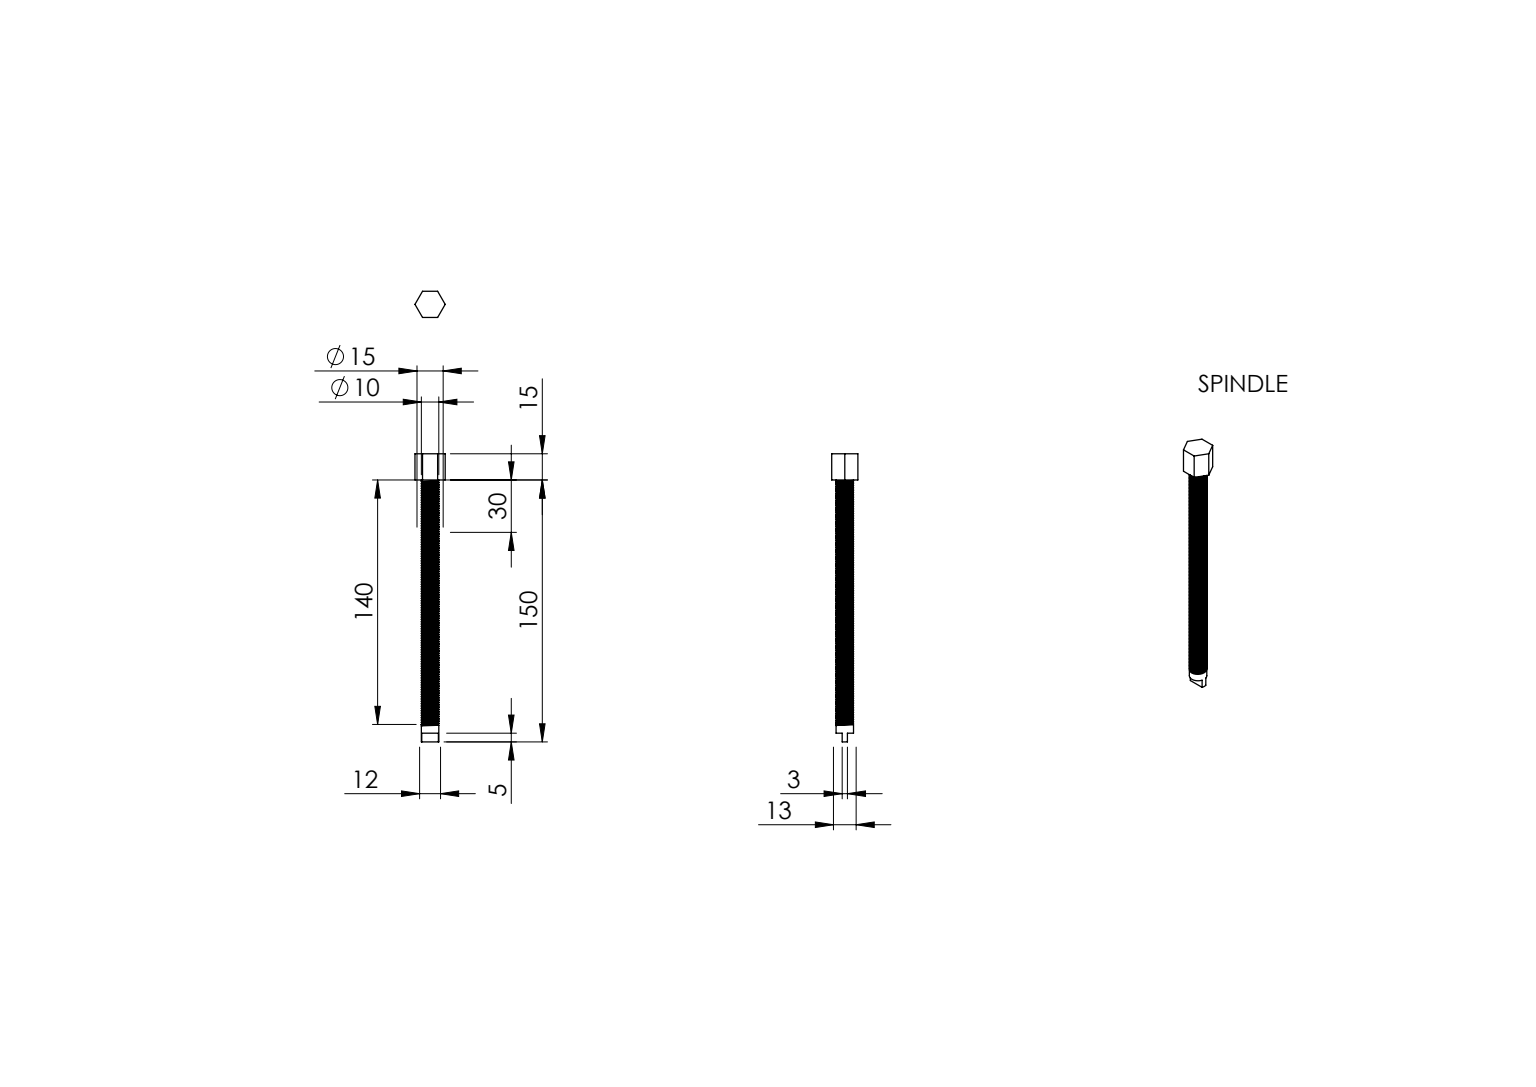
ISO-10303-21;
HEADER;
FILE_DESCRIPTION (('STEP AP214'),
    '1' );
FILE_NAME ('spindle.step',
    '2026-10-25T05:52:03',
    ( '' ),
    ( '' ),
    'SwSTEP 2.0',
    'SolidWorks 2026',
    '' );
FILE_SCHEMA (( 'AUTOMOTIVE_DESIGN' ));
ENDSEC;

DATA;
#2=AXIS2_PLACEMENT_3D ( 'NONE', #55045, #55372, #11606 ) ;
#7=ADVANCED_FACE ( 'NONE', ( #40534 ), #45685, .T. ) ;
#11=CARTESIAN_POINT ( 'NONE',  ( -4.458734124999999437, -91.56249999863440792, 0.000000000000000000 ) ) ;
#13=ORIENTED_EDGE ( 'NONE', *, *, #42928, .F. ) ;
#14=CARTESIAN_POINT ( 'NONE',  ( 4.330127018922154569, 30.00000000000000000, -7.499999999999971578 ) ) ;
#17=CARTESIAN_POINT ( 'NONE',  ( -6.972266317189433020E-16, -38.25000000000000000, -5.000000000000000000 ) ) ;
#19=CARTESIAN_POINT ( 'NONE',  ( -2.229367062499996610, 0.8541666680322613781, 3.861377020970582219 ) ) ;
#20=CARTESIAN_POINT ( 'NONE',  ( 0.000000000000000000, -120.0000000000000000, 0.000000000000000000 ) ) ;
#21=CARTESIAN_POINT ( 'NONE',  ( -3.152548672688508926E-16, -17.81249999863440792, -5.148502694627439702 ) ) ;
#22=EDGE_CURVE ( 'NONE', #55212, #17569, #39568, .T. ) ;
#25=LINE ( 'NONE', #58862, #59314 ) ;
#27=( BOUNDED_CURVE ( )  B_SPLINE_CURVE ( 2, ( #54507, #43875, #30044, #63521, #19445, #58375, #54824, #39058, #10756 ),
 .UNSPECIFIED., .F., .F. ) 
 B_SPLINE_CURVE_WITH_KNOTS ( ( 3, 2, 2, 2, 3 ),
 ( 0.2339285714285714302, 0.2345238095238095233, 0.2357142857142857095, 0.2369047619047618958, 0.2374999999999999889 ),
 .UNSPECIFIED. ) 
 CURVE ( )  GEOMETRIC_REPRESENTATION_ITEM ( )  RATIONAL_B_SPLINE_CURVE ( ( 0.9330127018922194093, 0.9330127018922194093, 1.000000000000000000, 0.8660254037844387076, 1.000000000000000000, 0.8660254037844387076, 1.000000000000000000, 0.9330127018922194093, 0.9330127018922194093 ) ) 
 REPRESENTATION_ITEM ( '' )  );
#28=CARTESIAN_POINT ( 'NONE',  ( 2.229367062500001939, 22.77083333469892423, 3.861377020970579999 ) ) ;
#29=ORIENTED_EDGE ( 'NONE', *, *, #3156, .T. ) ;
#30=CARTESIAN_POINT ( 'NONE',  ( -2.229367062499996610, -99.14583333196773651, 3.861377020970582219 ) ) ;
#32=CARTESIAN_POINT ( 'NONE',  ( -5.000000000000000000, -103.9583333306021444, -2.886751345948128211 ) ) ;
#33=CARTESIAN_POINT ( 'NONE',  ( -2.229367062499996610, -13.14583333196774007, 3.861377020970582219 ) ) ;
#36=CARTESIAN_POINT ( 'NONE',  ( 1.975475456537005874E-15, -87.75000000000001421, 5.000000000000000000 ) ) ;
#37=CARTESIAN_POINT ( 'NONE',  ( -3.535250795749689387E-16, -41.12499999726880162, -5.773502691896257311 ) ) ;
#39=CARTESIAN_POINT ( 'NONE',  ( -4.458734124999999437, 14.68750000136559386, 0.000000000000000000 ) ) ;
#41=VERTEX_POINT ( 'NONE', #30888 ) ;
#43=CARTESIAN_POINT ( 'NONE',  ( -4.458734124999999437, -60.31249999863440081, 0.000000000000000000 ) ) ;
#44=AXIS2_PLACEMENT_3D ( 'NONE', #51313, #36828, #41317 ) ;
#46=CARTESIAN_POINT ( 'NONE',  ( 5.000000000000000888, -109.4583333306021444, 2.886751345948126879 ) ) ;
#47=CARTESIAN_POINT ( 'NONE',  ( -5.000000000000000000, 6.999999999999999112, 0.000000000000000000 ) ) ;
#51=CARTESIAN_POINT ( 'NONE',  ( -4.458734124999998549, -53.22916666530107932, 2.574251347313722516 ) ) ;
#52=CARTESIAN_POINT ( 'NONE',  ( 5.000000000000000000, -87.29166666393548724, -2.886751345948129988 ) ) ;
#53=CARTESIAN_POINT ( 'NONE',  ( 4.458734124999999437, -32.81249999863440792, -5.460374474430324690E-16 ) ) ;
#56=CARTESIAN_POINT ( 'NONE',  ( -2.499999999999996447, -107.7083333306021444, 4.330127018922195425 ) ) ;
#58=CARTESIAN_POINT ( 'NONE',  ( -5.000000000000000000, -40.08333333333332860, -2.886751345948128211 ) ) ;
#61=ORIENTED_EDGE ( 'NONE', *, *, #4808, .T. ) ;
#62=CARTESIAN_POINT ( 'NONE',  ( -4.458734124999999437, -103.3958333319677365, -2.574251347313719407 ) ) ;
#63=CARTESIAN_POINT ( 'NONE',  ( -4.458734124999999437, 1.437500001365592972, 0.000000000000000000 ) ) ;
#70=ORIENTED_EDGE ( 'NONE', *, *, #62981, .F. ) ;
#71=CYLINDRICAL_SURFACE ( 'NONE', #27152, 5.000000000000000000 ) ;
#75=CARTESIAN_POINT ( 'NONE',  ( 2.229367062499998831, -23.89583333196773651, -3.861377020970580887 ) ) ;
#76=CARTESIAN_POINT ( 'NONE',  ( 1.464175926609780648E-14, 21.87500000273118062, -5.000000000000000000 ) ) ;
#84=ADVANCED_FACE ( 'NONE', ( #59208 ), #45044, .T. ) ;
#89=CARTESIAN_POINT ( 'NONE',  ( -2.229367062500000163, -75.72916666530106511, -3.861377020970580443 ) ) ;
#90=CARTESIAN_POINT ( 'NONE',  ( 0.000000000000000000, -120.0000000000000000, 5.000000000000000000 ) ) ;
#91=EDGE_CURVE ( 'NONE', #38750, #62586, #59395, .T. ) ;
#99=CARTESIAN_POINT ( 'NONE',  ( -2.229367062499996610, 2.604166668032259491, 3.861377020970582219 ) ) ;
#100=VERTEX_POINT ( 'NONE', #15137 ) ;
#102=CARTESIAN_POINT ( 'NONE',  ( -5.000000000000000000, -19.99999999999999645, 0.000000000000000000 ) ) ;
#103=CARTESIAN_POINT ( 'NONE',  ( -6.972266317189433020E-16, -41.12499999726880162, -5.000000000000000000 ) ) ;
#110=ADVANCED_FACE ( 'NONE', ( #11584 ), #11897, .T. ) ;
#111=CARTESIAN_POINT ( 'NONE',  ( 2.229367062500001939, -80.97916666530106511, 3.861377020970579999 ) ) ;
#113=CARTESIAN_POINT ( 'NONE',  ( 1.975475456537005874E-15, -0.6249999972688137229, 5.000000000000000000 ) ) ;
#114=CARTESIAN_POINT ( 'NONE',  ( -2.229367062499996610, 0.8541666680322613781, 3.861377020970582219 ) ) ;
#115=CARTESIAN_POINT ( 'NONE',  ( 5.000000000000000000, -83.41666666666667140, -2.886751345948129988 ) ) ;
#117=CARTESIAN_POINT ( 'NONE',  ( 4.458734125000001214, -63.14583333196774362, 2.574251347313718519 ) ) ;
#118=CARTESIAN_POINT ( 'NONE',  ( 5.000000000000000000, -24.37499999726881228, -6.123233995736766282E-16 ) ) ;
#120=CARTESIAN_POINT ( 'NONE',  ( 4.458734124999998549, 28.27083333469892779, -2.574251347313721627 ) ) ;
#121=CARTESIAN_POINT ( 'NONE',  ( -5.000000000000000000, -64.87499999726881583, 0.000000000000000000 ) ) ;
#123=CARTESIAN_POINT ( 'NONE',  ( -2.229367062499996610, -44.14583333196774362, 3.861377020970582219 ) ) ;
#124=CARTESIAN_POINT ( 'NONE',  ( 4.458734124999998549, -31.97916666530107577, -2.574251347313721627 ) ) ;
#127=CARTESIAN_POINT ( 'NONE',  ( -2.499999999999996447, 28.16666666666666785, 4.330127018922195425 ) ) ;
#129=CARTESIAN_POINT ( 'NONE',  ( -6.972266317189433020E-16, -50.24999999999999289, -5.000000000000000000 ) ) ;
#130=CARTESIAN_POINT ( 'NONE',  ( 4.458734124999998549, -37.72916666530107221, -2.574251347313721627 ) ) ;
#131=CARTESIAN_POINT ( 'NONE',  ( -2.500000000000000444, -73.04166666393548724, -4.330127018922193649 ) ) ;
#134=CARTESIAN_POINT ( 'NONE',  ( 9.457646018065525792E-16, -74.31249999863440792, 5.148502694627439702 ) ) ;
#139=CARTESIAN_POINT ( 'NONE',  ( -5.000000000000000000, -20.08333333333333215, -2.886751345948128211 ) ) ;
#143=VERTEX_POINT ( 'NONE', #12854 ) ;
#145=CARTESIAN_POINT ( 'NONE',  ( 5.000000000000000000, 22.70833333606451632, -2.886751345948129988 ) ) ;
#146=CARTESIAN_POINT ( 'NONE',  ( 1.975475456537005874E-15, 4.375000002731185056, 5.000000000000000000 ) ) ;
#151=CARTESIAN_POINT ( 'NONE',  ( -4.999999999999998224, -40.79166666393548724, 2.886751345948131764 ) ) ;
#152=CARTESIAN_POINT ( 'NONE',  ( -1.339745962155610925, 0.2053418012614791066, 5.000000000000000000 ) ) ;
#155=CARTESIAN_POINT ( 'NONE',  ( 4.458734124999999437, -23.81249999863440436, -5.460374474430324690E-16 ) ) ;
#156=CARTESIAN_POINT ( 'NONE',  ( -1.339745962155613812, -72.08034179853027013, -5.000000000000000000 ) ) ;
#159=( BOUNDED_CURVE ( )  B_SPLINE_CURVE ( 2, ( #57542, #18604, #23441, #33707, #13470, #33086, #62682, #47554, #43658 ),
 .UNSPECIFIED., .F., .F. ) 
 B_SPLINE_CURVE_WITH_KNOTS ( ( 3, 2, 2, 2, 3 ),
 ( 0.8089285714285714413, 0.8095238095238095344, 0.8107142857142857206, 0.8119047619047619069, 0.8125000000000000000 ),
 .UNSPECIFIED. ) 
 CURVE ( )  GEOMETRIC_REPRESENTATION_ITEM ( )  RATIONAL_B_SPLINE_CURVE ( ( 0.9330127018922194093, 0.9330127018922194093, 1.000000000000000000, 0.8660254037844387076, 1.000000000000000000, 0.8660254037844387076, 1.000000000000000000, 0.9330127018922194093, 0.9330127018922194093 ) ) 
 REPRESENTATION_ITEM ( '' )  );
#167=ORIENTED_EDGE ( 'NONE', *, *, #56942, .T. ) ;
#172=EDGE_LOOP ( 'NONE', ( #31219, #33556, #46683, #22321 ) ) ;
#174=CARTESIAN_POINT ( 'NONE',  ( -3.152548672688508926E-16, 18.43750000136559564, -5.148502694627439702 ) ) ;
#182=CARTESIAN_POINT ( 'NONE',  ( 9.457646018065525792E-16, -58.06249999863440081, 5.148502694627439702 ) ) ;
#183=DIRECTION ( 'NONE',  ( -0.000000000000000000, 1.000000000000000000, -0.000000000000000000 ) ) ;
#184=CARTESIAN_POINT ( 'NONE',  ( -2.229367062499996610, 16.85416666803225993, 3.861377020970582219 ) ) ;
#186=ADVANCED_FACE ( 'NONE', ( #26707 ), #62074, .T. ) ;
#187=CARTESIAN_POINT ( 'NONE',  ( 4.458734124999998549, -51.97916666530107221, -2.574251347313721627 ) ) ;
#188=CARTESIAN_POINT ( 'NONE',  ( 5.000000000000000000, -11.37499999726881583, -6.123233995736766282E-16 ) ) ;
#191=CARTESIAN_POINT ( 'NONE',  ( -2.500000000000000444, -74.16666666666665719, -4.330127018922193649 ) ) ;
#192=CARTESIAN_POINT ( 'NONE',  ( -4.458734124999997661, -109.2291666653010509, 2.574251347313722516 ) ) ;
#193=CARTESIAN_POINT ( 'NONE',  ( 4.458734124999998549, -12.97916666530107399, -2.574251347313721627 ) ) ;
#194=ORIENTED_EDGE ( 'NONE', *, *, #3576, .F. ) ;
#195=CARTESIAN_POINT ( 'NONE',  ( 1.339745962155608039, 23.29465819873852084, 5.000000000000003553 ) ) ;
#196=CARTESIAN_POINT ( 'NONE',  ( -2.229367062500000163, -96.47916666530105090, -3.861377020970580443 ) ) ;
#198=CARTESIAN_POINT ( 'NONE',  ( 9.457646018065525792E-16, -97.31249999863440792, 5.148502694627439702 ) ) ;
#199=FACE_OUTER_BOUND ( 'NONE', #51701, .T. ) ;
#200=CARTESIAN_POINT ( 'NONE',  ( -2.499999999999996447, -58.70833333060214443, 4.330127018922195425 ) ) ;
#204=CARTESIAN_POINT ( 'NONE',  ( -2.229367062500000163, -16.47916666530107577, -3.861377020970580443 ) ) ;
#205=CARTESIAN_POINT ( 'NONE',  ( -3.152548672688508926E-16, 4.187500001365595637, -5.148502694627439702 ) ) ;
#206=CARTESIAN_POINT ( 'NONE',  ( 9.457646018065525792E-16, -61.31249999863440792, 5.148502694627439702 ) ) ;
#211=CARTESIAN_POINT ( 'NONE',  ( -2.500000000000000444, -4.166666666666666075, -4.330127018922193649 ) ) ;
#212=ORIENTED_EDGE ( 'NONE', *, *, #23608, .F. ) ;
#216=DIRECTION ( 'NONE',  ( -0.000000000000000000, 1.000000000000000000, -0.000000000000000000 ) ) ;
#217=CARTESIAN_POINT ( 'NONE',  ( 2.229367062500001939, -84.97916666530107932, 3.861377020970579999 ) ) ;
#218=CARTESIAN_POINT ( 'NONE',  ( -2.229367062499996610, 19.60416666803225993, 3.861377020970582219 ) ) ;
#220=CARTESIAN_POINT ( 'NONE',  ( -4.999999999999998224, -88.79166666393548724, 2.886751345948131764 ) ) ;
#221=CYLINDRICAL_SURFACE ( 'NONE', #8092, 5.000000000000000000 ) ;
#224=CARTESIAN_POINT ( 'NONE',  ( -3.535250795749689387E-16, -77.25000000000000000, -5.773502691896257311 ) ) ;
#227=DIRECTION ( 'NONE',  ( 0.000000000000000000, 0.000000000000000000, 1.000000000000000000 ) ) ;
#228=ORIENTED_EDGE ( 'NONE', *, *, #38170, .T. ) ;
#241=CARTESIAN_POINT ( 'NONE',  ( 2.229367062499998831, -55.89583333196773651, -3.861377020970580887 ) ) ;
#245=ORIENTED_EDGE ( 'NONE', *, *, #34105, .T. ) ;
#248=VERTEX_POINT ( 'NONE', #17988 ) ;
#251=CARTESIAN_POINT ( 'NONE',  ( 2.229367062500001939, -104.2291666653010651, 3.861377020970579999 ) ) ;
#256=CARTESIAN_POINT ( 'NONE',  ( -4.458734124999997661, -41.22916666530107932, 2.574251347313722516 ) ) ;
#258=( BOUNDED_CURVE ( )  B_SPLINE_CURVE ( 2, ( #61184, #52477, #22580, #23193, #34020, #53641, #56988, #29181, #48808 ),
 .UNSPECIFIED., .F., .F. ) 
 B_SPLINE_CURVE_WITH_KNOTS ( ( 3, 2, 2, 2, 3 ),
 ( 0.2267857142857142849, 0.2273809523809523780, 0.2285714285714285643, 0.2297619047619047505, 0.2303571428571428714 ),
 .UNSPECIFIED. ) 
 CURVE ( )  GEOMETRIC_REPRESENTATION_ITEM ( )  RATIONAL_B_SPLINE_CURVE ( ( 0.9330127018922194093, 0.9330127018922194093, 1.000000000000000000, 0.8660254037844387076, 1.000000000000000000, 0.8660254037844387076, 1.000000000000000000, 0.9330127018922178550, 0.9330127018922194093 ) ) 
 REPRESENTATION_ITEM ( '' )  );
#260=CARTESIAN_POINT ( 'NONE',  ( 2.500000000000002220, 2.458333336064519870, 4.330127018922192761 ) ) ;
#261=CARTESIAN_POINT ( 'NONE',  ( -3.152548672688508926E-16, -11.56249999863440792, -5.148502694627439702 ) ) ;
#262=CARTESIAN_POINT ( 'NONE',  ( -4.458734124999999437, -101.5624999986344079, 0.000000000000000000 ) ) ;
#265=CARTESIAN_POINT ( 'NONE',  ( 4.458734125000001214, -33.14583333196774362, 2.574251347313718519 ) ) ;
#266=CARTESIAN_POINT ( 'NONE',  ( 1.060575238724906964E-15, 7.375000002731186832, 5.773502691896257311 ) ) ;
#270=DIRECTION ( 'NONE',  ( -0.000000000000000000, 1.000000000000000000, -0.000000000000000000 ) ) ;
#273=CARTESIAN_POINT ( 'NONE',  ( 4.458734124999998549, 6.020833334698928674, -2.574251347313721627 ) ) ;
#276=CARTESIAN_POINT ( 'NONE',  ( 1.339745962155615144, 9.294658198738520838, 4.999999999999999112 ) ) ;
#277=CARTESIAN_POINT ( 'NONE',  ( 5.000000000000000000, -96.41666666666664298, -2.886751345948129988 ) ) ;
#278=CARTESIAN_POINT ( 'NONE',  ( -2.229367062499996610, -29.14583333196774007, 3.861377020970582219 ) ) ;
#279=CARTESIAN_POINT ( 'NONE',  ( -4.999999999999998224, -35.91666666666666430, 2.886751345948131764 ) ) ;
#280=CARTESIAN_POINT ( 'NONE',  ( -3.152548672688508926E-16, -79.81249999863440792, -5.148502694627439702 ) ) ;
#282=CARTESIAN_POINT ( 'NONE',  ( 0.000000000000000000, -120.0000000000000000, 0.000000000000000000 ) ) ;
#284=CARTESIAN_POINT ( 'NONE',  ( -3.152548672688508926E-16, -3.562499998634408360, -5.148502694627439702 ) ) ;
#285=CARTESIAN_POINT ( 'NONE',  ( 9.457646018065525792E-16, 21.68750000136559208, 5.148502694627439702 ) ) ;
#286=CARTESIAN_POINT ( 'NONE',  ( 9.457646018065525792E-16, -42.31249999863440081, 5.148502694627439702 ) ) ;
#287=DIRECTION ( 'NONE',  ( 0.000000000000000000, 0.000000000000000000, 1.000000000000000000 ) ) ;
#291=CARTESIAN_POINT ( 'NONE',  ( 4.458734124999998549, -71.72916666530107932, -2.574251347313721627 ) ) ;
#292=CARTESIAN_POINT ( 'NONE',  ( 1.060575238724906964E-15, -104.6249999972688158, 5.773502691896257311 ) ) ;
#293=ADVANCED_FACE ( 'NONE', ( #61447 ), #37614, .T. ) ;
#295=CARTESIAN_POINT ( 'NONE',  ( -2.499999999999996447, 10.16666666666666785, 4.330127018922195425 ) ) ;
#296=CARTESIAN_POINT ( 'NONE',  ( -4.330127018922205195, 45.00000000000000000, -7.499999999999943157 ) ) ;
#298=CARTESIAN_POINT ( 'NONE',  ( 1.060575238724906964E-15, -58.75000000000000000, 5.773502691896257311 ) ) ;
#299=DIRECTION ( 'NONE',  ( -0.000000000000000000, 1.000000000000000000, -0.000000000000000000 ) ) ;
#302=CARTESIAN_POINT ( 'NONE',  ( 2.499999999999998668, -67.33333333333332860, -4.330127018922193649 ) ) ;
#309=ORIENTED_EDGE ( 'NONE', *, *, #57908, .T. ) ;
#310=CARTESIAN_POINT ( 'NONE',  ( -2.500000000000000444, -24.16666666666666430, -4.330127018922193649 ) ) ;
#311=CARTESIAN_POINT ( 'NONE',  ( 5.000000000000000000, -98.50000000000000000, -6.123233995736766282E-16 ) ) ;
#313=ORIENTED_EDGE ( 'NONE', *, *, #36524, .T. ) ;
#317=CARTESIAN_POINT ( 'NONE',  ( -3.152548672688508926E-16, -38.81249999863440081, -5.148502694627439702 ) ) ;
#318=CARTESIAN_POINT ( 'NONE',  ( -6.972266317189433020E-16, -68.12499999726881583, -5.000000000000000000 ) ) ;
#326=CARTESIAN_POINT ( 'NONE',  ( -4.458734124999999437, -88.64583333196773651, -2.574251347313719407 ) ) ;
#327=CARTESIAN_POINT ( 'NONE',  ( 6.123233995736766282E-16, -120.0000000000000000, -5.000000000000000000 ) ) ;
#329=CARTESIAN_POINT ( 'NONE',  ( -6.972266317189433020E-16, -19.12499999726880873, -5.000000000000000000 ) ) ;
#330=FACE_OUTER_BOUND ( 'NONE', #56792, .T. ) ;
#333=ORIENTED_EDGE ( 'NONE', *, *, #57023, .T. ) ;
#334=( BOUNDED_CURVE ( )  B_SPLINE_CURVE ( 2, ( #33009, #33633, #47175, #33318, #13071, #4059, #62915, #32690, #52322 ),
 .UNSPECIFIED., .F., .F. ) 
 B_SPLINE_CURVE_WITH_KNOTS ( ( 3, 2, 2, 2, 3 ),
 ( 0.05892857142857142738, 0.05952380952380952051, 0.06071428571428571369, 0.06190476190476190688, 0.06250000000000000000 ),
 .UNSPECIFIED. ) 
 CURVE ( )  GEOMETRIC_REPRESENTATION_ITEM ( )  RATIONAL_B_SPLINE_CURVE ( ( 0.9330127018922194093, 0.9330127018922194093, 1.000000000000000000, 0.8660254037844387076, 1.000000000000000000, 0.8660254037844387076, 1.000000000000000000, 0.9330127018922194093, 0.9330127018922194093 ) ) 
 REPRESENTATION_ITEM ( '' )  );
#335=CARTESIAN_POINT ( 'NONE',  ( -3.152548672688508926E-16, 5.437500001365592084, -5.148502694627439702 ) ) ;
#336=CARTESIAN_POINT ( 'NONE',  ( 2.500000000000002220, -1.541666663935480130, 4.330127018922192761 ) ) ;
#337=CARTESIAN_POINT ( 'NONE',  ( -4.458734124999998549, -17.47916666530106866, 2.574251347313722516 ) ) ;
#342=CARTESIAN_POINT ( 'NONE',  ( -4.458734124999999437, 21.35416666803225993, -2.574251347313719407 ) ) ;
#344=CARTESIAN_POINT ( 'NONE',  ( -4.458734124999999437, -97.31249999863440792, 0.000000000000000000 ) ) ;
#345=CARTESIAN_POINT ( 'NONE',  ( 1.339745962155612702, -47.29465819873852439, -5.000000000000000000 ) ) ;
#346=CARTESIAN_POINT ( 'NONE',  ( -2.499999999999996447, -103.7083333306021444, 4.330127018922195425 ) ) ;
#347=CARTESIAN_POINT ( 'NONE',  ( -3.152548672688508926E-16, -14.56249999863440436, -5.148502694627439702 ) ) ;
#350=CARTESIAN_POINT ( 'NONE',  ( -2.500000000000000444, -88.16666666666665719, -4.330127018922193649 ) ) ;
#351=CARTESIAN_POINT ( 'NONE',  ( 2.499999999999998668, -40.20833333060214443, -4.330127018922193649 ) ) ;
#353=CARTESIAN_POINT ( 'NONE',  ( -2.229367062500000163, 11.52083333469892601, -3.861377020970580443 ) ) ;
#354=CARTESIAN_POINT ( 'NONE',  ( 5.000000000000000888, -51.45833333060214443, 2.886751345948126879 ) ) ;
#357=CARTESIAN_POINT ( 'NONE',  ( -4.458734124999998549, -64.22916666530107932, 2.574251347313722516 ) ) ;
#358=ORIENTED_EDGE ( 'NONE', *, *, #35301, .F. ) ;
#361=CARTESIAN_POINT ( 'NONE',  ( -4.999999999999999112, 2.083333333333333037, 2.886751345948131764 ) ) ;
#363=CARTESIAN_POINT ( 'NONE',  ( -5.000000000000000000, -59.95833333060214443, -2.886751345948128211 ) ) ;
#364=CARTESIAN_POINT ( 'NONE',  ( -4.458734124999999437, -54.39583333196773651, -2.574251347313719407 ) ) ;
#365=CARTESIAN_POINT ( 'NONE',  ( 2.499999999999998668, -87.20833333060214443, -4.330127018922193649 ) ) ;
#367=CARTESIAN_POINT ( 'NONE',  ( 2.229367062500001939, -31.97916666530106866, 3.861377020970579999 ) ) ;
#368=CARTESIAN_POINT ( 'NONE',  ( -5.000000000000000000, 20.12500000273118772, 0.000000000000000000 ) ) ;
#370=CARTESIAN_POINT ( 'NONE',  ( -2.500000000000000444, -108.0416666639354730, -4.330127018922193649 ) ) ;
#372=CARTESIAN_POINT ( 'NONE',  ( -4.999999999999999112, -42.91666666666665719, 2.886751345948131764 ) ) ;
#375=EDGE_LOOP ( 'NONE', ( #48769, #4276, #28632, #46133 ) ) ;
#376=CARTESIAN_POINT ( 'NONE',  ( 4.458734124999999437, -100.8124999986344079, -5.460374474430324690E-16 ) ) ;
#377=CARTESIAN_POINT ( 'NONE',  ( -4.458734124999999437, 3.437500001365594748, 0.000000000000000000 ) ) ;
#378=CARTESIAN_POINT ( 'NONE',  ( 1.339745962155499015, -59.70534180126147561, 5.000000000000065725 ) ) ;
#382=AXIS2_PLACEMENT_3D ( 'NONE', #9332, #48570, #38915 ) ;
#383=FACE_BOUND ( 'NONE', #44585, .T. ) ;
#387=CARTESIAN_POINT ( 'NONE',  ( -4.999999999999998224, -10.91666666666666607, 2.886751345948131764 ) ) ;
#388=DIRECTION ( 'NONE',  ( -0.000000000000000000, 1.000000000000000000, -0.000000000000000000 ) ) ;
#393=CARTESIAN_POINT ( 'NONE',  ( 0.000000000000000000, -120.0000000000000000, 0.000000000000000000 ) ) ;
#394=CARTESIAN_POINT ( 'NONE',  ( -3.152548672688508926E-16, -22.81249999863440436, -5.148502694627439702 ) ) ;
#403=CARTESIAN_POINT ( 'NONE',  ( -5.000000000000000000, -82.87499999726881583, 0.000000000000000000 ) ) ;
#405=CARTESIAN_POINT ( 'NONE',  ( -2.229367062499996610, -71.39583333196773651, 3.861377020970582219 ) ) ;
#410=CARTESIAN_POINT ( 'NONE',  ( 5.000000000000000000, -31.37499999726880873, -6.123233995736766282E-16 ) ) ;
#413=CARTESIAN_POINT ( 'NONE',  ( -3.152548672688508926E-16, -4.812499998634402587, -5.148502694627439702 ) ) ;
#416=CARTESIAN_POINT ( 'NONE',  ( -1.339745962155613812, -45.20534180126146850, -5.000000000000000000 ) ) ;
#420=ORIENTED_EDGE ( 'NONE', *, *, #17481, .T. ) ;
#421=CARTESIAN_POINT ( 'NONE',  ( -4.458734124999997661, -81.22916666530106511, 2.574251347313722516 ) ) ;
#423=CARTESIAN_POINT ( 'NONE',  ( 2.229367062500001939, 1.020833334698927120, 3.861377020970579999 ) ) ;
#424=CARTESIAN_POINT ( 'NONE',  ( 5.000000000000000000, -86.50000000000000000, -6.123233995736766282E-16 ) ) ;
#426=CARTESIAN_POINT ( 'NONE',  ( 9.457646018065525792E-16, -63.31249999863440081, 5.148502694627439702 ) ) ;
#427=CARTESIAN_POINT ( 'NONE',  ( 5.000000000000000000, -27.37499999726880873, -6.123233995736766282E-16 ) ) ;
#430=CARTESIAN_POINT ( 'NONE',  ( 2.500000000000002220, -49.66666666666666430, 4.330127018922192761 ) ) ;
#431=( NAMED_UNIT ( * ) SI_UNIT ( $, .STERADIAN. ) SOLID_ANGLE_UNIT ( ) );
#432=CARTESIAN_POINT ( 'NONE',  ( -2.229367062500000163, -45.47916666530106511, -3.861377020970580443 ) ) ;
#433=CARTESIAN_POINT ( 'NONE',  ( 9.457646018065525792E-16, -30.31249999863440436, 5.148502694627439702 ) ) ;
#436=CARTESIAN_POINT ( 'NONE',  ( -4.999999999999999112, 19.08333333333333570, 2.886751345948131764 ) ) ;
#438=CARTESIAN_POINT ( 'NONE',  ( 0.000000000000000000, -120.0000000000000000, 5.000000000000000000 ) ) ;
#439=CARTESIAN_POINT ( 'NONE',  ( 2.229367062500001939, -35.97916666530107221, 3.861377020970579999 ) ) ;
#440=CARTESIAN_POINT ( 'NONE',  ( -3.535250795749689387E-16, -73.12499999726881583, -5.773502691896257311 ) ) ;
#444=CARTESIAN_POINT ( 'NONE',  ( 2.500000000000002220, -37.66666666666666430, 4.330127018922192761 ) ) ;
#446=CARTESIAN_POINT ( 'NONE',  ( -4.458734124999999437, -82.56249999863440792, 0.000000000000000000 ) ) ;
#450=DIRECTION ( 'NONE',  ( 0.000000000000000000, 0.000000000000000000, 1.000000000000000000 ) ) ;
#452=CARTESIAN_POINT ( 'NONE',  ( 2.500000000000002220, -26.66666666666666430, 4.330127018922192761 ) ) ;
#454=VERTEX_POINT ( 'NONE', #32796 ) ;
#456=VERTEX_POINT ( 'NONE', #52425 ) ;
#458=CARTESIAN_POINT ( 'NONE',  ( 5.000000000000000000, 19.62500000273118772, -6.123233995736766282E-16 ) ) ;
#459=( BOUNDED_CURVE ( )  B_SPLINE_CURVE ( 2, ( #55262, #6684, #6374, #54615, #16335, #1554, #60409, #25980, #45595 ),
 .UNSPECIFIED., .F., .F. ) 
 B_SPLINE_CURVE_WITH_KNOTS ( ( 3, 2, 2, 2, 3 ),
 ( 0.03035714285714285685, 0.03095238095238095344, 0.03214285714285713969, 0.03333333333333333287, 0.03392857142857143293 ),
 .UNSPECIFIED. ) 
 CURVE ( )  GEOMETRIC_REPRESENTATION_ITEM ( )  RATIONAL_B_SPLINE_CURVE ( ( 0.9330127018922194093, 0.9330127018922194093, 1.000000000000000000, 0.8660254037844387076, 1.000000000000000000, 0.8660254037844387076, 1.000000000000000000, 0.9330127018922189652, 0.9330127018922194093 ) ) 
 REPRESENTATION_ITEM ( '' )  );
#460=CARTESIAN_POINT ( 'NONE',  ( 5.000000000000000000, -48.37499999726880873, -6.123233995736766282E-16 ) ) ;
#462=ADVANCED_FACE ( 'NONE', ( #8357 ), #52728, .T. ) ;
#467=CARTESIAN_POINT ( 'NONE',  ( -2.500000000000000444, -0.1666666666666656582, -4.330127018922193649 ) ) ;
#468=EDGE_CURVE ( 'NONE', #15325, #14586, #24076, .T. ) ;
#469=DIRECTION ( 'NONE',  ( -0.000000000000000000, 1.000000000000000000, -0.000000000000000000 ) ) ;
#471=CARTESIAN_POINT ( 'NONE',  ( 4.458734124999999437, -19.81249999863440081, -5.460374474430324690E-16 ) ) ;
#479=ORIENTED_EDGE ( 'NONE', *, *, #43975, .F. ) ;
#480=CARTESIAN_POINT ( 'NONE',  ( -6.972266317189433020E-16, -87.25000000000001421, -5.000000000000000000 ) ) ;
#481=CARTESIAN_POINT ( 'NONE',  ( 5.000000000000000000, 11.70833333606451809, -2.886751345948130876 ) ) ;
#483=VERTEX_POINT ( 'NONE', #24090 ) ;
#486=CARTESIAN_POINT ( 'NONE',  ( 2.499999999999998668, -86.33333333333332860, -4.330127018922193649 ) ) ;
#488=ORIENTED_EDGE ( 'NONE', *, *, #59618, .T. ) ;
#489=CARTESIAN_POINT ( 'NONE',  ( -4.458734124999998549, 12.77083333469892601, 2.574251347313722516 ) ) ;
#494=CARTESIAN_POINT ( 'NONE',  ( 5.000000000000000000, -39.41666666666667851, -2.886751345948130876 ) ) ;
#496=CARTESIAN_POINT ( 'NONE',  ( 4.458734124999998549, -62.72916666530106511, -2.574251347313721627 ) ) ;
#498=CARTESIAN_POINT ( 'NONE',  ( 4.458734124999999437, 20.18750000136559208, -5.460374474430324690E-16 ) ) ;
#500=CARTESIAN_POINT ( 'NONE',  ( -4.458734124999999437, -50.56249999863440792, 0.000000000000000000 ) ) ;
#501=CARTESIAN_POINT ( 'NONE',  ( -2.500000000000000444, -12.04166666393547835, -4.330127018922193649 ) ) ;
#505=CARTESIAN_POINT ( 'NONE',  ( 1.975475456537005874E-15, -64.62499999726880162, 5.000000000000000000 ) ) ;
#506=CARTESIAN_POINT ( 'NONE',  ( -2.229367062499996610, -15.39583333196773651, 3.861377020970582219 ) ) ;
#508=CARTESIAN_POINT ( 'NONE',  ( -1.336351044127974539E-14, 23.24999999999999645, 5.000000000000000000 ) ) ;
#509=CARTESIAN_POINT ( 'NONE',  ( -2.229367062500000163, -103.4791666653010651, -3.861377020970580443 ) ) ;
#511=CARTESIAN_POINT ( 'NONE',  ( -2.229367062500000163, -98.72916666530105090, -3.861377020970580443 ) ) ;
#512=CARTESIAN_POINT ( 'NONE',  ( 6.123233995736766282E-16, -120.0000000000000000, -5.000000000000000000 ) ) ;
#513=CARTESIAN_POINT ( 'NONE',  ( -3.535250795749689387E-16, -58.12499999726880162, -5.773502691896257311 ) ) ;
#519=CARTESIAN_POINT ( 'NONE',  ( 2.229367062500001939, -15.97916666530107399, 3.861377020970579999 ) ) ;
#520=CARTESIAN_POINT ( 'NONE',  ( -4.458734124999999437, 5.437500001365592972, 0.000000000000000000 ) ) ;
#521=CARTESIAN_POINT ( 'NONE',  ( -4.458734124999997661, -62.47916666530106511, 2.574251347313722516 ) ) ;
#526=CARTESIAN_POINT ( 'NONE',  ( 1.060575238724906964E-15, -6.749999999999999112, 5.773502691896257311 ) ) ;
#527=EDGE_LOOP ( 'NONE', ( #5913, #22407, #27837, #31617 ) ) ;
#532=CARTESIAN_POINT ( 'NONE',  ( -4.458734124999998549, -93.22916666530107932, 2.574251347313722516 ) ) ;
#533=CARTESIAN_POINT ( 'NONE',  ( 9.457646018065525792E-16, 19.68750000136559208, 5.148502694627439702 ) ) ;
#534=( BOUNDED_CURVE ( )  B_SPLINE_CURVE ( 2, ( #52700, #32767, #28246, #52401, #4434, #8333, #37911, #43043, #33393 ),
 .UNSPECIFIED., .F., .F. ) 
 B_SPLINE_CURVE_WITH_KNOTS ( ( 3, 2, 2, 2, 3 ),
 ( 0.1982142857142857040, 0.1988095238095237971, 0.2000000000000000111, 0.2011904761904761973, 0.2017857142857142905 ),
 .UNSPECIFIED. ) 
 CURVE ( )  GEOMETRIC_REPRESENTATION_ITEM ( )  RATIONAL_B_SPLINE_CURVE ( ( 0.9330127018922194093, 0.9330127018922194093, 1.000000000000000000, 0.8660254037844387076, 1.000000000000000000, 0.8660254037844387076, 1.000000000000000000, 0.9330127018922194093, 0.9330127018922194093 ) ) 
 REPRESENTATION_ITEM ( '' )  );
#536=CARTESIAN_POINT ( 'NONE',  ( 1.975475456537005874E-15, -0.7499999999999996669, 5.000000000000000000 ) ) ;
#540=CARTESIAN_POINT ( 'NONE',  ( -2.499999999999996447, -74.83333333333332860, 4.330127018922195425 ) ) ;
#544=CARTESIAN_POINT ( 'NONE',  ( -4.999999999999998224, -97.91666666666667140, 2.886751345948131764 ) ) ;
#545=ORIENTED_EDGE ( 'NONE', *, *, #24179, .T. ) ;
#555=ORIENTED_EDGE ( 'NONE', *, *, #48721, .F. ) ;
#558=CARTESIAN_POINT ( 'NONE',  ( 4.458734125000001214, -60.14583333196774362, 2.574251347313718519 ) ) ;
#568=CARTESIAN_POINT ( 'NONE',  ( -4.458734124999998549, -105.4791666653010793, 2.574251347313722516 ) ) ;
#574=CARTESIAN_POINT ( 'NONE',  ( -4.458734124999999437, -44.31249999863440081, 0.000000000000000000 ) ) ;
#577=CARTESIAN_POINT ( 'NONE',  ( 2.229367062500001939, -46.97916666530106511, 3.861377020970579999 ) ) ;
#578=CARTESIAN_POINT ( 'NONE',  ( -2.499999999999996447, -70.83333333333332860, 4.330127018922195425 ) ) ;
#579=CARTESIAN_POINT ( 'NONE',  ( -4.458734124999999437, -10.39583333196773829, -2.574251347313719407 ) ) ;
#580=CARTESIAN_POINT ( 'NONE',  ( 2.499999999999998668, -100.3333333333333286, -4.330127018922193649 ) ) ;
#582=CARTESIAN_POINT ( 'NONE',  ( -2.229367062499996610, -33.39583333196772941, 3.861377020970582219 ) ) ;
#583=CARTESIAN_POINT ( 'NONE',  ( 1.060575238724906964E-15, 4.375000002731186832, 5.773502691896257311 ) ) ;
#586=( BOUNDED_CURVE ( )  B_SPLINE_CURVE ( 2, ( #13509, #41564, #52436, #23474, #18325, #8370, #57884, #43077, #62715 ),
 .UNSPECIFIED., .F., .F. ) 
 B_SPLINE_CURVE_WITH_KNOTS ( ( 3, 2, 2, 2, 3 ),
 ( 0.1375000000000000111, 0.1380952380952381042, 0.1392857142857142905, 0.1404761904761904767, 0.1410714285714285698 ),
 .UNSPECIFIED. ) 
 CURVE ( )  GEOMETRIC_REPRESENTATION_ITEM ( )  RATIONAL_B_SPLINE_CURVE ( ( 0.9330127018922194093, 0.9330127018922194093, 1.000000000000000000, 0.8660254037844387076, 1.000000000000000000, 0.8660254037844387076, 1.000000000000000000, 0.9330127018922194093, 0.9330127018922194093 ) ) 
 REPRESENTATION_ITEM ( '' )  );
#588=DIRECTION ( 'NONE',  ( 0.000000000000000000, 0.000000000000000000, 1.000000000000000000 ) ) ;
#591=CARTESIAN_POINT ( 'NONE',  ( -2.229367062500000163, -0.7291666653010709931, -3.861377020970580443 ) ) ;
#594=CARTESIAN_POINT ( 'NONE',  ( -6.972266317189433020E-16, -76.24999999999998579, -5.000000000000000000 ) ) ;
#595=CARTESIAN_POINT ( 'NONE',  ( -5.000000000000000000, -95.08333333333334281, -2.886751345948128211 ) ) ;
#596=CARTESIAN_POINT ( 'NONE',  ( 4.458734125000001214, -36.89583333196773651, 2.574251347313718519 ) ) ;
#597=CARTESIAN_POINT ( 'NONE',  ( -4.458734124999999437, -83.64583333196773651, -2.574251347313719407 ) ) ;
#601=EDGE_CURVE ( 'NONE', #58440, #60689, #40027, .T. ) ;
#602=CARTESIAN_POINT ( 'NONE',  ( -2.229367062499996610, -0.1458333319677394824, 3.861377020970582219 ) ) ;
#603=CARTESIAN_POINT ( 'NONE',  ( 9.457646018065525792E-16, 22.68750000136559564, 5.148502694627439702 ) ) ;
#604=CARTESIAN_POINT ( 'NONE',  ( -2.229367062500000163, -42.72916666530107932, -3.861377020970580443 ) ) ;
#607=AXIS2_PLACEMENT_3D ( 'NONE', #36007, #55638, #7380 ) ;
#611=CARTESIAN_POINT ( 'NONE',  ( -4.458734124999999437, -76.39583333196775072, -2.574251347313719407 ) ) ;
#612=CARTESIAN_POINT ( 'NONE',  ( -5.000000000000000000, -104.9583333306021444, -2.886751345948128211 ) ) ;
#615=CARTESIAN_POINT ( 'NONE',  ( -1.975475456537005874E-15, 28.25000000000000000, 5.000000000000000000 ) ) ;
#617=CARTESIAN_POINT ( 'NONE',  ( -5.000000000000000000, -61.08333333333333570, -2.886751345948128211 ) ) ;
#618=CARTESIAN_POINT ( 'NONE',  ( 1.975475456537005874E-15, -36.62499999726880873, 5.000000000000000000 ) ) ;
#621=CARTESIAN_POINT ( 'NONE',  ( 0.000000000000000000, -120.0000000000000000, 5.000000000000000000 ) ) ;
#622=CARTESIAN_POINT ( 'NONE',  ( -6.972266317189433020E-16, -71.12499999726878741, -5.000000000000000000 ) ) ;
#628=EDGE_LOOP ( 'NONE', ( #892, #35676, #47248, #5295 ) ) ;
#630=CARTESIAN_POINT ( 'NONE',  ( -5.000000000000000000, 11.12500000273118594, 0.000000000000000000 ) ) ;
#632=ORIENTED_EDGE ( 'NONE', *, *, #44976, .T. ) ;
#636=CARTESIAN_POINT ( 'NONE',  ( 9.457646018065525792E-16, -48.31249999863440081, 5.148502694627439702 ) ) ;
#637=CARTESIAN_POINT ( 'NONE',  ( 5.000000000000000000, -23.50000000000000000, -6.123233995736766282E-16 ) ) ;
#640=DIRECTION ( 'NONE',  ( -0.000000000000000000, 1.000000000000000000, -0.000000000000000000 ) ) ;
#646=CARTESIAN_POINT ( 'NONE',  ( -2.229367062500000163, -86.72916666530107932, -3.861377020970580443 ) ) ;
#648=ORIENTED_EDGE ( 'NONE', *, *, #24773, .F. ) ;
#649=CARTESIAN_POINT ( 'NONE',  ( 5.000000000000000000, -19.37499999726881583, -6.123233995736766282E-16 ) ) ;
#652=AXIS2_PLACEMENT_3D ( 'NONE', #63511, #37888, #42069 ) ;
#653=CARTESIAN_POINT ( 'NONE',  ( 1.339745962155612702, -38.29465819873851729, -5.000000000000000000 ) ) ;
#657=CARTESIAN_POINT ( 'NONE',  ( -3.152548672688508926E-16, 4.437500001365595637, -5.148502694627439702 ) ) ;
#659=CARTESIAN_POINT ( 'NONE',  ( -3.152548672688508926E-16, -15.81249999863440436, -5.148502694627439702 ) ) ;
#664=CARTESIAN_POINT ( 'NONE',  ( -4.458734124999999437, 19.35416666803225993, -2.574251347313719407 ) ) ;
#666=CARTESIAN_POINT ( 'NONE',  ( 4.458734124999999437, -96.81249999863440792, -5.460374474430324690E-16 ) ) ;
#669=CARTESIAN_POINT ( 'NONE',  ( 2.229367062499998831, -15.64583333196773651, -3.861377020970580887 ) ) ;
#670=CYLINDRICAL_SURFACE ( 'NONE', #55063, 5.000000000000000000 ) ;
#673=CARTESIAN_POINT ( 'NONE',  ( 5.000000000000000000, -42.29166666393548724, -2.886751345948129988 ) ) ;
#675=CARTESIAN_POINT ( 'NONE',  ( -2.229367062499996610, 12.85416666803226171, 3.861377020970582219 ) ) ;
#677=CARTESIAN_POINT ( 'NONE',  ( -5.000000000000000000, -47.87499999726880873, 0.000000000000000000 ) ) ;
#679=CARTESIAN_POINT ( 'NONE',  ( 2.229367062499998831, -60.64583333196774362, -3.861377020970580887 ) ) ;
#680=ORIENTED_EDGE ( 'NONE', *, *, #53512, .T. ) ;
#682=CARTESIAN_POINT ( 'NONE',  ( 5.000000000000000000, 4.583333333333331261, -2.886751345948129988 ) ) ;
#685=CARTESIAN_POINT ( 'NONE',  ( -4.458734124999999437, -54.31249999863440081, 0.000000000000000000 ) ) ;
#686=CARTESIAN_POINT ( 'NONE',  ( -2.500000000000000444, -88.04166666393548724, -4.330127018922193649 ) ) ;
#687=CARTESIAN_POINT ( 'NONE',  ( 4.458734124999999437, -35.81249999863440792, -5.460374474430324690E-16 ) ) ;
#691=CARTESIAN_POINT ( 'NONE',  ( 2.500000000000002220, -43.66666666666665719, 4.330127018922192761 ) ) ;
#692=CARTESIAN_POINT ( 'NONE',  ( -4.999999999999998224, -19.79166666393548013, 2.886751345948131764 ) ) ;
#693=CARTESIAN_POINT ( 'NONE',  ( 2.499999999999998668, -6.208333330602149758, -4.330127018922193649 ) ) ;
#694=ORIENTED_EDGE ( 'NONE', *, *, #17227, .T. ) ;
#695=CARTESIAN_POINT ( 'NONE',  ( -2.229367062500000163, -99.47916666530106511, -3.861377020970580443 ) ) ;
#696=CARTESIAN_POINT ( 'NONE',  ( 4.458734124999999437, 0.9375000013655959696, -5.460374474430324690E-16 ) ) ;
#698=DIRECTION ( 'NONE',  ( -0.000000000000000000, 1.000000000000000000, -0.000000000000000000 ) ) ;
#700=AXIS2_PLACEMENT_3D ( 'NONE', #30032, #21038, #15247 ) ;
#706=CARTESIAN_POINT ( 'NONE',  ( 5.000000000000000000, -33.41666666666666430, -2.886751345948130876 ) ) ;
#709=CARTESIAN_POINT ( 'NONE',  ( 1.975475456537005874E-15, -104.7500000000000000, 5.000000000000000000 ) ) ;
#712=CARTESIAN_POINT ( 'NONE',  ( -2.229367062500000163, -27.72916666530107221, -3.861377020970580443 ) ) ;
#718=( BOUNDED_CURVE ( )  B_SPLINE_CURVE ( 2, ( #63086, #49224, #9661, #38930, #18996, #18689, #48584, #44388, #39244 ),
 .UNSPECIFIED., .F., .F. ) 
 B_SPLINE_CURVE_WITH_KNOTS ( ( 3, 2, 2, 2, 3 ),
 ( 0.4874999999999999889, 0.4880952380952380820, 0.4892857142857142683, 0.4904761904761904545, 0.4910714285714285476 ),
 .UNSPECIFIED. ) 
 CURVE ( )  GEOMETRIC_REPRESENTATION_ITEM ( )  RATIONAL_B_SPLINE_CURVE ( ( 0.9330127018922194093, 0.9330127018922194093, 1.000000000000000000, 0.8660254037844387076, 1.000000000000000000, 0.8660254037844387076, 1.000000000000000000, 0.9330127018922194093, 0.9330127018922194093 ) ) 
 REPRESENTATION_ITEM ( '' )  );
#721=VERTEX_POINT ( 'NONE', #29522 ) ;
#724=CARTESIAN_POINT ( 'NONE',  ( 2.229367062500001939, -74.22916666530106511, 3.861377020970579999 ) ) ;
#729=CARTESIAN_POINT ( 'NONE',  ( 1.975475456537005874E-15, 8.249999999999998224, 5.000000000000000000 ) ) ;
#731=ADVANCED_FACE ( 'NONE', ( #5418 ), #49793, .T. ) ;
#732=CARTESIAN_POINT ( 'NONE',  ( 9.457646018065525792E-16, -6.312499998634404363, 5.148502694627439702 ) ) ;
#736=CARTESIAN_POINT ( 'NONE',  ( 1.339745962155615144, -91.70534180126148271, 4.999999999999999112 ) ) ;
#739=CARTESIAN_POINT ( 'NONE',  ( 1.339745962155612702, -47.16965819600733312, -5.000000000000000000 ) ) ;
#742=ORIENTED_EDGE ( 'NONE', *, *, #8306, .T. ) ;
#743=CARTESIAN_POINT ( 'NONE',  ( 4.458734125000000326, -83.89583333196773651, 2.574251347313718519 ) ) ;
#744=CARTESIAN_POINT ( 'NONE',  ( 2.229367062500001939, 2.020833334698927786, 3.861377020970579999 ) ) ;
#746=VECTOR ( 'NONE', #26616, 1000.000000000000000 ) ;
#747=CARTESIAN_POINT ( 'NONE',  ( 2.500000000000002220, -85.66666666666667140, 4.330127018922192761 ) ) ;
#750=CARTESIAN_POINT ( 'NONE',  ( -2.229367062499996610, -67.39583333196773651, 3.861377020970582219 ) ) ;
#752=CARTESIAN_POINT ( 'NONE',  ( 5.000000000000000000, -26.29166666393547658, -2.886751345948129988 ) ) ;
#753=EDGE_CURVE ( 'NONE', #43561, #42376, #30645, .T. ) ;
#756=CARTESIAN_POINT ( 'NONE',  ( -1.230605004983934782E-13, -37.62499999726881583, 5.000000000000000000 ) ) ;
#757=CARTESIAN_POINT ( 'NONE',  ( 0.000000000000000000, -120.0000000000000000, 0.000000000000000000 ) ) ;
#758=CARTESIAN_POINT ( 'NONE',  ( 4.458734125000001214, -44.89583333196774362, 2.574251347313718519 ) ) ;
#759=CARTESIAN_POINT ( 'NONE',  ( 4.458734125000000326, -32.14583333196773651, 2.574251347313718519 ) ) ;
#762=CARTESIAN_POINT ( 'NONE',  ( -4.999999999999999112, 18.08333333333333570, 2.886751345948131764 ) ) ;
#765=CARTESIAN_POINT ( 'NONE',  ( -3.152548672688508926E-16, -37.56249999863440792, -5.148502694627439702 ) ) ;
#766=CARTESIAN_POINT ( 'NONE',  ( 2.500000000000002220, -73.54166666393548724, 4.330127018922192761 ) ) ;
#767=EDGE_CURVE ( 'NONE', #37188, #62028, #48666, .T. ) ;
#771=CARTESIAN_POINT ( 'NONE',  ( 2.229367062500001939, -81.22916666530106511, 3.861377020970579999 ) ) ;
#775=CARTESIAN_POINT ( 'NONE',  ( 2.499999999999998668, -26.33333333333333215, -4.330127018922193649 ) ) ;
#781=CARTESIAN_POINT ( 'NONE',  ( 2.500000000000002220, 19.45833333606451632, 4.330127018922192761 ) ) ;
#787=EDGE_CURVE ( 'NONE', #24503, #3031, #46626, .T. ) ;
#788=CARTESIAN_POINT ( 'NONE',  ( 2.499999999999998668, 15.79166666939785202, -4.330127018922193649 ) ) ;
#792=CARTESIAN_POINT ( 'NONE',  ( 4.458734124999999437, -18.81249999863440792, -5.460374474430324690E-16 ) ) ;
#793=AXIS2_PLACEMENT_3D ( 'NONE', #44537, #6276, #15274 ) ;
#800=VERTEX_POINT ( 'NONE', #21492 ) ;
#801=CARTESIAN_POINT ( 'NONE',  ( 2.499999999999998668, 13.66666666666666785, -4.330127018922193649 ) ) ;
#803=ORIENTED_EDGE ( 'NONE', *, *, #57131, .F. ) ;
#805=CARTESIAN_POINT ( 'NONE',  ( -2.499999999999996447, -28.83333333333333570, 4.330127018922195425 ) ) ;
#810=CARTESIAN_POINT ( 'NONE',  ( 5.000000000000000888, 15.41666666666666607, 2.886751345948126879 ) ) ;
#813=ORIENTED_EDGE ( 'NONE', *, *, #11033, .F. ) ;
#815=EDGE_CURVE ( 'NONE', #26195, #10433, #15444, .T. ) ;
#817=CARTESIAN_POINT ( 'NONE',  ( 4.458734124999998549, 12.27083333469892423, -2.574251347313721627 ) ) ;
#823=CARTESIAN_POINT ( 'NONE',  ( 9.457646018065525792E-16, -66.06249999863440792, 5.148502694627439702 ) ) ;
#825=CARTESIAN_POINT ( 'NONE',  ( 9.457646018065525792E-16, 17.93750000136559208, 5.148502694627439702 ) ) ;
#829=CARTESIAN_POINT ( 'NONE',  ( -3.152548672688508926E-16, -47.81249999863440792, -5.148502694627439702 ) ) ;
#830=CARTESIAN_POINT ( 'NONE',  ( 2.499999999999998668, -9.208333330602146205, -4.330127018922193649 ) ) ;
#835=CARTESIAN_POINT ( 'NONE',  ( -6.972266317189433020E-16, -104.1249999972688016, -5.000000000000000000 ) ) ;
#836=CARTESIAN_POINT ( 'NONE',  ( -4.458734124999999437, -18.56249999863440792, 0.000000000000000000 ) ) ;
#839=( BOUNDED_CURVE ( )  B_SPLINE_CURVE ( 2, ( #2821, #22441, #42037, #31760, #12459, #52018, #26621, #2503, #46562 ),
 .UNSPECIFIED., .F., .F. ) 
 B_SPLINE_CURVE_WITH_KNOTS ( ( 3, 2, 2, 2, 3 ),
 ( 0.2232142857142857262, 0.2238095238095238193, 0.2250000000000000056, 0.2261904761904761918, 0.2267857142857142849 ),
 .UNSPECIFIED. ) 
 CURVE ( )  GEOMETRIC_REPRESENTATION_ITEM ( )  RATIONAL_B_SPLINE_CURVE ( ( 0.9330127018922194093, 0.9330127018922209636, 1.000000000000000000, 0.8660254037844387076, 1.000000000000000000, 0.8660254037844387076, 1.000000000000000000, 0.9330127018922194093, 0.9330127018922194093 ) ) 
 REPRESENTATION_ITEM ( '' )  );
#841=CARTESIAN_POINT ( 'NONE',  ( 9.457646018065525792E-16, -104.0624999986344221, 5.148502694627439702 ) ) ;
#844=CARTESIAN_POINT ( 'NONE',  ( 4.458734124999998549, -95.97916666530107932, -2.574251347313721627 ) ) ;
#846=CARTESIAN_POINT ( 'NONE',  ( 5.000000000000000000, -57.37499999726880162, -6.123233995736766282E-16 ) ) ;
#847=FACE_OUTER_BOUND ( 'NONE', #58279, .T. ) ;
#850=CARTESIAN_POINT ( 'NONE',  ( 2.229367062499998831, -19.64583333196774007, -3.861377020970580887 ) ) ;
#851=CARTESIAN_POINT ( 'NONE',  ( -2.229367062499996610, 6.604166668032259935, 3.861377020970582219 ) ) ;
#852=CARTESIAN_POINT ( 'NONE',  ( -3.152548672688508926E-16, -65.81249999863440792, -5.148502694627439702 ) ) ;
#853=CYLINDRICAL_SURFACE ( 'NONE', #14086, 5.000000000000000000 ) ;
#855=CYLINDRICAL_SURFACE ( 'NONE', #41979, 5.000000000000000000 ) ;
#857=CARTESIAN_POINT ( 'NONE',  ( -3.535250795749689387E-16, -11.25000000000000355, -5.773502691896257311 ) ) ;
#862=CARTESIAN_POINT ( 'NONE',  ( 2.499999999999998668, -38.20833333060213732, -4.330127018922193649 ) ) ;
#865=CARTESIAN_POINT ( 'NONE',  ( -6.972266317189433020E-16, -89.12499999726880162, -5.000000000000000000 ) ) ;
#866=CARTESIAN_POINT ( 'NONE',  ( -4.999999999999998224, -6.916666666666667851, 2.886751345948131764 ) ) ;
#867=CARTESIAN_POINT ( 'NONE',  ( -5.000000000000000000, 25.91666666666666430, -2.886751345948128211 ) ) ;
#869=CARTESIAN_POINT ( 'NONE',  ( 1.060575238724906964E-15, -76.74999999999998579, 5.773502691896257311 ) ) ;
#873=ORIENTED_EDGE ( 'NONE', *, *, #21285, .T. ) ;
#874=CARTESIAN_POINT ( 'NONE',  ( 5.000000000000000888, 26.41666666666666430, 2.886751345948126879 ) ) ;
#883=CARTESIAN_POINT ( 'NONE',  ( 2.229367062500001939, -60.22916666530106511, 3.861377020970579999 ) ) ;
#892=ORIENTED_EDGE ( 'NONE', *, *, #43199, .T. ) ;
#895=CARTESIAN_POINT ( 'NONE',  ( 4.458734124999999437, -108.0624999986343937, -5.460374474430324690E-16 ) ) ;
#901=CARTESIAN_POINT ( 'NONE',  ( 4.458734124999998549, -44.72916666530106511, -2.574251347313721627 ) ) ;
#903=ADVANCED_FACE ( 'NONE', ( #7018 ), #46246, .T. ) ;
#905=CARTESIAN_POINT ( 'NONE',  ( -4.458734124999999437, -49.39583333196772230, -2.574251347313719407 ) ) ;
#906=CARTESIAN_POINT ( 'NONE',  ( 4.648177544792955347E-16, 29.75000000000000355, -5.000000000000000000 ) ) ;
#908=CARTESIAN_POINT ( 'NONE',  ( 2.229367062499998831, -16.64583333196773651, -3.861377020970580887 ) ) ;
#909=EDGE_CURVE ( 'NONE', #38980, #44900, #59788, .T. ) ;
#910=AXIS2_PLACEMENT_3D ( 'NONE', #36745, #7477, #56375 ) ;
#911=CARTESIAN_POINT ( 'NONE',  ( -2.499999999999996447, -102.8333333333333286, 4.330127018922195425 ) ) ;
#913=CARTESIAN_POINT ( 'NONE',  ( -3.152548672688508926E-16, -32.81249999863440792, -5.148502694627439702 ) ) ;
#914=CARTESIAN_POINT ( 'NONE',  ( -2.500000000000000444, 5.958333336064519870, -4.330127018922193649 ) ) ;
#918=ADVANCED_FACE ( 'NONE', ( #38177 ), #14029, .T. ) ;
#921=DIRECTION ( 'NONE',  ( -0.000000000000000000, 1.000000000000000000, -0.000000000000000000 ) ) ;
#922=CARTESIAN_POINT ( 'NONE',  ( 4.458734124999998549, -2.979166665301069106, -2.574251347313721627 ) ) ;
#923=ORIENTED_EDGE ( 'NONE', *, *, #19611, .T. ) ;
#924=CARTESIAN_POINT ( 'NONE',  ( 1.975475456537005874E-15, 16.37500000273118417, 5.000000000000000000 ) ) ;
#925=ADVANCED_FACE ( 'NONE', ( #42359 ), #3454, .T. ) ;
#926=CARTESIAN_POINT ( 'NONE',  ( -6.972266317189433020E-16, 14.87500000273118594, -5.000000000000000000 ) ) ;
#927=CARTESIAN_POINT ( 'NONE',  ( -4.458734124999998549, -90.22916666530106511, 2.574251347313722516 ) ) ;
#928=CARTESIAN_POINT ( 'NONE',  ( 4.458734124999998549, -36.72916666530107221, -2.574251347313721627 ) ) ;
#930=CARTESIAN_POINT ( 'NONE',  ( -3.152548672688508926E-16, -82.81249999863442213, -5.148502694627439702 ) ) ;
#932=FACE_OUTER_BOUND ( 'NONE', #29020, .T. ) ;
#935=ADVANCED_FACE ( 'NONE', ( #47504 ), #8278, .T. ) ;
#936=CARTESIAN_POINT ( 'NONE',  ( 2.229367062499998831, -0.6458333319677399542, -3.861377020970580887 ) ) ;
#937=CARTESIAN_POINT ( 'NONE',  ( -4.458734124999999437, 19.35416666803225993, -2.574251347313719407 ) ) ;
#938=CARTESIAN_POINT ( 'NONE',  ( -2.229367062500000163, -49.72916666530107221, -3.861377020970580443 ) ) ;
#939=CARTESIAN_POINT ( 'NONE',  ( 1.339745962155612702, -11.29465819873852261, -5.000000000000000000 ) ) ;
#942=VERTEX_POINT ( 'NONE', #28513 ) ;
#944=AXIS2_PLACEMENT_3D ( 'NONE', #18569, #57192, #3782 ) ;
#946=CARTESIAN_POINT ( 'NONE',  ( -4.458734124999998549, -73.22916666530106511, 2.574251347313722516 ) ) ;
#947=CARTESIAN_POINT ( 'NONE',  ( -3.535250795749689387E-16, -109.1249999972687874, -5.773502691896257311 ) ) ;
#948=VECTOR ( 'NONE', #51988, 1000.000000000000000 ) ;
#950=CARTESIAN_POINT ( 'NONE',  ( 5.000000000000000888, -58.45833333060214443, 2.886751345948126879 ) ) ;
#951=DIRECTION ( 'NONE',  ( 0.000000000000000000, -1.000000000000000000, 0.000000000000000000 ) ) ;
#953=CARTESIAN_POINT ( 'NONE',  ( -4.999999999999999112, -58.91666666666665719, 2.886751345948131764 ) ) ;
#954=CARTESIAN_POINT ( 'NONE',  ( -5.000000000000000000, -75.08333333333332860, -2.886751345948128211 ) ) ;
#956=ORIENTED_EDGE ( 'NONE', *, *, #28390, .F. ) ;
#958=CARTESIAN_POINT ( 'NONE',  ( 1.975475456537005874E-15, -98.74999999999998579, 5.000000000000000000 ) ) ;
#969=VERTEX_POINT ( 'NONE', #23705 ) ;
#973=CARTESIAN_POINT ( 'NONE',  ( 2.229367062500001939, -48.22916666530106511, 3.861377020970579999 ) ) ;
#974=CARTESIAN_POINT ( 'NONE',  ( -4.999999999999998224, -15.79166666393548191, 2.886751345948131764 ) ) ;
#980=CARTESIAN_POINT ( 'NONE',  ( 0.000000000000000000, -120.0000000000000000, 0.000000000000000000 ) ) ;
#982=CARTESIAN_POINT ( 'NONE',  ( -4.458734124999998549, -94.47916666530106511, 2.574251347313722516 ) ) ;
#984=( BOUNDED_CURVE ( )  B_SPLINE_CURVE ( 2, ( #59068, #30097, #20468, #34605, #24972, #45223, #53603, #25608, #29453 ),
 .UNSPECIFIED., .F., .F. ) 
 B_SPLINE_CURVE_WITH_KNOTS ( ( 3, 2, 2, 2, 3 ),
 ( 0.8803571428571428381, 0.8809523809523809312, 0.8821428571428571175, 0.8833333333333333037, 0.8839285714285713969 ),
 .UNSPECIFIED. ) 
 CURVE ( )  GEOMETRIC_REPRESENTATION_ITEM ( )  RATIONAL_B_SPLINE_CURVE ( ( 0.9330127018922194093, 0.9330127018922194093, 1.000000000000000000, 0.8660254037844387076, 1.000000000000000000, 0.8660254037844387076, 1.000000000000000000, 0.9330127018922194093, 0.9330127018922194093 ) ) 
 REPRESENTATION_ITEM ( '' )  );
#986=CARTESIAN_POINT ( 'NONE',  ( 0.000000000000000000, -120.0000000000000000, 0.000000000000000000 ) ) ;
#991=EDGE_LOOP ( 'NONE', ( #39298, #2335, #23008, #40199 ) ) ;
#992=CARTESIAN_POINT ( 'NONE',  ( -2.229367062500000163, 4.520833334698926897, -3.861377020970580443 ) ) ;
#993=CARTESIAN_POINT ( 'NONE',  ( 2.500000000000002220, -50.54166666393547303, 4.330127018922192761 ) ) ;
#994=CARTESIAN_POINT ( 'NONE',  ( -2.229367062500000163, -19.72916666530107221, -3.861377020970580443 ) ) ;
#995=CARTESIAN_POINT ( 'NONE',  ( -2.500000000000000444, -101.1666666666666572, -4.330127018922193649 ) ) ;
#997=CARTESIAN_POINT ( 'NONE',  ( -5.000000000000000000, 4.041666669397852019, -2.886751345948128211 ) ) ;
#999=CARTESIAN_POINT ( 'NONE',  ( -2.229367062499996610, 16.60416666803225638, 3.861377020970582219 ) ) ;
#1000=ORIENTED_EDGE ( 'NONE', *, *, #7134, .T. ) ;
#1001=CARTESIAN_POINT ( 'NONE',  ( -1.339745962155613812, -19.08034179853029144, -5.000000000000000000 ) ) ;
#1002=LINE ( 'NONE', #6128, #35999 ) ;
#1003=CARTESIAN_POINT ( 'NONE',  ( -3.152548672688508926E-16, -21.56249999863440081, -5.148502694627439702 ) ) ;
#1007=CARTESIAN_POINT ( 'NONE',  ( -4.999999999999999112, -44.79166666393547303, 2.886751345948131764 ) ) ;
#1008=CARTESIAN_POINT ( 'NONE',  ( 2.500000000000002220, -67.54166666393547303, 4.330127018922192761 ) ) ;
#1009=CARTESIAN_POINT ( 'NONE',  ( 4.458734124999998549, 14.27083333469892601, -2.574251347313721627 ) ) ;
#1010=CARTESIAN_POINT ( 'NONE',  ( -1.339745962155610925, -8.669658196007331341, 5.000000000000000000 ) ) ;
#1011=CARTESIAN_POINT ( 'NONE',  ( -2.500000000000000444, -48.04166666393547303, -4.330127018922193649 ) ) ;
#1013=CARTESIAN_POINT ( 'NONE',  ( -4.458734124999998549, -69.22916666530107932, 2.574251347313722516 ) ) ;
#1014=EDGE_LOOP ( 'NONE', ( #25292, #37955, #18501, #1392 ) ) ;
#1016=CARTESIAN_POINT ( 'NONE',  ( -5.000000000000000000, 2.916666666666668739, -2.886751345948128211 ) ) ;
#1018=CARTESIAN_POINT ( 'NONE',  ( -6.972266317189433020E-16, -17.25000000000000000, -5.000000000000000000 ) ) ;
#1019=CARTESIAN_POINT ( 'NONE',  ( 4.458734125000001214, -59.89583333196774362, 2.574251347313718519 ) ) ;
#1020=CARTESIAN_POINT ( 'NONE',  ( 5.000000000000000888, -90.45833333060214443, 2.886751345948126879 ) ) ;
#1021=CARTESIAN_POINT ( 'NONE',  ( -4.458734124999997661, -33.22916666530106511, 2.574251347313722516 ) ) ;
#1022=CARTESIAN_POINT ( 'NONE',  ( -1.339745962155610925, -41.66965819600731891, 5.000000000000000000 ) ) ;
#1023=CARTESIAN_POINT ( 'NONE',  ( 1.975475456537005874E-15, -43.75000000000000000, 5.000000000000000000 ) ) ;
#1024=CARTESIAN_POINT ( 'NONE',  ( -5.000000000000000000, -107.9583333306021444, -2.886751345948128211 ) ) ;
#1027=CARTESIAN_POINT ( 'NONE',  ( -2.499999999999996447, -43.83333333333333570, 4.330127018922195425 ) ) ;
#1031=CARTESIAN_POINT ( 'NONE',  ( -2.229367062499996610, -106.1458333319677365, 3.861377020970582219 ) ) ;
#1032=CARTESIAN_POINT ( 'NONE',  ( 4.458734125000001214, 3.854166668032260823, 2.574251347313718519 ) ) ;
#1034=( BOUNDED_CURVE ( )  B_SPLINE_CURVE ( 2, ( #14476, #10930, #49533, #49847, #34097, #44379, #43745, #59193, #4835 ),
 .UNSPECIFIED., .F., .F. ) 
 B_SPLINE_CURVE_WITH_KNOTS ( ( 3, 2, 2, 2, 3 ),
 ( 0.6017857142857142572, 0.6023809523809523503, 0.6035714285714285365, 0.6047619047619047228, 0.6053571428571428159 ),
 .UNSPECIFIED. ) 
 CURVE ( )  GEOMETRIC_REPRESENTATION_ITEM ( )  RATIONAL_B_SPLINE_CURVE ( ( 0.9330127018922194093, 0.9330127018922194093, 1.000000000000000000, 0.8660254037844387076, 1.000000000000000000, 0.8660254037844387076, 1.000000000000000000, 0.9330127018922194093, 0.9330127018922194093 ) ) 
 REPRESENTATION_ITEM ( '' )  );
#1042=CARTESIAN_POINT ( 'NONE',  ( -6.972266317189433020E-16, -6.249999999999999112, -5.000000000000000000 ) ) ;
#1044=CARTESIAN_POINT ( 'NONE',  ( -5.000000000000000000, -55.95833333060214443, -2.886751345948128211 ) ) ;
#1047=CARTESIAN_POINT ( 'NONE',  ( -4.458734124999998549, -30.47916666530107221, 2.574251347313722516 ) ) ;
#1048=CARTESIAN_POINT ( 'NONE',  ( 0.000000000000000000, -120.0000000000000000, 0.000000000000000000 ) ) ;
#1055=CARTESIAN_POINT ( 'NONE',  ( 1.975475456537005874E-15, -20.62499999726881228, 5.000000000000000000 ) ) ;
#1057=CARTESIAN_POINT ( 'NONE',  ( -3.152548672688508926E-16, -78.81249999863440792, -5.148502694627439702 ) ) ;
#1060=FACE_OUTER_BOUND ( 'NONE', #7597, .T. ) ;
#1063=CARTESIAN_POINT ( 'NONE',  ( 2.229367062500001939, -3.229166665301069550, 3.861377020970579999 ) ) ;
#1064=ORIENTED_EDGE ( 'NONE', *, *, #24039, .F. ) ;
#1066=CARTESIAN_POINT ( 'NONE',  ( 5.000000000000000000, -91.41666666666665719, -2.886751345948130876 ) ) ;
#1074=CARTESIAN_POINT ( 'NONE',  ( -3.152548672688508926E-16, -80.56249999863440792, -5.148502694627439702 ) ) ;
#1075=CYLINDRICAL_SURFACE ( 'NONE', #55203, 5.000000000000000000 ) ;
#1076=CARTESIAN_POINT ( 'NONE',  ( -4.458734124999999437, -1.312499998634406140, 0.000000000000000000 ) ) ;
#1078=CARTESIAN_POINT ( 'NONE',  ( 0.000000000000000000, -120.0000000000000000, 0.000000000000000000 ) ) ;
#1079=CARTESIAN_POINT ( 'NONE',  ( 4.458734125000001214, -71.14583333196773651, 2.574251347313718519 ) ) ;
#1080=CARTESIAN_POINT ( 'NONE',  ( -5.000000000000000000, -27.95833333060214798, -2.886751345948128211 ) ) ;
#1082=CARTESIAN_POINT ( 'NONE',  ( -3.152548672688508926E-16, 29.43750000136559564, -5.148502694627439702 ) ) ;
#1084=CARTESIAN_POINT ( 'NONE',  ( -2.229367062499996610, -48.14583333196772941, 3.861377020970582219 ) ) ;
#1085=CARTESIAN_POINT ( 'NONE',  ( -2.229367062500000163, -33.72916666530107221, -3.861377020970580443 ) ) ;
#1087=CARTESIAN_POINT ( 'NONE',  ( -1.336351044127974539E-14, 22.37500000273118417, 5.000000000000000000 ) ) ;
#1088=CARTESIAN_POINT ( 'NONE',  ( -3.535250795749689387E-16, 18.75000000000000000, -5.773502691896257311 ) ) ;
#1091=CARTESIAN_POINT ( 'NONE',  ( -2.229367062499996610, -42.14583333196773651, 3.861377020970582219 ) ) ;
#1092=CARTESIAN_POINT ( 'NONE',  ( 2.499999999999998668, -73.20833333060214443, -4.330127018922193649 ) ) ;
#1096=CARTESIAN_POINT ( 'NONE',  ( 4.458734124999999437, -78.06249999863440792, -5.460374474430324690E-16 ) ) ;
#1100=CARTESIAN_POINT ( 'NONE',  ( -2.499999999999996447, -25.83333333333333215, 4.330127018922195425 ) ) ;
#1106=CARTESIAN_POINT ( 'NONE',  ( -4.999999999999999112, 24.20833333606451987, 2.886751345948131764 ) ) ;
#1110=( BOUNDED_CURVE ( )  B_SPLINE_CURVE ( 2, ( #33713, #52706, #63004, #19228, #38844, #58787, #33400, #14404, #9581 ),
 .UNSPECIFIED., .F., .F. ) 
 B_SPLINE_CURVE_WITH_KNOTS ( ( 3, 2, 2, 2, 3 ),
 ( 0.1267857142857142794, 0.1273809523809523725, 0.1285714285714285587, 0.1297619047619047727, 0.1303571428571428659 ),
 .UNSPECIFIED. ) 
 CURVE ( )  GEOMETRIC_REPRESENTATION_ITEM ( )  RATIONAL_B_SPLINE_CURVE ( ( 0.9330127018922194093, 0.9330127018922194093, 1.000000000000000000, 0.8660254037844387076, 1.000000000000000000, 0.8660254037844387076, 1.000000000000000000, 0.9330127018922194093, 0.9330127018922194093 ) ) 
 REPRESENTATION_ITEM ( '' )  );
#1113=CARTESIAN_POINT ( 'NONE',  ( 2.493747252781420335E-13, -91.12499999726880162, -5.000000000000000000 ) ) ;
#1114=CARTESIAN_POINT ( 'NONE',  ( 1.339745962155612702, 15.83034180399266511, -5.000000000000000000 ) ) ;
#1115=CARTESIAN_POINT ( 'NONE',  ( 5.000000000000000000, -33.37499999726880873, -6.123233995736766282E-16 ) ) ;
#1116=CARTESIAN_POINT ( 'NONE',  ( -4.999999999999998224, -61.91666666666666430, 2.886751345948131764 ) ) ;
#1117=CARTESIAN_POINT ( 'NONE',  ( 1.339745962155615144, -56.58034179853028434, 4.999999999999999112 ) ) ;
#1119=CARTESIAN_POINT ( 'NONE',  ( -2.500000000000000444, -79.16666666666665719, -4.330127018922193649 ) ) ;
#1120=CARTESIAN_POINT ( 'NONE',  ( -2.229367062499996610, -15.39583333196773651, 3.861377020970582219 ) ) ;
#1121=CARTESIAN_POINT ( 'NONE',  ( -1.339745962155497683, -78.08034179853028434, -5.000000000000066613 ) ) ;
#1124=AXIS2_PLACEMENT_3D ( 'NONE', #5510, #698, #6795 ) ;
#1134=CARTESIAN_POINT ( 'NONE',  ( -5.000000000000000000, -86.08333333333332860, -2.886751345948128211 ) ) ;
#1137=CARTESIAN_POINT ( 'NONE',  ( 5.000000000000000000, -99.50000000000000000, -6.123233995736766282E-16 ) ) ;
#1141=ORIENTED_EDGE ( 'NONE', *, *, #54678, .F. ) ;
#1143=CARTESIAN_POINT ( 'NONE',  ( -2.229367062500000163, 12.52083333469892601, -3.861377020970580443 ) ) ;
#1146=CARTESIAN_POINT ( 'NONE',  ( 5.000000000000000000, -44.41666666666665719, -2.886751345948130876 ) ) ;
#1148=CARTESIAN_POINT ( 'NONE',  ( 2.229367062499998831, -64.64583333196773651, -3.861377020970580887 ) ) ;
#1150=CARTESIAN_POINT ( 'NONE',  ( -4.458734124999998549, 17.77083333469892779, 2.574251347313722516 ) ) ;
#1151=CARTESIAN_POINT ( 'NONE',  ( -2.499999999999996447, 18.16666666666666430, 4.330127018922195425 ) ) ;
#1153=CARTESIAN_POINT ( 'NONE',  ( 2.229367062500001939, -52.22916666530107221, 3.861377020970579999 ) ) ;
#1154=ADVANCED_FACE ( 'NONE', ( #33345 ), #853, .T. ) ;
#1155=CARTESIAN_POINT ( 'NONE',  ( 5.000000000000000000, -7.374999997268813168, -6.123233995736766282E-16 ) ) ;
#1159=CARTESIAN_POINT ( 'NONE',  ( 0.000000000000000000, -120.0000000000000000, 5.000000000000000000 ) ) ;
#1160=CARTESIAN_POINT ( 'NONE',  ( 9.457646018065525792E-16, -17.31249999863440792, 5.148502694627439702 ) ) ;
#1161=ORIENTED_EDGE ( 'NONE', *, *, #40622, .F. ) ;
#1162=CARTESIAN_POINT ( 'NONE',  ( -6.972266317189433020E-16, -47.12499999726880873, -5.000000000000000000 ) ) ;
#1163=CARTESIAN_POINT ( 'NONE',  ( 2.229367062499998831, -105.6458333319677365, -3.861377020970580887 ) ) ;
#1165=ORIENTED_EDGE ( 'NONE', *, *, #33801, .T. ) ;
#1166=CARTESIAN_POINT ( 'NONE',  ( 9.457646018065525792E-16, -99.31249999863442213, 5.148502694627439702 ) ) ;
#1168=CARTESIAN_POINT ( 'NONE',  ( -3.535250795749689387E-16, -55.12499999726880162, -5.773502691896257311 ) ) ;
#1172=CARTESIAN_POINT ( 'NONE',  ( -2.229367062500000163, -25.47916666530106866, -3.861377020970580443 ) ) ;
#1173=CARTESIAN_POINT ( 'NONE',  ( 9.457646018065525792E-16, 7.687500001365596525, 5.148502694627439702 ) ) ;
#1174=CARTESIAN_POINT ( 'NONE',  ( 4.458734125000000326, -62.14583333196774362, 2.574251347313718519 ) ) ;
#1179=CARTESIAN_POINT ( 'NONE',  ( 5.000000000000000888, -11.58333333333333570, 2.886751345948126879 ) ) ;
#1181=EDGE_LOOP ( 'NONE', ( #9569, #56457, #6169, #33546 ) ) ;
#1183=( BOUNDED_CURVE ( )  B_SPLINE_CURVE ( 2, ( #28033, #13244, #17451, #56695, #22273, #7167, #56377, #26777, #61199 ),
 .UNSPECIFIED., .F., .F. ) 
 B_SPLINE_CURVE_WITH_KNOTS ( ( 3, 2, 2, 2, 3 ),
 ( 0.3553571428571428714, 0.3559523809523809645, 0.3571428571428571508, 0.3583333333333333370, 0.3589285714285714302 ),
 .UNSPECIFIED. ) 
 CURVE ( )  GEOMETRIC_REPRESENTATION_ITEM ( )  RATIONAL_B_SPLINE_CURVE ( ( 0.9330127018922194093, 0.9330127018922194093, 1.000000000000000000, 0.8660254037844387076, 1.000000000000000000, 0.8660254037844387076, 1.000000000000000000, 0.9330127018922194093, 0.9330127018922194093 ) ) 
 REPRESENTATION_ITEM ( '' )  );
#1184=CARTESIAN_POINT ( 'NONE',  ( 6.123233995736766282E-16, -120.0000000000000000, -5.000000000000000000 ) ) ;
#1185=CARTESIAN_POINT ( 'NONE',  ( 1.975475456537005874E-15, -92.74999999999998579, 5.000000000000000000 ) ) ;
#1190=CARTESIAN_POINT ( 'NONE',  ( 1.339745962155612702, -95.16965819600731891, -5.000000000000000000 ) ) ;
#1191=LINE ( 'NONE', #50372, #9804 ) ;
#1193=CARTESIAN_POINT ( 'NONE',  ( -2.499999999999996447, -72.83333333333332860, 4.330127018922195425 ) ) ;
#1195=ORIENTED_EDGE ( 'NONE', *, *, #5962, .T. ) ;
#1196=CARTESIAN_POINT ( 'NONE',  ( -1.230605004983934782E-13, -25.75000000000000355, 5.000000000000000000 ) ) ;
#1197=ORIENTED_EDGE ( 'NONE', *, *, #20141, .F. ) ;
#1202=VERTEX_POINT ( 'NONE', #39414 ) ;
#1204=EDGE_CURVE ( 'NONE', #32122, #25684, #59052, .T. ) ;
#1205=ORIENTED_EDGE ( 'NONE', *, *, #3063, .F. ) ;
#1208=EDGE_CURVE ( 'NONE', #47640, #6601, #61484, .T. ) ;
#1215=CARTESIAN_POINT ( 'NONE',  ( 0.000000000000000000, -120.0000000000000000, 0.000000000000000000 ) ) ;
#1217=PRODUCT_CONTEXT ( 'NONE', #16684, 'mechanical' ) ;
#1219=CARTESIAN_POINT ( 'NONE',  ( 4.458734124999999437, 29.18750000136559208, -5.460374474430324690E-16 ) ) ;
#1226=CARTESIAN_POINT ( 'NONE',  ( -2.229367062500000163, -43.47916666530106511, -3.861377020970580443 ) ) ;
#1229=CARTESIAN_POINT ( 'NONE',  ( -2.229367062500000163, -49.47916666530107221, -3.861377020970580443 ) ) ;
#1230=LINE ( 'NONE', #50088, #56356 ) ;
#1231=ADVANCED_FACE ( 'NONE', ( #34589 ), #45209, .T. ) ;
#1232=CARTESIAN_POINT ( 'NONE',  ( -4.458734124999999437, -17.31249999863440792, 0.000000000000000000 ) ) ;
#1233=CARTESIAN_POINT ( 'NONE',  ( 5.000000000000000000, -100.5000000000000000, -6.123233995736766282E-16 ) ) ;
#1234=CARTESIAN_POINT ( 'NONE',  ( -2.229367062500000163, -35.72916666530107221, -3.861377020970580443 ) ) ;
#1235=CARTESIAN_POINT ( 'NONE',  ( -4.999999999999999112, 4.208333336064518093, 2.886751345948131764 ) ) ;
#1236=CARTESIAN_POINT ( 'NONE',  ( 1.975475456537005874E-15, -50.75000000000000000, 5.000000000000000000 ) ) ;
#1240=CARTESIAN_POINT ( 'NONE',  ( -6.972266317189433020E-16, -30.12499999726880873, -5.000000000000000000 ) ) ;
#1241=CARTESIAN_POINT ( 'NONE',  ( 4.458734124999998549, -0.9791666653010712151, -2.574251347313721627 ) ) ;
#1242=ORIENTED_EDGE ( 'NONE', *, *, #53664, .F. ) ;
#1245=CARTESIAN_POINT ( 'NONE',  ( -2.229367062500000163, -87.47916666530107932, -3.861377020970580443 ) ) ;
#1246=CARTESIAN_POINT ( 'NONE',  ( -2.229367062500000163, -33.47916666530107221, -3.861377020970580443 ) ) ;
#1248=CARTESIAN_POINT ( 'NONE',  ( 2.229367062499998831, -83.89583333196773651, -3.861377020970580887 ) ) ;
#1252=CARTESIAN_POINT ( 'NONE',  ( 4.458734124999998549, -5.729166665301072214, -2.574251347313721627 ) ) ;
#1253=CARTESIAN_POINT ( 'NONE',  ( 4.458734125000001214, 21.85416666803225993, 2.574251347313718519 ) ) ;
#1254=CARTESIAN_POINT ( 'NONE',  ( 4.458734124999999437, -49.06249999863440792, -5.460374474430324690E-16 ) ) ;
#1261=CARTESIAN_POINT ( 'NONE',  ( 4.458734124999999437, -76.81249999863440792, -5.460374474430324690E-16 ) ) ;
#1262=CARTESIAN_POINT ( 'NONE',  ( 9.457646018065525792E-16, 28.68750000136559208, 5.148502694627439702 ) ) ;
#1266=CARTESIAN_POINT ( 'NONE',  ( -2.500000000000000444, 9.833333333333332149, -4.330127018922193649 ) ) ;
#1269=CARTESIAN_POINT ( 'NONE',  ( -2.500000000000000444, -58.16666666666665719, -4.330127018922193649 ) ) ;
#1271=DIRECTION ( 'NONE',  ( -0.000000000000000000, 1.000000000000000000, -0.000000000000000000 ) ) ;
#1274=CARTESIAN_POINT ( 'NONE',  ( -4.999999999999998224, -72.79166666393548724, 2.886751345948131764 ) ) ;
#1275=CARTESIAN_POINT ( 'NONE',  ( 5.000000000000000000, -52.29166666393547303, -2.886751345948130876 ) ) ;
#1286=EDGE_CURVE ( 'NONE', #12722, #37461, #37163, .T. ) ;
#1291=ADVANCED_FACE ( 'NONE', ( #21734 ), #1809, .T. ) ;
#1293=CARTESIAN_POINT ( 'NONE',  ( 4.458734124999999437, -48.06249999863440792, -5.460374474430324690E-16 ) ) ;
#1294=CARTESIAN_POINT ( 'NONE',  ( 5.000000000000000000, -23.41666666666667140, -2.886751345948130876 ) ) ;
#1297=ADVANCED_FACE ( 'NONE', ( #41638 ), #6305, .F. ) ;
#1304=CARTESIAN_POINT ( 'NONE',  ( 4.458734125000001214, -93.14583333196773651, 2.574251347313718519 ) ) ;
#1310=CARTESIAN_POINT ( 'NONE',  ( 1.339745962155615144, -82.58034179853028434, 4.999999999999999112 ) ) ;
#1311=ORIENTED_EDGE ( 'NONE', *, *, #48302, .T. ) ;
#1312=CARTESIAN_POINT ( 'NONE',  ( -4.458734124999999437, -4.395833331967740065, -2.574251347313719407 ) ) ;
#1314=CARTESIAN_POINT ( 'NONE',  ( 5.000000000000000000, -50.37499999726881583, -6.123233995736766282E-16 ) ) ;
#1315=CARTESIAN_POINT ( 'NONE',  ( 4.458734124999998549, -19.97916666530106866, -2.574251347313721627 ) ) ;
#1320=CARTESIAN_POINT ( 'NONE',  ( -2.229367062500000163, 15.27083333469892779, -3.861377020970580443 ) ) ;
#1321=ORIENTED_EDGE ( 'NONE', *, *, #37875, .F. ) ;
#1323=CARTESIAN_POINT ( 'NONE',  ( 4.458734124999998549, -21.72916666530107221, -2.574251347313721627 ) ) ;
#1324=DIRECTION ( 'NONE',  ( -0.000000000000000000, 1.000000000000000000, -0.000000000000000000 ) ) ;
#1326=CARTESIAN_POINT ( 'NONE',  ( 5.000000000000000000, -45.29166666393546592, -2.886751345948129988 ) ) ;
#1327=CARTESIAN_POINT ( 'NONE',  ( -5.000000000000000000, 21.12500000273118417, 0.000000000000000000 ) ) ;
#1328=CARTESIAN_POINT ( 'NONE',  ( -2.229367062500000163, 13.52083333469892779, -3.861377020970580443 ) ) ;
#1334=CARTESIAN_POINT ( 'NONE',  ( -4.458734124999999437, -69.39583333196773651, -2.574251347313719407 ) ) ;
#1336=CARTESIAN_POINT ( 'NONE',  ( -5.000000000000000000, 5.000000000000000888, 0.000000000000000000 ) ) ;
#1338=CARTESIAN_POINT ( 'NONE',  ( -4.458734124999999437, -60.39583333196773651, -2.574251347313719407 ) ) ;
#1339=CARTESIAN_POINT ( 'NONE',  ( -4.999999999999999112, -95.79166666393548724, 2.886751345948131764 ) ) ;
#1340=CARTESIAN_POINT ( 'NONE',  ( -4.458734124999999437, -34.31249999863440792, 0.000000000000000000 ) ) ;
#1341=LINE ( 'NONE', #40544, #38061 ) ;
#1346=CARTESIAN_POINT ( 'NONE',  ( -4.999999999999999112, -40.91666666666667140, 2.886751345948131764 ) ) ;
#1348=CARTESIAN_POINT ( 'NONE',  ( 1.339745962155612702, -17.16965819600733312, -5.000000000000000000 ) ) ;
#1349=ORIENTED_EDGE ( 'NONE', *, *, #54312, .T. ) ;
#1350=CARTESIAN_POINT ( 'NONE',  ( -4.458734124999999437, -108.3958333319677365, -2.574251347313719407 ) ) ;
#1351=CARTESIAN_POINT ( 'NONE',  ( 2.229367062500001939, -3.229166665301069550, 3.861377020970579999 ) ) ;
#1358=ORIENTED_EDGE ( 'NONE', *, *, #9494, .F. ) ;
#1359=CARTESIAN_POINT ( 'NONE',  ( 5.000000000000000000, -33.50000000000000000, -6.123233995736766282E-16 ) ) ;
#1360=CARTESIAN_POINT ( 'NONE',  ( -1.975475456537005874E-15, 28.37500000273118772, 5.000000000000000000 ) ) ;
#1363=( BOUNDED_CURVE ( )  B_SPLINE_CURVE ( 2, ( #26122, #14945, #56035, #36405, #34554, #39383, #16787, #16151, #11951 ),
 .UNSPECIFIED., .F., .F. ) 
 B_SPLINE_CURVE_WITH_KNOTS ( ( 3, 2, 2, 2, 3 ),
 ( 0.8196428571428571175, 0.8202380952380952106, 0.8214285714285713969, 0.8226190476190475831, 0.8232142857142856762 ),
 .UNSPECIFIED. ) 
 CURVE ( )  GEOMETRIC_REPRESENTATION_ITEM ( )  RATIONAL_B_SPLINE_CURVE ( ( 0.9330127018922194093, 0.9330127018922194093, 1.000000000000000000, 0.8660254037844387076, 1.000000000000000000, 0.8660254037844387076, 1.000000000000000000, 0.9330127018922194093, 0.9330127018922194093 ) ) 
 REPRESENTATION_ITEM ( '' )  );
#1367=CARTESIAN_POINT ( 'NONE',  ( 2.229367062499998831, -32.89583333196773651, -3.861377020970580887 ) ) ;
#1370=EDGE_CURVE ( 'NONE', #3563, #63012, #37238, .T. ) ;
#1374=EDGE_CURVE ( 'NONE', #51281, #47780, #57350, .T. ) ;
#1377=ORIENTED_EDGE ( 'NONE', *, *, #11489, .T. ) ;
#1378=CARTESIAN_POINT ( 'NONE',  ( -4.458734124999998549, -76.47916666530105090, 2.574251347313722516 ) ) ;
#1379=CARTESIAN_POINT ( 'NONE',  ( -6.972266317189433020E-16, 12.87500000273118417, -5.000000000000000000 ) ) ;
#1381=CARTESIAN_POINT ( 'NONE',  ( 5.000000000000000000, -16.50000000000000000, -6.123233995736766282E-16 ) ) ;
#1384=CARTESIAN_POINT ( 'NONE',  ( -4.458734124999998549, -4.479166665301070438, 2.574251347313722516 ) ) ;
#1385=EDGE_LOOP ( 'NONE', ( #55922, #57745, #15564, #16254 ) ) ;
#1386=CARTESIAN_POINT ( 'NONE',  ( 6.123233995736766282E-16, -120.0000000000000000, -5.000000000000000000 ) ) ;
#1391=FACE_OUTER_BOUND ( 'NONE', #60635, .T. ) ;
#1392=ORIENTED_EDGE ( 'NONE', *, *, #63423, .T. ) ;
#1393=CARTESIAN_POINT ( 'NONE',  ( 2.229367062499998831, -82.64583333196773651, -3.861377020970580887 ) ) ;
#1394=CARTESIAN_POINT ( 'NONE',  ( -5.000000000000000000, -97.00000000000000000, 0.000000000000000000 ) ) ;
#1395=CARTESIAN_POINT ( 'NONE',  ( 2.229367062500001939, -5.979166665301072214, 3.861377020970579999 ) ) ;
#1397=CARTESIAN_POINT ( 'NONE',  ( -4.458734124999999437, -72.64583333196773651, -2.574251347313719407 ) ) ;
#1398=CARTESIAN_POINT ( 'NONE',  ( -4.999999999999999112, -29.79166666393548368, 2.886751345948131764 ) ) ;
#1400=CARTESIAN_POINT ( 'NONE',  ( -2.500000000000000444, -41.16666666666667140, -4.330127018922193649 ) ) ;
#1403=CARTESIAN_POINT ( 'NONE',  ( -4.458734124999999437, -49.39583333196773651, -2.574251347313719407 ) ) ;
#1404=CARTESIAN_POINT ( 'NONE',  ( 4.458734124999999437, -32.06249999863440792, -5.460374474430324690E-16 ) ) ;
#1408=CARTESIAN_POINT ( 'NONE',  ( -4.999999999999999112, 20.08333333333333215, 2.886751345948131764 ) ) ;
#1410=CARTESIAN_POINT ( 'NONE',  ( 0.000000000000000000, -120.0000000000000000, 0.000000000000000000 ) ) ;
#1411=CARTESIAN_POINT ( 'NONE',  ( 2.229367062500001939, -42.97916666530107932, 3.861377020970579999 ) ) ;
#1412=CARTESIAN_POINT ( 'NONE',  ( 1.060575238724906964E-15, -77.62499999726881583, 5.773502691896257311 ) ) ;
#1416=EDGE_CURVE ( 'NONE', #60061, #26022, #22367, .T. ) ;
#1417=CARTESIAN_POINT ( 'NONE',  ( 1.339745962155615144, -37.70534180126148271, 4.999999999999999112 ) ) ;
#1418=CARTESIAN_POINT ( 'NONE',  ( 4.458734124999998549, -79.97916666530106511, -2.574251347313721627 ) ) ;
#1421=CARTESIAN_POINT ( 'NONE',  ( 2.499999999999998668, -29.33333333333332860, -4.330127018922193649 ) ) ;
#1425=VERTEX_POINT ( 'NONE', #55825 ) ;
#1427=CARTESIAN_POINT ( 'NONE',  ( -5.000000000000000000, 21.04166666939785202, -2.886751345948128211 ) ) ;
#1428=CARTESIAN_POINT ( 'NONE',  ( -2.499999999999996447, -60.70833333060214443, 4.330127018922195425 ) ) ;
#1438=CARTESIAN_POINT ( 'NONE',  ( 4.458734124999998549, -13.97916666530107221, -2.574251347313721627 ) ) ;
#1445=VERTEX_POINT ( 'NONE', #31049 ) ;
#1449=CARTESIAN_POINT ( 'NONE',  ( -6.972266317189433020E-16, -58.24999999999999289, -5.000000000000000000 ) ) ;
#1451=ORIENTED_EDGE ( 'NONE', *, *, #60890, .F. ) ;
#1452=CARTESIAN_POINT ( 'NONE',  ( -5.000000000000000000, -10.00000000000000178, 0.000000000000000000 ) ) ;
#1456=ORIENTED_EDGE ( 'NONE', *, *, #51051, .T. ) ;
#1458=CARTESIAN_POINT ( 'NONE',  ( 5.000000000000000000, 11.58333333333333393, -2.886751345948130876 ) ) ;
#1459=CARTESIAN_POINT ( 'NONE',  ( -4.458734124999998549, 14.77083333469892779, 2.574251347313722516 ) ) ;
#1462=CARTESIAN_POINT ( 'NONE',  ( -6.972266317189433020E-16, -73.12499999726878741, -5.000000000000000000 ) ) ;
#1464=CARTESIAN_POINT ( 'NONE',  ( -4.458734124999997661, -63.22916666530106511, 2.574251347313722516 ) ) ;
#1466=CARTESIAN_POINT ( 'NONE',  ( -2.229367062499996610, 12.85416666803226171, 3.861377020970582219 ) ) ;
#1468=CARTESIAN_POINT ( 'NONE',  ( 1.975475456537005874E-15, -80.62499999726881583, 5.000000000000000000 ) ) ;
#1469=CARTESIAN_POINT ( 'NONE',  ( -4.458734124999998549, -52.47916666530107221, 2.574251347313722516 ) ) ;
#1470=CARTESIAN_POINT ( 'NONE',  ( -2.500000000000000444, -15.04166666393548191, -4.330127018922193649 ) ) ;
#1475=CARTESIAN_POINT ( 'NONE',  ( 9.457646018065525792E-16, -18.31249999863440792, 5.148502694627439702 ) ) ;
#1476=ORIENTED_EDGE ( 'NONE', *, *, #16143, .T. ) ;
#1477=CARTESIAN_POINT ( 'NONE',  ( -3.152548672688508926E-16, -102.5624999986344079, -5.148502694627439702 ) ) ;
#1480=CARTESIAN_POINT ( 'NONE',  ( -4.458734124999999437, -100.6458333319677223, -2.574251347313719407 ) ) ;
#1481=CARTESIAN_POINT ( 'NONE',  ( 2.229367062499998831, -25.64583333196773651, -3.861377020970580887 ) ) ;
#1482=CARTESIAN_POINT ( 'NONE',  ( -5.000000000000000000, -58.95833333060213732, -2.886751345948128211 ) ) ;
#1486=CARTESIAN_POINT ( 'NONE',  ( 2.229367062500001939, -21.97916666530107221, 3.861377020970579999 ) ) ;
#1487=CARTESIAN_POINT ( 'NONE',  ( -4.458734124999997661, -65.47916666530106511, 2.574251347313722516 ) ) ;
#1492=CARTESIAN_POINT ( 'NONE',  ( 5.000000000000000000, -11.49999999999999645, -6.123233995736766282E-16 ) ) ;
#1494=VERTEX_POINT ( 'NONE', #33583 ) ;
#1496=DIRECTION ( 'NONE',  ( 0.000000000000000000, 0.000000000000000000, 1.000000000000000000 ) ) ;
#1497=CARTESIAN_POINT ( 'NONE',  ( -6.972266317189433020E-16, -92.24999999999998579, -5.000000000000000000 ) ) ;
#1499=AXIS2_PLACEMENT_3D ( 'NONE', #26170, #6879, #40327 ) ;
#1501=( BOUNDED_CURVE ( )  B_SPLINE_CURVE ( 2, ( #6880, #21036, #31302, #45470, #15576, #11369, #26811, #59967, #1751 ),
 .UNSPECIFIED., .F., .F. ) 
 B_SPLINE_CURVE_WITH_KNOTS ( ( 3, 2, 2, 2, 3 ),
 ( 0.2874999999999999778, 0.2880952380952380709, 0.2892857142857143127, 0.2904761904761904989, 0.2910714285714285920 ),
 .UNSPECIFIED. ) 
 CURVE ( )  GEOMETRIC_REPRESENTATION_ITEM ( )  RATIONAL_B_SPLINE_CURVE ( ( 0.9330127018922194093, 0.9330127018922194093, 1.000000000000000000, 0.8660254037844387076, 1.000000000000000000, 0.8660254037844387076, 1.000000000000000000, 0.9330127018922194093, 0.9330127018922194093 ) ) 
 REPRESENTATION_ITEM ( '' )  );
#1502=CYLINDRICAL_SURFACE ( 'NONE', #16298, 5.000000000000000000 ) ;
#1503=CARTESIAN_POINT ( 'NONE',  ( -1.339745962155613812, 25.79465819873851729, -5.000000000000000000 ) ) ;
#1505=CARTESIAN_POINT ( 'NONE',  ( 2.500000000000002220, -78.66666666666665719, 4.330127018922192761 ) ) ;
#1508=CARTESIAN_POINT ( 'NONE',  ( 5.000000000000000000, -80.29166666393547303, -2.886751345948130876 ) ) ;
#1523=CARTESIAN_POINT ( 'NONE',  ( -1.339745962155610925, -83.79465819873851729, 5.000000000000000000 ) ) ;
#1524=EDGE_LOOP ( 'NONE', ( #16159, #35442, #61894, #52375 ) ) ;
#1525=SHAPE_DEFINITION_REPRESENTATION ( #33781, #3639 ) ;
#1526=CARTESIAN_POINT ( 'NONE',  ( -2.229367062500000163, -75.47916666530106511, -3.861377020970580443 ) ) ;
#1527=CARTESIAN_POINT ( 'NONE',  ( 2.229367062500001939, -110.2291666653010651, 3.861377020970579999 ) ) ;
#1528=CARTESIAN_POINT ( 'NONE',  ( 1.339745962155615144, 20.29465819873851729, 4.999999999999999112 ) ) ;
#1533=CARTESIAN_POINT ( 'NONE',  ( 2.229367062500001939, -43.97916666530106511, 3.861377020970579999 ) ) ;
#1536=CARTESIAN_POINT ( 'NONE',  ( 2.229367062499998831, -51.64583333196773651, -3.861377020970580887 ) ) ;
#1540=CARTESIAN_POINT ( 'NONE',  ( 2.229367062499998831, -15.64583333196773651, -3.861377020970580887 ) ) ;
#1541=CARTESIAN_POINT ( 'NONE',  ( -5.000000000000000000, -102.0000000000000142, 0.000000000000000000 ) ) ;
#1542=AXIS2_PLACEMENT_3D ( 'NONE', #31166, #26034, #35687 ) ;
#1544=CARTESIAN_POINT ( 'NONE',  ( -4.458734124999999437, -37.64583333196773651, -2.574251347313719407 ) ) ;
#1545=CARTESIAN_POINT ( 'NONE',  ( 5.000000000000000000, 5.708333336064518981, -2.886751345948129988 ) ) ;
#1549=CARTESIAN_POINT ( 'NONE',  ( 5.000000000000000000, 24.58333333333333215, -2.886751345948130876 ) ) ;
#1550=CARTESIAN_POINT ( 'NONE',  ( -6.972266317189433020E-16, -81.12499999726881583, -5.000000000000000000 ) ) ;
#1551=CARTESIAN_POINT ( 'NONE',  ( -3.152548672688508926E-16, 1.187500001365596081, -5.148502694627439702 ) ) ;
#1553=VERTEX_POINT ( 'NONE', #23312 ) ;
#1554=CARTESIAN_POINT ( 'NONE',  ( 5.000000000000000888, 24.54166666939784847, 2.886751345948126879 ) ) ;
#1555=CARTESIAN_POINT ( 'NONE',  ( 2.499999999999998668, -57.33333333333333570, -4.330127018922193649 ) ) ;
#1556=CARTESIAN_POINT ( 'NONE',  ( -2.229367062499996610, -90.14583333196773651, 3.861377020970582219 ) ) ;
#1557=CARTESIAN_POINT ( 'NONE',  ( -3.152548672688508926E-16, -37.56249999863440792, -5.148502694627439702 ) ) ;
#1559=CARTESIAN_POINT ( 'NONE',  ( -2.229367062499996610, -81.39583333196773651, 3.861377020970582219 ) ) ;
#1561=CARTESIAN_POINT ( 'NONE',  ( -4.999999999999998224, -52.91666666666666430, 2.886751345948131764 ) ) ;
#1563=CARTESIAN_POINT ( 'NONE',  ( 9.457646018065525792E-16, -7.062499998634404363, 5.148502694627439702 ) ) ;
#1564=CARTESIAN_POINT ( 'NONE',  ( -4.458734124999998549, 24.52083333469892779, 2.574251347313722516 ) ) ;
#1566=CARTESIAN_POINT ( 'NONE',  ( 2.229367062499998831, -49.89583333196772941, -3.861377020970580887 ) ) ;
#1570=CARTESIAN_POINT ( 'NONE',  ( 1.339745962155612702, -109.1696581960073331, -5.000000000000000000 ) ) ;
#1574=CARTESIAN_POINT ( 'NONE',  ( -2.229367062500000163, -72.47916666530107932, -3.861377020970580443 ) ) ;
#1575=CARTESIAN_POINT ( 'NONE',  ( -4.458734124999999437, 27.43750000136559208, 0.000000000000000000 ) ) ;
#1581=CARTESIAN_POINT ( 'NONE',  ( 5.000000000000000888, -66.58333333333332860, 2.886751345948126879 ) ) ;
#1582=CARTESIAN_POINT ( 'NONE',  ( 1.975475456537005874E-15, -74.75000000000000000, 5.000000000000000000 ) ) ;
#1588=CARTESIAN_POINT ( 'NONE',  ( -6.972266317189433020E-16, -107.1249999972687874, -5.000000000000000000 ) ) ;
#1591=CARTESIAN_POINT ( 'NONE',  ( -6.972266317189433020E-16, -62.24999999999999289, -5.000000000000000000 ) ) ;
#1597=CARTESIAN_POINT ( 'NONE',  ( 0.000000000000000000, -120.0000000000000000, 5.000000000000000000 ) ) ;
#1598=CARTESIAN_POINT ( 'NONE',  ( 5.000000000000000000, 27.62500000273118417, -6.123233995736766282E-16 ) ) ;
#1603=CARTESIAN_POINT ( 'NONE',  ( 4.458734124999998549, -43.97916666530105800, -2.574251347313721627 ) ) ;
#1606=CARTESIAN_POINT ( 'NONE',  ( -6.972266317189433020E-16, -82.12499999726881583, -5.000000000000000000 ) ) ;
#1612=CARTESIAN_POINT ( 'NONE',  ( 2.229367062500001939, -95.22916666530106511, 3.861377020970579999 ) ) ;
#1613=DIRECTION ( 'NONE',  ( -0.000000000000000000, 1.000000000000000000, -0.000000000000000000 ) ) ;
#1619=VERTEX_POINT ( 'NONE', #52623 ) ;
#1620=CARTESIAN_POINT ( 'NONE',  ( -2.229367062500000163, -1.479166665301071770, -3.861377020970580443 ) ) ;
#1622=ADVANCED_FACE ( 'NONE', ( #51995 ), #17590, .T. ) ;
#1624=CARTESIAN_POINT ( 'NONE',  ( -2.229367062499996610, -20.39583333196774007, 3.861377020970582219 ) ) ;
#1629=CARTESIAN_POINT ( 'NONE',  ( 9.457646018065525792E-16, 17.68750000136559208, 5.148502694627439702 ) ) ;
#1632=DIRECTION ( 'NONE',  ( -0.000000000000000000, 1.000000000000000000, -0.000000000000000000 ) ) ;
#1633=CARTESIAN_POINT ( 'NONE',  ( 4.458734125000001214, -21.89583333196773296, 2.574251347313718519 ) ) ;
#1638=CARTESIAN_POINT ( 'NONE',  ( -4.999999999999999112, -48.79166666393547303, 2.886751345948131764 ) ) ;
#1639=CARTESIAN_POINT ( 'NONE',  ( -1.339745962155585168, -2.080341798530294550, -5.000000000000015987 ) ) ;
#1640=CARTESIAN_POINT ( 'NONE',  ( 2.229367062500001939, 9.020833334698927786, 3.861377020970579999 ) ) ;
#1641=CARTESIAN_POINT ( 'NONE',  ( 0.000000000000000000, -120.0000000000000000, 5.000000000000000000 ) ) ;
#1645=CARTESIAN_POINT ( 'NONE',  ( -2.229367062500000163, -69.47916666530107932, -3.861377020970580443 ) ) ;
#1647=CARTESIAN_POINT ( 'NONE',  ( 5.000000000000000000, 0.5000000000000004441, -6.123233995736766282E-16 ) ) ;
#1650=CARTESIAN_POINT ( 'NONE',  ( -4.458734124999999437, -58.39583333196774362, -2.574251347313719407 ) ) ;
#1651=CARTESIAN_POINT ( 'NONE',  ( 2.500000000000002220, -96.54166666393545881, 4.330127018922192761 ) ) ;
#1653=CARTESIAN_POINT ( 'NONE',  ( -4.999999999999998224, -79.91666666666667140, 2.886751345948131764 ) ) ;
#1654=CARTESIAN_POINT ( 'NONE',  ( 2.499999999999998668, -56.33333333333333570, -4.330127018922193649 ) ) ;
#1657=CARTESIAN_POINT ( 'NONE',  ( -5.000000000000000000, -41.08333333333333570, -2.886751345948128211 ) ) ;
#1659=DIRECTION ( 'NONE',  ( 0.000000000000000000, 0.000000000000000000, 1.000000000000000000 ) ) ;
#1660=VERTEX_POINT ( 'NONE', #26923 ) ;
#1661=CARTESIAN_POINT ( 'NONE',  ( 4.458734125000001214, -107.8958333319677365, 2.574251347313718519 ) ) ;
#1662=CARTESIAN_POINT ( 'NONE',  ( -2.229367062499996610, -1.395833331967737179, 3.861377020970582219 ) ) ;
#1663=CARTESIAN_POINT ( 'NONE',  ( 5.000000000000000000, -59.41666666666665719, -2.886751345948130876 ) ) ;
#1670=CARTESIAN_POINT ( 'NONE',  ( 3.253724281355068545E-15, 27.87500000273118772, -5.000000000000000000 ) ) ;
#1673=CARTESIAN_POINT ( 'NONE',  ( -2.500000000000000444, -56.04166666393548013, -4.330127018922193649 ) ) ;
#1675=CARTESIAN_POINT ( 'NONE',  ( -4.458734124999999437, -29.64583333196773651, -2.574251347313719407 ) ) ;
#1681=VECTOR ( 'NONE', #20231, 1000.000000000000000 ) ;
#1685=CARTESIAN_POINT ( 'NONE',  ( -4.999999999999998224, -93.79166666393547303, 2.886751345948131764 ) ) ;
#1686=ORIENTED_EDGE ( 'NONE', *, *, #60219, .F. ) ;
#1687=CARTESIAN_POINT ( 'NONE',  ( 2.229367062500001939, -76.22916666530106511, 3.861377020970579999 ) ) ;
#1690=CARTESIAN_POINT ( 'NONE',  ( 1.339745962155612702, -16.29465819873851729, -5.000000000000000000 ) ) ;
#1691=LINE ( 'NONE', #11628, #28101 ) ;
#1693=CARTESIAN_POINT ( 'NONE',  ( 4.458734124999999437, -3.062499998634407472, -5.460374474430324690E-16 ) ) ;
#1696=EDGE_CURVE ( 'NONE', #13658, #4410, #2677, .T. ) ;
#1698=VERTEX_POINT ( 'NONE', #56516 ) ;
#1705=CARTESIAN_POINT ( 'NONE',  ( -4.458734124999999437, -85.39583333196773651, -2.574251347313719407 ) ) ;
#1706=CYLINDRICAL_SURFACE ( 'NONE', #25393, 5.000000000000000000 ) ;
#1707=CARTESIAN_POINT ( 'NONE',  ( 2.229367062500001939, -2.979166665301069550, 3.861377020970579999 ) ) ;
#1709=CARTESIAN_POINT ( 'NONE',  ( -4.999999999999999112, -31.79166666393548724, 2.886751345948131764 ) ) ;
#1710=CARTESIAN_POINT ( 'NONE',  ( 4.458734124999999437, 22.18750000136559564, -5.460374474430324690E-16 ) ) ;
#1711=CARTESIAN_POINT ( 'NONE',  ( -1.339745962155613812, -38.08034179853029144, -5.000000000000000000 ) ) ;
#1714=CARTESIAN_POINT ( 'NONE',  ( 4.458734124999998549, -51.72916666530107221, -2.574251347313721627 ) ) ;
#1715=CARTESIAN_POINT ( 'NONE',  ( -4.458734124999997661, -37.47916666530107221, 2.574251347313722516 ) ) ;
#1718=CARTESIAN_POINT ( 'NONE',  ( 6.123233995736766282E-16, -120.0000000000000000, -5.000000000000000000 ) ) ;
#1719=CARTESIAN_POINT ( 'NONE',  ( 5.000000000000000000, 20.58333333333333570, -2.886751345948129988 ) ) ;
#1722=CARTESIAN_POINT ( 'NONE',  ( 2.500000000000002220, -26.54166666393547658, 4.330127018922192761 ) ) ;
#1723=CARTESIAN_POINT ( 'NONE',  ( -4.458734124999998549, -44.22916666530106511, 2.574251347313722516 ) ) ;
#1724=CARTESIAN_POINT ( 'NONE',  ( -5.000000000000000000, -76.95833333060214443, -2.886751345948128211 ) ) ;
#1725=VECTOR ( 'NONE', #54297, 1000.000000000000000 ) ;
#1730=CARTESIAN_POINT ( 'NONE',  ( 4.458734125000000326, -82.14583333196772230, 2.574251347313718519 ) ) ;
#1734=CARTESIAN_POINT ( 'NONE',  ( 1.060575238724906964E-15, -28.74999999999999645, 5.773502691896257311 ) ) ;
#1739=CARTESIAN_POINT ( 'NONE',  ( -2.229367062499996610, -90.14583333196773651, 3.861377020970582219 ) ) ;
#1740=CARTESIAN_POINT ( 'NONE',  ( 2.229367062500001939, 14.77083333469892779, 3.861377020970579999 ) ) ;
#1741=( BOUNDED_CURVE ( )  B_SPLINE_CURVE ( 2, ( #41175, #26079, #1654, #26718, #36681, #56315, #60187, #51171, #11275 ),
 .UNSPECIFIED., .F., .F. ) 
 B_SPLINE_CURVE_WITH_KNOTS ( ( 3, 2, 2, 2, 3 ),
 ( 0.6160714285714286031, 0.6166666666666666963, 0.6178571428571428825, 0.6190476190476190688, 0.6196428571428571619 ),
 .UNSPECIFIED. ) 
 CURVE ( )  GEOMETRIC_REPRESENTATION_ITEM ( )  RATIONAL_B_SPLINE_CURVE ( ( 0.9330127018922194093, 0.9330127018922194093, 1.000000000000000000, 0.8660254037844387076, 1.000000000000000000, 0.8660254037844387076, 1.000000000000000000, 0.9330127018922194093, 0.9330127018922194093 ) ) 
 REPRESENTATION_ITEM ( '' )  );
#1742=CARTESIAN_POINT ( 'NONE',  ( -4.999999999999999112, 16.20833333606451987, 2.886751345948131764 ) ) ;
#1749=CARTESIAN_POINT ( 'NONE',  ( -1.339745962155610925, -109.7946581987385315, 5.000000000000000000 ) ) ;
#1751=CARTESIAN_POINT ( 'NONE',  ( 1.975475456537005874E-15, -11.62499999726881406, 5.000000000000000000 ) ) ;
#1753=CARTESIAN_POINT ( 'NONE',  ( 1.975475456537005874E-15, -74.75000000000000000, 5.000000000000000000 ) ) ;
#1755=CARTESIAN_POINT ( 'NONE',  ( -2.229367062499996610, -16.39583333196773651, 3.861377020970582219 ) ) ;
#1763=FACE_OUTER_BOUND ( 'NONE', #1385, .T. ) ;
#1765=( BOUNDED_CURVE ( )  B_SPLINE_CURVE ( 2, ( #28669, #24484, #14503, #43771, #52507, #33197, #48286, #58889, #23856 ),
 .UNSPECIFIED., .F., .F. ) 
 B_SPLINE_CURVE_WITH_KNOTS ( ( 3, 2, 2, 2, 3 ),
 ( 0.3089285714285714413, 0.3095238095238095344, 0.3107142857142857206, 0.3119047619047619069, 0.3125000000000000000 ),
 .UNSPECIFIED. ) 
 CURVE ( )  GEOMETRIC_REPRESENTATION_ITEM ( )  RATIONAL_B_SPLINE_CURVE ( ( 0.9330127018922194093, 0.9330127018922194093, 1.000000000000000000, 0.8660254037844387076, 1.000000000000000000, 0.8660254037844387076, 1.000000000000000000, 0.9330127018922194093, 0.9330127018922194093 ) ) 
 REPRESENTATION_ITEM ( '' )  );
#1766=CARTESIAN_POINT ( 'NONE',  ( -1.339745962155610925, -27.79465819873851729, 5.000000000000000000 ) ) ;
#1767=CARTESIAN_POINT ( 'NONE',  ( 6.123233995736766282E-16, -120.0000000000000000, -5.000000000000000000 ) ) ;
#1771=CARTESIAN_POINT ( 'NONE',  ( -4.999999999999998224, -9.916666666666662522, 2.886751345948131764 ) ) ;
#1779=CARTESIAN_POINT ( 'NONE',  ( -4.458734124999998549, 13.77083333469892779, 2.574251347313722516 ) ) ;
#1783=CARTESIAN_POINT ( 'NONE',  ( -1.230605004983934782E-13, -25.75000000000000355, 5.000000000000000000 ) ) ;
#1786=CARTESIAN_POINT ( 'NONE',  ( -4.458734124999999437, -67.31249999863440792, 0.000000000000000000 ) ) ;
#1788=CARTESIAN_POINT ( 'NONE',  ( 4.458734125000001214, 15.10416666803225993, 2.574251347313718519 ) ) ;
#1791=CARTESIAN_POINT ( 'NONE',  ( 2.229367062499998831, -54.89583333196773651, -3.861377020970580887 ) ) ;
#1792=CARTESIAN_POINT ( 'NONE',  ( -4.999999999999999112, -13.79166666393548191, 2.886751345948131764 ) ) ;
#1796=CARTESIAN_POINT ( 'NONE',  ( -4.458734124999999437, -17.64583333196773651, -2.574251347313719407 ) ) ;
#1799=CARTESIAN_POINT ( 'NONE',  ( -4.458734124999999437, -101.3958333319677365, -2.574251347313719407 ) ) ;
#1801=ORIENTED_EDGE ( 'NONE', *, *, #51159, .T. ) ;
#1802=CARTESIAN_POINT ( 'NONE',  ( -4.458734124999999437, -104.6458333319677365, -2.574251347313719407 ) ) ;
#1803=CARTESIAN_POINT ( 'NONE',  ( -2.229367062499996610, -29.14583333196774007, 3.861377020970582219 ) ) ;
#1804=CARTESIAN_POINT ( 'NONE',  ( 5.000000000000000888, -61.45833333060214443, 2.886751345948126879 ) ) ;
#1807=CARTESIAN_POINT ( 'NONE',  ( 4.458734125000000326, -21.89583333196773296, 2.574251347313718519 ) ) ;
#1808=CARTESIAN_POINT ( 'NONE',  ( -4.458734124999999437, -65.64583333196773651, -2.574251347313719407 ) ) ;
#1809=CYLINDRICAL_SURFACE ( 'NONE', #53128, 5.000000000000000000 ) ;
#1813=CARTESIAN_POINT ( 'NONE',  ( -2.500000000000000444, -10.16666666666666430, -4.330127018922193649 ) ) ;
#1817=CARTESIAN_POINT ( 'NONE',  ( 1.975475456537005874E-15, -84.62499999726880162, 5.000000000000000000 ) ) ;
#1825=CARTESIAN_POINT ( 'NONE',  ( 5.000000000000000888, -95.45833333060213022, 2.886751345948126879 ) ) ;
#1826=FACE_OUTER_BOUND ( 'NONE', #36269, .T. ) ;
#1829=ORIENTED_EDGE ( 'NONE', *, *, #16228, .T. ) ;
#1830=DIRECTION ( 'NONE',  ( -0.000000000000000000, 1.000000000000000000, -0.000000000000000000 ) ) ;
#1832=CARTESIAN_POINT ( 'NONE',  ( 1.339745962155616255, 26.70534180126147561, -4.999999999999997335 ) ) ;
#1836=EDGE_LOOP ( 'NONE', ( #48086, #31159, #39054, #10785 ) ) ;
#1839=CARTESIAN_POINT ( 'NONE',  ( -6.972266317189433020E-16, -109.1249999972688016, -5.000000000000000000 ) ) ;
#1842=CARTESIAN_POINT ( 'NONE',  ( -6.972266317189433020E-16, -62.12499999726880162, -5.000000000000000000 ) ) ;
#1847=ORIENTED_EDGE ( 'NONE', *, *, #37550, .T. ) ;
#1848=CARTESIAN_POINT ( 'NONE',  ( -4.458734124999999437, -77.31249999863440792, 0.000000000000000000 ) ) ;
#1849=CARTESIAN_POINT ( 'NONE',  ( 2.229367062499998831, 29.35416666803225993, -3.861377020970580887 ) ) ;
#1850=CARTESIAN_POINT ( 'NONE',  ( -2.499999999999996447, -53.83333333333332860, 4.330127018922195425 ) ) ;
#1856=CARTESIAN_POINT ( 'NONE',  ( 2.229367062500001939, -44.97916666530106511, 3.861377020970579999 ) ) ;
#1858=DIRECTION ( 'NONE',  ( -0.000000000000000000, 1.000000000000000000, -0.000000000000000000 ) ) ;
#1859=CARTESIAN_POINT ( 'NONE',  ( 4.458734125000000326, -48.89583333196772941, 2.574251347313718519 ) ) ;
#1861=CARTESIAN_POINT ( 'NONE',  ( -4.458734124999999437, 26.60416666803225993, -2.574251347313719407 ) ) ;
#1862=AXIS2_PLACEMENT_3D ( 'NONE', #35867, #40358, #56122 ) ;
#1864=CARTESIAN_POINT ( 'NONE',  ( -5.000000000000000000, -107.9999999999999858, 0.000000000000000000 ) ) ;
#1866=CARTESIAN_POINT ( 'NONE',  ( -4.458734124999999437, -39.64583333196774362, -2.574251347313719407 ) ) ;
#1867=CARTESIAN_POINT ( 'NONE',  ( 2.500000000000002220, 2.458333336064519870, 4.330127018922192761 ) ) ;
#1872=CARTESIAN_POINT ( 'NONE',  ( -3.152548672688508926E-16, -96.56249999863440792, -5.148502694627439702 ) ) ;
#1873=CARTESIAN_POINT ( 'NONE',  ( 1.464175926609780648E-14, 24.74999999999999645, -5.000000000000000000 ) ) ;
#1874=CARTESIAN_POINT ( 'NONE',  ( -4.458734124999997661, -0.4791666653010707710, 2.574251347313722516 ) ) ;
#1875=ORIENTED_EDGE ( 'NONE', *, *, #27621, .F. ) ;
#1877=CARTESIAN_POINT ( 'NONE',  ( -5.000000000000000000, -76.00000000000000000, 0.000000000000000000 ) ) ;
#1878=CARTESIAN_POINT ( 'NONE',  ( -2.229367062500000163, -85.47916666530107932, -3.861377020970580443 ) ) ;
#1880=CARTESIAN_POINT ( 'NONE',  ( 9.457646018065525792E-16, -88.31249999863439371, 5.148502694627439702 ) ) ;
#1883=AXIS2_PLACEMENT_3D ( 'NONE', #26755, #6824, #31573 ) ;
#1886=CARTESIAN_POINT ( 'NONE',  ( 4.458734125000000326, -7.895833331967735624, 2.574251347313718519 ) ) ;
#1887=CARTESIAN_POINT ( 'NONE',  ( 4.458734124999998549, 19.02083333469892779, -2.574251347313721627 ) ) ;
#1888=CARTESIAN_POINT ( 'NONE',  ( -2.229367062499996610, -50.39583333196772941, 3.861377020970582219 ) ) ;
#1895=CARTESIAN_POINT ( 'NONE',  ( -4.458734124999998549, -74.22916666530106511, 2.574251347313722516 ) ) ;
#1896=CARTESIAN_POINT ( 'NONE',  ( 1.060575238724906964E-15, -109.6249999972688016, 5.773502691896257311 ) ) ;
#1901=CARTESIAN_POINT ( 'NONE',  ( 1.060575238724906964E-15, -62.75000000000000000, 5.773502691896257311 ) ) ;
#1902=CARTESIAN_POINT ( 'NONE',  ( 5.000000000000000888, -90.45833333060214443, 2.886751345948126879 ) ) ;
#1905=DIRECTION ( 'NONE',  ( -0.000000000000000000, 1.000000000000000000, -0.000000000000000000 ) ) ;
#1915=ORIENTED_EDGE ( 'NONE', *, *, #21762, .T. ) ;
#1917=CARTESIAN_POINT ( 'NONE',  ( 5.000000000000000888, -59.45833333060214443, 2.886751345948126879 ) ) ;
#1919=VERTEX_POINT ( 'NONE', #29736 ) ;
#1922=CARTESIAN_POINT ( 'NONE',  ( -3.152548672688508926E-16, -45.81249999863440081, -5.148502694627439702 ) ) ;
#1923=CARTESIAN_POINT ( 'NONE',  ( -5.000000000000000000, -96.00000000000000000, 0.000000000000000000 ) ) ;
#1926=CARTESIAN_POINT ( 'NONE',  ( -4.999999999999998224, -81.79166666393547303, 2.886751345948131764 ) ) ;
#1931=EDGE_CURVE ( 'NONE', #35992, #58774, #49368, .T. ) ;
#1932=CARTESIAN_POINT ( 'NONE',  ( -6.972266317189433020E-16, -59.12499999726880873, -5.000000000000000000 ) ) ;
#1936=CARTESIAN_POINT ( 'NONE',  ( -2.229367062500000163, -94.72916666530106511, -3.861377020970580443 ) ) ;
#1943=CARTESIAN_POINT ( 'NONE',  ( 5.000000000000000888, -60.58333333333332860, 2.886751345948126879 ) ) ;
#1944=EDGE_CURVE ( 'NONE', #5440, #14049, #63525, .T. ) ;
#1945=CARTESIAN_POINT ( 'NONE',  ( -4.458734124999999437, -2.395833331967737845, -2.574251347313719407 ) ) ;
#1947=CARTESIAN_POINT ( 'NONE',  ( -4.458734124999999437, -22.64583333196773296, -2.574251347313719407 ) ) ;
#1951=CARTESIAN_POINT ( 'NONE',  ( 1.975475456537005874E-15, 17.25000000000000000, 5.000000000000000000 ) ) ;
#1953=CARTESIAN_POINT ( 'NONE',  ( 2.229367062500001939, 14.77083333469892779, 3.861377020970579999 ) ) ;
#1955=DIRECTION ( 'NONE',  ( 0.000000000000000000, 0.000000000000000000, 1.000000000000000000 ) ) ;
#1956=CARTESIAN_POINT ( 'NONE',  ( 1.975475456537005874E-15, -57.62499999726880873, 5.000000000000000000 ) ) ;
#1957=CARTESIAN_POINT ( 'NONE',  ( 1.060575238724906964E-15, -83.75000000000000000, 5.773502691896257311 ) ) ;
#1958=CARTESIAN_POINT ( 'NONE',  ( 4.458734125000001214, -17.89583333196774007, 2.574251347313718519 ) ) ;
#1962=EDGE_CURVE ( 'NONE', #14760, #21496, #4343, .T. ) ;
#1963=CARTESIAN_POINT ( 'NONE',  ( 2.500000000000002220, -47.54166666393547303, 4.330127018922192761 ) ) ;
#1964=CARTESIAN_POINT ( 'NONE',  ( -4.458734124999999437, 9.604166668032259935, -2.574251347313719407 ) ) ;
#1965=DIRECTION ( 'NONE',  ( 0.000000000000000000, 0.000000000000000000, 1.000000000000000000 ) ) ;
#1968=CARTESIAN_POINT ( 'NONE',  ( 4.458734124999998549, -65.72916666530106511, -2.574251347313721627 ) ) ;
#1971=CARTESIAN_POINT ( 'NONE',  ( -2.500000000000000444, -2.166666666666663854, -4.330127018922193649 ) ) ;
#1974=CARTESIAN_POINT ( 'NONE',  ( -4.458734124999999437, -59.39583333196773651, -2.574251347313719407 ) ) ;
#1975=CARTESIAN_POINT ( 'NONE',  ( -3.535250795749689387E-16, -97.12499999726881583, -5.773502691896257311 ) ) ;
#1979=CARTESIAN_POINT ( 'NONE',  ( -2.500000000000000444, -49.16666666666666430, -4.330127018922193649 ) ) ;
#1981=CARTESIAN_POINT ( 'NONE',  ( -5.000000000000000000, -108.0833333333333712, -2.886751345948128211 ) ) ;
#1983=CARTESIAN_POINT ( 'NONE',  ( 4.458734124999999437, -106.8124999986343937, -5.460374474430324690E-16 ) ) ;
#1984=CARTESIAN_POINT ( 'NONE',  ( -2.229367062500000163, -0.7291666653010709931, -3.861377020970580443 ) ) ;
#1993=CARTESIAN_POINT ( 'NONE',  ( 0.000000000000000000, -120.0000000000000000, 0.000000000000000000 ) ) ;
#1996=CARTESIAN_POINT ( 'NONE',  ( -1.339745962155610925, -48.66965819600732601, 5.000000000000000000 ) ) ;
#1998=CARTESIAN_POINT ( 'NONE',  ( -2.229367062500000163, -30.72916666530107221, -3.861377020970580443 ) ) ;
#2007=DIRECTION ( 'NONE',  ( 0.000000000000000000, 0.000000000000000000, 1.000000000000000000 ) ) ;
#2010=CARTESIAN_POINT ( 'NONE',  ( 4.458734124999999437, -78.06249999863440792, -5.460374474430324690E-16 ) ) ;
#2011=CARTESIAN_POINT ( 'NONE',  ( -1.339745962155613812, 12.91965820146970678, -5.000000000000000000 ) ) ;
#2013=CARTESIAN_POINT ( 'NONE',  ( 1.339745962155615144, -16.70534180126147561, 4.999999999999999112 ) ) ;
#2016=CARTESIAN_POINT ( 'NONE',  ( 4.458734124999999437, -8.062499998634404363, -5.460374474430324690E-16 ) ) ;
#2021=CARTESIAN_POINT ( 'NONE',  ( -2.229367062499996610, -4.395833331967740065, 3.861377020970582219 ) ) ;
#2026=ORIENTED_EDGE ( 'NONE', *, *, #62327, .F. ) ;
#2027=CARTESIAN_POINT ( 'NONE',  ( -4.458734124999999437, -89.31249999863440792, 0.000000000000000000 ) ) ;
#2029=CARTESIAN_POINT ( 'NONE',  ( 4.458734124999998549, -0.7291666653010709931, -2.574251347313721627 ) ) ;
#2031=CARTESIAN_POINT ( 'NONE',  ( -2.499999999999996447, -31.70833333060214798, 4.330127018922195425 ) ) ;
#2033=CARTESIAN_POINT ( 'NONE',  ( 2.229367062500001939, 26.02083333469892779, 3.861377020970579999 ) ) ;
#2034=CARTESIAN_POINT ( 'NONE',  ( -1.339745962155613812, -56.20534180126148271, -5.000000000000000000 ) ) ;
#2036=CARTESIAN_POINT ( 'NONE',  ( 2.229367062500001939, -51.97916666530107221, 3.861377020970579999 ) ) ;
#2037=CARTESIAN_POINT ( 'NONE',  ( 4.458734124999998549, -37.97916666530107221, -2.574251347313721627 ) ) ;
#2039=CARTESIAN_POINT ( 'NONE',  ( -2.229367062499996610, -39.39583333196773651, 3.861377020970582219 ) ) ;
#2041=CARTESIAN_POINT ( 'NONE',  ( 5.000000000000000000, 13.58333333333333215, -2.886751345948129988 ) ) ;
#2043=CARTESIAN_POINT ( 'NONE',  ( -8.660254037844341113, 45.00000000000000000, 6.047423072554883697E-14 ) ) ;
#2044=CARTESIAN_POINT ( 'NONE',  ( -2.229367062499996610, -40.14583333196773651, 3.861377020970582219 ) ) ;
#2045=CARTESIAN_POINT ( 'NONE',  ( -4.999999999999999112, -76.79166666393547303, 2.886751345948131764 ) ) ;
#2048=CARTESIAN_POINT ( 'NONE',  ( -6.972266317189433020E-16, -59.25000000000000000, -5.000000000000000000 ) ) ;
#2049=CARTESIAN_POINT ( 'NONE',  ( 2.229367062499998831, -83.89583333196773651, -3.861377020970580887 ) ) ;
#2052=CARTESIAN_POINT ( 'NONE',  ( 2.499999999999998668, -30.33333333333332860, -4.330127018922193649 ) ) ;
#2054=ORIENTED_EDGE ( 'NONE', *, *, #50275, .T. ) ;
#2056=VERTEX_POINT ( 'NONE', #16554 ) ;
#2057=CARTESIAN_POINT ( 'NONE',  ( -4.458734124999999437, -90.39583333196773651, -2.574251347313719407 ) ) ;
#2058=CARTESIAN_POINT ( 'NONE',  ( 4.458734125000001214, 11.85416666803225993, 2.574251347313718519 ) ) ;
#2059=VECTOR ( 'NONE', #54352, 1000.000000000000000 ) ;
#2060=CARTESIAN_POINT ( 'NONE',  ( -5.000000000000000000, 18.04166666939785557, -2.886751345948128211 ) ) ;
#2064=( BOUNDED_CURVE ( )  B_SPLINE_CURVE ( 2, ( #15831, #36724, #60226, #50561, #56355, #55394, #50238, #25801, #36084 ),
 .UNSPECIFIED., .F., .F. ) 
 B_SPLINE_CURVE_WITH_KNOTS ( ( 3, 2, 2, 2, 3 ),
 ( 0.3125000000000000000, 0.3130952380952380931, 0.3142857142857142794, 0.3154761904761904656, 0.3160714285714285587 ),
 .UNSPECIFIED. ) 
 CURVE ( )  GEOMETRIC_REPRESENTATION_ITEM ( )  RATIONAL_B_SPLINE_CURVE ( ( 0.9330127018922194093, 0.9330127018922194093, 1.000000000000000000, 0.8660254037844387076, 1.000000000000000000, 0.8660254037844387076, 1.000000000000000000, 0.9330127018922194093, 0.9330127018922194093 ) ) 
 REPRESENTATION_ITEM ( '' )  );
#2068=CARTESIAN_POINT ( 'NONE',  ( -6.972266317189433020E-16, -52.12499999726880873, -5.000000000000000000 ) ) ;
#2070=EDGE_CURVE ( 'NONE', #4248, #1202, #45820, .T. ) ;
#2071=CARTESIAN_POINT ( 'NONE',  ( 5.000000000000000000, 28.70833333606451987, -2.886751345948130876 ) ) ;
#2073=CARTESIAN_POINT ( 'NONE',  ( -6.972266317189433020E-16, -96.25000000000000000, -5.000000000000000000 ) ) ;
#2074=CYLINDRICAL_SURFACE ( 'NONE', #5782, 5.000000000000000000 ) ;
#2075=CARTESIAN_POINT ( 'NONE',  ( 4.458734125000001214, -17.14583333196773651, 2.574251347313718519 ) ) ;
#2076=EDGE_CURVE ( 'NONE', #14691, #5147, #48299, .T. ) ;
#2082=EDGE_CURVE ( 'NONE', #53065, #23818, #20747, .T. ) ;
#2086=ORIENTED_EDGE ( 'NONE', *, *, #4425, .T. ) ;
#2089=CARTESIAN_POINT ( 'NONE',  ( -4.458734124999999437, -60.56249999863440081, 0.000000000000000000 ) ) ;
#2091=CARTESIAN_POINT ( 'NONE',  ( 1.975475456537005874E-15, -85.75000000000000000, 5.000000000000000000 ) ) ;
#2093=EDGE_CURVE ( 'NONE', #6014, #15910, #20426, .T. ) ;
#2096=ADVANCED_FACE ( 'NONE', ( #27466 ), #7234, .T. ) ;
#2103=CARTESIAN_POINT ( 'NONE',  ( -2.229367062500000163, 6.520833334698928674, -3.861377020970580443 ) ) ;
#2109=CARTESIAN_POINT ( 'NONE',  ( 2.229367062500001939, -72.97916666530107932, 3.861377020970579999 ) ) ;
#2110=CARTESIAN_POINT ( 'NONE',  ( 6.123233995736766282E-16, -120.0000000000000000, -5.000000000000000000 ) ) ;
#2111=CARTESIAN_POINT ( 'NONE',  ( 2.229367062500001939, 11.02083333469892956, 3.861377020970579999 ) ) ;
#2113=CARTESIAN_POINT ( 'NONE',  ( 4.458734125000001214, -57.14583333196773651, 2.574251347313718519 ) ) ;
#2114=CARTESIAN_POINT ( 'NONE',  ( -5.000000000000000000, -15.87499999726881406, 0.000000000000000000 ) ) ;
#2115=CARTESIAN_POINT ( 'NONE',  ( -2.499999999999996447, -32.70833333060215153, 4.330127018922195425 ) ) ;
#2119=CARTESIAN_POINT ( 'NONE',  ( -3.152548672688508926E-16, -20.81249999863440081, -5.148502694627439702 ) ) ;
#2120=( BOUNDED_CURVE ( )  B_SPLINE_CURVE ( 2, ( #43014, #52673, #32419, #36938, #12485, #62018, #61390, #32098, #52980 ),
 .UNSPECIFIED., .F., .F. ) 
 B_SPLINE_CURVE_WITH_KNOTS ( ( 3, 2, 2, 2, 3 ),
 ( 0.7267857142857142572, 0.7273809523809523503, 0.7285714285714285365, 0.7297619047619047228, 0.7303571428571428159 ),
 .UNSPECIFIED. ) 
 CURVE ( )  GEOMETRIC_REPRESENTATION_ITEM ( )  RATIONAL_B_SPLINE_CURVE ( ( 0.9330127018922194093, 0.9330127018922194093, 1.000000000000000000, 0.8660254037844387076, 1.000000000000000000, 0.8660254037844387076, 1.000000000000000000, 0.9330127018922194093, 0.9330127018922194093 ) ) 
 REPRESENTATION_ITEM ( '' )  );
#2122=CARTESIAN_POINT ( 'NONE',  ( 2.229367062499998831, -108.6458333319677365, -3.861377020970580887 ) ) ;
#2124=EDGE_LOOP ( 'NONE', ( #16966, #31387, #25754, #11709 ) ) ;
#2125=CARTESIAN_POINT ( 'NONE',  ( -4.458734124999999437, -102.5624999986344079, 0.000000000000000000 ) ) ;
#2126=CARTESIAN_POINT ( 'NONE',  ( -4.458734124999998549, -24.22916666530107577, 2.574251347313722516 ) ) ;
#2127=CARTESIAN_POINT ( 'NONE',  ( 2.500000000000002220, -60.54166666393547303, 4.330127018922192761 ) ) ;
#2130=CARTESIAN_POINT ( 'NONE',  ( 4.458734124999999437, -24.81249999863440436, -5.460374474430324690E-16 ) ) ;
#2131=CARTESIAN_POINT ( 'NONE',  ( -3.152548672688508926E-16, -67.81249999863440792, -5.148502694627439702 ) ) ;
#2135=CARTESIAN_POINT ( 'NONE',  ( 1.060575238724906964E-15, -12.74999999999999822, 5.773502691896257311 ) ) ;
#2139=CARTESIAN_POINT ( 'NONE',  ( 5.000000000000000888, -84.45833333060214443, 2.886751345948126879 ) ) ;
#2146=CARTESIAN_POINT ( 'NONE',  ( 0.000000000000000000, -120.0000000000000000, 0.000000000000000000 ) ) ;
#2149=ORIENTED_EDGE ( 'NONE', *, *, #40155, .F. ) ;
#2152=CARTESIAN_POINT ( 'NONE',  ( 1.975475456537005874E-15, -85.75000000000000000, 5.000000000000000000 ) ) ;
#2159=ORIENTED_EDGE ( 'NONE', *, *, #22101, .F. ) ;
#2162=( BOUNDED_CURVE ( )  B_SPLINE_CURVE ( 2, ( #4261, #52529, #43482, #28999, #4563, #18103, #63127, #34147, #32905 ),
 .UNSPECIFIED., .F., .F. ) 
 B_SPLINE_CURVE_WITH_KNOTS ( ( 3, 2, 2, 2, 3 ),
 ( 0.1589285714285714191, 0.1595238095238095122, 0.1607142857142857262, 0.1619047619047619124, 0.1625000000000000056 ),
 .UNSPECIFIED. ) 
 CURVE ( )  GEOMETRIC_REPRESENTATION_ITEM ( )  RATIONAL_B_SPLINE_CURVE ( ( 0.9330127018922194093, 0.9330127018922194093, 1.000000000000000000, 0.8660254037844387076, 1.000000000000000000, 0.8660254037844387076, 1.000000000000000000, 0.9330127018922194093, 0.9330127018922194093 ) ) 
 REPRESENTATION_ITEM ( '' )  );
#2164=ORIENTED_EDGE ( 'NONE', *, *, #52265, .F. ) ;
#2170=CARTESIAN_POINT ( 'NONE',  ( 4.458734124999999437, -77.81249999863440792, -5.460374474430324690E-16 ) ) ;
#2171=CARTESIAN_POINT ( 'NONE',  ( -4.458734124999998549, 23.77083333469892423, 2.574251347313722516 ) ) ;
#2172=CARTESIAN_POINT ( 'NONE',  ( 5.000000000000000888, -18.58333333333333215, 2.886751345948126879 ) ) ;
#2173=ORIENTED_EDGE ( 'NONE', *, *, #3151, .F. ) ;
#2174=CARTESIAN_POINT ( 'NONE',  ( -5.000000000000000000, 5.125000002731184168, 0.000000000000000000 ) ) ;
#2179=CARTESIAN_POINT ( 'NONE',  ( 0.000000000000000000, 45.00000000000000000, 0.000000000000000000 ) ) ;
#2182=CARTESIAN_POINT ( 'NONE',  ( 4.458734124999999437, -56.81249999863440081, -5.460374474430324690E-16 ) ) ;
#2184=CARTESIAN_POINT ( 'NONE',  ( -3.152548672688508926E-16, 27.43750000136559564, -5.148502694627439702 ) ) ;
#2185=CARTESIAN_POINT ( 'NONE',  ( 1.060575238724906964E-15, -105.7500000000000000, 5.773502691896257311 ) ) ;
#2187=CARTESIAN_POINT ( 'NONE',  ( 4.458734124999999437, -37.06249999863440792, -5.460374474430324690E-16 ) ) ;
#2188=CARTESIAN_POINT ( 'NONE',  ( -4.999999999999999112, 1.208333336064518759, 2.886751345948131764 ) ) ;
#2192=CARTESIAN_POINT ( 'NONE',  ( 5.000000000000000000, -71.50000000000000000, -6.123233995736766282E-16 ) ) ;
#2193=CARTESIAN_POINT ( 'NONE',  ( -2.229367062500000163, -98.47916666530105090, -3.861377020970580443 ) ) ;
#2194=CARTESIAN_POINT ( 'NONE',  ( -2.229367062500000163, -7.729166665301073991, -3.861377020970580443 ) ) ;
#2195=VERTEX_POINT ( 'NONE', #36812 ) ;
#2196=CYLINDRICAL_SURFACE ( 'NONE', #3727, 5.000000000000000000 ) ;
#2197=CARTESIAN_POINT ( 'NONE',  ( -4.999999999999998224, -85.79166666393547303, 2.886751345948131764 ) ) ;
#2198=CARTESIAN_POINT ( 'NONE',  ( 2.229367062499998831, -89.64583333196773651, -3.861377020970580887 ) ) ;
#2199=CARTESIAN_POINT ( 'NONE',  ( 5.000000000000000888, 27.41666666666666430, 2.886751345948126879 ) ) ;
#2200=CARTESIAN_POINT ( 'NONE',  ( -4.458734124999999437, -88.64583333196773651, -2.574251347313719407 ) ) ;
#2204=CARTESIAN_POINT ( 'NONE',  ( -4.458734124999997661, -7.229166665301073103, 2.574251347313722516 ) ) ;
#2205=CARTESIAN_POINT ( 'NONE',  ( 2.229367062499998831, 16.10416666803225993, -3.861377020970580887 ) ) ;
#2206=CARTESIAN_POINT ( 'NONE',  ( -3.152548672688508926E-16, -50.81249999863440792, -5.148502694627439702 ) ) ;
#2211=EDGE_LOOP ( 'NONE', ( #28542, #61628, #21308, #51062 ) ) ;
#2214=CARTESIAN_POINT ( 'NONE',  ( 4.458734124999999437, -78.81249999863440792, -5.460374474430324690E-16 ) ) ;
#2215=CARTESIAN_POINT ( 'NONE',  ( 5.000000000000000888, -108.4583333306021444, 2.886751345948126879 ) ) ;
#2220=CARTESIAN_POINT ( 'NONE',  ( -5.000000000000000000, -65.00000000000000000, 0.000000000000000000 ) ) ;
#2221=CARTESIAN_POINT ( 'NONE',  ( 1.339745962155615144, -63.58034179853028434, 4.999999999999999112 ) ) ;
#2223=ORIENTED_EDGE ( 'NONE', *, *, #18261, .T. ) ;
#2225=CARTESIAN_POINT ( 'NONE',  ( -6.972266317189433020E-16, 7.750000000000000000, -5.000000000000000000 ) ) ;
#2233=ORIENTED_EDGE ( 'NONE', *, *, #6777, .F. ) ;
#2235=CARTESIAN_POINT ( 'NONE',  ( 1.339745962155612702, -28.29465819873851729, -5.000000000000000000 ) ) ;
#2240=CARTESIAN_POINT ( 'NONE',  ( -4.458734124999998549, -50.47916666530107221, 2.574251347313722516 ) ) ;
#2247=( BOUNDED_CURVE ( )  B_SPLINE_CURVE ( 2, ( #54981, #10910, #2547, #1926, #41127, #11859, #41443, #31475, #1606 ),
 .UNSPECIFIED., .F., .F. ) 
 B_SPLINE_CURVE_WITH_KNOTS ( ( 3, 2, 2, 2, 3 ),
 ( 0.7910714285714285365, 0.7916666666666666297, 0.7928571428571428159, 0.7940476190476190022, 0.7946428571428570953 ),
 .UNSPECIFIED. ) 
 CURVE ( )  GEOMETRIC_REPRESENTATION_ITEM ( )  RATIONAL_B_SPLINE_CURVE ( ( 0.9330127018922194093, 0.9330127018922194093, 1.000000000000000000, 0.8660254037844387076, 1.000000000000000000, 0.8660254037844387076, 1.000000000000000000, 0.9330127018922194093, 0.9330127018922194093 ) ) 
 REPRESENTATION_ITEM ( '' )  );
#2250=CARTESIAN_POINT ( 'NONE',  ( 9.457646018065525792E-16, -92.31249999863439371, 5.148502694627439702 ) ) ;
#2252=VERTEX_POINT ( 'NONE', #27158 ) ;
#2253=LINE ( 'NONE', #6744, #62191 ) ;
#2256=DIRECTION ( 'NONE',  ( -0.000000000000000000, 1.000000000000000000, -0.000000000000000000 ) ) ;
#2257=CARTESIAN_POINT ( 'NONE',  ( 9.457646018065525792E-16, -1.062499998634405696, 5.148502694627439702 ) ) ;
#2258=CARTESIAN_POINT ( 'NONE',  ( 4.458734125000000326, -97.14583333196773651, 2.574251347313718519 ) ) ;
#2261=CARTESIAN_POINT ( 'NONE',  ( 4.458734124999998549, -22.97916666530107221, -2.574251347313721627 ) ) ;
#2264=CARTESIAN_POINT ( 'NONE',  ( -6.972266317189433020E-16, -72.25000000000000000, -5.000000000000000000 ) ) ;
#2265=CARTESIAN_POINT ( 'NONE',  ( 1.975475456537005874E-15, 23.37500000273118417, 5.000000000000000000 ) ) ;
#2267=CARTESIAN_POINT ( 'NONE',  ( -2.229367062499996610, 15.60416666803225993, 3.861377020970582219 ) ) ;
#2268=ORIENTED_EDGE ( 'NONE', *, *, #4808, .F. ) ;
#2269=CARTESIAN_POINT ( 'NONE',  ( -2.499999999999996447, -80.83333333333332860, 4.330127018922195425 ) ) ;
#2271=CARTESIAN_POINT ( 'NONE',  ( 2.499999999999998668, -85.33333333333332860, -4.330127018922193649 ) ) ;
#2272=CARTESIAN_POINT ( 'NONE',  ( -4.458734124999999437, -17.31249999863440792, 0.000000000000000000 ) ) ;
#2273=ADVANCED_FACE ( 'NONE', ( #17818 ), #37443, .T. ) ;
#2276=CARTESIAN_POINT ( 'NONE',  ( 5.000000000000000000, -48.37499999726880873, -6.123233995736766282E-16 ) ) ;
#2278=CARTESIAN_POINT ( 'NONE',  ( -2.229367062500000163, 9.520833334698927786, -3.861377020970580443 ) ) ;
#2279=CARTESIAN_POINT ( 'NONE',  ( -2.499999999999996447, -62.70833333060214443, 4.330127018922195425 ) ) ;
#2282=CARTESIAN_POINT ( 'NONE',  ( 4.458734124999999437, -65.81249999863440792, -5.460374474430324690E-16 ) ) ;
#2283=AXIS2_PLACEMENT_3D ( 'NONE', #9713, #54096, #35441 ) ;
#2285=CARTESIAN_POINT ( 'NONE',  ( 5.000000000000000000, 1.583333333333332593, -2.886751345948129988 ) ) ;
#2288=CARTESIAN_POINT ( 'NONE',  ( -4.458734124999998549, -58.22916666530105800, 2.574251347313722516 ) ) ;
#2289=CARTESIAN_POINT ( 'NONE',  ( -5.000000000000000000, -93.87499999726881583, 0.000000000000000000 ) ) ;
#2294=CARTESIAN_POINT ( 'NONE',  ( -5.000000000000000000, -49.00000000000000000, 0.000000000000000000 ) ) ;
#2295=CARTESIAN_POINT ( 'NONE',  ( -1.339745962155599601, 18.79465819873852084, -5.000000000000007994 ) ) ;
#2297=ORIENTED_EDGE ( 'NONE', *, *, #4813, .T. ) ;
#2298=CARTESIAN_POINT ( 'NONE',  ( -2.229367062500000163, -108.4791666653010651, -3.861377020970580443 ) ) ;
#2299=CARTESIAN_POINT ( 'NONE',  ( 2.229367062500001939, -0.2291666653010705768, 3.861377020970579999 ) ) ;
#2300=CARTESIAN_POINT ( 'NONE',  ( -2.499999999999996447, -99.70833333060214443, 4.330127018922195425 ) ) ;
#2306=ORIENTED_EDGE ( 'NONE', *, *, #44904, .F. ) ;
#2308=ORIENTED_EDGE ( 'NONE', *, *, #9368, .T. ) ;
#2312=CARTESIAN_POINT ( 'NONE',  ( 9.457646018065525792E-16, -31.31249999863440436, 5.148502694627439702 ) ) ;
#2319=CARTESIAN_POINT ( 'NONE',  ( -4.458734124999999437, -77.56249999863440792, 0.000000000000000000 ) ) ;
#2321=EDGE_LOOP ( 'NONE', ( #44063, #41136, #26482, #32285 ) ) ;
#2322=DIRECTION ( 'NONE',  ( -0.000000000000000000, 1.000000000000000000, -0.000000000000000000 ) ) ;
#2324=CARTESIAN_POINT ( 'NONE',  ( -3.152548672688508926E-16, -8.812499998634406140, -5.148502694627439702 ) ) ;
#2327=CARTESIAN_POINT ( 'NONE',  ( -2.499999999999996447, -92.70833333060214443, 4.330127018922195425 ) ) ;
#2328=CARTESIAN_POINT ( 'NONE',  ( -4.458734124999999437, -8.562499998634406140, 0.000000000000000000 ) ) ;
#2335=ORIENTED_EDGE ( 'NONE', *, *, #44341, .T. ) ;
#2336=CARTESIAN_POINT ( 'NONE',  ( 4.458734124999998549, -87.72916666530107932, -2.574251347313721627 ) ) ;
#2337=CARTESIAN_POINT ( 'NONE',  ( 0.000000000000000000, -120.0000000000000000, 0.000000000000000000 ) ) ;
#2338=CARTESIAN_POINT ( 'NONE',  ( -2.229367062499996610, -1.145833331967736957, 3.861377020970582219 ) ) ;
#2341=CARTESIAN_POINT ( 'NONE',  ( 5.000000000000000888, -29.45833333060214798, 2.886751345948126879 ) ) ;
#2343=CARTESIAN_POINT ( 'NONE',  ( 2.229367062500001939, 23.02083333469892423, 3.861377020970579999 ) ) ;
#2346=CARTESIAN_POINT ( 'NONE',  ( 4.458734125000001214, -49.89583333196772941, 2.574251347313718519 ) ) ;
#2347=CARTESIAN_POINT ( 'NONE',  ( -4.458734124999997661, -39.47916666530106511, 2.574251347313722516 ) ) ;
#2349=CARTESIAN_POINT ( 'NONE',  ( -5.000000000000000000, -18.00000000000000355, 0.000000000000000000 ) ) ;
#2350=CARTESIAN_POINT ( 'NONE',  ( 5.000000000000000888, 15.41666666666666607, 2.886751345948126879 ) ) ;
#2354=CARTESIAN_POINT ( 'NONE',  ( -3.152548672688508926E-16, -43.56249999863440081, -5.148502694627439702 ) ) ;
#2355=CARTESIAN_POINT ( 'NONE',  ( -5.000000000000000000, -77.95833333060214443, -2.886751345948128211 ) ) ;
#2357=CARTESIAN_POINT ( 'NONE',  ( 1.339745962155615144, -65.58034179853029855, 4.999999999999999112 ) ) ;
#2358=CARTESIAN_POINT ( 'NONE',  ( -1.339745962155610925, -63.66965819600734022, 5.000000000000000000 ) ) ;
#2359=ADVANCED_FACE ( 'NONE', ( #20525 ), #50429, .T. ) ;
#2360=CARTESIAN_POINT ( 'NONE',  ( 9.457646018065525792E-16, -84.31249999863440792, 5.148502694627439702 ) ) ;
#2362=CARTESIAN_POINT ( 'NONE',  ( -6.972266317189433020E-16, -64.24999999999998579, -5.000000000000000000 ) ) ;
#2363=CARTESIAN_POINT ( 'NONE',  ( 2.499999999999998668, -34.33333333333332860, -4.330127018922193649 ) ) ;
#2368=CARTESIAN_POINT ( 'NONE',  ( 4.458734125000001214, -90.89583333196772230, 2.574251347313718519 ) ) ;
#2369=CARTESIAN_POINT ( 'NONE',  ( -3.152548672688508926E-16, 12.18750000136559564, -5.148502694627439702 ) ) ;
#2370=CARTESIAN_POINT ( 'NONE',  ( -4.999999999999999112, 14.20833333606451809, 2.886751345948131764 ) ) ;
#2371=CARTESIAN_POINT ( 'NONE',  ( -2.500000000000000444, -44.04166666393546592, -4.330127018922193649 ) ) ;
#2375=CARTESIAN_POINT ( 'NONE',  ( -5.000000000000000000, -52.00000000000000711, 0.000000000000000000 ) ) ;
#2376=DIRECTION ( 'NONE',  ( 0.000000000000000000, 0.000000000000000000, 1.000000000000000000 ) ) ;
#2378=CARTESIAN_POINT ( 'NONE',  ( 2.499999999999998668, -109.3333333333333428, -4.330127018922193649 ) ) ;
#2381=CARTESIAN_POINT ( 'NONE',  ( -2.500000000000000444, -43.16666666666665719, -4.330127018922193649 ) ) ;
#2382=CARTESIAN_POINT ( 'NONE',  ( 9.457646018065525792E-16, -16.31249999863440436, 5.148502694627439702 ) ) ;
#2390=ORIENTED_EDGE ( 'NONE', *, *, #52798, .F. ) ;
#2392=VERTEX_POINT ( 'NONE', #53967 ) ;
#2393=CARTESIAN_POINT ( 'NONE',  ( 4.458734124999998549, -63.97916666530107221, -2.574251347313721627 ) ) ;
#2401=ORIENTED_EDGE ( 'NONE', *, *, #36542, .T. ) ;
#2402=CARTESIAN_POINT ( 'NONE',  ( 4.458734124999999437, 8.187500001365595637, -5.460374474430324690E-16 ) ) ;
#2407=CARTESIAN_POINT ( 'NONE',  ( 2.229367062499998831, -70.64583333196773651, -3.861377020970580887 ) ) ;
#2408=CARTESIAN_POINT ( 'NONE',  ( 2.229367062499998831, 12.35416666803226171, -3.861377020970580887 ) ) ;
#2409=( BOUNDED_CURVE ( )  B_SPLINE_CURVE ( 2, ( #60001, #11092, #55497, #10139, #59678, #19788, #50339, #25575, #24940 ),
 .UNSPECIFIED., .F., .F. ) 
 B_SPLINE_CURVE_WITH_KNOTS ( ( 3, 2, 2, 2, 3 ),
 ( 0.3875000000000000111, 0.3880952380952381042, 0.3892857142857142905, 0.3904761904761904767, 0.3910714285714285698 ),
 .UNSPECIFIED. ) 
 CURVE ( )  GEOMETRIC_REPRESENTATION_ITEM ( )  RATIONAL_B_SPLINE_CURVE ( ( 0.9330127018922194093, 0.9330127018922194093, 1.000000000000000000, 0.8660254037844387076, 1.000000000000000000, 0.8660254037844387076, 1.000000000000000000, 0.9330127018922194093, 0.9330127018922194093 ) ) 
 REPRESENTATION_ITEM ( '' )  );
#2410=CARTESIAN_POINT ( 'NONE',  ( 1.975475456537005874E-15, -69.62499999726880162, 5.000000000000000000 ) ) ;
#2411=ADVANCED_FACE ( 'NONE', ( #60084 ), #30472, .T. ) ;
#2412=CARTESIAN_POINT ( 'NONE',  ( -5.000000000000000000, -42.08333333333333570, -2.886751345948128211 ) ) ;
#2413=EDGE_CURVE ( 'NONE', #58748, #60011, #44630, .T. ) ;
#2414=CARTESIAN_POINT ( 'NONE',  ( -4.458734124999998549, -54.47916666530107932, 2.574251347313722516 ) ) ;
#2415=CARTESIAN_POINT ( 'NONE',  ( -2.499999999999996447, -14.70833333060214976, 4.330127018922195425 ) ) ;
#2416=CARTESIAN_POINT ( 'NONE',  ( -1.339745962155613812, -100.2053418012614685, -5.000000000000000000 ) ) ;
#2420=CARTESIAN_POINT ( 'NONE',  ( -4.458734124999999437, -19.64583333196774362, -2.574251347313719407 ) ) ;
#2422=CARTESIAN_POINT ( 'NONE',  ( -4.999999999999998224, -101.9166666666666572, 2.886751345948131764 ) ) ;
#2423=CARTESIAN_POINT ( 'NONE',  ( 4.458734125000001214, -106.8958333319677649, 2.574251347313718519 ) ) ;
#2426=CARTESIAN_POINT ( 'NONE',  ( 2.229367062500001939, -102.2291666653010651, 3.861377020970579999 ) ) ;
#2427=CARTESIAN_POINT ( 'NONE',  ( -2.229367062500000163, -26.47916666530106866, -3.861377020970580443 ) ) ;
#2428=CARTESIAN_POINT ( 'NONE',  ( 2.499999999999998668, -65.20833333060213022, -4.330127018922193649 ) ) ;
#2433=CARTESIAN_POINT ( 'NONE',  ( 4.458734124999998549, -25.72916666530107221, -2.574251347313721627 ) ) ;
#2435=CARTESIAN_POINT ( 'NONE',  ( 4.458734124999999437, -70.06249999863439371, -5.460374474430324690E-16 ) ) ;
#2438=CARTESIAN_POINT ( 'NONE',  ( -6.972266317189433020E-16, 6.750000000000000000, -5.000000000000000000 ) ) ;
#2440=CARTESIAN_POINT ( 'NONE',  ( 5.000000000000000000, -17.50000000000000000, -6.123233995736766282E-16 ) ) ;
#2445=LINE ( 'NONE', #36848, #63314 ) ;
#2446=CARTESIAN_POINT ( 'NONE',  ( 0.000000000000000000, -120.0000000000000000, 0.000000000000000000 ) ) ;
#2447=ADVANCED_FACE ( 'NONE', ( #11177 ), #20197, .T. ) ;
#2449=DIRECTION ( 'NONE',  ( -0.000000000000000000, 1.000000000000000000, -0.000000000000000000 ) ) ;
#2451=CARTESIAN_POINT ( 'NONE',  ( 1.975475456537005874E-15, -5.750000000000000000, 5.000000000000000000 ) ) ;
#2455=ORIENTED_EDGE ( 'NONE', *, *, #3063, .T. ) ;
#2462=ORIENTED_EDGE ( 'NONE', *, *, #3084, .T. ) ;
#2472=CARTESIAN_POINT ( 'NONE',  ( -2.229367062500000163, -78.47916666530106511, -3.861377020970580443 ) ) ;
#2473=CARTESIAN_POINT ( 'NONE',  ( -4.458734124999999437, 25.60416666803225993, -2.574251347313719407 ) ) ;
#2476=DIRECTION ( 'NONE',  ( -0.000000000000000000, 1.000000000000000000, -0.000000000000000000 ) ) ;
#2480=CARTESIAN_POINT ( 'NONE',  ( 2.500000000000002220, 0.4583333360645182042, 4.330127018922192761 ) ) ;
#2481=CARTESIAN_POINT ( 'NONE',  ( -1.339745962155610925, -82.79465819873851729, 5.000000000000000000 ) ) ;
#2482=( BOUNDED_CURVE ( )  B_SPLINE_CURVE ( 2, ( #63473, #34830, #58640, #14878, #24220, #10058, #34486, #54120, #53802 ),
 .UNSPECIFIED., .F., .F. ) 
 B_SPLINE_CURVE_WITH_KNOTS ( ( 3, 2, 2, 2, 3 ),
 ( 0.5124999999999999556, 0.5130952380952380487, 0.5142857142857142350, 0.5154761904761904212, 0.5160714285714286254 ),
 .UNSPECIFIED. ) 
 CURVE ( )  GEOMETRIC_REPRESENTATION_ITEM ( )  RATIONAL_B_SPLINE_CURVE ( ( 0.9330127018922194093, 0.9330127018922194093, 1.000000000000000000, 0.8660254037844387076, 1.000000000000000000, 0.8660254037844387076, 1.000000000000000000, 0.9330127018922130810, 0.9330127018922194093 ) ) 
 REPRESENTATION_ITEM ( '' )  );
#2484=CARTESIAN_POINT ( 'NONE',  ( 9.457646018065525792E-16, -54.06249999863440081, 5.148502694627439702 ) ) ;
#2486=CARTESIAN_POINT ( 'NONE',  ( -4.458734124999999437, 28.60416666803226349, -2.574251347313719407 ) ) ;
#2487=CARTESIAN_POINT ( 'NONE',  ( -2.499999999999996447, -106.8333333333333428, 4.330127018922195425 ) ) ;
#2490=CARTESIAN_POINT ( 'NONE',  ( 2.229367062500001939, -36.22916666530107221, 3.861377020970579999 ) ) ;
#2491=CARTESIAN_POINT ( 'NONE',  ( 2.500000000000002220, 3.458333336064517205, 4.330127018922192761 ) ) ;
#2496=CARTESIAN_POINT ( 'NONE',  ( 4.458734124999999437, -104.8124999986344079, -5.460374474430324690E-16 ) ) ;
#2497=CARTESIAN_POINT ( 'NONE',  ( 4.458734124999998549, -7.979166665301073991, -2.574251347313721627 ) ) ;
#2499=CARTESIAN_POINT ( 'NONE',  ( -2.229367062500000163, -95.47916666530107932, -3.861377020970580443 ) ) ;
#2501=CARTESIAN_POINT ( 'NONE',  ( -4.458734124999999437, -87.64583333196773651, -2.574251347313719407 ) ) ;
#2503=CARTESIAN_POINT ( 'NONE',  ( 1.339745962155615144, -2.580341798530292774, 4.999999999999999112 ) ) ;
#2505=CARTESIAN_POINT ( 'NONE',  ( 4.458734125000000326, -9.895833331967738289, 2.574251347313718519 ) ) ;
#2506=CARTESIAN_POINT ( 'NONE',  ( 9.457646018065525792E-16, 17.68750000136559564, 5.148502694627439702 ) ) ;
#2507=CARTESIAN_POINT ( 'NONE',  ( -2.229367062500000163, -51.72916666530107221, -3.861377020970580443 ) ) ;
#2508=CARTESIAN_POINT ( 'NONE',  ( -2.916731409357579869E-14, 17.37500000273118417, 5.000000000000000888 ) ) ;
#2511=CARTESIAN_POINT ( 'NONE',  ( 1.975475456537005874E-15, -38.75000000000000000, 5.000000000000000000 ) ) ;
#2513=ORIENTED_EDGE ( 'NONE', *, *, #57459, .T. ) ;
#2516=EDGE_CURVE ( 'NONE', #47219, #23230, #28945, .T. ) ;
#2517=CARTESIAN_POINT ( 'NONE',  ( -4.458734124999999437, -82.39583333196773651, -2.574251347313719407 ) ) ;
#2518=CARTESIAN_POINT ( 'NONE',  ( 4.458734124999999437, 22.93750000136559564, -5.460374474430324690E-16 ) ) ;
#2522=CARTESIAN_POINT ( 'NONE',  ( 1.975475456537005874E-15, -93.74999999999998579, 5.000000000000000000 ) ) ;
#2525=CARTESIAN_POINT ( 'NONE',  ( -5.000000000000000000, -64.00000000000000000, 0.000000000000000000 ) ) ;
#2526=FACE_OUTER_BOUND ( 'NONE', #42486, .T. ) ;
#2528=ORIENTED_EDGE ( 'NONE', *, *, #40622, .T. ) ;
#2530=CARTESIAN_POINT ( 'NONE',  ( -1.339745962155610259, 27.79465819873852084, -5.000000000000002665 ) ) ;
#2538=VERTEX_POINT ( 'NONE', #1873 ) ;
#2544=CARTESIAN_POINT ( 'NONE',  ( -2.229367062499996610, -51.39583333196773651, 3.861377020970582219 ) ) ;
#2547=CARTESIAN_POINT ( 'NONE',  ( -2.499999999999996447, -81.70833333060213022, 4.330127018922195425 ) ) ;
#2552=CARTESIAN_POINT ( 'NONE',  ( 1.975475456537005874E-15, 1.250000000000000000, 5.000000000000000000 ) ) ;
#2555=CARTESIAN_POINT ( 'NONE',  ( 2.229367062500001939, -99.22916666530105090, 3.861377020970579999 ) ) ;
#2556=CARTESIAN_POINT ( 'NONE',  ( 1.975475456537005874E-15, -35.62499999726880162, 5.000000000000000000 ) ) ;
#2560=CARTESIAN_POINT ( 'NONE',  ( 5.000000000000000000, -60.41666666666665719, -2.886751345948130876 ) ) ;
#2561=CARTESIAN_POINT ( 'NONE',  ( 2.229367062499998831, 0.3541666680322609340, -3.861377020970580887 ) ) ;
#2562=CARTESIAN_POINT ( 'NONE',  ( 9.457646018065525792E-16, -94.31249999863440792, 5.148502694627439702 ) ) ;
#2564=CARTESIAN_POINT ( 'NONE',  ( 9.457646018065525792E-16, -21.31249999863440081, 5.148502694627439702 ) ) ;
#2565=CARTESIAN_POINT ( 'NONE',  ( -5.000000000000000000, -67.08333333333332860, -2.886751345948128211 ) ) ;
#2569=CARTESIAN_POINT ( 'NONE',  ( 5.000000000000000000, 23.62500000273118417, -6.123233995736766282E-16 ) ) ;
#2571=CARTESIAN_POINT ( 'NONE',  ( 2.229367062500001939, 11.77083333469892601, 3.861377020970579999 ) ) ;
#2572=VERTEX_POINT ( 'NONE', #1550 ) ;
#2573=CARTESIAN_POINT ( 'NONE',  ( -1.339745962155610925, -4.794658198738520838, 5.000000000000000000 ) ) ;
#2574=CARTESIAN_POINT ( 'NONE',  ( 1.339745962155612702, -61.29465819873851729, -5.000000000000000000 ) ) ;
#2575=CARTESIAN_POINT ( 'NONE',  ( -2.500000000000000444, -92.16666666666665719, -4.330127018922193649 ) ) ;
#2576=CARTESIAN_POINT ( 'NONE',  ( -4.458734124999999437, -27.31249999863440081, 0.000000000000000000 ) ) ;
#2578=CARTESIAN_POINT ( 'NONE',  ( -4.458734124999999437, -70.64583333196773651, -2.574251347313719407 ) ) ;
#2582=CARTESIAN_POINT ( 'NONE',  ( -3.535250795749689387E-16, -52.12499999726881583, -5.773502691896257311 ) ) ;
#2583=CARTESIAN_POINT ( 'NONE',  ( 5.000000000000000000, -24.41666666666666430, -2.886751345948130876 ) ) ;
#2584=CARTESIAN_POINT ( 'NONE',  ( -2.229367062500000163, 10.52083333469892779, -3.861377020970580443 ) ) ;
#2585=CARTESIAN_POINT ( 'NONE',  ( 0.000000000000000000, -120.0000000000000000, 0.000000000000000000 ) ) ;
#2587=CARTESIAN_POINT ( 'NONE',  ( 4.458734124999999437, -73.81249999863440792, -5.460374474430324690E-16 ) ) ;
#2589=CARTESIAN_POINT ( 'NONE',  ( 5.000000000000000888, 1.416666666666666741, 2.886751345948126879 ) ) ;
#2592=CARTESIAN_POINT ( 'NONE',  ( -4.458734124999998549, -65.22916666530106511, 2.574251347313722516 ) ) ;
#2593=CARTESIAN_POINT ( 'NONE',  ( 5.000000000000000000, -94.29166666393547303, -2.886751345948129988 ) ) ;
#2594=AXIS2_PLACEMENT_3D ( 'NONE', #44281, #15661, #14382 ) ;
#2598=CARTESIAN_POINT ( 'NONE',  ( 5.000000000000000000, -49.41666666666667140, -2.886751345948129988 ) ) ;
#2599=CARTESIAN_POINT ( 'NONE',  ( 1.975475456537005874E-15, -22.74999999999999645, 5.000000000000000000 ) ) ;
#2600=CARTESIAN_POINT ( 'NONE',  ( -6.972266317189433020E-16, 15.75000000000000000, -5.000000000000000000 ) ) ;
#2601=ORIENTED_EDGE ( 'NONE', *, *, #27108, .F. ) ;
#2603=CARTESIAN_POINT ( 'NONE',  ( -3.152548672688508926E-16, 0.1875000013655953035, -5.148502694627439702 ) ) ;
#2607=( BOUNDED_CURVE ( )  B_SPLINE_CURVE ( 2, ( #61040, #21796, #55579, #1549, #16331, #26935, #56529, #55891, #51697 ),
 .UNSPECIFIED., .F., .F. ) 
 B_SPLINE_CURVE_WITH_KNOTS ( ( 3, 2, 2, 2, 3 ),
 ( 0.03750000000000000555, 0.03809523809523809867, 0.03928571428571428492, 0.04047619047619047811, 0.04107142857142857123 ),
 .UNSPECIFIED. ) 
 CURVE ( )  GEOMETRIC_REPRESENTATION_ITEM ( )  RATIONAL_B_SPLINE_CURVE ( ( 0.9330127018922194093, 0.9330127018922197424, 1.000000000000000000, 0.8660254037844387076, 1.000000000000000000, 0.8660254037844387076, 1.000000000000000000, 0.9330127018922194093, 0.9330127018922194093 ) ) 
 REPRESENTATION_ITEM ( '' )  );
#2608=CARTESIAN_POINT ( 'NONE',  ( -4.999999999999998224, -5.916666666666666963, 2.886751345948131764 ) ) ;
#2612=CARTESIAN_POINT ( 'NONE',  ( 2.500000000000002220, -100.5416666639354588, 4.330127018922192761 ) ) ;
#2618=CARTESIAN_POINT ( 'NONE',  ( -2.229367062499996610, -36.39583333196773651, 3.861377020970582219 ) ) ;
#2627=CARTESIAN_POINT ( 'NONE',  ( 5.000000000000000000, -70.29166666393547303, -2.886751345948130876 ) ) ;
#2628=CARTESIAN_POINT ( 'NONE',  ( 9.457646018065525792E-16, -83.31249999863440792, 5.148502694627439702 ) ) ;
#2632=DIRECTION ( 'NONE',  ( -0.000000000000000000, 1.000000000000000000, -0.000000000000000000 ) ) ;
#2634=CARTESIAN_POINT ( 'NONE',  ( -4.458734124999999437, -8.562499998634406140, 0.000000000000000000 ) ) ;
#2638=CARTESIAN_POINT ( 'NONE',  ( 2.499999999999998668, 2.791666669397851130, -4.330127018922193649 ) ) ;
#2639=CARTESIAN_POINT ( 'NONE',  ( 4.458734124999998549, -6.979166665301073103, -2.574251347313721627 ) ) ;
#2644=CARTESIAN_POINT ( 'NONE',  ( -2.229367062499996610, 26.60416666803225993, 3.861377020970582219 ) ) ;
#2646=CARTESIAN_POINT ( 'NONE',  ( -4.458734124999997661, -86.22916666530107932, 2.574251347313722516 ) ) ;
#2647=CARTESIAN_POINT ( 'NONE',  ( -6.972266317189433020E-16, -97.24999999999998579, -5.000000000000000000 ) ) ;
#2648=CARTESIAN_POINT ( 'NONE',  ( -4.458734124999999437, -10.31249999863440792, 0.000000000000000000 ) ) ;
#2649=DIRECTION ( 'NONE',  ( -0.000000000000000000, 1.000000000000000000, -0.000000000000000000 ) ) ;
#2650=FACE_OUTER_BOUND ( 'NONE', #1836, .T. ) ;
#2651=CARTESIAN_POINT ( 'NONE',  ( 2.500000000000002220, -31.54166666393548724, 4.330127018922192761 ) ) ;
#2652=CARTESIAN_POINT ( 'NONE',  ( -6.972266317189433020E-16, -23.24999999999999645, -5.000000000000000000 ) ) ;
#2653=CARTESIAN_POINT ( 'NONE',  ( 2.229367062499998831, 24.35416666803225993, -3.861377020970580887 ) ) ;
#2654=CARTESIAN_POINT ( 'NONE',  ( 5.000000000000000000, -7.500000000000000000, -6.123233995736766282E-16 ) ) ;
#2656=CARTESIAN_POINT ( 'NONE',  ( 4.458734125000001214, -51.89583333196773651, 2.574251347313718519 ) ) ;
#2659=CARTESIAN_POINT ( 'NONE',  ( -5.000000000000000000, 12.91666666666666785, -2.886751345948128211 ) ) ;
#2662=CARTESIAN_POINT ( 'NONE',  ( -2.229367062499996610, -49.14583333196772941, 3.861377020970582219 ) ) ;
#2663=CARTESIAN_POINT ( 'NONE',  ( -3.535250795749689387E-16, -81.12499999726881583, -5.773502691896257311 ) ) ;
#2667=CARTESIAN_POINT ( 'NONE',  ( -2.229367062499996610, -83.39583333196773651, 3.861377020970582219 ) ) ;
#2669=CARTESIAN_POINT ( 'NONE',  ( -2.499999999999996447, -30.83333333333333215, 4.330127018922195425 ) ) ;
#2670=CARTESIAN_POINT ( 'NONE',  ( 0.000000000000000000, -120.0000000000000000, 0.000000000000000000 ) ) ;
#2673=ORIENTED_EDGE ( 'NONE', *, *, #4895, .F. ) ;
#2674=CARTESIAN_POINT ( 'NONE',  ( 2.229367062499998831, -88.64583333196773651, -3.861377020970580887 ) ) ;
#2675=CARTESIAN_POINT ( 'NONE',  ( 2.229367062499998831, 15.10416666803225993, -3.861377020970580887 ) ) ;
#2676=CARTESIAN_POINT ( 'NONE',  ( -2.500000000000000444, 16.95833333606451987, -4.330127018922193649 ) ) ;
#2677=( BOUNDED_CURVE ( )  B_SPLINE_CURVE ( 2, ( #42016, #2481, #46540, #61656, #22094, #18211, #37832, #41693, #37207 ),
 .UNSPECIFIED., .F., .F. ) 
 B_SPLINE_CURVE_WITH_KNOTS ( ( 3, 2, 2, 2, 3 ),
 ( 0.8053571428571428825, 0.8059523809523809756, 0.8071428571428571619, 0.8083333333333333481, 0.8089285714285714413 ),
 .UNSPECIFIED. ) 
 CURVE ( )  GEOMETRIC_REPRESENTATION_ITEM ( )  RATIONAL_B_SPLINE_CURVE ( ( 0.9330127018922194093, 0.9330127018922194093, 1.000000000000000000, 0.8660254037844387076, 1.000000000000000000, 0.8660254037844387076, 1.000000000000000000, 0.9330127018922194093, 0.9330127018922194093 ) ) 
 REPRESENTATION_ITEM ( '' )  );
#2678=CARTESIAN_POINT ( 'NONE',  ( -2.499999999999996447, -34.70833333060213732, 4.330127018922195425 ) ) ;
#2681=AXIS2_PLACEMENT_3D ( 'NONE', #2146, #22705, #31706 ) ;
#2682=CARTESIAN_POINT ( 'NONE',  ( -1.339745962155613812, 14.91965820146970678, -5.000000000000000000 ) ) ;
#2683=CARTESIAN_POINT ( 'NONE',  ( 5.000000000000000000, -79.50000000000000000, -6.123233995736766282E-16 ) ) ;
#2684=CARTESIAN_POINT ( 'NONE',  ( -5.000000000000000000, 19.99999999999999645, 0.000000000000000000 ) ) ;
#2691=CARTESIAN_POINT ( 'NONE',  ( 4.458734124999999437, -19.06249999863440792, -5.460374474430324690E-16 ) ) ;
#2700=VERTEX_POINT ( 'NONE', #3054 ) ;
#2701=CARTESIAN_POINT ( 'NONE',  ( 6.123233995736766282E-16, -120.0000000000000000, -5.000000000000000000 ) ) ;
#2703=CARTESIAN_POINT ( 'NONE',  ( 2.229367062499998831, -60.89583333196774362, -3.861377020970580887 ) ) ;
#2704=CARTESIAN_POINT ( 'NONE',  ( 1.339745962155612702, -7.169658196007335782, -5.000000000000000000 ) ) ;
#2710=DIRECTION ( 'NONE',  ( 0.000000000000000000, 0.000000000000000000, 1.000000000000000000 ) ) ;
#2712=ORIENTED_EDGE ( 'NONE', *, *, #56737, .T. ) ;
#2714=CARTESIAN_POINT ( 'NONE',  ( 1.975475456537005874E-15, -45.74999999999999289, 5.000000000000000000 ) ) ;
#2716=CARTESIAN_POINT ( 'NONE',  ( 2.229367062499998831, 9.354166668032261711, -3.861377020970580887 ) ) ;
#2720=AXIS2_PLACEMENT_3D ( 'NONE', #6000, #60350, #59706 ) ;
#2721=VERTEX_POINT ( 'NONE', #47104 ) ;
#2722=CARTESIAN_POINT ( 'NONE',  ( 4.458734124999998549, -68.72916666530107932, -2.574251347313721627 ) ) ;
#2723=CARTESIAN_POINT ( 'NONE',  ( 5.000000000000000000, -10.29166666393547658, -2.886751345948130876 ) ) ;
#2724=CARTESIAN_POINT ( 'NONE',  ( 2.229367062499998831, 11.35416666803225993, -3.861377020970580887 ) ) ;
#2726=EDGE_CURVE ( 'NONE', #20337, #16995, #39645, .T. ) ;
#2727=VECTOR ( 'NONE', #57635, 1000.000000000000000 ) ;
#2729=CARTESIAN_POINT ( 'NONE',  ( -4.458734124999999437, -57.64583333196773651, -2.574251347313719407 ) ) ;
#2730=CARTESIAN_POINT ( 'NONE',  ( -3.535250795749689387E-16, -16.12499999726881228, -5.773502691896257311 ) ) ;
#2732=CARTESIAN_POINT ( 'NONE',  ( 1.975475456537005874E-15, -57.62499999726880873, 5.000000000000000000 ) ) ;
#2733=CARTESIAN_POINT ( 'NONE',  ( -4.458734124999999437, -34.39583333196772941, -2.574251347313719407 ) ) ;
#2734=CARTESIAN_POINT ( 'NONE',  ( 4.458734124999998549, -23.97916666530107577, -2.574251347313721627 ) ) ;
#2737=CARTESIAN_POINT ( 'NONE',  ( 2.229367062500001939, -107.9791666653010651, 3.861377020970579999 ) ) ;
#2740=CARTESIAN_POINT ( 'NONE',  ( -2.229367062500000163, -103.7291666653010651, -3.861377020970580443 ) ) ;
#2741=CARTESIAN_POINT ( 'NONE',  ( -4.458734124999999437, -25.31249999863440792, 0.000000000000000000 ) ) ;
#2742=CARTESIAN_POINT ( 'NONE',  ( 5.000000000000000000, -61.37499999726880873, -6.123233995736766282E-16 ) ) ;
#2746=CARTESIAN_POINT ( 'NONE',  ( -2.229367062499996610, -31.14583333196773651, 3.861377020970582219 ) ) ;
#2747=CARTESIAN_POINT ( 'NONE',  ( 9.457646018065525792E-16, -72.31249999863439371, 5.148502694627439702 ) ) ;
#2748=CARTESIAN_POINT ( 'NONE',  ( -1.339745962155613812, -40.08034179853028434, -5.000000000000000000 ) ) ;
#2750=CARTESIAN_POINT ( 'NONE',  ( 5.000000000000000000, -32.29166666393548724, -2.886751345948130876 ) ) ;
#2752=CARTESIAN_POINT ( 'NONE',  ( -4.999999999999999112, -16.91666666666666430, 2.886751345948131764 ) ) ;
#2754=VERTEX_POINT ( 'NONE', #18463 ) ;
#2757=CARTESIAN_POINT ( 'NONE',  ( -6.972266317189433020E-16, -8.124999997268814056, -5.000000000000000000 ) ) ;
#2761=CARTESIAN_POINT ( 'NONE',  ( 1.243387493232115550E-13, -20.12499999726881228, -5.000000000000000000 ) ) ;
#2762=CARTESIAN_POINT ( 'NONE',  ( -5.000000000000000000, -80.95833333060214443, -2.886751345948128211 ) ) ;
#2763=CARTESIAN_POINT ( 'NONE',  ( 0.000000000000000000, -120.0000000000000000, 5.000000000000000000 ) ) ;
#2766=ORIENTED_EDGE ( 'NONE', *, *, #63624, .T. ) ;
#2767=CARTESIAN_POINT ( 'NONE',  ( -2.500000000000000444, -30.04166666393548013, -4.330127018922193649 ) ) ;
#2769=VECTOR ( 'NONE', #9044, 1000.000000000000000 ) ;
#2774=EDGE_CURVE ( 'NONE', #57091, #47264, #46252, .T. ) ;
#2776=EDGE_CURVE ( 'NONE', #21697, #14134, #35538, .T. ) ;
#2782=CARTESIAN_POINT ( 'NONE',  ( -1.339745962155613812, -39.08034179853028434, -5.000000000000000000 ) ) ;
#2788=CARTESIAN_POINT ( 'NONE',  ( -2.229367062500000163, -81.47916666530106511, -3.861377020970580443 ) ) ;
#2790=CARTESIAN_POINT ( 'NONE',  ( 9.457646018065525792E-16, 21.93750000136559208, 5.148502694627439702 ) ) ;
#2791=CARTESIAN_POINT ( 'NONE',  ( 1.339745962155612702, -18.29465819873851729, -5.000000000000000000 ) ) ;
#2797=CARTESIAN_POINT ( 'NONE',  ( 5.000000000000000000, -74.37499999726880162, -6.123233995736766282E-16 ) ) ;
#2800=CARTESIAN_POINT ( 'NONE',  ( -2.229367062500000163, -53.47916666530107221, -3.861377020970580443 ) ) ;
#2802=CARTESIAN_POINT ( 'NONE',  ( -2.229367062499996610, 28.85416666803226349, 3.861377020970582219 ) ) ;
#2803=CARTESIAN_POINT ( 'NONE',  ( -3.535250795749689387E-16, -109.2499999999999858, -5.773502691896257311 ) ) ;
#2804=( BOUNDED_CURVE ( )  B_SPLINE_CURVE ( 2, ( #31119, #16336, #45915, #49468, #1877, #39488, #54616, #15057, #594 ),
 .UNSPECIFIED., .F., .F. ) 
 B_SPLINE_CURVE_WITH_KNOTS ( ( 3, 2, 2, 2, 3 ),
 ( 0.7553571428571428381, 0.7559523809523809312, 0.7571428571428571175, 0.7583333333333333037, 0.7589285714285713969 ),
 .UNSPECIFIED. ) 
 CURVE ( )  GEOMETRIC_REPRESENTATION_ITEM ( )  RATIONAL_B_SPLINE_CURVE ( ( 0.9330127018922194093, 0.9330127018922194093, 1.000000000000000000, 0.8660254037844387076, 1.000000000000000000, 0.8660254037844387076, 1.000000000000000000, 0.9330127018922194093, 0.9330127018922194093 ) ) 
 REPRESENTATION_ITEM ( '' )  );
#2805=CARTESIAN_POINT ( 'NONE',  ( 0.000000000000000000, -120.0000000000000000, 5.000000000000000000 ) ) ;
#2806=CARTESIAN_POINT ( 'NONE',  ( 4.458734124999999437, -38.06249999863440792, -5.460374474430324690E-16 ) ) ;
#2807=CARTESIAN_POINT ( 'NONE',  ( 1.060575238724906964E-15, 0.3750000027311871098, 5.773502691896257311 ) ) ;
#2811=CARTESIAN_POINT ( 'NONE',  ( 4.458734124999999437, -102.8124999986344079, -5.460374474430324690E-16 ) ) ;
#2812=CARTESIAN_POINT ( 'NONE',  ( -4.458734124999999437, -4.645833331967739177, -2.574251347313719407 ) ) ;
#2814=CIRCLE ( 'NONE', #11006, 5.000000000000000000 ) ;
#2816=CARTESIAN_POINT ( 'NONE',  ( 4.458734124999999437, -93.81249999863440792, -5.460374474430324690E-16 ) ) ;
#2818=CARTESIAN_POINT ( 'NONE',  ( -3.152548672688508926E-16, -88.81249999863439371, -5.148502694627439702 ) ) ;
#2821=CARTESIAN_POINT ( 'NONE',  ( 6.158835246850667461E-14, -2.124999997268816276, -4.999999999999999112 ) ) ;
#2824=CARTESIAN_POINT ( 'NONE',  ( 2.229367062500001939, -11.97916666530107044, 3.861377020970579999 ) ) ;
#2825=CARTESIAN_POINT ( 'NONE',  ( -4.458734124999999437, 18.35416666803225993, -2.574251347313719407 ) ) ;
#2826=CARTESIAN_POINT ( 'NONE',  ( 4.458734124999999437, -52.06249999863440792, -5.460374474430324690E-16 ) ) ;
#2828=CARTESIAN_POINT ( 'NONE',  ( -1.339745962155610925, -105.7946581987385315, 5.000000000000000000 ) ) ;
#2830=DIRECTION ( 'NONE',  ( -0.000000000000000000, 1.000000000000000000, -0.000000000000000000 ) ) ;
#2831=ORIENTED_EDGE ( 'NONE', *, *, #18533, .T. ) ;
#2834=CARTESIAN_POINT ( 'NONE',  ( 5.000000000000000000, 26.70833333606451632, -2.886751345948130876 ) ) ;
#2835=CARTESIAN_POINT ( 'NONE',  ( -3.152548672688508926E-16, -77.56249999863440792, -5.148502694627439702 ) ) ;
#2836=CARTESIAN_POINT ( 'NONE',  ( -3.152548672688508926E-16, 24.18750000136559564, -5.148502694627439702 ) ) ;
#2839=LINE ( 'NONE', #37245, #25673 ) ;
#2842=CARTESIAN_POINT ( 'NONE',  ( 5.000000000000000888, -62.58333333333333570, 2.886751345948126879 ) ) ;
#2843=CARTESIAN_POINT ( 'NONE',  ( 0.000000000000000000, -120.0000000000000000, 0.000000000000000000 ) ) ;
#2845=ORIENTED_EDGE ( 'NONE', *, *, #59869, .T. ) ;
#2846=CARTESIAN_POINT ( 'NONE',  ( 1.975475456537005874E-15, -18.62499999726881228, 5.000000000000000000 ) ) ;
#2847=CARTESIAN_POINT ( 'NONE',  ( 2.500000000000002220, 7.333333333333333925, 4.330127018922192761 ) ) ;
#2848=CARTESIAN_POINT ( 'NONE',  ( -5.000000000000000000, -108.9583333306021586, -2.886751345948128211 ) ) ;
#2851=CYLINDRICAL_SURFACE ( 'NONE', #652, 5.000000000000000000 ) ;
#2855=VERTEX_POINT ( 'NONE', #34186 ) ;
#2861=CARTESIAN_POINT ( 'NONE',  ( -4.458734124999998549, -53.47916666530106511, 2.574251347313722516 ) ) ;
#2863=EDGE_CURVE ( 'NONE', #20764, #3550, #59279, .T. ) ;
#2864=AXIS2_PLACEMENT_3D ( 'NONE', #6988, #26600, #46216 ) ;
#2877=CARTESIAN_POINT ( 'NONE',  ( 9.457646018065525792E-16, -99.31249999863442213, 5.148502694627439702 ) ) ;
#2880=EDGE_CURVE ( 'NONE', #63081, #9589, #45866, .T. ) ;
#2884=CARTESIAN_POINT ( 'NONE',  ( -6.972266317189433020E-16, -60.24999999999999289, -5.000000000000000000 ) ) ;
#2885=CARTESIAN_POINT ( 'NONE',  ( 2.229367062500001939, -6.979166665301073103, 3.861377020970579999 ) ) ;
#2886=CARTESIAN_POINT ( 'NONE',  ( -4.458734124999997661, -94.47916666530106511, 2.574251347313722516 ) ) ;
#2887=EDGE_CURVE ( 'NONE', #483, #4248, #10921, .T. ) ;
#2889=CARTESIAN_POINT ( 'NONE',  ( -4.458734124999999437, -20.64583333196774007, -2.574251347313719407 ) ) ;
#2896=CARTESIAN_POINT ( 'NONE',  ( 9.457646018065525792E-16, 9.687500001365593860, 5.148502694627439702 ) ) ;
#2897=VERTEX_POINT ( 'NONE', #40295 ) ;
#2898=DIRECTION ( 'NONE',  ( 0.000000000000000000, 0.000000000000000000, 1.000000000000000000 ) ) ;
#2899=CARTESIAN_POINT ( 'NONE',  ( 1.975475456537005874E-15, -61.74999999999999289, 5.000000000000000000 ) ) ;
#2900=CARTESIAN_POINT ( 'NONE',  ( 2.500000000000002220, -91.66666666666665719, 4.330127018922192761 ) ) ;
#2901=CARTESIAN_POINT ( 'NONE',  ( -2.229367062499996610, -23.14583333196773651, 3.861377020970582219 ) ) ;
#2903=CARTESIAN_POINT ( 'NONE',  ( 2.229367062500001939, -73.22916666530107932, 3.861377020970579999 ) ) ;
#2907=CARTESIAN_POINT ( 'NONE',  ( 4.458734125000000326, 6.104166668032262599, 2.574251347313718519 ) ) ;
#2908=DIRECTION ( 'NONE',  ( 0.000000000000000000, 0.000000000000000000, 1.000000000000000000 ) ) ;
#2911=CARTESIAN_POINT ( 'NONE',  ( -4.458734124999999437, -73.39583333196773651, -2.574251347313719407 ) ) ;
#2913=VECTOR ( 'NONE', #14624, 1000.000000000000000 ) ;
#2915=CARTESIAN_POINT ( 'NONE',  ( 2.499999999999998668, -1.333333333333332149, -4.330127018922193649 ) ) ;
#2918=CARTESIAN_POINT ( 'NONE',  ( 4.458734124999998549, -66.72916666530106511, -2.574251347313721627 ) ) ;
#2919=CARTESIAN_POINT ( 'NONE',  ( 5.000000000000000000, -100.3749999972688158, -6.123233995736766282E-16 ) ) ;
#2920=CARTESIAN_POINT ( 'NONE',  ( 1.975475456537005874E-15, -37.74999999999999289, 5.000000000000000000 ) ) ;
#2924=CARTESIAN_POINT ( 'NONE',  ( -3.535250795749689387E-16, -46.25000000000000000, -5.773502691896257311 ) ) ;
#2925=CARTESIAN_POINT ( 'NONE',  ( -1.339745962155610925, -22.79465819873851729, 5.000000000000000000 ) ) ;
#2926=CARTESIAN_POINT ( 'NONE',  ( -1.339745962155610925, 16.20534180126147916, 5.000000000000000000 ) ) ;
#2927=ORIENTED_EDGE ( 'NONE', *, *, #14223, .F. ) ;
#2928=CARTESIAN_POINT ( 'NONE',  ( -2.480964764533239819E-13, -94.75000000000000000, 5.000000000000000000 ) ) ;
#2932=AXIS2_PLACEMENT_3D ( 'NONE', #9738, #29342, #44147 ) ;
#2933=CARTESIAN_POINT ( 'NONE',  ( 1.975475456537005874E-15, -5.750000000000000000, 5.000000000000000000 ) ) ;
#2943=CARTESIAN_POINT ( 'NONE',  ( 2.229367062500001939, -36.22916666530107221, 3.861377020970579999 ) ) ;
#2944=LINE ( 'NONE', #61166, #46103 ) ;
#2952=CARTESIAN_POINT ( 'NONE',  ( 2.229367062500001939, -82.22916666530106511, 3.861377020970579999 ) ) ;
#2954=ORIENTED_EDGE ( 'NONE', *, *, #32208, .T. ) ;
#2957=DIRECTION ( 'NONE',  ( -0.000000000000000000, 1.000000000000000000, -0.000000000000000000 ) ) ;
#2959=CARTESIAN_POINT ( 'NONE',  ( 4.458734124999999437, -39.81249999863440081, -5.460374474430324690E-16 ) ) ;
#2960=CARTESIAN_POINT ( 'NONE',  ( 4.458734124999998549, -10.97916666530107044, -2.574251347313721627 ) ) ;
#2961=ORIENTED_EDGE ( 'NONE', *, *, #12199, .F. ) ;
#2962=DIRECTION ( 'NONE',  ( -0.000000000000000000, 1.000000000000000000, -0.000000000000000000 ) ) ;
#2963=EDGE_CURVE ( 'NONE', #7464, #1553, #17517, .T. ) ;
#2964=DIRECTION ( 'NONE',  ( -0.000000000000000000, 1.000000000000000000, -0.000000000000000000 ) ) ;
#2965=CARTESIAN_POINT ( 'NONE',  ( 2.229367062499998831, -4.895833331967740065, -3.861377020970580887 ) ) ;
#2970=CARTESIAN_POINT ( 'NONE',  ( 4.458734124999999437, 26.93750000136559564, -5.460374474430324690E-16 ) ) ;
#2972=CARTESIAN_POINT ( 'NONE',  ( 4.458734124999999437, -86.81249999863439371, -5.460374474430324690E-16 ) ) ;
#2974=CARTESIAN_POINT ( 'NONE',  ( 2.229367062500001939, -10.97916666530107044, 3.861377020970579999 ) ) ;
#2978=CARTESIAN_POINT ( 'NONE',  ( 2.500000000000002220, -35.54166666393547303, 4.330127018922192761 ) ) ;
#2980=CARTESIAN_POINT ( 'NONE',  ( -4.458734124999997661, 24.77083333469893134, 2.574251347313722516 ) ) ;
#2983=CARTESIAN_POINT ( 'NONE',  ( -2.229367062499996610, -59.14583333196773651, 3.861377020970582219 ) ) ;
#2986=CARTESIAN_POINT ( 'NONE',  ( 2.500000000000002220, 16.33333333333333215, 4.330127018922192761 ) ) ;
#2988=CARTESIAN_POINT ( 'NONE',  ( -5.000000000000000000, -46.08333333333333570, -2.886751345948128211 ) ) ;
#2989=CARTESIAN_POINT ( 'NONE',  ( -4.458734124999999437, -48.39583333196772941, -2.574251347313719407 ) ) ;
#2990=CARTESIAN_POINT ( 'NONE',  ( 5.000000000000000000, -84.37499999726880162, -6.123233995736766282E-16 ) ) ;
#2993=CARTESIAN_POINT ( 'NONE',  ( 5.000000000000000000, -37.37499999726881583, -6.123233995736766282E-16 ) ) ;
#2994=CARTESIAN_POINT ( 'NONE',  ( 1.975475456537005874E-15, -63.62499999726880873, 5.000000000000000000 ) ) ;
#2995=CARTESIAN_POINT ( 'NONE',  ( -4.458734124999997661, -84.47916666530107932, 2.574251347313722516 ) ) ;
#2997=CARTESIAN_POINT ( 'NONE',  ( -4.999999999999999112, -33.91666666666666430, 2.886751345948131764 ) ) ;
#2998=CARTESIAN_POINT ( 'NONE',  ( 5.000000000000000888, 8.541666669397853795, 2.886751345948126879 ) ) ;
#2999=EDGE_LOOP ( 'NONE', ( #61011, #60381, #46824, #52985 ) ) ;
#3002=CARTESIAN_POINT ( 'NONE',  ( -4.458734124999999437, -94.39583333196773651, -2.574251347313719407 ) ) ;
#3003=CARTESIAN_POINT ( 'NONE',  ( -4.458734124999999437, 13.43750000136559386, 0.000000000000000000 ) ) ;
#3004=CARTESIAN_POINT ( 'NONE',  ( -2.500000000000000444, 17.95833333606451632, -4.330127018922193649 ) ) ;
#3007=VECTOR ( 'NONE', #37825, 1000.000000000000000 ) ;
#3010=CARTESIAN_POINT ( 'NONE',  ( -5.000000000000000000, -82.08333333333332860, -2.886751345948128211 ) ) ;
#3012=CARTESIAN_POINT ( 'NONE',  ( 5.000000000000000888, -40.45833333060214443, 2.886751345948126879 ) ) ;
#3013=CARTESIAN_POINT ( 'NONE',  ( -1.339745962155610925, -25.66965819600733312, 5.000000000000000000 ) ) ;
#3014=CARTESIAN_POINT ( 'NONE',  ( 5.000000000000000000, -109.4166666666666572, -2.886751345948130876 ) ) ;
#3017=CARTESIAN_POINT ( 'NONE',  ( -5.000000000000000000, -43.00000000000000000, 0.000000000000000000 ) ) ;
#3018=CARTESIAN_POINT ( 'NONE',  ( -2.229367062499996610, -21.39583333196774007, 3.861377020970582219 ) ) ;
#3028=ORIENTED_EDGE ( 'NONE', *, *, #23709, .F. ) ;
#3029=CARTESIAN_POINT ( 'NONE',  ( 2.229367062500001939, -66.22916666530106511, 3.861377020970579999 ) ) ;
#3031=VERTEX_POINT ( 'NONE', #49628 ) ;
#3034=DIRECTION ( 'NONE',  ( -0.000000000000000000, 1.000000000000000000, -0.000000000000000000 ) ) ;
#3037=FACE_OUTER_BOUND ( 'NONE', #57444, .T. ) ;
#3038=CARTESIAN_POINT ( 'NONE',  ( -4.458734124999999437, 9.604166668032259935, -2.574251347313719407 ) ) ;
#3042=CARTESIAN_POINT ( 'NONE',  ( 1.975475456537005874E-15, -77.75000000000000000, 5.000000000000000000 ) ) ;
#3043=CARTESIAN_POINT ( 'NONE',  ( 0.000000000000000000, -120.0000000000000000, 0.000000000000000000 ) ) ;
#3045=CARTESIAN_POINT ( 'NONE',  ( -4.458734124999999437, -70.39583333196773651, -2.574251347313719407 ) ) ;
#3047=CARTESIAN_POINT ( 'NONE',  ( 9.457646018065525792E-16, 7.937500001365594748, 5.148502694627439702 ) ) ;
#3049=CARTESIAN_POINT ( 'NONE',  ( -6.972266317189433020E-16, -89.24999999999998579, -5.000000000000000000 ) ) ;
#3050=CARTESIAN_POINT ( 'NONE',  ( 2.229367062499998831, -59.89583333196774362, -3.861377020970580887 ) ) ;
#3051=CARTESIAN_POINT ( 'NONE',  ( -3.535250795749689387E-16, -20.12499999726881228, -5.773502691896257311 ) ) ;
#3054=CARTESIAN_POINT ( 'NONE',  ( -5.000000000000000000, 29.12500000273118417, 0.000000000000000000 ) ) ;
#3055=CARTESIAN_POINT ( 'NONE',  ( -4.458734124999999437, -38.39583333196773651, -2.574251347313719407 ) ) ;
#3056=CARTESIAN_POINT ( 'NONE',  ( 2.229367062499998831, -23.89583333196773651, -3.861377020970580887 ) ) ;
#3057=ORIENTED_EDGE ( 'NONE', *, *, #41664, .F. ) ;
#3059=CARTESIAN_POINT ( 'NONE',  ( 9.457646018065525792E-16, -108.0624999986343937, 5.148502694627439702 ) ) ;
#3062=CARTESIAN_POINT ( 'NONE',  ( 2.229367062499998831, -108.8958333319677365, -3.861377020970580887 ) ) ;
#3063=EDGE_CURVE ( 'NONE', #59413, #24823, #50379, .T. ) ;
#3064=CARTESIAN_POINT ( 'NONE',  ( 2.229367062499998831, -31.64583333196773651, -3.861377020970580887 ) ) ;
#3065=CARTESIAN_POINT ( 'NONE',  ( -2.499999999999996447, -61.70833333060214443, 4.330127018922195425 ) ) ;
#3068=CARTESIAN_POINT ( 'NONE',  ( -4.458734124999999437, -30.39583333196773651, -2.574251347313719407 ) ) ;
#3069=CARTESIAN_POINT ( 'NONE',  ( 2.229367062500001939, -67.22916666530106511, 3.861377020970579999 ) ) ;
#3072=CARTESIAN_POINT ( 'NONE',  ( 1.339745962155615144, -32.70534180126148271, 4.999999999999999112 ) ) ;
#3074=CARTESIAN_POINT ( 'NONE',  ( -2.499999999999996447, -16.83333333333333215, 4.330127018922195425 ) ) ;
#3077=CARTESIAN_POINT ( 'NONE',  ( -2.499999999999996447, -81.83333333333332860, 4.330127018922195425 ) ) ;
#3079=CARTESIAN_POINT ( 'NONE',  ( -4.999999999999998224, -86.79166666393547303, 2.886751345948131764 ) ) ;
#3082=CARTESIAN_POINT ( 'NONE',  ( 2.500000000000002220, 25.33333333333333215, 4.330127018922192761 ) ) ;
#3084=EDGE_CURVE ( 'NONE', #41255, #41671, #52460, .T. ) ;
#3086=CARTESIAN_POINT ( 'NONE',  ( 1.339745962155615144, -14.70534180126147916, 4.999999999999999112 ) ) ;
#3093=CYLINDRICAL_SURFACE ( 'NONE', #39880, 5.000000000000000000 ) ;
#3101=CARTESIAN_POINT ( 'NONE',  ( -5.000000000000000000, -12.08333333333333570, -2.886751345948128211 ) ) ;
#3106=CARTESIAN_POINT ( 'NONE',  ( -2.500000000000000444, 22.95833333606451632, -4.330127018922193649 ) ) ;
#3108=CARTESIAN_POINT ( 'NONE',  ( -2.229367062499996610, -81.14583333196773651, 3.861377020970582219 ) ) ;
#3109=CARTESIAN_POINT ( 'NONE',  ( 2.229367062499998831, 26.35416666803225993, -3.861377020970580887 ) ) ;
#3117=CARTESIAN_POINT ( 'NONE',  ( 9.457646018065525792E-16, -56.06249999863440792, 5.148502694627439702 ) ) ;
#3119=CARTESIAN_POINT ( 'NONE',  ( 2.229367062500001939, 22.02083333469892779, 3.861377020970579999 ) ) ;
#3120=CARTESIAN_POINT ( 'NONE',  ( -2.500000000000000444, -107.1666666666666572, -4.330127018922193649 ) ) ;
#3122=CARTESIAN_POINT ( 'NONE',  ( -3.152548672688508926E-16, -46.81249999863440081, -5.148502694627439702 ) ) ;
#3123=CARTESIAN_POINT ( 'NONE',  ( -2.499999999999996447, -3.708333330602147537, 4.330127018922195425 ) ) ;
#3127=CARTESIAN_POINT ( 'NONE',  ( 4.458734124999998549, -103.7291666653010651, -2.574251347313721627 ) ) ;
#3129=CARTESIAN_POINT ( 'NONE',  ( -4.458734124999999437, -6.645833331967741842, -2.574251347313719407 ) ) ;
#3131=CARTESIAN_POINT ( 'NONE',  ( -1.339745962155610925, -35.66965819600732601, 5.000000000000000000 ) ) ;
#3132=CARTESIAN_POINT ( 'NONE',  ( 4.458734124999998549, -95.72916666530109353, -2.574251347313721627 ) ) ;
#3134=CARTESIAN_POINT ( 'NONE',  ( -2.229367062500000163, -91.72916666530106511, -3.861377020970580443 ) ) ;
#3135=EDGE_CURVE ( 'NONE', #43948, #34069, #59007, .T. ) ;
#3137=DIRECTION ( 'NONE',  ( -0.000000000000000000, 1.000000000000000000, -0.000000000000000000 ) ) ;
#3139=AXIS2_PLACEMENT_3D ( 'NONE', #24468, #52495, #62143 ) ;
#3140=CARTESIAN_POINT ( 'NONE',  ( -2.229367062499996610, -14.14583333196774184, 3.861377020970582219 ) ) ;
#3141=CARTESIAN_POINT ( 'NONE',  ( -4.458734124999998549, 17.52083333469892779, 2.574251347313722516 ) ) ;
#3142=CARTESIAN_POINT ( 'NONE',  ( -4.458734124999999437, -55.64583333196773651, -2.574251347313719407 ) ) ;
#3143=CARTESIAN_POINT ( 'NONE',  ( 1.975475456537005874E-15, -68.74999999999998579, 5.000000000000000000 ) ) ;
#3150=CARTESIAN_POINT ( 'NONE',  ( 5.000000000000000888, -76.58333333333335702, 2.886751345948126879 ) ) ;
#3151=EDGE_CURVE ( 'NONE', #26615, #14537, #10538, .T. ) ;
#3152=CARTESIAN_POINT ( 'NONE',  ( -2.229367062499996610, -80.14583333196773651, 3.861377020970582219 ) ) ;
#3153=CARTESIAN_POINT ( 'NONE',  ( -2.229367062499996610, 23.60416666803225993, 3.861377020970582219 ) ) ;
#3155=LINE ( 'NONE', #28527, #6161 ) ;
#3156=EDGE_CURVE ( 'NONE', #49359, #15910, #1183, .T. ) ;
#3159=CARTESIAN_POINT ( 'NONE',  ( -5.000000000000000000, -68.99999999999998579, 0.000000000000000000 ) ) ;
#3164=CARTESIAN_POINT ( 'NONE',  ( -6.972266317189433020E-16, -34.25000000000000000, -5.000000000000000000 ) ) ;
#3165=CARTESIAN_POINT ( 'NONE',  ( 2.499999999999998668, -40.33333333333332860, -4.330127018922193649 ) ) ;
#3169=( BOUNDED_CURVE ( )  B_SPLINE_CURVE ( 2, ( #33180, #43129, #53730, #23839, #4843, #14172, #43442, #9981, #28961 ),
 .UNSPECIFIED., .F., .F. ) 
 B_SPLINE_CURVE_WITH_KNOTS ( ( 3, 2, 2, 2, 3 ),
 ( 0.8125000000000000000, 0.8130952380952380931, 0.8142857142857142794, 0.8154761904761904656, 0.8160714285714285587 ),
 .UNSPECIFIED. ) 
 CURVE ( )  GEOMETRIC_REPRESENTATION_ITEM ( )  RATIONAL_B_SPLINE_CURVE ( ( 0.9330127018922194093, 0.9330127018922194093, 1.000000000000000000, 0.8660254037844387076, 1.000000000000000000, 0.8660254037844387076, 1.000000000000000000, 0.9330127018922194093, 0.9330127018922194093 ) ) 
 REPRESENTATION_ITEM ( '' )  );
#3172=ORIENTED_EDGE ( 'NONE', *, *, #35301, .T. ) ;
#3175=ORIENTED_EDGE ( 'NONE', *, *, #41664, .T. ) ;
#3179=CARTESIAN_POINT ( 'NONE',  ( -3.152548672688508926E-16, -53.81249999863439371, -5.148502694627439702 ) ) ;
#3183=AXIS2_PLACEMENT_3D ( 'NONE', #41821, #17708, #61467 ) ;
#3185=ADVANCED_FACE ( 'NONE', ( #41874 ), #52171, .T. ) ;
#3190=FACE_OUTER_BOUND ( 'NONE', #21725, .T. ) ;
#3192=CARTESIAN_POINT ( 'NONE',  ( 4.458734124999999437, -98.06249999863440792, -5.460374474430324690E-16 ) ) ;
#3194=ORIENTED_EDGE ( 'NONE', *, *, #27163, .F. ) ;
#3198=CARTESIAN_POINT ( 'NONE',  ( 2.229367062499998831, -6.645833331967741842, -3.861377020970580887 ) ) ;
#3199=CARTESIAN_POINT ( 'NONE',  ( 2.229367062500001939, -93.22916666530106511, 3.861377020970579999 ) ) ;
#3201=CARTESIAN_POINT ( 'NONE',  ( 4.458734124999999437, -28.06249999863440081, -5.460374474430324690E-16 ) ) ;
#3202=CARTESIAN_POINT ( 'NONE',  ( -6.972266317189433020E-16, -69.24999999999998579, -5.000000000000000000 ) ) ;
#3208=CARTESIAN_POINT ( 'NONE',  ( -2.229367062499996610, 11.60416666803225993, 3.861377020970582219 ) ) ;
#3210=CARTESIAN_POINT ( 'NONE',  ( -1.339745962155610925, -52.66965819600733312, 5.000000000000000000 ) ) ;
#3211=CARTESIAN_POINT ( 'NONE',  ( 2.499999999999998668, -61.33333333333333570, -4.330127018922193649 ) ) ;
#3212=CARTESIAN_POINT ( 'NONE',  ( 5.000000000000000000, -92.50000000000000000, -6.123233995736766282E-16 ) ) ;
#3213=CARTESIAN_POINT ( 'NONE',  ( 9.457646018065525792E-16, -27.06249999863440081, 5.148502694627439702 ) ) ;
#3214=CARTESIAN_POINT ( 'NONE',  ( -1.339745962155613812, 6.919658201469707670, -5.000000000000000000 ) ) ;
#3215=CARTESIAN_POINT ( 'NONE',  ( 4.458734125000001214, -70.14583333196773651, 2.574251347313718519 ) ) ;
#3216=CYLINDRICAL_SURFACE ( 'NONE', #48840, 5.000000000000000000 ) ;
#3219=EDGE_CURVE ( 'NONE', #28403, #43327, #40978, .T. ) ;
#3221=CARTESIAN_POINT ( 'NONE',  ( -3.152548672688508926E-16, 4.437500001365595637, -5.148502694627439702 ) ) ;
#3224=EDGE_CURVE ( 'NONE', #42594, #4186, #20892, .T. ) ;
#3226=CARTESIAN_POINT ( 'NONE',  ( -4.458734124999998549, -72.22916666530107932, 2.574251347313722516 ) ) ;
#3228=CARTESIAN_POINT ( 'NONE',  ( 2.500000000000002220, -4.666666666666666075, 4.330127018922192761 ) ) ;
#3231=CARTESIAN_POINT ( 'NONE',  ( 2.229367062500001939, -61.97916666530106511, 3.861377020970579999 ) ) ;
#3232=CARTESIAN_POINT ( 'NONE',  ( 5.000000000000000000, -98.37499999726881583, -6.123233995736766282E-16 ) ) ;
#3233=EDGE_CURVE ( 'NONE', #4714, #42402, #36478, .T. ) ;
#3237=CARTESIAN_POINT ( 'NONE',  ( -2.229367062499996610, -106.3958333319677365, 3.861377020970582219 ) ) ;
#3239=CARTESIAN_POINT ( 'NONE',  ( 5.000000000000000000, -47.50000000000000000, -6.123233995736766282E-16 ) ) ;
#3243=ORIENTED_EDGE ( 'NONE', *, *, #3971, .F. ) ;
#3245=( BOUNDED_CURVE ( )  B_SPLINE_CURVE ( 2, ( #58511, #49491, #63036, #53680, #5112, #33433, #48536, #14120, #59148 ),
 .UNSPECIFIED., .F., .F. ) 
 B_SPLINE_CURVE_WITH_KNOTS ( ( 3, 2, 2, 2, 3 ),
 ( 0.6839285714285714413, 0.6845238095238095344, 0.6857142857142857206, 0.6869047619047619069, 0.6875000000000000000 ),
 .UNSPECIFIED. ) 
 CURVE ( )  GEOMETRIC_REPRESENTATION_ITEM ( )  RATIONAL_B_SPLINE_CURVE ( ( 0.9330127018922194093, 0.9330127018922194093, 1.000000000000000000, 0.8660254037844387076, 1.000000000000000000, 0.8660254037844387076, 1.000000000000000000, 0.9330127018922194093, 0.9330127018922194093 ) ) 
 REPRESENTATION_ITEM ( '' )  );
#3246=CARTESIAN_POINT ( 'NONE',  ( 0.000000000000000000, -120.0000000000000000, 0.000000000000000000 ) ) ;
#3249=EDGE_CURVE ( 'NONE', #40250, #22002, #18796, .T. ) ;
#3251=CARTESIAN_POINT ( 'NONE',  ( 6.123233995736766282E-16, -120.0000000000000000, -5.000000000000000000 ) ) ;
#3254=ORIENTED_EDGE ( 'NONE', *, *, #38398, .T. ) ;
#3261=CARTESIAN_POINT ( 'NONE',  ( 4.458734124999998549, -37.97916666530107932, -2.574251347313721627 ) ) ;
#3270=CARTESIAN_POINT ( 'NONE',  ( -3.152548672688508926E-16, -84.81249999863439371, -5.148502694627439702 ) ) ;
#3272=EDGE_LOOP ( 'NONE', ( #36500, #63136, #61501, #59483 ) ) ;
#3273=CARTESIAN_POINT ( 'NONE',  ( -1.339745962155613812, -95.08034179853028434, -5.000000000000000000 ) ) ;
#3274=( BOUNDED_CURVE ( )  B_SPLINE_CURVE ( 2, ( #8834, #9451, #48378, #50200, #20630, #53210, #55033, #5824, #28753 ),
 .UNSPECIFIED., .F., .F. ) 
 B_SPLINE_CURVE_WITH_KNOTS ( ( 3, 2, 2, 2, 3 ),
 ( 0.2017857142857142905, 0.2023809523809523836, 0.2035714285714285698, 0.2047619047619047561, 0.2053571428571428492 ),
 .UNSPECIFIED. ) 
 CURVE ( )  GEOMETRIC_REPRESENTATION_ITEM ( )  RATIONAL_B_SPLINE_CURVE ( ( 0.9330127018922194093, 0.9330127018922194093, 1.000000000000000000, 0.8660254037844387076, 1.000000000000000000, 0.8660254037844387076, 1.000000000000000000, 0.9330127018922194093, 0.9330127018922194093 ) ) 
 REPRESENTATION_ITEM ( '' )  );
#3277=CARTESIAN_POINT ( 'NONE',  ( 4.458734124999998549, -8.979166665301073991, -2.574251347313721627 ) ) ;
#3280=CARTESIAN_POINT ( 'NONE',  ( 2.229367062499998831, -6.895833331967741842, -3.861377020970580887 ) ) ;
#3285=CARTESIAN_POINT ( 'NONE',  ( 4.458734124999999437, 27.93750000136559208, -5.460374474430324690E-16 ) ) ;
#3287=CARTESIAN_POINT ( 'NONE',  ( 9.457646018065525792E-16, -92.06249999863439371, 5.148502694627439702 ) ) ;
#3289=CARTESIAN_POINT ( 'NONE',  ( 4.458734125000001214, -9.895833331967736513, 2.574251347313718519 ) ) ;
#3292=CARTESIAN_POINT ( 'NONE',  ( -2.500000000000000444, 14.83333333333333215, -4.330127018922193649 ) ) ;
#3293=CARTESIAN_POINT ( 'NONE',  ( 5.000000000000000888, -33.45833333060215153, 2.886751345948126879 ) ) ;
#3295=CARTESIAN_POINT ( 'NONE',  ( -4.458734124999997661, 18.77083333469892779, 2.574251347313722516 ) ) ;
#3297=CARTESIAN_POINT ( 'NONE',  ( 4.458734125000001214, -55.89583333196773651, 2.574251347313718519 ) ) ;
#3300=CARTESIAN_POINT ( 'NONE',  ( 5.000000000000000000, 12.58333333333333215, -2.886751345948129988 ) ) ;
#3302=CARTESIAN_POINT ( 'NONE',  ( -5.000000000000000000, -46.00000000000000000, 0.000000000000000000 ) ) ;
#3303=CARTESIAN_POINT ( 'NONE',  ( 4.458734124999998549, -50.72916666530107932, -2.574251347313721627 ) ) ;
#3304=CARTESIAN_POINT ( 'NONE',  ( 2.500000000000002220, -85.54166666393547303, 4.330127018922192761 ) ) ;
#3308=CARTESIAN_POINT ( 'NONE',  ( -3.152548672688508926E-16, -86.81249999863439371, -5.148502694627439702 ) ) ;
#3310=CARTESIAN_POINT ( 'NONE',  ( 5.000000000000000888, -33.58333333333332860, 2.886751345948126879 ) ) ;
#3315=ORIENTED_EDGE ( 'NONE', *, *, #51602, .T. ) ;
#3316=CARTESIAN_POINT ( 'NONE',  ( -2.229367062499996610, -98.14583333196773651, 3.861377020970582219 ) ) ;
#3317=CARTESIAN_POINT ( 'NONE',  ( 2.229367062499998831, 7.104166668032259935, -3.861377020970580887 ) ) ;
#3318=CARTESIAN_POINT ( 'NONE',  ( -2.499999999999996447, 10.29166666939785024, 4.330127018922195425 ) ) ;
#3319=CARTESIAN_POINT ( 'NONE',  ( -4.999999999999998224, -43.79166666393546592, 2.886751345948131764 ) ) ;
#3323=CARTESIAN_POINT ( 'NONE',  ( -4.999999999999998224, -39.91666666666667140, 2.886751345948131764 ) ) ;
#3324=CARTESIAN_POINT ( 'NONE',  ( -2.499999999999996447, -80.83333333333332860, 4.330127018922195425 ) ) ;
#3325=EDGE_CURVE ( 'NONE', #42376, #58224, #10165, .T. ) ;
#3328=CARTESIAN_POINT ( 'NONE',  ( 1.339745962155612702, -63.29465819873851729, -5.000000000000000000 ) ) ;
#3333=CARTESIAN_POINT ( 'NONE',  ( 2.229367062500001939, -19.22916666530106866, 3.861377020970579999 ) ) ;
#3341=ORIENTED_EDGE ( 'NONE', *, *, #11857, .F. ) ;
#3343=ORIENTED_EDGE ( 'NONE', *, *, #42928, .T. ) ;
#3344=CARTESIAN_POINT ( 'NONE',  ( -4.458734124999999437, -67.56249999863440792, 0.000000000000000000 ) ) ;
#3345=CARTESIAN_POINT ( 'NONE',  ( -6.972266317189433020E-16, -16.25000000000000000, -5.000000000000000000 ) ) ;
#3351=CARTESIAN_POINT ( 'NONE',  ( 0.000000000000000000, -120.0000000000000000, 0.000000000000000000 ) ) ;
#3352=CARTESIAN_POINT ( 'NONE',  ( -4.458734124999999437, 10.60416666803225993, -2.574251347313719407 ) ) ;
#3355=CARTESIAN_POINT ( 'NONE',  ( -5.000000000000000000, 6.125000002731185056, 0.000000000000000000 ) ) ;
#3357=ORIENTED_EDGE ( 'NONE', *, *, #61839, .F. ) ;
#3358=CARTESIAN_POINT ( 'NONE',  ( -4.458734124999999437, -72.39583333196773651, -2.574251347313719407 ) ) ;
#3359=CARTESIAN_POINT ( 'NONE',  ( -1.336351044127974539E-14, 22.24999999999999645, 5.000000000000000000 ) ) ;
#3360=CARTESIAN_POINT ( 'NONE',  ( -2.229367062500000163, 8.520833334698926009, -3.861377020970580443 ) ) ;
#3362=CARTESIAN_POINT ( 'NONE',  ( 1.975475456537005874E-15, -88.74999999999998579, 5.000000000000000000 ) ) ;
#3363=CARTESIAN_POINT ( 'NONE',  ( 2.229367062500001939, -60.22916666530106511, 3.861377020970579999 ) ) ;
#3364=CARTESIAN_POINT ( 'NONE',  ( 2.499999999999998668, -19.20833333060214798, -4.330127018922193649 ) ) ;
#3366=LINE ( 'NONE', #35310, #56306 ) ;
#3367=CARTESIAN_POINT ( 'NONE',  ( 5.000000000000000000, -30.37499999726881228, -6.123233995736766282E-16 ) ) ;
#3370=CARTESIAN_POINT ( 'NONE',  ( -4.458734124999998549, -43.22916666530105800, 2.574251347313722516 ) ) ;
#3371=CARTESIAN_POINT ( 'NONE',  ( 4.458734125000000326, -23.14583333196772941, 2.574251347313718519 ) ) ;
#3373=DIRECTION ( 'NONE',  ( -0.000000000000000000, 1.000000000000000000, -0.000000000000000000 ) ) ;
#3374=CARTESIAN_POINT ( 'NONE',  ( -2.229367062500000163, -108.4791666653010651, -3.861377020970580443 ) ) ;
#3377=CARTESIAN_POINT ( 'NONE',  ( -2.229367062499996610, -108.3958333319677365, 3.861377020970582219 ) ) ;
#3378=CARTESIAN_POINT ( 'NONE',  ( 2.229367062500001939, -30.97916666530107221, 3.861377020970579999 ) ) ;
#3379=CARTESIAN_POINT ( 'NONE',  ( -5.000000000000000000, -66.95833333060214443, -2.886751345948128211 ) ) ;
#3383=CARTESIAN_POINT ( 'NONE',  ( 4.458734124999998549, -29.72916666530107221, -2.574251347313721627 ) ) ;
#3384=CARTESIAN_POINT ( 'NONE',  ( 2.229367062499998831, -69.89583333196773651, -3.861377020970580887 ) ) ;
#3387=CARTESIAN_POINT ( 'NONE',  ( 5.000000000000000000, -32.37499999726880873, -6.123233995736766282E-16 ) ) ;
#3388=CARTESIAN_POINT ( 'NONE',  ( 0.000000000000000000, -120.0000000000000000, 0.000000000000000000 ) ) ;
#3389=CARTESIAN_POINT ( 'NONE',  ( 1.060575238724906964E-15, -14.75000000000000000, 5.773502691896257311 ) ) ;
#3391=ORIENTED_EDGE ( 'NONE', *, *, #468, .F. ) ;
#3392=CARTESIAN_POINT ( 'NONE',  ( -4.999999999999998224, -81.91666666666667140, 2.886751345948131764 ) ) ;
#3394=CARTESIAN_POINT ( 'NONE',  ( -3.535250795749689387E-16, 25.87500000273118772, -5.773502691896257311 ) ) ;
#3395=CARTESIAN_POINT ( 'NONE',  ( 1.339745962155612702, -81.16965819600734733, -5.000000000000000000 ) ) ;
#3404=ORIENTED_EDGE ( 'NONE', *, *, #38840, .T. ) ;
#3411=ORIENTED_EDGE ( 'NONE', *, *, #17799, .F. ) ;
#3412=( BOUNDED_CURVE ( )  B_SPLINE_CURVE ( 2, ( #11523, #60747, #55607, #7351, #45622, #16672, #21820, #27272, #36293 ),
 .UNSPECIFIED., .F., .F. ) 
 B_SPLINE_CURVE_WITH_KNOTS ( ( 3, 2, 2, 2, 3 ),
 ( 0.6196428571428571619, 0.6202380952380952550, 0.6214285714285714413, 0.6226190476190476275, 0.6232142857142857206 ),
 .UNSPECIFIED. ) 
 CURVE ( )  GEOMETRIC_REPRESENTATION_ITEM ( )  RATIONAL_B_SPLINE_CURVE ( ( 0.9330127018922194093, 0.9330127018922194093, 1.000000000000000000, 0.8660254037844387076, 1.000000000000000000, 0.8660254037844387076, 1.000000000000000000, 0.9330127018922194093, 0.9330127018922194093 ) ) 
 REPRESENTATION_ITEM ( '' )  );
#3413=CARTESIAN_POINT ( 'NONE',  ( 1.975475456537005874E-15, -11.74999999999999645, 5.000000000000000000 ) ) ;
#3416=EDGE_CURVE ( 'NONE', #54097, #21555, #54510, .T. ) ;
#3419=ORIENTED_EDGE ( 'NONE', *, *, #28398, .T. ) ;
#3420=CARTESIAN_POINT ( 'NONE',  ( 2.229367062499998831, -80.64583333196773651, -3.861377020970580887 ) ) ;
#3421=CARTESIAN_POINT ( 'NONE',  ( 4.458734124999999437, 23.18750000136559564, -5.460374474430324690E-16 ) ) ;
#3422=DIRECTION ( 'NONE',  ( 0.000000000000000000, 0.000000000000000000, 1.000000000000000000 ) ) ;
#3424=CARTESIAN_POINT ( 'NONE',  ( 2.499999999999998668, -69.20833333060214443, -4.330127018922193649 ) ) ;
#3430=CARTESIAN_POINT ( 'NONE',  ( 2.500000000000002220, 4.333333333333331261, 4.330127018922192761 ) ) ;
#3431=CARTESIAN_POINT ( 'NONE',  ( 4.458734124999998549, -53.72916666530107932, -2.574251347313721627 ) ) ;
#3433=CARTESIAN_POINT ( 'NONE',  ( -4.458734124999999437, 22.68750000136559564, 0.000000000000000000 ) ) ;
#3434=CARTESIAN_POINT ( 'NONE',  ( 5.000000000000000888, -97.58333333333332860, 2.886751345948126879 ) ) ;
#3436=CARTESIAN_POINT ( 'NONE',  ( 2.229367062499998831, -42.89583333196773651, -3.861377020970580887 ) ) ;
#3437=CARTESIAN_POINT ( 'NONE',  ( -2.499999999999996447, -2.708333330602146649, 4.330127018922195425 ) ) ;
#3441=CARTESIAN_POINT ( 'NONE',  ( -4.458734124999999437, -100.3958333319677365, -2.574251347313719407 ) ) ;
#3442=CARTESIAN_POINT ( 'NONE',  ( 4.458734124999998549, -6.979166665301073103, -2.574251347313721627 ) ) ;
#3445=CARTESIAN_POINT ( 'NONE',  ( 9.457646018065525792E-16, -91.06249999863439371, 5.148502694627439702 ) ) ;
#3447=CARTESIAN_POINT ( 'NONE',  ( -3.152548672688508926E-16, -93.81249999863440792, -5.148502694627439702 ) ) ;
#3451=CARTESIAN_POINT ( 'NONE',  ( -4.458734124999999437, -12.31249999863440259, 0.000000000000000000 ) ) ;
#3452=CARTESIAN_POINT ( 'NONE',  ( -3.152548672688508926E-16, 11.18750000136559564, -5.148502694627439702 ) ) ;
#3453=CARTESIAN_POINT ( 'NONE',  ( -4.458734124999999437, -53.56249999863439371, 0.000000000000000000 ) ) ;
#3454=CYLINDRICAL_SURFACE ( 'NONE', #36649, 5.000000000000000000 ) ;
#3457=LINE ( 'NONE', #27885, #15470 ) ;
#3458=ORIENTED_EDGE ( 'NONE', *, *, #37048, .T. ) ;
#3462=CYLINDRICAL_SURFACE ( 'NONE', #45221, 5.000000000000000000 ) ;
#3464=CARTESIAN_POINT ( 'NONE',  ( -4.458734124999999437, -81.39583333196773651, -2.574251347313719407 ) ) ;
#3465=CARTESIAN_POINT ( 'NONE',  ( -4.458734124999998549, 24.52083333469892779, 2.574251347313722516 ) ) ;
#3471=CARTESIAN_POINT ( 'NONE',  ( -5.000000000000000000, -72.08333333333332860, -2.886751345948128211 ) ) ;
#3475=CARTESIAN_POINT ( 'NONE',  ( 0.000000000000000000, -120.0000000000000000, 0.000000000000000000 ) ) ;
#3476=CARTESIAN_POINT ( 'NONE',  ( -4.999999999999998224, -108.7916666639354730, 2.886751345948131764 ) ) ;
#3482=VERTEX_POINT ( 'NONE', #15779 ) ;
#3485=ORIENTED_EDGE ( 'NONE', *, *, #31168, .F. ) ;
#3488=CARTESIAN_POINT ( 'NONE',  ( 2.229367062500001939, -51.22916666530107221, 3.861377020970579999 ) ) ;
#3496=ORIENTED_EDGE ( 'NONE', *, *, #18968, .T. ) ;
#3498=CARTESIAN_POINT ( 'NONE',  ( -2.229367062499996610, -99.39583333196773651, 3.861377020970582219 ) ) ;
#3503=CARTESIAN_POINT ( 'NONE',  ( 6.123233995736766282E-16, -120.0000000000000000, -5.000000000000000000 ) ) ;
#3504=CARTESIAN_POINT ( 'NONE',  ( 2.229367062499998831, -7.645833331967735624, -3.861377020970580887 ) ) ;
#3505=CARTESIAN_POINT ( 'NONE',  ( 2.229367062499998831, -92.89583333196773651, -3.861377020970580887 ) ) ;
#3506=AXIS2_PLACEMENT_3D ( 'NONE', #21936, #46383, #51216 ) ;
#3507=EDGE_CURVE ( 'NONE', #8539, #41687, #56207, .T. ) ;
#3509=CARTESIAN_POINT ( 'NONE',  ( 9.457646018065525792E-16, -30.31249999863440436, 5.148502694627439702 ) ) ;
#3511=CARTESIAN_POINT ( 'NONE',  ( -2.499999999999996447, -66.83333333333332860, 4.330127018922195425 ) ) ;
#3515=CARTESIAN_POINT ( 'NONE',  ( -5.000000000000000000, -34.00000000000000000, 0.000000000000000000 ) ) ;
#3517=CARTESIAN_POINT ( 'NONE',  ( 4.458734125000000326, 10.85416666803225993, 2.574251347313718519 ) ) ;
#3521=CARTESIAN_POINT ( 'NONE',  ( 1.060575238724906964E-15, -88.74999999999998579, 5.773502691896257311 ) ) ;
#3522=CARTESIAN_POINT ( 'NONE',  ( -3.152548672688508926E-16, -24.56249999863440792, -5.148502694627439702 ) ) ;
#3524=CARTESIAN_POINT ( 'NONE',  ( 2.229367062499998831, -73.89583333196773651, -3.861377020970580887 ) ) ;
#3527=EDGE_CURVE ( 'NONE', #39251, #38768, #46894, .T. ) ;
#3529=CARTESIAN_POINT ( 'NONE',  ( -4.458734124999999437, 0.6875000013655957476, 0.000000000000000000 ) ) ;
#3530=CARTESIAN_POINT ( 'NONE',  ( 4.458734124999998549, 28.02083333469892779, -2.574251347313721627 ) ) ;
#3531=CARTESIAN_POINT ( 'NONE',  ( -4.458734124999999437, -36.56249999863440792, 0.000000000000000000 ) ) ;
#3532=CARTESIAN_POINT ( 'NONE',  ( -1.339745962155610925, -3.669658196007335338, 5.000000000000000000 ) ) ;
#3534=CARTESIAN_POINT ( 'NONE',  ( -2.229367062500000163, -70.47916666530107932, -3.861377020970580443 ) ) ;
#3536=CARTESIAN_POINT ( 'NONE',  ( -5.000000000000000000, -8.000000000000000000, 0.000000000000000000 ) ) ;
#3539=CARTESIAN_POINT ( 'NONE',  ( -2.229367062499996610, -65.14583333196773651, 3.861377020970582219 ) ) ;
#3540=CARTESIAN_POINT ( 'NONE',  ( -5.000000000000000000, -100.8749999972688158, 0.000000000000000000 ) ) ;
#3544=EDGE_CURVE ( 'NONE', #28828, #31465, #43411, .T. ) ;
#3545=CARTESIAN_POINT ( 'NONE',  ( -4.458734124999999437, -106.5624999986343937, 0.000000000000000000 ) ) ;
#3547=CARTESIAN_POINT ( 'NONE',  ( -2.500000000000000444, -56.16666666666667140, -4.330127018922193649 ) ) ;
#3548=CARTESIAN_POINT ( 'NONE',  ( -5.000000000000000000, -23.00000000000000000, 0.000000000000000000 ) ) ;
#3550=VERTEX_POINT ( 'NONE', #54702 ) ;
#3551=DIRECTION ( 'NONE',  ( -0.000000000000000000, 1.000000000000000000, -0.000000000000000000 ) ) ;
#3557=( BOUNDED_CURVE ( )  B_SPLINE_CURVE ( 2, ( #44109, #54085, #44430, #14210, #58912, #49269, #53145, #34453, #53456 ),
 .UNSPECIFIED., .F., .F. ) 
 B_SPLINE_CURVE_WITH_KNOTS ( ( 3, 2, 2, 2, 3 ),
 ( 0.3589285714285714302, 0.3595238095238095233, 0.3607142857142857095, 0.3619047619047618958, 0.3624999999999999889 ),
 .UNSPECIFIED. ) 
 CURVE ( )  GEOMETRIC_REPRESENTATION_ITEM ( )  RATIONAL_B_SPLINE_CURVE ( ( 0.9330127018922194093, 0.9330127018922194093, 1.000000000000000000, 0.8660254037844387076, 1.000000000000000000, 0.8660254037844387076, 1.000000000000000000, 0.9330127018922194093, 0.9330127018922194093 ) ) 
 REPRESENTATION_ITEM ( '' )  );
#3563=VERTEX_POINT ( 'NONE', #50518 ) ;
#3567=CARTESIAN_POINT ( 'NONE',  ( -4.458734124999999437, -36.64583333196773651, -2.574251347313719407 ) ) ;
#3576=EDGE_CURVE ( 'NONE', #36690, #31117, #59855, .T. ) ;
#3578=CARTESIAN_POINT ( 'NONE',  ( 4.458734125000001214, -84.14583333196772230, 2.574251347313718519 ) ) ;
#3580=EDGE_LOOP ( 'NONE', ( #14311, #22974, #57435, #14940 ) ) ;
#3585=VERTEX_POINT ( 'NONE', #15136 ) ;
#3588=CARTESIAN_POINT ( 'NONE',  ( -3.152548672688508926E-16, -14.81249999863440436, -5.148502694627439702 ) ) ;
#3589=ADVANCED_FACE ( 'NONE', ( #5807 ), #25424, .T. ) ;
#3590=CARTESIAN_POINT ( 'NONE',  ( 0.000000000000000000, -120.0000000000000000, 0.000000000000000000 ) ) ;
#3594=CARTESIAN_POINT ( 'NONE',  ( 9.457646018065525792E-16, 24.68750000136559208, 5.148502694627439702 ) ) ;
#3596=CARTESIAN_POINT ( 'NONE',  ( -3.152548672688508926E-16, -91.56249999863440792, -5.148502694627439702 ) ) ;
#3598=DIRECTION ( 'NONE',  ( 0.000000000000000000, 0.000000000000000000, 1.000000000000000000 ) ) ;
#3599=CARTESIAN_POINT ( 'NONE',  ( -4.458734124999998549, -6.229166665301072214, 2.574251347313722516 ) ) ;
#3600=CARTESIAN_POINT ( 'NONE',  ( 1.975475456537005874E-15, -51.75000000000000000, 5.000000000000000000 ) ) ;
#3602=CARTESIAN_POINT ( 'NONE',  ( 5.000000000000000888, -36.45833333060214443, 2.886751345948126879 ) ) ;
#3604=CARTESIAN_POINT ( 'NONE',  ( -4.458734124999997661, 19.77083333469893134, 2.574251347313722516 ) ) ;
#3605=CARTESIAN_POINT ( 'NONE',  ( -2.500000000000000444, -4.166666666666666075, -4.330127018922193649 ) ) ;
#3607=CARTESIAN_POINT ( 'NONE',  ( 2.229367062499998831, -58.64583333196773651, -3.861377020970580887 ) ) ;
#3611=CARTESIAN_POINT ( 'NONE',  ( 2.500000000000002220, 9.333333333333332149, 4.330127018922192761 ) ) ;
#3614=CARTESIAN_POINT ( 'NONE',  ( 2.229367062500001939, -45.97916666530106511, 3.861377020970579999 ) ) ;
#3615=CARTESIAN_POINT ( 'NONE',  ( -3.535250795749689387E-16, -86.12499999726880162, -5.773502691896257311 ) ) ;
#3618=CARTESIAN_POINT ( 'NONE',  ( -5.000000000000000000, -104.9583333306021444, -2.886751345948128211 ) ) ;
#3619=CARTESIAN_POINT ( 'NONE',  ( -4.458734124999997661, -88.47916666530107932, 2.574251347313722516 ) ) ;
#3621=CARTESIAN_POINT ( 'NONE',  ( 5.000000000000000000, -37.50000000000000711, -6.123233995736766282E-16 ) ) ;
#3622=CARTESIAN_POINT ( 'NONE',  ( 1.339745962155615144, 8.419658201469706782, 4.999999999999999112 ) ) ;
#3623=VERTEX_POINT ( 'NONE', #56622 ) ;
#3626=CARTESIAN_POINT ( 'NONE',  ( -4.458734124999998549, -97.22916666530105090, 2.574251347313722516 ) ) ;
#3627=CARTESIAN_POINT ( 'NONE',  ( -4.458734124999999437, 6.437500001365593860, 0.000000000000000000 ) ) ;
#3628=CARTESIAN_POINT ( 'NONE',  ( 5.000000000000000000, 10.70833333606452165, -2.886751345948129988 ) ) ;
#3636=CARTESIAN_POINT ( 'NONE',  ( -6.972266317189433020E-16, -109.2499999999999716, -5.000000000000000000 ) ) ;
#3638=CARTESIAN_POINT ( 'NONE',  ( -6.972266317189433020E-16, -101.1249999972688158, -5.000000000000000000 ) ) ;
#3639=SHAPE_REPRESENTATION ( 'spindle', ( #43054 ), #29681 ) ;
#3640=CARTESIAN_POINT ( 'NONE',  ( -5.000000000000000000, 24.04166666939785202, -2.886751345948128211 ) ) ;
#3641=CARTESIAN_POINT ( 'NONE',  ( 9.457646018065525792E-16, -17.31249999863440436, 5.148502694627439702 ) ) ;
#3642=DIRECTION ( 'NONE',  ( -0.000000000000000000, 1.000000000000000000, -0.000000000000000000 ) ) ;
#3650=ADVANCED_FACE ( 'NONE', ( #11895 ), #17987, .T. ) ;
#3653=ORIENTED_EDGE ( 'NONE', *, *, #12294, .F. ) ;
#3654=CARTESIAN_POINT ( 'NONE',  ( -4.458734124999998549, -70.47916666530107932, 2.574251347313722516 ) ) ;
#3657=EDGE_CURVE ( 'NONE', #44744, #47006, #61104, .T. ) ;
#3661=CARTESIAN_POINT ( 'NONE',  ( -3.152548672688508926E-16, 3.187500001365594748, -5.148502694627439702 ) ) ;
#3662=ORIENTED_EDGE ( 'NONE', *, *, #24049, .T. ) ;
#3663=CARTESIAN_POINT ( 'NONE',  ( -5.000000000000000000, -54.99999999999999289, 0.000000000000000000 ) ) ;
#3664=CARTESIAN_POINT ( 'NONE',  ( -4.458734124999999437, 1.687500001365593194, 0.000000000000000000 ) ) ;
#3668=CARTESIAN_POINT ( 'NONE',  ( -6.972266317189433020E-16, 5.875000002731184168, -5.000000000000000000 ) ) ;
#3671=EDGE_CURVE ( 'NONE', #62900, #4805, #57254, .T. ) ;
#3672=CARTESIAN_POINT ( 'NONE',  ( 4.458734125000000326, -73.89583333196773651, 2.574251347313718519 ) ) ;
#3673=CYLINDRICAL_SURFACE ( 'NONE', #48970, 5.000000000000000000 ) ;
#3674=CARTESIAN_POINT ( 'NONE',  ( -2.229367062499996610, 4.854166668032261711, 3.861377020970582219 ) ) ;
#3677=CARTESIAN_POINT ( 'NONE',  ( -4.458734124999999437, -58.56249999863440081, 0.000000000000000000 ) ) ;
#3678=CARTESIAN_POINT ( 'NONE',  ( -5.000000000000000000, -18.87499999726881583, 0.000000000000000000 ) ) ;
#3680=CARTESIAN_POINT ( 'NONE',  ( 5.000000000000000000, -42.29166666393548724, -2.886751345948130876 ) ) ;
#3682=CARTESIAN_POINT ( 'NONE',  ( -6.972266317189433020E-16, -106.1249999972688016, -5.000000000000000000 ) ) ;
#3684=CARTESIAN_POINT ( 'NONE',  ( 4.458734125000001214, -41.89583333196773651, 2.574251347313718519 ) ) ;
#3685=CARTESIAN_POINT ( 'NONE',  ( -3.152548672688508926E-16, -28.81249999863440792, -5.148502694627439702 ) ) ;
#3687=CARTESIAN_POINT ( 'NONE',  ( -5.000000000000000000, 25.91666666666666430, -2.886751345948128211 ) ) ;
#3690=CARTESIAN_POINT ( 'NONE',  ( 4.458734125000001214, -110.1458333319677507, 2.574251347313718519 ) ) ;
#3691=CARTESIAN_POINT ( 'NONE',  ( 2.229367062499998831, -34.64583333196772941, -3.861377020970580887 ) ) ;
#3692=CARTESIAN_POINT ( 'NONE',  ( -2.499999999999996447, -68.70833333060214443, 4.330127018922195425 ) ) ;
#3693=VECTOR ( 'NONE', #27014, 1000.000000000000000 ) ;
#3696=CARTESIAN_POINT ( 'NONE',  ( -3.152548672688508926E-16, -27.56249999863440081, -5.148502694627439702 ) ) ;
#3697=CARTESIAN_POINT ( 'NONE',  ( -2.229367062500000163, -72.72916666530107932, -3.861377020970580443 ) ) ;
#3702=CARTESIAN_POINT ( 'NONE',  ( -5.000000000000000000, -18.99999999999999645, 0.000000000000000000 ) ) ;
#3707=CARTESIAN_POINT ( 'NONE',  ( -2.499999999999996447, 26.29166666939785202, 4.330127018922195425 ) ) ;
#3713=CARTESIAN_POINT ( 'NONE',  ( 1.975475456537005874E-15, -80.62499999726881583, 5.000000000000000000 ) ) ;
#3715=CARTESIAN_POINT ( 'NONE',  ( -6.972266317189433020E-16, -12.24999999999999645, -5.000000000000000000 ) ) ;
#3721=EDGE_LOOP ( 'NONE', ( #43039, #8029, #29160, #50605 ) ) ;
#3725=CARTESIAN_POINT ( 'NONE',  ( -1.339745962155610925, -102.6696581960073331, 5.000000000000000000 ) ) ;
#3727=AXIS2_PLACEMENT_3D ( 'NONE', #32943, #41395, #36578 ) ;
#3728=CARTESIAN_POINT ( 'NONE',  ( -6.972266317189433020E-16, -46.12499999726880873, -5.000000000000000000 ) ) ;
#3734=CARTESIAN_POINT ( 'NONE',  ( -2.229367062499996610, -84.14583333196773651, 3.861377020970582219 ) ) ;
#3735=CARTESIAN_POINT ( 'NONE',  ( 2.229367062499998831, 20.35416666803225993, -3.861377020970580887 ) ) ;
#3736=CARTESIAN_POINT ( 'NONE',  ( 5.000000000000000000, -12.37499999726881050, -6.123233995736766282E-16 ) ) ;
#3737=ORIENTED_EDGE ( 'NONE', *, *, #54173, .F. ) ;
#3744=CARTESIAN_POINT ( 'NONE',  ( 9.457646018065525792E-16, -61.06249999863440081, 5.148502694627439702 ) ) ;
#3746=CARTESIAN_POINT ( 'NONE',  ( 4.458734125000001214, 24.10416666803226349, 2.574251347313718519 ) ) ;
#3747=CARTESIAN_POINT ( 'NONE',  ( 2.493747252781420335E-13, -42.25000000000000711, -5.000000000000000000 ) ) ;
#3749=CARTESIAN_POINT ( 'NONE',  ( -2.229367062500000163, -44.72916666530106511, -3.861377020970580443 ) ) ;
#3750=CARTESIAN_POINT ( 'NONE',  ( 5.000000000000000000, -3.291666663935477910, -2.886751345948129988 ) ) ;
#3754=CARTESIAN_POINT ( 'NONE',  ( 4.458734125000000326, -104.8958333319677365, 2.574251347313718519 ) ) ;
#3755=CARTESIAN_POINT ( 'NONE',  ( -2.229367062499996610, -12.39583333196774007, 3.861377020970582219 ) ) ;
#3757=LINE ( 'NONE', #9200, #47426 ) ;
#3758=CARTESIAN_POINT ( 'NONE',  ( 4.458734124999999437, -90.81249999863440792, -5.460374474430324690E-16 ) ) ;
#3760=CARTESIAN_POINT ( 'NONE',  ( -2.229367062500000163, -89.72916666530106511, -3.861377020970580443 ) ) ;
#3761=CARTESIAN_POINT ( 'NONE',  ( 2.499999999999998668, -53.20833333060213732, -4.330127018922193649 ) ) ;
#3764=CARTESIAN_POINT ( 'NONE',  ( -2.229367062500000163, -11.47916666530107044, -3.861377020970580443 ) ) ;
#3765=CARTESIAN_POINT ( 'NONE',  ( 4.458734124999999437, 10.93750000136559386, -5.460374474430324690E-16 ) ) ;
#3766=CARTESIAN_POINT ( 'NONE',  ( 9.457646018065525792E-16, -56.31249999863440081, 5.148502694627439702 ) ) ;
#3770=CARTESIAN_POINT ( 'NONE',  ( 1.975475456537005874E-15, -63.74999999999998579, 5.000000000000000000 ) ) ;
#3771=EDGE_LOOP ( 'NONE', ( #48876, #9479, #16547, #41357 ) ) ;
#3776=CARTESIAN_POINT ( 'NONE',  ( -4.458734124999999437, -84.39583333196773651, -2.574251347313719407 ) ) ;
#3777=CARTESIAN_POINT ( 'NONE',  ( -3.152548672688508926E-16, 23.18750000136559208, -5.148502694627439702 ) ) ;
#3778=AXIS2_PLACEMENT_3D ( 'NONE', #53921, #5360, #48770 ) ;
#3781=CARTESIAN_POINT ( 'NONE',  ( 6.123233995736766282E-16, -120.0000000000000000, -5.000000000000000000 ) ) ;
#3782=DIRECTION ( 'NONE',  ( 0.000000000000000000, 0.000000000000000000, 1.000000000000000000 ) ) ;
#3784=CARTESIAN_POINT ( 'NONE',  ( 5.000000000000000888, -70.58333333333332860, 2.886751345948126879 ) ) ;
#3787=ORIENTED_EDGE ( 'NONE', *, *, #58331, .F. ) ;
#3788=CARTESIAN_POINT ( 'NONE',  ( 5.000000000000000000, -18.37499999726881583, -6.123233995736766282E-16 ) ) ;
#3789=( BOUNDED_CURVE ( )  B_SPLINE_CURVE ( 2, ( #49664, #35512, #6562, #55133, #25220, #50944, #34876, #26499, #46114 ),
 .UNSPECIFIED., .F., .F. ) 
 B_SPLINE_CURVE_WITH_KNOTS ( ( 3, 2, 2, 2, 3 ),
 ( 0.08035714285714286309, 0.08095238095238095621, 0.08214285714285714246, 0.08333333333333332871, 0.08392857142857143571 ),
 .UNSPECIFIED. ) 
 CURVE ( )  GEOMETRIC_REPRESENTATION_ITEM ( )  RATIONAL_B_SPLINE_CURVE ( ( 0.9330127018922192983, 0.9330127018922200755, 1.000000000000000000, 0.8660254037844387076, 1.000000000000000000, 0.8660254037844387076, 1.000000000000000000, 0.9330127018922185211, 0.9330127018922192983 ) ) 
 REPRESENTATION_ITEM ( '' )  );
#3791=CARTESIAN_POINT ( 'NONE',  ( 1.975475456537005874E-15, 16.24999999999999645, 5.000000000000000000 ) ) ;
#3794=FACE_OUTER_BOUND ( 'NONE', #3890, .T. ) ;
#3800=VERTEX_POINT ( 'NONE', #61130 ) ;
#3802=CARTESIAN_POINT ( 'NONE',  ( 9.457646018065525792E-16, -57.31249999863440081, 5.148502694627439702 ) ) ;
#3809=VERTEX_POINT ( 'NONE', #46639 ) ;
#3812=CARTESIAN_POINT ( 'NONE',  ( 2.229367062500001939, -102.2291666653010651, 3.861377020970579999 ) ) ;
#3814=( BOUNDED_CURVE ( )  B_SPLINE_CURVE ( 2, ( #34936, #29771, #43310, #63576, #15314, #5349, #54228, #62945, #24011 ),
 .UNSPECIFIED., .F., .F. ) 
 B_SPLINE_CURVE_WITH_KNOTS ( ( 3, 2, 2, 2, 3 ),
 ( 0.6875000000000000000, 0.6880952380952380931, 0.6892857142857142794, 0.6904761904761904656, 0.6910714285714285587 ),
 .UNSPECIFIED. ) 
 CURVE ( )  GEOMETRIC_REPRESENTATION_ITEM ( )  RATIONAL_B_SPLINE_CURVE ( ( 0.9330127018922194093, 0.9330127018922194093, 1.000000000000000000, 0.8660254037844387076, 1.000000000000000000, 0.8660254037844387076, 1.000000000000000000, 0.9330127018922194093, 0.9330127018922194093 ) ) 
 REPRESENTATION_ITEM ( '' )  );
#3818=VECTOR ( 'NONE', #8253, 1000.000000000000000 ) ;
#3820=VECTOR ( 'NONE', #27949, 1000.000000000000000 ) ;
#3821=CARTESIAN_POINT ( 'NONE',  ( -4.458734124999999437, -6.395833331967740953, -2.574251347313719407 ) ) ;
#3822=CARTESIAN_POINT ( 'NONE',  ( -3.152548672688508926E-16, -102.8124999986344079, -5.148502694627439702 ) ) ;
#3824=CARTESIAN_POINT ( 'NONE',  ( 4.458734125000001214, -29.14583333196774362, 2.574251347313718519 ) ) ;
#3828=CARTESIAN_POINT ( 'NONE',  ( -2.499999999999996447, -90.83333333333332860, 4.330127018922195425 ) ) ;
#3831=( BOUNDED_CURVE ( )  B_SPLINE_CURVE ( 2, ( #6948, #60984, #12074, #46811, #26559, #52277, #8214, #27817, #46178 ),
 .UNSPECIFIED., .F., .F. ) 
 B_SPLINE_CURVE_WITH_KNOTS ( ( 3, 2, 2, 2, 3 ),
 ( 0.2267857142857142849, 0.2273809523809523780, 0.2285714285714285643, 0.2297619047619047505, 0.2303571428571428714 ),
 .UNSPECIFIED. ) 
 CURVE ( )  GEOMETRIC_REPRESENTATION_ITEM ( )  RATIONAL_B_SPLINE_CURVE ( ( 0.9330127018922194093, 0.9330127018922194093, 1.000000000000000000, 0.8660254037844387076, 1.000000000000000000, 0.8660254037844387076, 1.000000000000000000, 0.9330127018922178550, 0.9330127018922194093 ) ) 
 REPRESENTATION_ITEM ( '' )  );
#3832=CARTESIAN_POINT ( 'NONE',  ( 4.458734125000000326, 5.854166668032262599, 2.574251347313718519 ) ) ;
#3836=CARTESIAN_POINT ( 'NONE',  ( -5.000000000000000000, -91.00000000000000000, 0.000000000000000000 ) ) ;
#3837=CARTESIAN_POINT ( 'NONE',  ( 9.457646018065525792E-16, -26.06249999863440792, 5.148502694627439702 ) ) ;
#3838=CARTESIAN_POINT ( 'NONE',  ( -5.000000000000000000, -76.95833333060214443, -2.886751345948128211 ) ) ;
#3839=CARTESIAN_POINT ( 'NONE',  ( -4.458734124999999437, -75.64583333196775072, -2.574251347313719407 ) ) ;
#3841=CARTESIAN_POINT ( 'NONE',  ( 1.975475456537005874E-15, -79.62499999726881583, 5.000000000000000000 ) ) ;
#3843=CARTESIAN_POINT ( 'NONE',  ( -2.229367062500000163, 5.520833334698927786, -3.861377020970580443 ) ) ;
#3844=CARTESIAN_POINT ( 'NONE',  ( 9.457646018065525792E-16, 27.68750000136559208, 5.148502694627439702 ) ) ;
#3845=CARTESIAN_POINT ( 'NONE',  ( 2.229367062499998831, -39.89583333196773651, -3.861377020970580887 ) ) ;
#3849=CARTESIAN_POINT ( 'NONE',  ( 9.457646018065525792E-16, -63.06249999863440081, 5.148502694627439702 ) ) ;
#3850=CARTESIAN_POINT ( 'NONE',  ( 1.060575238724906964E-15, -99.62499999726880162, 5.773502691896257311 ) ) ;
#3852=CARTESIAN_POINT ( 'NONE',  ( 1.339745962155615144, -41.70534180126147561, 4.999999999999999112 ) ) ;
#3853=CARTESIAN_POINT ( 'NONE',  ( -1.339745962155613812, -64.20534180126146850, -5.000000000000000000 ) ) ;
#3854=CARTESIAN_POINT ( 'NONE',  ( 4.458734124999999437, -105.0624999986344079, -5.460374474430324690E-16 ) ) ;
#3856=CARTESIAN_POINT ( 'NONE',  ( 5.000000000000000000, -52.41666666666666430, -2.886751345948129988 ) ) ;
#3857=CARTESIAN_POINT ( 'NONE',  ( -6.972266317189433020E-16, -75.25000000000000000, -5.000000000000000000 ) ) ;
#3860=LINE ( 'NONE', #27040, #55105 ) ;
#3865=VECTOR ( 'NONE', #61236, 1000.000000000000000 ) ;
#3866=CARTESIAN_POINT ( 'NONE',  ( -5.000000000000000000, -30.87499999726881228, 0.000000000000000000 ) ) ;
#3870=ORIENTED_EDGE ( 'NONE', *, *, #62642, .T. ) ;
#3871=DIRECTION ( 'NONE',  ( 0.000000000000000000, 0.000000000000000000, 1.000000000000000000 ) ) ;
#3878=CARTESIAN_POINT ( 'NONE',  ( -4.458734124999998549, -33.47916666530107221, 2.574251347313722516 ) ) ;
#3879=FACE_OUTER_BOUND ( 'NONE', #42621, .T. ) ;
#3884=EDGE_CURVE ( 'NONE', #23270, #21555, #26706, .T. ) ;
#3886=CARTESIAN_POINT ( 'NONE',  ( -1.339745962155610925, -24.66965819600733667, 5.000000000000000000 ) ) ;
#3888=CARTESIAN_POINT ( 'NONE',  ( -4.458734124999999437, -84.56249999863439371, 0.000000000000000000 ) ) ;
#3890=EDGE_LOOP ( 'NONE', ( #53784, #7300, #13847, #48952 ) ) ;
#3897=ADVANCED_FACE ( 'NONE', ( #56299 ), #22203, .T. ) ;
#3898=CARTESIAN_POINT ( 'NONE',  ( 4.458734125000001214, -12.14583333196774007, 2.574251347313718519 ) ) ;
#3901=CARTESIAN_POINT ( 'NONE',  ( -6.972266317189433020E-16, -77.12499999726881583, -5.000000000000000000 ) ) ;
#3903=CARTESIAN_POINT ( 'NONE',  ( 4.458734124999998549, 24.02083333469892423, -2.574251347313721627 ) ) ;
#3904=EDGE_LOOP ( 'NONE', ( #33694, #33349, #12495, #21799 ) ) ;
#3905=CARTESIAN_POINT ( 'NONE',  ( 2.229367062499998831, -92.64583333196773651, -3.861377020970580887 ) ) ;
#3908=CARTESIAN_POINT ( 'NONE',  ( -4.458734124999998549, -7.229166665301073103, 2.574251347313722516 ) ) ;
#3911=DIRECTION ( 'NONE',  ( 0.000000000000000000, 0.000000000000000000, 1.000000000000000000 ) ) ;
#3914=CARTESIAN_POINT ( 'NONE',  ( 1.060575238724906964E-15, -35.62499999726881583, 5.773502691896257311 ) ) ;
#3915=CARTESIAN_POINT ( 'NONE',  ( 1.339745962155612702, -29.29465819873852084, -5.000000000000000000 ) ) ;
#3916=CARTESIAN_POINT ( 'NONE',  ( -3.152548672688508926E-16, 17.43750000136559564, -5.148502694627439702 ) ) ;
#3919=CARTESIAN_POINT ( 'NONE',  ( 4.458734124999999437, -55.81249999863440081, -5.460374474430324690E-16 ) ) ;
#3922=CARTESIAN_POINT ( 'NONE',  ( 2.499999999999998668, 8.666666666666666075, -4.330127018922193649 ) ) ;
#3924=CARTESIAN_POINT ( 'NONE',  ( -1.339745962155613812, -46.20534180126146850, -5.000000000000000000 ) ) ;
#3925=CARTESIAN_POINT ( 'NONE',  ( -3.152548672688508926E-16, -46.56249999863440792, -5.148502694627439702 ) ) ;
#3926=CARTESIAN_POINT ( 'NONE',  ( -5.000000000000000000, -81.95833333060213022, -2.886751345948128211 ) ) ;
#3927=EDGE_CURVE ( 'NONE', #5440, #34951, #42747, .T. ) ;
#3929=FACE_OUTER_BOUND ( 'NONE', #47982, .T. ) ;
#3930=( BOUNDED_CURVE ( )  B_SPLINE_CURVE ( 2, ( #62335, #13119, #63270, #38196, #4404, #18256, #62960, #37559, #52671 ),
 .UNSPECIFIED., .F., .F. ) 
 B_SPLINE_CURVE_WITH_KNOTS ( ( 3, 2, 2, 2, 3 ),
 ( 0.8553571428571428159, 0.8559523809523809090, 0.8571428571428570953, 0.8583333333333332815, 0.8589285714285714857 ),
 .UNSPECIFIED. ) 
 CURVE ( )  GEOMETRIC_REPRESENTATION_ITEM ( )  RATIONAL_B_SPLINE_CURVE ( ( 0.9330127018922194093, 0.9330127018922194093, 1.000000000000000000, 0.8660254037844387076, 1.000000000000000000, 0.8660254037844387076, 1.000000000000000000, 0.9330127018922130810, 0.9330127018922194093 ) ) 
 REPRESENTATION_ITEM ( '' )  );
#3931=CARTESIAN_POINT ( 'NONE',  ( -1.339745962155613812, -105.0803417985302843, -5.000000000000000000 ) ) ;
#3932=CARTESIAN_POINT ( 'NONE',  ( -4.458734124999999437, -88.56249999863439371, 0.000000000000000000 ) ) ;
#3934=CARTESIAN_POINT ( 'NONE',  ( 1.060575238724906964E-15, -36.75000000000000711, 5.773502691896257311 ) ) ;
#3935=FACE_OUTER_BOUND ( 'NONE', #43740, .T. ) ;
#3937=CARTESIAN_POINT ( 'NONE',  ( 2.500000000000002220, -22.66666666666666785, 4.330127018922192761 ) ) ;
#3938=VERTEX_POINT ( 'NONE', #53983 ) ;
#3939=CARTESIAN_POINT ( 'NONE',  ( 4.458734124999998549, -93.72916666530105090, -2.574251347313721627 ) ) ;
#3940=CARTESIAN_POINT ( 'NONE',  ( 4.458734125000001214, 5.854166668032262599, 2.574251347313718519 ) ) ;
#3941=CARTESIAN_POINT ( 'NONE',  ( 5.000000000000000000, 13.70833333606451987, -2.886751345948129988 ) ) ;
#3945=DIRECTION ( 'NONE',  ( 0.000000000000000000, -1.000000000000000000, 0.000000000000000000 ) ) ;
#3948=DIRECTION ( 'NONE',  ( -0.000000000000000000, 1.000000000000000000, -0.000000000000000000 ) ) ;
#3950=ADVANCED_FACE ( 'NONE', ( #14736 ), #30260, .T. ) ;
#3951=CARTESIAN_POINT ( 'NONE',  ( 2.499999999999998668, -19.33333333333333570, -4.330127018922193649 ) ) ;
#3954=CARTESIAN_POINT ( 'NONE',  ( -4.458734124999998549, -17.47916666530106866, 2.574251347313722516 ) ) ;
#3966=CARTESIAN_POINT ( 'NONE',  ( 9.457646018065525792E-16, -65.31249999863440792, 5.148502694627439702 ) ) ;
#3969=ORIENTED_EDGE ( 'NONE', *, *, #18886, .T. ) ;
#3971=EDGE_CURVE ( 'NONE', #35606, #62202, #62722, .T. ) ;
#3973=CARTESIAN_POINT ( 'NONE',  ( 4.458734125000001214, -0.1458333319677394824, 2.574251347313718519 ) ) ;
#3975=CARTESIAN_POINT ( 'NONE',  ( -1.339745962155610925, -54.79465819873851018, 5.000000000000000000 ) ) ;
#3978=CARTESIAN_POINT ( 'NONE',  ( -6.972266317189433020E-16, 16.74999999999999645, -5.000000000000000000 ) ) ;
#3980=( BOUNDED_CURVE ( )  B_SPLINE_CURVE ( 2, ( #21109, #20796, #40399, #544, #6324, #16287, #49735, #50056, #25615 ),
 .UNSPECIFIED., .F., .F. ) 
 B_SPLINE_CURVE_WITH_KNOTS ( ( 3, 2, 2, 2, 3 ),
 ( 0.9124999999999999778, 0.9130952380952380709, 0.9142857142857142572, 0.9154761904761904434, 0.9160714285714285365 ),
 .UNSPECIFIED. ) 
 CURVE ( )  GEOMETRIC_REPRESENTATION_ITEM ( )  RATIONAL_B_SPLINE_CURVE ( ( 0.9330127018922194093, 0.9330127018922194093, 1.000000000000000000, 0.8660254037844387076, 1.000000000000000000, 0.8660254037844387076, 1.000000000000000000, 0.9330127018922194093, 0.9330127018922194093 ) ) 
 REPRESENTATION_ITEM ( '' )  );
#3982=CARTESIAN_POINT ( 'NONE',  ( -2.229367062500000163, -78.47916666530106511, -3.861377020970580443 ) ) ;
#3984=CARTESIAN_POINT ( 'NONE',  ( 9.457646018065525792E-16, 9.937500001365592084, 5.148502694627439702 ) ) ;
#3986=CARTESIAN_POINT ( 'NONE',  ( 2.229367062499998831, -57.89583333196773651, -3.861377020970580887 ) ) ;
#3987=CARTESIAN_POINT ( 'NONE',  ( -2.499999999999996447, -21.70833333060214798, 4.330127018922195425 ) ) ;
#3988=CYLINDRICAL_SURFACE ( 'NONE', #2932, 5.000000000000000000 ) ;
#3989=CARTESIAN_POINT ( 'NONE',  ( 5.000000000000000000, -42.37499999726880873, -6.123233995736766282E-16 ) ) ;
#3991=CARTESIAN_POINT ( 'NONE',  ( 4.458734124999998549, -38.72916666530106511, -2.574251347313721627 ) ) ;
#3993=CARTESIAN_POINT ( 'NONE',  ( 4.458734124999998549, -28.97916666530108287, -2.574251347313721627 ) ) ;
#3996=CARTESIAN_POINT ( 'NONE',  ( -2.499999999999996447, 24.16666666666666785, 4.330127018922195425 ) ) ;
#3999=CARTESIAN_POINT ( 'NONE',  ( -2.229367062499996610, -109.3958333319677365, 3.861377020970582219 ) ) ;
#4001=CARTESIAN_POINT ( 'NONE',  ( 2.229367062499998831, -32.64583333196773651, -3.861377020970580887 ) ) ;
#4002=CARTESIAN_POINT ( 'NONE',  ( 1.060575238724906964E-15, -68.62499999726881583, 5.773502691896257311 ) ) ;
#4007=CARTESIAN_POINT ( 'NONE',  ( 9.457646018065525792E-16, -77.31249999863440792, 5.148502694627439702 ) ) ;
#4010=EDGE_CURVE ( 'NONE', #37866, #62194, #3860, .T. ) ;
#4011=CARTESIAN_POINT ( 'NONE',  ( -5.000000000000000000, -27.87499999726880873, 0.000000000000000000 ) ) ;
#4012=CARTESIAN_POINT ( 'NONE',  ( 5.000000000000000888, -21.58333333333332860, 2.886751345948126879 ) ) ;
#4018=CARTESIAN_POINT ( 'NONE',  ( 2.499999999999998668, 24.79166666939785202, -4.330127018922193649 ) ) ;
#4019=CARTESIAN_POINT ( 'NONE',  ( -6.972266317189433020E-16, 0.8750000027311866102, -5.000000000000000000 ) ) ;
#4022=EDGE_CURVE ( 'NONE', #24536, #2392, #18332, .T. ) ;
#4024=CARTESIAN_POINT ( 'NONE',  ( -4.999999999999998224, -51.79166666393547303, 2.886751345948131764 ) ) ;
#4025=CARTESIAN_POINT ( 'NONE',  ( 5.000000000000000888, -14.58333333333333215, 2.886751345948126879 ) ) ;
#4028=ORIENTED_EDGE ( 'NONE', *, *, #7875, .T. ) ;
#4031=EDGE_CURVE ( 'NONE', #49961, #4714, #8119, .T. ) ;
#4035=ORIENTED_EDGE ( 'NONE', *, *, #40149, .T. ) ;
#4037=ORIENTED_EDGE ( 'NONE', *, *, #26102, .F. ) ;
#4038=DIRECTION ( 'NONE',  ( -0.000000000000000000, 1.000000000000000000, -0.000000000000000000 ) ) ;
#4039=CARTESIAN_POINT ( 'NONE',  ( -1.339745962155613812, -12.20534180126147739, -5.000000000000000000 ) ) ;
#4047=EDGE_LOOP ( 'NONE', ( #37236, #3028, #58834, #32365 ) ) ;
#4048=CARTESIAN_POINT ( 'NONE',  ( -4.458734124999998549, -84.22916666530107932, 2.574251347313722516 ) ) ;
#4049=CARTESIAN_POINT ( 'NONE',  ( 2.229367062499998831, 19.35416666803225993, -3.861377020970580887 ) ) ;
#4050=CARTESIAN_POINT ( 'NONE',  ( -6.972266317189433020E-16, -18.12499999726881228, -5.000000000000000000 ) ) ;
#4055=CARTESIAN_POINT ( 'NONE',  ( 1.339745962155615144, -4.580341798530294994, 4.999999999999999112 ) ) ;
#4058=CARTESIAN_POINT ( 'NONE',  ( -4.458734124999997661, -61.22916666530106511, 2.574251347313722516 ) ) ;
#4059=CARTESIAN_POINT ( 'NONE',  ( 5.000000000000000888, 21.41666666666666430, 2.886751345948126879 ) ) ;
#4060=CARTESIAN_POINT ( 'NONE',  ( 4.458734124999999437, 23.18750000136559564, -5.460374474430324690E-16 ) ) ;
#4061=CARTESIAN_POINT ( 'NONE',  ( 5.000000000000000000, -42.41666666666667140, -2.886751345948130876 ) ) ;
#4063=CARTESIAN_POINT ( 'NONE',  ( -4.458734124999999437, -44.56249999863440081, 0.000000000000000000 ) ) ;
#4064=CARTESIAN_POINT ( 'NONE',  ( 5.000000000000000000, -2.291666663935477466, -2.886751345948129988 ) ) ;
#4068=CARTESIAN_POINT ( 'NONE',  ( -4.458734124999999437, -106.3958333319677365, -2.574251347313719407 ) ) ;
#4069=CARTESIAN_POINT ( 'NONE',  ( -2.229367062500000163, -9.729166665301068662, -3.861377020970580443 ) ) ;
#4071=CARTESIAN_POINT ( 'NONE',  ( -6.972266317189433020E-16, -46.24999999999999289, -5.000000000000000000 ) ) ;
#4072=CARTESIAN_POINT ( 'NONE',  ( 9.457646018065525792E-16, -98.06249999863440792, 5.148502694627439702 ) ) ;
#4074=CARTESIAN_POINT ( 'NONE',  ( 4.458734124999998549, -91.97916666530107932, -2.574251347313721627 ) ) ;
#4075=CARTESIAN_POINT ( 'NONE',  ( 2.499999999999998668, -54.20833333060213732, -4.330127018922193649 ) ) ;
#4079=CARTESIAN_POINT ( 'NONE',  ( -4.458734124999999437, -13.39583333196774007, -2.574251347313719407 ) ) ;
#4080=CARTESIAN_POINT ( 'NONE',  ( 2.229367062499998831, 10.10416666803225993, -3.861377020970580887 ) ) ;
#4081=CARTESIAN_POINT ( 'NONE',  ( -2.229367062499996610, -59.39583333196773651, 3.861377020970582219 ) ) ;
#4082=CARTESIAN_POINT ( 'NONE',  ( -1.339745962155610925, -68.79465819873850307, 5.000000000000000000 ) ) ;
#4083=CARTESIAN_POINT ( 'NONE',  ( 2.499999999999998668, -15.20833333060214443, -4.330127018922193649 ) ) ;
#4092=CARTESIAN_POINT ( 'NONE',  ( 4.458734124999998549, -84.72916666530106511, -2.574251347313721627 ) ) ;
#4093=CARTESIAN_POINT ( 'NONE',  ( -2.229367062499996610, 18.60416666803225993, 3.861377020970582219 ) ) ;
#4099=CARTESIAN_POINT ( 'NONE',  ( 2.499999999999998668, -70.33333333333332860, -4.330127018922193649 ) ) ;
#4102=VERTEX_POINT ( 'NONE', #44018 ) ;
#4103=CARTESIAN_POINT ( 'NONE',  ( 2.500000000000002220, -79.66666666666665719, 4.330127018922192761 ) ) ;
#4104=CARTESIAN_POINT ( 'NONE',  ( -4.999999999999998224, -79.79166666393545881, 2.886751345948131764 ) ) ;
#4108=( BOUNDED_CURVE ( )  B_SPLINE_CURVE ( 2, ( #46172, #57105, #55827, #11742, #32007, #13022, #23004, #3072, #17545 ),
 .UNSPECIFIED., .F., .F. ) 
 B_SPLINE_CURVE_WITH_KNOTS ( ( 3, 2, 2, 2, 3 ),
 ( 0.4446428571428571175, 0.4452380952380952106, 0.4464285714285714524, 0.4476190476190476386, 0.4482142857142857317 ),
 .UNSPECIFIED. ) 
 CURVE ( )  GEOMETRIC_REPRESENTATION_ITEM ( )  RATIONAL_B_SPLINE_CURVE ( ( 0.9330127018922194093, 0.9330127018922194093, 1.000000000000000000, 0.8660254037844387076, 1.000000000000000000, 0.8660254037844387076, 1.000000000000000000, 0.9330127018922194093, 0.9330127018922194093 ) ) 
 REPRESENTATION_ITEM ( '' )  );
#4109=EDGE_CURVE ( 'NONE', #44442, #20861, #49990, .T. ) ;
#4115=VERTEX_POINT ( 'NONE', #5115 ) ;
#4118=CARTESIAN_POINT ( 'NONE',  ( 2.229367062500001939, -57.22916666530107932, 3.861377020970579999 ) ) ;
#4121=ORIENTED_EDGE ( 'NONE', *, *, #11770, .F. ) ;
#4128=CARTESIAN_POINT ( 'NONE',  ( 2.229367062499998831, -104.8958333319677365, -3.861377020970580887 ) ) ;
#4133=CARTESIAN_POINT ( 'NONE',  ( -2.229367062499996610, -39.14583333196773651, 3.861377020970582219 ) ) ;
#4136=CARTESIAN_POINT ( 'NONE',  ( 2.229367062499998831, -12.64583333196774007, -3.861377020970580887 ) ) ;
#4137=CARTESIAN_POINT ( 'NONE',  ( 4.458734124999999437, -99.06249999863440792, -5.460374474430324690E-16 ) ) ;
#4139=CARTESIAN_POINT ( 'NONE',  ( 4.458734125000001214, -28.14583333196774007, 2.574251347313718519 ) ) ;
#4143=CARTESIAN_POINT ( 'NONE',  ( 1.339745962155615144, -21.58034179853029855, 4.999999999999999112 ) ) ;
#4146=CARTESIAN_POINT ( 'NONE',  ( 9.457646018065525792E-16, 3.687500001365594748, 5.148502694627439702 ) ) ;
#4147=ORIENTED_EDGE ( 'NONE', *, *, #28311, .F. ) ;
#4149=AXIS2_PLACEMENT_3D ( 'NONE', #6578, #3034, #22009 ) ;
#4150=CARTESIAN_POINT ( 'NONE',  ( -5.000000000000000000, 16.12500000273118417, 0.000000000000000000 ) ) ;
#4151=CARTESIAN_POINT ( 'NONE',  ( 5.000000000000000000, -95.41666666666667140, -2.886751345948129988 ) ) ;
#4152=CARTESIAN_POINT ( 'NONE',  ( 4.458734124999998549, -30.72916666530107221, -2.574251347313721627 ) ) ;
#4154=CARTESIAN_POINT ( 'NONE',  ( 9.457646018065525792E-16, -76.31249999863439371, 5.148502694627439702 ) ) ;
#4158=CARTESIAN_POINT ( 'NONE',  ( -2.229367062500000163, 4.520833334698926897, -3.861377020970580443 ) ) ;
#4159=CARTESIAN_POINT ( 'NONE',  ( -2.229367062500000163, 29.27083333469892779, -3.861377020970580443 ) ) ;
#4160=CARTESIAN_POINT ( 'NONE',  ( 4.458734124999999437, -44.06249999863440081, -5.460374474430324690E-16 ) ) ;
#4167=CARTESIAN_POINT ( 'NONE',  ( 4.458734124999999437, -66.81249999863440792, -5.460374474430324690E-16 ) ) ;
#4168=CARTESIAN_POINT ( 'NONE',  ( 5.000000000000000888, -102.4583333306021444, 2.886751345948126879 ) ) ;
#4170=CARTESIAN_POINT ( 'NONE',  ( 0.000000000000000000, -120.0000000000000000, 0.000000000000000000 ) ) ;
#4171=CARTESIAN_POINT ( 'NONE',  ( -4.458734124999997661, -107.4791666653010651, 2.574251347313722516 ) ) ;
#4173=CARTESIAN_POINT ( 'NONE',  ( -2.499999999999996447, -55.83333333333332860, 4.330127018922195425 ) ) ;
#4178=CARTESIAN_POINT ( 'NONE',  ( -6.972266317189433020E-16, 20.74999999999999645, -5.000000000000000000 ) ) ;
#4186=VERTEX_POINT ( 'NONE', #38565 ) ;
#4187=LINE ( 'NONE', #19596, #44621 ) ;
#4194=CARTESIAN_POINT ( 'NONE',  ( -2.229367062499996610, -40.39583333196773651, 3.861377020970582219 ) ) ;
#4201=CARTESIAN_POINT ( 'NONE',  ( 1.975475456537005874E-15, -26.74999999999999645, 5.000000000000000000 ) ) ;
#4203=CARTESIAN_POINT ( 'NONE',  ( -3.152548672688508926E-16, -89.81249999863439371, -5.148502694627439702 ) ) ;
#4206=LINE ( 'NONE', #29253, #60123 ) ;
#4209=CARTESIAN_POINT ( 'NONE',  ( 1.975475456537005874E-15, -104.7500000000000000, 5.000000000000000000 ) ) ;
#4212=ORIENTED_EDGE ( 'NONE', *, *, #58230, .T. ) ;
#4213=CARTESIAN_POINT ( 'NONE',  ( -5.000000000000000000, -14.08333333333333037, -2.886751345948128211 ) ) ;
#4214=CARTESIAN_POINT ( 'NONE',  ( -3.152548672688508926E-16, -9.812499998634406140, -5.148502694627439702 ) ) ;
#4219=CARTESIAN_POINT ( 'NONE',  ( 2.229367062500001939, 18.77083333469892779, 3.861377020970579999 ) ) ;
#4221=CARTESIAN_POINT ( 'NONE',  ( -2.229367062499996610, -93.14583333196773651, 3.861377020970582219 ) ) ;
#4223=LINE ( 'NONE', #9039, #45216 ) ;
#4224=CARTESIAN_POINT ( 'NONE',  ( 4.458734124999998549, -11.72916666530107044, -2.574251347313721627 ) ) ;
#4228=CARTESIAN_POINT ( 'NONE',  ( -3.535250795749689387E-16, -43.12499999726880162, -5.773502691896257311 ) ) ;
#4229=CARTESIAN_POINT ( 'NONE',  ( 2.229367062499998831, 17.35416666803225993, -3.861377020970580887 ) ) ;
#4230=CARTESIAN_POINT ( 'NONE',  ( 5.000000000000000888, -46.45833333060214443, 2.886751345948126879 ) ) ;
#4232=CARTESIAN_POINT ( 'NONE',  ( 2.229367062499998831, -57.64583333196773651, -3.861377020970580887 ) ) ;
#4235=CARTESIAN_POINT ( 'NONE',  ( -5.000000000000000000, 8.000000000000000000, 0.000000000000000000 ) ) ;
#4238=CARTESIAN_POINT ( 'NONE',  ( -2.229367062500000163, -51.47916666530107221, -3.861377020970580443 ) ) ;
#4239=CARTESIAN_POINT ( 'NONE',  ( -4.999999999999999112, -82.79166666393547303, 2.886751345948131764 ) ) ;
#4243=CARTESIAN_POINT ( 'NONE',  ( -3.152548672688508926E-16, -90.81249999863440792, -5.148502694627439702 ) ) ;
#4245=CARTESIAN_POINT ( 'NONE',  ( 5.000000000000000888, -36.58333333333332149, 2.886751345948126879 ) ) ;
#4246=CARTESIAN_POINT ( 'NONE',  ( -2.499999999999996447, -19.70833333060214798, 4.330127018922195425 ) ) ;
#4248=VERTEX_POINT ( 'NONE', #38880 ) ;
#4249=CARTESIAN_POINT ( 'NONE',  ( 2.229367062499998831, -93.64583333196772230, -3.861377020970580887 ) ) ;
#4250=CARTESIAN_POINT ( 'NONE',  ( 2.229367062500001939, 9.770833334698927786, 3.861377020970579999 ) ) ;
#4251=CARTESIAN_POINT ( 'NONE',  ( 2.500000000000002220, 13.45833333606451987, 4.330127018922192761 ) ) ;
#4255=CARTESIAN_POINT ( 'NONE',  ( -1.339745962155640457, 3.205341801261477830, 4.999999999999984901 ) ) ;
#4261=CARTESIAN_POINT ( 'NONE',  ( -6.972266317189433020E-16, 6.875000002731185944, -5.000000000000000000 ) ) ;
#4262=CARTESIAN_POINT ( 'NONE',  ( 9.457646018065525792E-16, -23.31249999863440436, 5.148502694627439702 ) ) ;
#4263=CARTESIAN_POINT ( 'NONE',  ( -2.499999999999996447, 22.29166666939785202, 4.330127018922195425 ) ) ;
#4271=VERTEX_POINT ( 'NONE', #14437 ) ;
#4274=CARTESIAN_POINT ( 'NONE',  ( -4.458734124999999437, -69.56249999863439371, 0.000000000000000000 ) ) ;
#4275=SURFACE_SIDE_STYLE ('',( #38986 ) ) ;
#4276=ORIENTED_EDGE ( 'NONE', *, *, #50870, .F. ) ;
#4279=EDGE_CURVE ( 'NONE', #42594, #6575, #53054, .T. ) ;
#4280=CARTESIAN_POINT ( 'NONE',  ( -4.458734124999999437, -0.6458333319677399542, -2.574251347313719407 ) ) ;
#4281=ORIENTED_EDGE ( 'NONE', *, *, #45553, .F. ) ;
#4282=( BOUNDED_CURVE ( )  B_SPLINE_CURVE ( 2, ( #21909, #41506, #35428, #23169, #42152, #27674, #27049, #32823, #13201 ),
 .UNSPECIFIED., .F., .F. ) 
 B_SPLINE_CURVE_WITH_KNOTS ( ( 3, 2, 2, 2, 3 ),
 ( 0.7946428571428570953, 0.7952380952380951884, 0.7964285714285713746, 0.7976190476190476719, 0.7982142857142857650 ),
 .UNSPECIFIED. ) 
 CURVE ( )  GEOMETRIC_REPRESENTATION_ITEM ( )  RATIONAL_B_SPLINE_CURVE ( ( 0.9330127018922194093, 0.9330127018922194093, 1.000000000000000000, 0.8660254037844387076, 1.000000000000000000, 0.8660254037844387076, 1.000000000000000000, 0.9330127018922194093, 0.9330127018922194093 ) ) 
 REPRESENTATION_ITEM ( '' )  );
#4286=CARTESIAN_POINT ( 'NONE',  ( 1.339745962155615144, 16.29465819873851729, 4.999999999999999112 ) ) ;
#4289=CARTESIAN_POINT ( 'NONE',  ( -2.229367062499996610, -75.14583333196773651, 3.861377020970582219 ) ) ;
#4291=CARTESIAN_POINT ( 'NONE',  ( -4.458734124999999437, 6.687500001365593860, 0.000000000000000000 ) ) ;
#4292=( BOUNDED_CURVE ( )  B_SPLINE_CURVE ( 2, ( #59380, #14035, #53282, #53908, #54557, #19174, #10480, #48758, #10167 ),
 .UNSPECIFIED., .F., .F. ) 
 B_SPLINE_CURVE_WITH_KNOTS ( ( 3, 2, 2, 2, 3 ),
 ( 0.8625000000000000444, 0.8630952380952381375, 0.8642857142857143238, 0.8654761904761905100, 0.8660714285714286031 ),
 .UNSPECIFIED. ) 
 CURVE ( )  GEOMETRIC_REPRESENTATION_ITEM ( )  RATIONAL_B_SPLINE_CURVE ( ( 0.9330127018922194093, 0.9330127018922194093, 1.000000000000000000, 0.8660254037844387076, 1.000000000000000000, 0.8660254037844387076, 1.000000000000000000, 0.9330127018922194093, 0.9330127018922194093 ) ) 
 REPRESENTATION_ITEM ( '' )  );
#4294=CARTESIAN_POINT ( 'NONE',  ( 4.458734125000001214, -66.14583333196772230, 2.574251347313718519 ) ) ;
#4295=CARTESIAN_POINT ( 'NONE',  ( 5.000000000000000000, -18.37499999726881583, -6.123233995736766282E-16 ) ) ;
#4298=FACE_OUTER_BOUND ( 'NONE', #20781, .T. ) ;
#4301=CARTESIAN_POINT ( 'NONE',  ( -2.229367062500000163, -42.47916666530107932, -3.861377020970580443 ) ) ;
#4302=CARTESIAN_POINT ( 'NONE',  ( -4.458734124999999437, -29.56249999863440436, 0.000000000000000000 ) ) ;
#4304=CARTESIAN_POINT ( 'NONE',  ( 5.000000000000000000, 23.50000000000000000, -6.123233995736766282E-16 ) ) ;
#4306=CARTESIAN_POINT ( 'NONE',  ( -2.229367062500000163, -107.7291666653010651, -3.861377020970580443 ) ) ;
#4307=CARTESIAN_POINT ( 'NONE',  ( -4.458734124999999437, -37.39583333196773651, -2.574251347313719407 ) ) ;
#4308=CARTESIAN_POINT ( 'NONE',  ( 2.499999999999998668, -68.20833333060214443, -4.330127018922193649 ) ) ;
#4311=CARTESIAN_POINT ( 'NONE',  ( -3.152548672688508926E-16, -72.81249999863439371, -5.148502694627439702 ) ) ;
#4316=CARTESIAN_POINT ( 'NONE',  ( -5.000000000000000000, -20.99999999999999645, 0.000000000000000000 ) ) ;
#4320=CARTESIAN_POINT ( 'NONE',  ( -6.972266317189433020E-16, -16.12499999726881228, -5.000000000000000000 ) ) ;
#4322=FACE_OUTER_BOUND ( 'NONE', #21709, .T. ) ;
#4323=CARTESIAN_POINT ( 'NONE',  ( -5.000000000000000000, -110.8749999972688016, 0.000000000000000000 ) ) ;
#4328=ADVANCED_FACE ( 'NONE', ( #29223 ), #33749, .T. ) ;
#4331=CARTESIAN_POINT ( 'NONE',  ( -2.499999999999996447, -87.70833333060214443, 4.330127018922195425 ) ) ;
#4332=CARTESIAN_POINT ( 'NONE',  ( 1.975475456537005874E-15, 0.2500000000000001665, 5.000000000000000000 ) ) ;
#4336=ORIENTED_EDGE ( 'NONE', *, *, #30666, .F. ) ;
#4338=ORIENTED_EDGE ( 'NONE', *, *, #22028, .T. ) ;
#4339=CYLINDRICAL_SURFACE ( 'NONE', #40947, 5.000000000000000000 ) ;
#4340=DIRECTION ( 'NONE',  ( -0.000000000000000000, 1.000000000000000000, -0.000000000000000000 ) ) ;
#4343=( BOUNDED_CURVE ( )  B_SPLINE_CURVE ( 2, ( #33941, #24287, #39075, #58703, #29408, #49041, #4986, #24609, #35860 ),
 .UNSPECIFIED., .F., .F. ) 
 B_SPLINE_CURVE_WITH_KNOTS ( ( 3, 2, 2, 2, 3 ),
 ( 0.9303571428571428825, 0.9309523809523809756, 0.9321428571428571619, 0.9333333333333333481, 0.9339285714285714413 ),
 .UNSPECIFIED. ) 
 CURVE ( )  GEOMETRIC_REPRESENTATION_ITEM ( )  RATIONAL_B_SPLINE_CURVE ( ( 0.9330127018922194093, 0.9330127018922194093, 1.000000000000000000, 0.8660254037844387076, 1.000000000000000000, 0.8660254037844387076, 1.000000000000000000, 0.9330127018922194093, 0.9330127018922194093 ) ) 
 REPRESENTATION_ITEM ( '' )  );
#4348=EDGE_CURVE ( 'NONE', #55556, #52254, #44659, .T. ) ;
#4351=CARTESIAN_POINT ( 'NONE',  ( -3.152548672688508926E-16, 21.43750000136559564, -5.148502694627439702 ) ) ;
#4356=CARTESIAN_POINT ( 'NONE',  ( 5.000000000000000000, -4.374999997268816720, -6.123233995736766282E-16 ) ) ;
#4359=CARTESIAN_POINT ( 'NONE',  ( 4.458734125000000326, -61.89583333196774362, 2.574251347313718519 ) ) ;
#4361=CARTESIAN_POINT ( 'NONE',  ( 2.229367062499998831, 22.35416666803225993, -3.861377020970580887 ) ) ;
#4363=CARTESIAN_POINT ( 'NONE',  ( 2.499999999999998668, -102.2083333306021444, -4.330127018922193649 ) ) ;
#4365=CARTESIAN_POINT ( 'NONE',  ( -4.458734124999999437, -46.56249999863440792, 0.000000000000000000 ) ) ;
#4366=CARTESIAN_POINT ( 'NONE',  ( -4.999999999999999112, -1.791666663935480353, 2.886751345948131764 ) ) ;
#4371=CARTESIAN_POINT ( 'NONE',  ( 6.123233995736766282E-16, -120.0000000000000000, -5.000000000000000000 ) ) ;
#4372=( BOUNDED_CURVE ( )  B_SPLINE_CURVE ( 2, ( #32527, #42177, #2638, #37359, #60071, #30461, #260, #9886, #20830 ),
 .UNSPECIFIED., .F., .F. ) 
 B_SPLINE_CURVE_WITH_KNOTS ( ( 3, 2, 2, 2, 3 ),
 ( 0.1875000000000000000, 0.1880952380952380931, 0.1892857142857142794, 0.1904761904761904656, 0.1910714285714285865 ),
 .UNSPECIFIED. ) 
 CURVE ( )  GEOMETRIC_REPRESENTATION_ITEM ( )  RATIONAL_B_SPLINE_CURVE ( ( 0.9330127018922194093, 0.9330127018922194093, 1.000000000000000000, 0.8660254037844387076, 1.000000000000000000, 0.8660254037844387076, 1.000000000000000000, 0.9330127018922178550, 0.9330127018922194093 ) ) 
 REPRESENTATION_ITEM ( '' )  );
#4373=CARTESIAN_POINT ( 'NONE',  ( -3.152548672688508926E-16, -12.81249999863440259, -5.148502694627439702 ) ) ;
#4374=ORIENTED_EDGE ( 'NONE', *, *, #21746, .T. ) ;
#4375=CARTESIAN_POINT ( 'NONE',  ( -4.458734124999998549, -98.22916666530105090, 2.574251347313722516 ) ) ;
#4377=CARTESIAN_POINT ( 'NONE',  ( 4.458734124999998549, -89.97916666530105090, -2.574251347313721627 ) ) ;
#4378=CARTESIAN_POINT ( 'NONE',  ( -5.000000000000000000, -52.95833333060214443, -2.886751345948128211 ) ) ;
#4379=CARTESIAN_POINT ( 'NONE',  ( -4.999999999999998224, -36.79166666393548013, 2.886751345948131764 ) ) ;
#4382=CARTESIAN_POINT ( 'NONE',  ( -4.458734124999999437, -19.39583333196774007, -2.574251347313719407 ) ) ;
#4383=CARTESIAN_POINT ( 'NONE',  ( 4.458734125000001214, 8.854166668032261711, 2.574251347313718519 ) ) ;
#4384=CARTESIAN_POINT ( 'NONE',  ( 2.229367062499998831, -58.89583333196773651, -3.861377020970580887 ) ) ;
#4389=ORIENTED_EDGE ( 'NONE', *, *, #22773, .T. ) ;
#4392=CARTESIAN_POINT ( 'NONE',  ( -1.339745962155610925, -8.794658198738519062, 5.000000000000000000 ) ) ;
#4394=CARTESIAN_POINT ( 'NONE',  ( 4.458734124999999437, -86.81249999863439371, -5.460374474430324690E-16 ) ) ;
#4395=CARTESIAN_POINT ( 'NONE',  ( -4.458734124999998549, 17.52083333469892779, 2.574251347313722516 ) ) ;
#4400=CARTESIAN_POINT ( 'NONE',  ( 5.000000000000000000, -70.50000000000000000, -6.123233995736766282E-16 ) ) ;
#4404=CARTESIAN_POINT ( 'NONE',  ( -5.000000000000000000, -90.00000000000000000, 0.000000000000000000 ) ) ;
#4410=VERTEX_POINT ( 'NONE', #35985 ) ;
#4414=ORIENTED_EDGE ( 'NONE', *, *, #12655, .F. ) ;
#4416=DIRECTION ( 'NONE',  ( -0.000000000000000000, 1.000000000000000000, -0.000000000000000000 ) ) ;
#4417=CARTESIAN_POINT ( 'NONE',  ( -2.229367062499996610, -59.39583333196773651, 3.861377020970582219 ) ) ;
#4425=EDGE_CURVE ( 'NONE', #2855, #56096, #38521, .T. ) ;
#4428=CARTESIAN_POINT ( 'NONE',  ( -4.458734124999998549, -104.4791666653010651, 2.574251347313722516 ) ) ;
#4429=CARTESIAN_POINT ( 'NONE',  ( -2.500000000000000444, -27.04166666393548013, -4.330127018922193649 ) ) ;
#4430=ORIENTED_EDGE ( 'NONE', *, *, #31510, .F. ) ;
#4433=CARTESIAN_POINT ( 'NONE',  ( -2.229367062499996610, -38.14583333196773651, 3.861377020970582219 ) ) ;
#4434=CARTESIAN_POINT ( 'NONE',  ( -5.000000000000000000, 1.125000002731184390, 0.000000000000000000 ) ) ;
#4435=CARTESIAN_POINT ( 'NONE',  ( 4.458734124999998549, -12.72916666530107044, -2.574251347313721627 ) ) ;
#4436=CARTESIAN_POINT ( 'NONE',  ( 4.458734124999999437, -103.0624999986344079, -5.460374474430324690E-16 ) ) ;
#4438=CARTESIAN_POINT ( 'NONE',  ( 4.458734125000001214, -27.14583333196774717, 2.574251347313718519 ) ) ;
#4443=CARTESIAN_POINT ( 'NONE',  ( 2.499999999999998668, -17.33333333333333215, -4.330127018922193649 ) ) ;
#4446=CARTESIAN_POINT ( 'NONE',  ( 4.458734124999999437, 2.937500001365594304, -5.460374474430324690E-16 ) ) ;
#4449=ADVANCED_FACE ( 'NONE', ( #41426 ), #20557, .T. ) ;
#4450=CARTESIAN_POINT ( 'NONE',  ( 6.123233995736766282E-16, -120.0000000000000000, -5.000000000000000000 ) ) ;
#4451=CARTESIAN_POINT ( 'NONE',  ( 2.499999999999998668, -96.33333333333332860, -4.330127018922193649 ) ) ;
#4452=CARTESIAN_POINT ( 'NONE',  ( 4.458734125000001214, -27.89583333196774007, 2.574251347313718519 ) ) ;
#4453=CARTESIAN_POINT ( 'NONE',  ( 5.000000000000000000, -73.50000000000000000, -6.123233995736766282E-16 ) ) ;
#4454=CARTESIAN_POINT ( 'NONE',  ( -2.229367062500000163, -74.72916666530106511, -3.861377020970580443 ) ) ;
#4456=DIRECTION ( 'NONE',  ( 0.000000000000000000, 0.000000000000000000, 1.000000000000000000 ) ) ;
#4457=AXIS2_PLACEMENT_3D ( 'NONE', #16713, #2256, #46299 ) ;
#4459=ADVANCED_FACE ( 'NONE', ( #60754 ), #40792, .T. ) ;
#4460=CARTESIAN_POINT ( 'NONE',  ( 2.229367062499998831, 2.354166668032262599, -3.861377020970580887 ) ) ;
#4461=CARTESIAN_POINT ( 'NONE',  ( -2.229367062500000163, 25.27083333469892779, -3.861377020970580443 ) ) ;
#4462=CARTESIAN_POINT ( 'NONE',  ( 4.458734125000000326, -45.14583333196774362, 2.574251347313718519 ) ) ;
#4468=CARTESIAN_POINT ( 'NONE',  ( 4.458734125000001214, -70.89583333196773651, 2.574251347313718519 ) ) ;
#4469=CARTESIAN_POINT ( 'NONE',  ( 5.000000000000000000, -104.3749999972688158, -6.123233995736766282E-16 ) ) ;
#4470=( BOUNDED_CURVE ( )  B_SPLINE_CURVE ( 2, ( #42801, #56981, #17427, #42482, #62121, #37042, #62753, #3273, #37351 ),
 .UNSPECIFIED., .F., .F. ) 
 B_SPLINE_CURVE_WITH_KNOTS ( ( 3, 2, 2, 2, 3 ),
 ( 0.8839285714285713969, 0.8845238095238094900, 0.8857142857142856762, 0.8869047619047618625, 0.8874999999999999556 ),
 .UNSPECIFIED. ) 
 CURVE ( )  GEOMETRIC_REPRESENTATION_ITEM ( )  RATIONAL_B_SPLINE_CURVE ( ( 0.9330127018922194093, 0.9330127018922194093, 1.000000000000000000, 0.8660254037844387076, 1.000000000000000000, 0.8660254037844387076, 1.000000000000000000, 0.9330127018922194093, 0.9330127018922194093 ) ) 
 REPRESENTATION_ITEM ( '' )  );
#4474=CARTESIAN_POINT ( 'NONE',  ( -4.999999999999999112, -51.91666666666667140, 2.886751345948131764 ) ) ;
#4487=DIRECTION ( 'NONE',  ( -0.000000000000000000, 1.000000000000000000, -0.000000000000000000 ) ) ;
#4493=CARTESIAN_POINT ( 'NONE',  ( -4.458734124999999437, -42.64583333196773651, -2.574251347313719407 ) ) ;
#4496=CARTESIAN_POINT ( 'NONE',  ( 1.975475456537005874E-15, -29.74999999999999645, 5.000000000000000000 ) ) ;
#4500=AXIS2_PLACEMENT_3D ( 'NONE', #34995, #35309, #54285 ) ;
#4501=EDGE_CURVE ( 'NONE', #36690, #26096, #27451, .T. ) ;
#4504=CARTESIAN_POINT ( 'NONE',  ( 4.458734125000001214, -88.14583333196773651, 2.574251347313718519 ) ) ;
#4511=ORIENTED_EDGE ( 'NONE', *, *, #52265, .T. ) ;
#4512=CARTESIAN_POINT ( 'NONE',  ( -6.972266317189433020E-16, -71.12499999726878741, -5.000000000000000000 ) ) ;
#4513=CARTESIAN_POINT ( 'NONE',  ( -2.229367062500000163, -12.72916666530107044, -3.861377020970580443 ) ) ;
#4516=CARTESIAN_POINT ( 'NONE',  ( -1.339745962155613812, 3.919658201469705894, -5.000000000000000000 ) ) ;
#4518=( BOUNDED_CURVE ( )  B_SPLINE_CURVE ( 2, ( #45378, #35100, #56, #10638, #10956, #1024, #370, #39583, #10326 ),
 .UNSPECIFIED., .F., .F. ) 
 B_SPLINE_CURVE_WITH_KNOTS ( ( 3, 2, 2, 2, 3 ),
 ( 0.9767857142857142572, 0.9773809523809523503, 0.9785714285714285365, 0.9797619047619047228, 0.9803571428571428159 ),
 .UNSPECIFIED. ) 
 CURVE ( )  GEOMETRIC_REPRESENTATION_ITEM ( )  RATIONAL_B_SPLINE_CURVE ( ( 0.9330127018922194093, 0.9330127018922194093, 1.000000000000000000, 0.8660254037844387076, 1.000000000000000000, 0.8660254037844387076, 1.000000000000000000, 0.9330127018922194093, 0.9330127018922194093 ) ) 
 REPRESENTATION_ITEM ( '' )  );
#4519=CARTESIAN_POINT ( 'NONE',  ( 4.458734125000000326, 21.85416666803225993, 2.574251347313718519 ) ) ;
#4520=ORIENTED_EDGE ( 'NONE', *, *, #47358, .F. ) ;
#4521=CARTESIAN_POINT ( 'NONE',  ( 4.458734125000000326, -90.89583333196773651, 2.574251347313718519 ) ) ;
#4524=CARTESIAN_POINT ( 'NONE',  ( 9.457646018065525792E-16, -15.06249999863440259, 5.148502694627439702 ) ) ;
#4525=CARTESIAN_POINT ( 'NONE',  ( 3.253724281355068545E-15, 28.75000000000000000, -5.000000000000000000 ) ) ;
#4526=DIRECTION ( 'NONE',  ( -0.000000000000000000, 1.000000000000000000, -0.000000000000000000 ) ) ;
#4528=CARTESIAN_POINT ( 'NONE',  ( 1.060575238724906964E-15, -40.62499999726880162, 5.773502691896257311 ) ) ;
#4529=CARTESIAN_POINT ( 'NONE',  ( 2.500000000000002220, -49.54166666393547303, 4.330127018922192761 ) ) ;
#4530=CARTESIAN_POINT ( 'NONE',  ( -2.229367062499996610, 16.85416666803225993, 3.861377020970582219 ) ) ;
#4531=CARTESIAN_POINT ( 'NONE',  ( -5.000000000000000000, 12.04166666939785202, -2.886751345948128211 ) ) ;
#4534=CARTESIAN_POINT ( 'NONE',  ( 2.229367062499998831, -64.64583333196773651, -3.861377020970580887 ) ) ;
#4536=CARTESIAN_POINT ( 'NONE',  ( -2.500000000000000444, 8.833333333333332149, -4.330127018922193649 ) ) ;
#4539=CARTESIAN_POINT ( 'NONE',  ( 2.229367062499998831, -53.64583333196773651, -3.861377020970580887 ) ) ;
#4540=CARTESIAN_POINT ( 'NONE',  ( 1.060575238724906964E-15, -89.62499999726881583, 5.773502691896257311 ) ) ;
#4544=CARTESIAN_POINT ( 'NONE',  ( 9.457646018065525792E-16, -90.31249999863439371, 5.148502694627439702 ) ) ;
#4546=CARTESIAN_POINT ( 'NONE',  ( 5.000000000000000888, -35.58333333333332860, 2.886751345948126879 ) ) ;
#4547=CARTESIAN_POINT ( 'NONE',  ( -1.339745962155610925, 19.20534180126147916, 5.000000000000000000 ) ) ;
#4550=CARTESIAN_POINT ( 'NONE',  ( -4.458734124999998549, -103.2291666653010509, 2.574251347313722516 ) ) ;
#4551=CARTESIAN_POINT ( 'NONE',  ( 9.457646018065525792E-16, 10.68750000136559386, 5.148502694627439702 ) ) ;
#4552=CARTESIAN_POINT ( 'NONE',  ( -1.339745962155613812, -44.08034179853027723, -5.000000000000000000 ) ) ;
#4558=ORIENTED_EDGE ( 'NONE', *, *, #49892, .T. ) ;
#4559=CARTESIAN_POINT ( 'NONE',  ( -1.339745962155610925, -10.79465819873852261, 5.000000000000000000 ) ) ;
#4563=CARTESIAN_POINT ( 'NONE',  ( 5.000000000000000000, 6.625000002731185944, -6.123233995736766282E-16 ) ) ;
#4564=CARTESIAN_POINT ( 'NONE',  ( -2.229367062500000163, -26.72916666530106866, -3.861377020970580443 ) ) ;
#4567=( BOUNDED_CURVE ( )  B_SPLINE_CURVE ( 2, ( #7718, #31832, #2269, #22511, #32460, #42106, #12215, #7401, #37601 ),
 .UNSPECIFIED., .F., .F. ) 
 B_SPLINE_CURVE_WITH_KNOTS ( ( 3, 2, 2, 2, 3 ),
 ( 0.7910714285714285365, 0.7916666666666666297, 0.7928571428571428159, 0.7940476190476190022, 0.7946428571428570953 ),
 .UNSPECIFIED. ) 
 CURVE ( )  GEOMETRIC_REPRESENTATION_ITEM ( )  RATIONAL_B_SPLINE_CURVE ( ( 0.9330127018922194093, 0.9330127018922194093, 1.000000000000000000, 0.8660254037844387076, 1.000000000000000000, 0.8660254037844387076, 1.000000000000000000, 0.9330127018922194093, 0.9330127018922194093 ) ) 
 REPRESENTATION_ITEM ( '' )  );
#4573=VERTEX_POINT ( 'NONE', #11211 ) ;
#4576=CARTESIAN_POINT ( 'NONE',  ( 2.229367062499998831, -73.89583333196773651, -3.861377020970580887 ) ) ;
#4578=PRESENTATION_STYLE_ASSIGNMENT (( #54434 ) ) ;
#4584=CARTESIAN_POINT ( 'NONE',  ( -2.229367062499996610, -0.3958333319677397322, 3.861377020970582219 ) ) ;
#4586=VECTOR ( 'NONE', #28624, 1000.000000000000000 ) ;
#4588=CARTESIAN_POINT ( 'NONE',  ( 5.000000000000000000, -69.37499999726880162, -6.123233995736766282E-16 ) ) ;
#4591=CARTESIAN_POINT ( 'NONE',  ( 1.975475456537005874E-15, 6.375000002731185944, 5.000000000000000000 ) ) ;
#4593=VERTEX_POINT ( 'NONE', #54961 ) ;
#4594=CARTESIAN_POINT ( 'NONE',  ( 4.458734124999999437, -73.81249999863440792, -5.460374474430324690E-16 ) ) ;
#4596=CARTESIAN_POINT ( 'NONE',  ( 9.457646018065525792E-16, 1.937500001365593416, 5.148502694627439702 ) ) ;
#4598=CARTESIAN_POINT ( 'NONE',  ( 9.457646018065525792E-16, -67.31249999863440792, 5.148502694627439702 ) ) ;
#4599=CARTESIAN_POINT ( 'NONE',  ( -3.535250795749689387E-16, -27.12499999726881583, -5.773502691896257311 ) ) ;
#4601=FACE_OUTER_BOUND ( 'NONE', #46987, .T. ) ;
#4604=CARTESIAN_POINT ( 'NONE',  ( 4.458734124999998549, -45.72916666530106511, -2.574251347313721627 ) ) ;
#4605=CARTESIAN_POINT ( 'NONE',  ( 4.458734124999999437, -28.06249999863440081, -5.460374474430324690E-16 ) ) ;
#4608=CARTESIAN_POINT ( 'NONE',  ( 1.060575238724906964E-15, 28.24999999999999645, 5.773502691896257311 ) ) ;
#4610=CARTESIAN_POINT ( 'NONE',  ( -6.972266317189433020E-16, -54.12499999726880162, -5.000000000000000000 ) ) ;
#4611=CARTESIAN_POINT ( 'NONE',  ( -3.152548672688508926E-16, -35.56249999863440792, -5.148502694627439702 ) ) ;
#4612=CARTESIAN_POINT ( 'NONE',  ( -2.500000000000000444, -67.04166666393547303, -4.330127018922193649 ) ) ;
#4615=CARTESIAN_POINT ( 'NONE',  ( -3.152548672688508926E-16, -76.81249999863440792, -5.148502694627439702 ) ) ;
#4618=CARTESIAN_POINT ( 'NONE',  ( -4.999999999999998224, -27.79166666393548013, 2.886751345948131764 ) ) ;
#4619=CARTESIAN_POINT ( 'NONE',  ( 0.000000000000000000, -120.0000000000000000, 0.000000000000000000 ) ) ;
#4620=CARTESIAN_POINT ( 'NONE',  ( -5.000000000000000000, -21.08333333333333570, -2.886751345948128211 ) ) ;
#4624=CARTESIAN_POINT ( 'NONE',  ( 1.975475456537005874E-15, -58.75000000000000000, 5.000000000000000000 ) ) ;
#4626=CARTESIAN_POINT ( 'NONE',  ( 1.060575238724906964E-15, 26.37500000273118417, 5.773502691896257311 ) ) ;
#4634=LINE ( 'NONE', #24258, #26583 ) ;
#4635=CARTESIAN_POINT ( 'NONE',  ( 5.000000000000000000, -89.29166666393547303, -2.886751345948130876 ) ) ;
#4637=CARTESIAN_POINT ( 'NONE',  ( 9.457646018065525792E-16, -23.06249999863440792, 5.148502694627439702 ) ) ;
#4638=CARTESIAN_POINT ( 'NONE',  ( 1.339745962155615144, -97.58034179853028434, 4.999999999999999112 ) ) ;
#4644=ORIENTED_EDGE ( 'NONE', *, *, #1370, .F. ) ;
#4647=EDGE_LOOP ( 'NONE', ( #40631, #25304, #24848, #59086 ) ) ;
#4649=CARTESIAN_POINT ( 'NONE',  ( -5.000000000000000000, -28.99999999999999645, 0.000000000000000000 ) ) ;
#4651=ORIENTED_EDGE ( 'NONE', *, *, #26359, .F. ) ;
#4654=CARTESIAN_POINT ( 'NONE',  ( 1.975475456537005874E-15, -86.62499999726880162, 5.000000000000000000 ) ) ;
#4657=ADVANCED_FACE ( 'NONE', ( #61388 ), #27902, .T. ) ;
#4659=CARTESIAN_POINT ( 'NONE',  ( -4.458734124999998549, 19.77083333469892779, 2.574251347313722516 ) ) ;
#4661=ORIENTED_EDGE ( 'NONE', *, *, #53617, .T. ) ;
#4664=CARTESIAN_POINT ( 'NONE',  ( -6.972266317189433020E-16, -79.12499999726881583, -5.000000000000000000 ) ) ;
#4666=CARTESIAN_POINT ( 'NONE',  ( 2.229367062500001939, -57.97916666530107932, 3.861377020970579999 ) ) ;
#4668=CARTESIAN_POINT ( 'NONE',  ( -4.458734124999999437, 16.68750000136559564, 0.000000000000000000 ) ) ;
#4671=CARTESIAN_POINT ( 'NONE',  ( -3.152548672688508926E-16, -49.81249999863440081, -5.148502694627439702 ) ) ;
#4673=CARTESIAN_POINT ( 'NONE',  ( -5.000000000000000000, -9.958333330602144429, -2.886751345948128211 ) ) ;
#4677=CARTESIAN_POINT ( 'NONE',  ( -4.458734124999997661, -108.2291666653010651, 2.574251347313722516 ) ) ;
#4678=CARTESIAN_POINT ( 'NONE',  ( 4.458734124999998549, -9.979166665301068662, -2.574251347313721627 ) ) ;
#4681=CARTESIAN_POINT ( 'NONE',  ( 4.458734125000001214, -100.8958333319677365, 2.574251347313718519 ) ) ;
#4683=CARTESIAN_POINT ( 'NONE',  ( -4.458734124999999437, -95.56249999863440792, 0.000000000000000000 ) ) ;
#4685=CARTESIAN_POINT ( 'NONE',  ( -3.535250795749689387E-16, -50.12499999726881583, -5.773502691896257311 ) ) ;
#4686=CARTESIAN_POINT ( 'NONE',  ( -1.339745962155610925, -36.66965819600732601, 5.000000000000000000 ) ) ;
#4689=CARTESIAN_POINT ( 'NONE',  ( -2.229367062500000163, -20.47916666530107221, -3.861377020970580443 ) ) ;
#4690=CARTESIAN_POINT ( 'NONE',  ( -2.229367062500000163, 11.27083333469892601, -3.861377020970580443 ) ) ;
#4691=CARTESIAN_POINT ( 'NONE',  ( 2.229367062500001939, -61.22916666530106511, 3.861377020970579999 ) ) ;
#4696=CARTESIAN_POINT ( 'NONE',  ( -5.000000000000000000, -3.999999999999996447, 0.000000000000000000 ) ) ;
#4697=EDGE_LOOP ( 'NONE', ( #61118, #37356, #57344, #313 ) ) ;
#4700=CARTESIAN_POINT ( 'NONE',  ( -4.999999999999998224, -8.916666666666662522, 2.886751345948131764 ) ) ;
#4701=CARTESIAN_POINT ( 'NONE',  ( -6.972266317189433020E-16, -67.12499999726881583, -5.000000000000000000 ) ) ;
#4702=CARTESIAN_POINT ( 'NONE',  ( 4.458734124999999437, -82.81249999863440792, -5.460374474430324690E-16 ) ) ;
#4703=CARTESIAN_POINT ( 'NONE',  ( 4.458734125000001214, 20.85416666803226349, 2.574251347313718519 ) ) ;
#4706=EDGE_CURVE ( 'NONE', #54885, #42214, #34018, .T. ) ;
#4707=EDGE_CURVE ( 'NONE', #63145, #49750, #17126, .T. ) ;
#4712=CARTESIAN_POINT ( 'NONE',  ( 2.500000000000002220, -73.66666666666665719, 4.330127018922192761 ) ) ;
#4714=VERTEX_POINT ( 'NONE', #22466 ) ;
#4727=EDGE_LOOP ( 'NONE', ( #46555, #26307, #57460, #4558 ) ) ;
#4729=DIRECTION ( 'NONE',  ( -0.000000000000000000, 1.000000000000000000, -0.000000000000000000 ) ) ;
#4730=CARTESIAN_POINT ( 'NONE',  ( -4.458734124999998549, -57.47916666530108643, 2.574251347313722516 ) ) ;
#4733=ORIENTED_EDGE ( 'NONE', *, *, #14068, .T. ) ;
#4739=CARTESIAN_POINT ( 'NONE',  ( 9.457646018065525792E-16, -103.3124999986344079, 5.148502694627439702 ) ) ;
#4744=CARTESIAN_POINT ( 'NONE',  ( 4.458734124999999437, -38.81249999863440081, -5.460374474430324690E-16 ) ) ;
#4747=CARTESIAN_POINT ( 'NONE',  ( -4.458734124999998549, -13.22916666530107221, 2.574251347313722516 ) ) ;
#4748=CARTESIAN_POINT ( 'NONE',  ( -3.152548672688508926E-16, -100.8124999986343937, -5.148502694627439702 ) ) ;
#4749=ORIENTED_EDGE ( 'NONE', *, *, #23243, .F. ) ;
#4751=CARTESIAN_POINT ( 'NONE',  ( 2.229367062499998831, -33.89583333196772941, -3.861377020970580887 ) ) ;
#4752=DIRECTION ( 'NONE',  ( 1.000000000000000000, 0.000000000000000000, -3.614007241618347908E-17 ) ) ;
#4757=CARTESIAN_POINT ( 'NONE',  ( -4.458734124999999437, 2.354166668032262599, -2.574251347313719407 ) ) ;
#4760=CARTESIAN_POINT ( 'NONE',  ( -2.499999999999996447, 2.166666666666667407, 4.330127018922195425 ) ) ;
#4761=CARTESIAN_POINT ( 'NONE',  ( -1.339745962155610925, 16.33034180399266333, 5.000000000000000000 ) ) ;
#4762=CARTESIAN_POINT ( 'NONE',  ( -3.535250795749689387E-16, -94.25000000000000000, -5.773502691896257311 ) ) ;
#4763=CARTESIAN_POINT ( 'NONE',  ( -3.152548672688508926E-16, -32.56249999863440792, -5.148502694627439702 ) ) ;
#4765=CARTESIAN_POINT ( 'NONE',  ( 4.458734125000001214, -78.14583333196775072, 2.574251347313718519 ) ) ;
#4766=VECTOR ( 'NONE', #3551, 1000.000000000000000 ) ;
#4769=VECTOR ( 'NONE', #10133, 1000.000000000000000 ) ;
#4771=CARTESIAN_POINT ( 'NONE',  ( 4.458734124999999437, 0.1875000013655953035, -5.460374474430324690E-16 ) ) ;
#4772=CARTESIAN_POINT ( 'NONE',  ( 4.458734125000001214, 24.85416666803225993, 2.574251347313718519 ) ) ;
#4773=CARTESIAN_POINT ( 'NONE',  ( 2.229367062500001939, -42.22916666530107932, 3.861377020970579999 ) ) ;
#4778=CARTESIAN_POINT ( 'NONE',  ( 4.458734124999998549, -69.72916666530107932, -2.574251347313721627 ) ) ;
#4779=CARTESIAN_POINT ( 'NONE',  ( -2.500000000000000444, -108.0416666639354730, -4.330127018922193649 ) ) ;
#4782=ADVANCED_FACE ( 'NONE', ( #9229 ), #29148, .T. ) ;
#4783=CARTESIAN_POINT ( 'NONE',  ( -6.972266317189433020E-16, -58.12499999726880162, -5.000000000000000000 ) ) ;
#4784=CARTESIAN_POINT ( 'NONE',  ( 2.229367062500001939, -109.2291666653010651, 3.861377020970579999 ) ) ;
#4786=CARTESIAN_POINT ( 'NONE',  ( -5.000000000000000000, -55.08333333333332860, -2.886751345948128211 ) ) ;
#4787=ADVANCED_FACE ( 'NONE', ( #49417 ), #53293, .T. ) ;
#4788=CARTESIAN_POINT ( 'NONE',  ( 6.123233995736766282E-16, -120.0000000000000000, -5.000000000000000000 ) ) ;
#4790=ORIENTED_EDGE ( 'NONE', *, *, #47134, .T. ) ;
#4791=DIRECTION ( 'NONE',  ( 0.000000000000000000, 0.000000000000000000, 1.000000000000000000 ) ) ;
#4792=CARTESIAN_POINT ( 'NONE',  ( -2.499999999999996447, 13.16666666666666607, 4.330127018922195425 ) ) ;
#4795=EDGE_CURVE ( 'NONE', #456, #10433, #18874, .T. ) ;
#4802=CARTESIAN_POINT ( 'NONE',  ( 1.339745962155615144, 5.294658198738519950, 4.999999999999999112 ) ) ;
#4805=VERTEX_POINT ( 'NONE', #8919 ) ;
#4808=EDGE_CURVE ( 'NONE', #33230, #23099, #14292, .T. ) ;
#4810=CARTESIAN_POINT ( 'NONE',  ( -4.458734124999999437, -40.56249999863440081, 0.000000000000000000 ) ) ;
#4813=EDGE_CURVE ( 'NONE', #27768, #11599, #43042, .T. ) ;
#4814=CARTESIAN_POINT ( 'NONE',  ( -5.000000000000000000, -56.95833333060214443, -2.886751345948128211 ) ) ;
#4819=ADVANCED_FACE ( 'NONE', ( #49092 ), #5038, .T. ) ;
#4822=CARTESIAN_POINT ( 'NONE',  ( 4.458734125000001214, -91.14583333196773651, 2.574251347313718519 ) ) ;
#4823=CARTESIAN_POINT ( 'NONE',  ( 1.339745962155612702, -108.2946581987385315, -5.000000000000000000 ) ) ;
#4830=CARTESIAN_POINT ( 'NONE',  ( 4.458734124999999437, 4.187500001365595637, -5.460374474430324690E-16 ) ) ;
#4831=CARTESIAN_POINT ( 'NONE',  ( -1.339745962155610925, -70.66965819600731891, 5.000000000000000000 ) ) ;
#4832=CARTESIAN_POINT ( 'NONE',  ( -2.229367062499996610, -14.39583333196774184, 3.861377020970582219 ) ) ;
#4833=CARTESIAN_POINT ( 'NONE',  ( 1.975475456537005874E-15, -105.6249999972688016, 5.000000000000000000 ) ) ;
#4835=CARTESIAN_POINT ( 'NONE',  ( 1.975475456537005874E-15, -55.62499999726880873, 5.000000000000000000 ) ) ;
#4837=CARTESIAN_POINT ( 'NONE',  ( 4.458734124999999437, 20.93750000136559208, -5.460374474430324690E-16 ) ) ;
#4839=CARTESIAN_POINT ( 'NONE',  ( 4.458734125000000326, -98.89583333196773651, 2.574251347313718519 ) ) ;
#4842=CARTESIAN_POINT ( 'NONE',  ( 2.229367062499998831, -13.64583333196774184, -3.861377020970580887 ) ) ;
#4843=CARTESIAN_POINT ( 'NONE',  ( -5.000000000000000000, -84.87499999726880162, 0.000000000000000000 ) ) ;
#4846=CARTESIAN_POINT ( 'NONE',  ( -5.000000000000000000, -88.08333333333332860, -2.886751345948128211 ) ) ;
#4847=CARTESIAN_POINT ( 'NONE',  ( -3.535250795749689387E-16, -42.12499999726880873, -5.773502691896257311 ) ) ;
#4849=CARTESIAN_POINT ( 'NONE',  ( 2.229367062500001939, 13.02083333469892779, 3.861377020970579999 ) ) ;
#4853=CARTESIAN_POINT ( 'NONE',  ( 4.458734125000001214, -63.89583333196772941, 2.574251347313718519 ) ) ;
#4856=CARTESIAN_POINT ( 'NONE',  ( 1.975475456537005874E-15, -45.74999999999999289, 5.000000000000000000 ) ) ;
#4857=CARTESIAN_POINT ( 'NONE',  ( -5.000000000000000000, 12.00000000000000000, 0.000000000000000000 ) ) ;
#4859=CARTESIAN_POINT ( 'NONE',  ( 2.229367062500001939, -50.97916666530107221, 3.861377020970579999 ) ) ;
#4860=CARTESIAN_POINT ( 'NONE',  ( -5.000000000000000000, -91.87499999726880162, 0.000000000000000000 ) ) ;
#4861=AXIS2_PLACEMENT_3D ( 'NONE', #9735, #23910, #29031 ) ;
#4862=CARTESIAN_POINT ( 'NONE',  ( -3.152548672688508926E-16, -26.56249999863440436, -5.148502694627439702 ) ) ;
#4864=CARTESIAN_POINT ( 'NONE',  ( -1.339745962155610925, -16.79465819873852084, 5.000000000000000000 ) ) ;
#4869=CARTESIAN_POINT ( 'NONE',  ( -2.500000000000000444, -36.16666666666666430, -4.330127018922193649 ) ) ;
#4872=ORIENTED_EDGE ( 'NONE', *, *, #43262, .T. ) ;
#4873=CARTESIAN_POINT ( 'NONE',  ( -4.458734124999999437, -99.31249999863440792, 0.000000000000000000 ) ) ;
#4874=CARTESIAN_POINT ( 'NONE',  ( -4.458734124999999437, 2.354166668032262599, -2.574251347313719407 ) ) ;
#4881=VERTEX_POINT ( 'NONE', #39435 ) ;
#4883=FACE_OUTER_BOUND ( 'NONE', #375, .T. ) ;
#4886=CARTESIAN_POINT ( 'NONE',  ( -1.339745962155610925, -89.66965819600733312, 5.000000000000000000 ) ) ;
#4887=CARTESIAN_POINT ( 'NONE',  ( -4.458734124999999437, -22.64583333196773296, -2.574251347313719407 ) ) ;
#4888=CARTESIAN_POINT ( 'NONE',  ( -1.339745962155618253, 22.33034180399266333, 4.999999999999996447 ) ) ;
#4895=EDGE_CURVE ( 'NONE', #11599, #62971, #59075, .T. ) ;
#4896=ORIENTED_EDGE ( 'NONE', *, *, #62203, .T. ) ;
#4898=EDGE_LOOP ( 'NONE', ( #55155, #25428, #63452, #40701 ) ) ;
#4899=CARTESIAN_POINT ( 'NONE',  ( -4.458734124999999437, -75.64583333196775072, -2.574251347313719407 ) ) ;
#4903=CARTESIAN_POINT ( 'NONE',  ( 5.000000000000000888, 12.41666666666666607, 2.886751345948126879 ) ) ;
#4904=( BOUNDED_CURVE ( )  B_SPLINE_CURVE ( 2, ( #9818, #29428, #20122, #5979, #34919, #39405, #48741, #39724, #25587 ),
 .UNSPECIFIED., .F., .F. ) 
 B_SPLINE_CURVE_WITH_KNOTS ( ( 3, 2, 2, 2, 3 ),
 ( 0.2696428571428571286, 0.2702380952380952217, 0.2714285714285714080, 0.2726190476190475942, 0.2732142857142857428 ),
 .UNSPECIFIED. ) 
 CURVE ( )  GEOMETRIC_REPRESENTATION_ITEM ( )  RATIONAL_B_SPLINE_CURVE ( ( 0.9330127018922194093, 0.9330127018922194093, 1.000000000000000000, 0.8660254037844387076, 1.000000000000000000, 0.8660254037844387076, 1.000000000000000000, 0.9330127018922163007, 0.9330127018922194093 ) ) 
 REPRESENTATION_ITEM ( '' )  );
#4905=VECTOR ( 'NONE', #10783, 1000.000000000000000 ) ;
#4908=CARTESIAN_POINT ( 'NONE',  ( 2.229367062500001939, 3.770833334698926009, 3.861377020970579999 ) ) ;
#4909=ORIENTED_EDGE ( 'NONE', *, *, #60890, .T. ) ;
#4910=FACE_OUTER_BOUND ( 'NONE', #50234, .T. ) ;
#4911=DIRECTION ( 'NONE',  ( 0.000000000000000000, -1.000000000000000000, 0.000000000000000000 ) ) ;
#4917=EDGE_LOOP ( 'NONE', ( #4281, #56889, #33435, #10917 ) ) ;
#4918=CARTESIAN_POINT ( 'NONE',  ( 9.457646018065525792E-16, -77.06249999863440792, 5.148502694627439702 ) ) ;
#4920=CARTESIAN_POINT ( 'NONE',  ( -2.229367062500000163, 1.520833334698927564, -3.861377020970580443 ) ) ;
#4921=CARTESIAN_POINT ( 'NONE',  ( 2.500000000000002220, -87.66666666666667140, 4.330127018922192761 ) ) ;
#4922=DIRECTION ( 'NONE',  ( -0.000000000000000000, 1.000000000000000000, -0.000000000000000000 ) ) ;
#4923=CARTESIAN_POINT ( 'NONE',  ( -3.152548672688508926E-16, -63.81249999863440792, -5.148502694627439702 ) ) ;
#4924=CARTESIAN_POINT ( 'NONE',  ( -2.500000000000000444, -24.04166666393548368, -4.330127018922193649 ) ) ;
#4925=DIRECTION ( 'NONE',  ( 0.000000000000000000, 0.000000000000000000, 1.000000000000000000 ) ) ;
#4926=CARTESIAN_POINT ( 'NONE',  ( -6.972266317189433020E-16, -0.2500000000000001665, -5.000000000000000000 ) ) ;
#4928=CARTESIAN_POINT ( 'NONE',  ( 5.000000000000000000, -3.374999997268816276, -6.123233995736766282E-16 ) ) ;
#4929=CARTESIAN_POINT ( 'NONE',  ( 2.229367062500001939, -47.97916666530106511, 3.861377020970579999 ) ) ;
#4930=CARTESIAN_POINT ( 'NONE',  ( 4.458734124999999437, -31.06249999863440436, -5.460374474430324690E-16 ) ) ;
#4932=CARTESIAN_POINT ( 'NONE',  ( 1.975475456537005874E-15, -96.75000000000000000, 5.000000000000000000 ) ) ;
#4933=CARTESIAN_POINT ( 'NONE',  ( 1.060575238724906964E-15, 26.25000000000000000, 5.773502691896257311 ) ) ;
#4935=CARTESIAN_POINT ( 'NONE',  ( 9.457646018065525792E-16, -40.06249999863439371, 5.148502694627439702 ) ) ;
#4936=CARTESIAN_POINT ( 'NONE',  ( 5.000000000000000888, -72.45833333060213022, 2.886751345948126879 ) ) ;
#4939=CARTESIAN_POINT ( 'NONE',  ( 9.457646018065525792E-16, -73.31249999863439371, 5.148502694627439702 ) ) ;
#4944=CARTESIAN_POINT ( 'NONE',  ( -3.535250795749689387E-16, -22.24999999999999645, -5.773502691896257311 ) ) ;
#4946=ORIENTED_EDGE ( 'NONE', *, *, #24234, .F. ) ;
#4950=CARTESIAN_POINT ( 'NONE',  ( -5.000000000000000000, 21.12500000273118417, 0.000000000000000000 ) ) ;
#4954=AXIS2_PLACEMENT_3D ( 'NONE', #40234, #59871, #15793 ) ;
#4959=LINE ( 'NONE', #19748, #50802 ) ;
#4962=CARTESIAN_POINT ( 'NONE',  ( 2.229367062499998831, -23.64583333196773651, -3.861377020970580887 ) ) ;
#4963=CARTESIAN_POINT ( 'NONE',  ( -2.499999999999996447, -71.70833333060214443, 4.330127018922195425 ) ) ;
#4970=CARTESIAN_POINT ( 'NONE',  ( -6.972266317189433020E-16, -87.25000000000001421, -5.000000000000000000 ) ) ;
#4971=CARTESIAN_POINT ( 'NONE',  ( -1.339745962155610925, -67.66965819600733312, 5.000000000000000000 ) ) ;
#4974=CARTESIAN_POINT ( 'NONE',  ( -5.000000000000000000, 11.00000000000000000, 0.000000000000000000 ) ) ;
#4978=VERTEX_POINT ( 'NONE', #31380 ) ;
#4980=CARTESIAN_POINT ( 'NONE',  ( -2.229367062500000163, 20.52083333469892779, -3.861377020970580443 ) ) ;
#4985=DIRECTION ( 'NONE',  ( 0.000000000000000000, 0.000000000000000000, 1.000000000000000000 ) ) ;
#4986=CARTESIAN_POINT ( 'NONE',  ( 2.500000000000002220, -100.6666666666666572, 4.330127018922192761 ) ) ;
#4988=CARTESIAN_POINT ( 'NONE',  ( -6.972266317189433020E-16, -70.25000000000000000, -5.000000000000000000 ) ) ;
#4989=CARTESIAN_POINT ( 'NONE',  ( 4.458734125000000326, -58.89583333196773651, 2.574251347313718519 ) ) ;
#4991=CARTESIAN_POINT ( 'NONE',  ( -4.458734124999998549, 16.77083333469892779, 2.574251347313722516 ) ) ;
#4995=CARTESIAN_POINT ( 'NONE',  ( -1.339745962155625802, 18.20534180126147206, 4.999999999999991118 ) ) ;
#4996=CARTESIAN_POINT ( 'NONE',  ( -2.229367062500000163, -51.72916666530107221, -3.861377020970580443 ) ) ;
#4997=CARTESIAN_POINT ( 'NONE',  ( -3.535250795749689387E-16, -8.124999997268814056, -5.773502691896257311 ) ) ;
#4998=CARTESIAN_POINT ( 'NONE',  ( -2.480964764533239819E-13, -72.75000000000000000, 5.000000000000000000 ) ) ;
#4999=CARTESIAN_POINT ( 'NONE',  ( 0.000000000000000000, 30.00000000000000000, 0.000000000000000000 ) ) ;
#5000=CARTESIAN_POINT ( 'NONE',  ( -5.000000000000000000, -74.08333333333330017, -2.886751345948128211 ) ) ;
#5001=CARTESIAN_POINT ( 'NONE',  ( -2.229367062499996610, -106.1458333319677365, 3.861377020970582219 ) ) ;
#5002=CARTESIAN_POINT ( 'NONE',  ( 9.457646018065525792E-16, -11.31249999863440792, 5.148502694627439702 ) ) ;
#5004=CARTESIAN_POINT ( 'NONE',  ( 2.499999999999998668, 23.66666666666666430, -4.330127018922193649 ) ) ;
#5005=CARTESIAN_POINT ( 'NONE',  ( -4.458734124999999437, -96.39583333196772230, -2.574251347313719407 ) ) ;
#5007=CARTESIAN_POINT ( 'NONE',  ( 2.229367062499998831, -97.89583333196773651, -3.861377020970580887 ) ) ;
#5009=CARTESIAN_POINT ( 'NONE',  ( -5.000000000000000000, -55.95833333060215153, -2.886751345948128211 ) ) ;
#5012=EDGE_CURVE ( 'NONE', #58623, #8918, #16755, .T. ) ;
#5014=CARTESIAN_POINT ( 'NONE',  ( -2.229367062500000163, -17.47916666530106866, -3.861377020970580443 ) ) ;
#5015=CARTESIAN_POINT ( 'NONE',  ( -2.229367062500000163, 7.270833334698929562, -3.861377020970580443 ) ) ;
#5016=CARTESIAN_POINT ( 'NONE',  ( 9.457646018065525792E-16, -59.31249999863440081, 5.148502694627439702 ) ) ;
#5017=DIRECTION ( 'NONE',  ( 0.000000000000000000, 0.000000000000000000, 1.000000000000000000 ) ) ;
#5019=CARTESIAN_POINT ( 'NONE',  ( -6.972266317189433020E-16, -8.124999997268814056, -5.000000000000000000 ) ) ;
#5021=CARTESIAN_POINT ( 'NONE',  ( -5.000000000000000000, -4.083333333333334814, -2.886751345948128211 ) ) ;
#5027=CARTESIAN_POINT ( 'NONE',  ( -4.458734124999998549, -83.22916666530106511, 2.574251347313722516 ) ) ;
#5028=CARTESIAN_POINT ( 'NONE',  ( -3.152548672688508926E-16, 21.18750000136559208, -5.148502694627439702 ) ) ;
#5029=( BOUNDED_CURVE ( )  B_SPLINE_CURVE ( 2, ( #25087, #49845, #10606, #24774, #20599, #45028, #995, #40203, #59839 ),
 .UNSPECIFIED., .F., .F. ) 
 B_SPLINE_CURVE_WITH_KNOTS ( ( 3, 2, 2, 2, 3 ),
 ( 0.9339285714285714413, 0.9345238095238095344, 0.9357142857142857206, 0.9369047619047619069, 0.9375000000000000000 ),
 .UNSPECIFIED. ) 
 CURVE ( )  GEOMETRIC_REPRESENTATION_ITEM ( )  RATIONAL_B_SPLINE_CURVE ( ( 0.9330127018922194093, 0.9330127018922194093, 1.000000000000000000, 0.8660254037844387076, 1.000000000000000000, 0.8660254037844387076, 1.000000000000000000, 0.9330127018922194093, 0.9330127018922194093 ) ) 
 REPRESENTATION_ITEM ( '' )  );
#5035=CARTESIAN_POINT ( 'NONE',  ( 5.000000000000000888, -75.58333333333334281, 2.886751345948126879 ) ) ;
#5038=CYLINDRICAL_SURFACE ( 'NONE', #33560, 5.000000000000000000 ) ;
#5039=PRODUCT ( 'spindle', 'spindle', '', ( #1217 ) ) ;
#5050=ORIENTED_EDGE ( 'NONE', *, *, #43708, .F. ) ;
#5053=CARTESIAN_POINT ( 'NONE',  ( -4.458734124999999437, -55.64583333196773651, -2.574251347313719407 ) ) ;
#5061=CARTESIAN_POINT ( 'NONE',  ( -3.152548672688508926E-16, -103.8124999986344221, -5.148502694627439702 ) ) ;
#5066=CARTESIAN_POINT ( 'NONE',  ( 9.457646018065525792E-16, -41.06249999863440081, 5.148502694627439702 ) ) ;
#5069=DIRECTION ( 'NONE',  ( -0.000000000000000000, 1.000000000000000000, -0.000000000000000000 ) ) ;
#5070=EDGE_CURVE ( 'NONE', #28793, #57369, #3980, .T. ) ;
#5071=CARTESIAN_POINT ( 'NONE',  ( 4.458734125000001214, -10.89583333196773651, 2.574251347313718519 ) ) ;
#5072=CARTESIAN_POINT ( 'NONE',  ( -2.229367062500000163, -102.7291666653010651, -3.861377020970580443 ) ) ;
#5075=CARTESIAN_POINT ( 'NONE',  ( 2.229367062500001939, -33.22916666530106511, 3.861377020970579999 ) ) ;
#5076=CARTESIAN_POINT ( 'NONE',  ( -5.000000000000000000, 5.041666669397853795, -2.886751345948128211 ) ) ;
#5077=CARTESIAN_POINT ( 'NONE',  ( 1.975475456537005874E-15, -19.75000000000000000, 5.000000000000000000 ) ) ;
#5079=( BOUNDED_CURVE ( )  B_SPLINE_CURVE ( 2, ( #35669, #21831, #6716, #12168, #50775, #7360, #30837, #26969, #1588 ),
 .UNSPECIFIED., .F., .F. ) 
 B_SPLINE_CURVE_WITH_KNOTS ( ( 3, 2, 2, 2, 3 ),
 ( 0.9696428571428571397, 0.9702380952380952328, 0.9714285714285714191, 0.9726190476190476053, 0.9732142857142856984 ),
 .UNSPECIFIED. ) 
 CURVE ( )  GEOMETRIC_REPRESENTATION_ITEM ( )  RATIONAL_B_SPLINE_CURVE ( ( 0.9330127018922194093, 0.9330127018922194093, 1.000000000000000000, 0.8660254037844387076, 1.000000000000000000, 0.8660254037844387076, 1.000000000000000000, 0.9330127018922194093, 0.9330127018922194093 ) ) 
 REPRESENTATION_ITEM ( '' )  );
#5084=CARTESIAN_POINT ( 'NONE',  ( 2.229367062499998831, 4.104166668032260823, -3.861377020970580887 ) ) ;
#5088=CARTESIAN_POINT ( 'NONE',  ( 1.060575238724906964E-15, -93.75000000000000000, 5.773502691896257311 ) ) ;
#5089=CARTESIAN_POINT ( 'NONE',  ( 2.229367062500001939, -29.97916666530107221, 3.861377020970579999 ) ) ;
#5091=CARTESIAN_POINT ( 'NONE',  ( -2.499999999999996447, -35.83333333333332860, 4.330127018922195425 ) ) ;
#5092=CARTESIAN_POINT ( 'NONE',  ( -2.229367062500000163, -82.72916666530106511, -3.861377020970580443 ) ) ;
#5095=LINE ( 'NONE', #62702, #1725 ) ;
#5097=CARTESIAN_POINT ( 'NONE',  ( -4.458734124999997661, -3.229166665301069550, 2.574251347313722516 ) ) ;
#5098=CARTESIAN_POINT ( 'NONE',  ( 4.458734124999998549, 24.02083333469892423, -2.574251347313721627 ) ) ;
#5099=EDGE_CURVE ( 'NONE', #22073, #56652, #45864, .T. ) ;
#5100=CARTESIAN_POINT ( 'NONE',  ( -3.152548672688508926E-16, -41.81249999863440081, -5.148502694627439702 ) ) ;
#5101=CARTESIAN_POINT ( 'NONE',  ( -2.500000000000000444, -46.04166666393547303, -4.330127018922193649 ) ) ;
#5103=ORIENTED_EDGE ( 'NONE', *, *, #28849, .F. ) ;
#5105=CARTESIAN_POINT ( 'NONE',  ( -3.152548672688508926E-16, -71.56249999863440792, -5.148502694627439702 ) ) ;
#5106=CARTESIAN_POINT ( 'NONE',  ( 5.000000000000000888, -105.4583333306021444, 2.886751345948126879 ) ) ;
#5108=CARTESIAN_POINT ( 'NONE',  ( 7.204675194429079505E-15, 26.74999999999999645, -5.000000000000000000 ) ) ;
#5109=CARTESIAN_POINT ( 'NONE',  ( 0.000000000000000000, -120.0000000000000000, 5.000000000000000000 ) ) ;
#5111=CARTESIAN_POINT ( 'NONE',  ( -2.499999999999996447, -61.83333333333333570, 4.330127018922195425 ) ) ;
#5112=CARTESIAN_POINT ( 'NONE',  ( -5.000000000000000000, -66.00000000000000000, 0.000000000000000000 ) ) ;
#5114=ORIENTED_EDGE ( 'NONE', *, *, #48302, .F. ) ;
#5115=CARTESIAN_POINT ( 'NONE',  ( 1.975475456537005874E-15, -62.74999999999998579, 5.000000000000000000 ) ) ;
#5124=DIRECTION ( 'NONE',  ( -0.000000000000000000, 1.000000000000000000, -0.000000000000000000 ) ) ;
#5127=ORIENTED_EDGE ( 'NONE', *, *, #40874, .T. ) ;
#5131=CARTESIAN_POINT ( 'NONE',  ( -4.458734124999999437, -43.64583333196774362, -2.574251347313719407 ) ) ;
#5132=CARTESIAN_POINT ( 'NONE',  ( -2.500000000000000444, -16.04166666393548368, -4.330127018922193649 ) ) ;
#5133=( BOUNDED_CURVE ( )  B_SPLINE_CURVE ( 2, ( #15915, #49367, #54520, #1146, #35536, #35859, #55485, #55164, #49686 ),
 .UNSPECIFIED., .F., .F. ) 
 B_SPLINE_CURVE_WITH_KNOTS ( ( 3, 2, 2, 2, 3 ),
 ( 0.5303571428571428603, 0.5309523809523809534, 0.5321428571428571397, 0.5333333333333333259, 0.5339285714285714191 ),
 .UNSPECIFIED. ) 
 CURVE ( )  GEOMETRIC_REPRESENTATION_ITEM ( )  RATIONAL_B_SPLINE_CURVE ( ( 0.9330127018922194093, 0.9330127018922194093, 1.000000000000000000, 0.8660254037844387076, 1.000000000000000000, 0.8660254037844387076, 1.000000000000000000, 0.9330127018922194093, 0.9330127018922194093 ) ) 
 REPRESENTATION_ITEM ( '' )  );
#5135=CARTESIAN_POINT ( 'NONE',  ( -2.500000000000000444, -57.04166666393548013, -4.330127018922193649 ) ) ;
#5142=CARTESIAN_POINT ( 'NONE',  ( 4.458734125000001214, -87.14583333196772230, 2.574251347313718519 ) ) ;
#5145=CARTESIAN_POINT ( 'NONE',  ( -1.339745962155613812, 13.91965820146970678, -5.000000000000000000 ) ) ;
#5147=VERTEX_POINT ( 'NONE', #1196 ) ;
#5148=CARTESIAN_POINT ( 'NONE',  ( 2.229367062499998831, 3.354166668032259935, -3.861377020970580887 ) ) ;
#5152=CARTESIAN_POINT ( 'NONE',  ( -2.229367062500000163, -18.72916666530106866, -3.861377020970580443 ) ) ;
#5153=EDGE_CURVE ( 'NONE', #63596, #53365, #15649, .T. ) ;
#5156=CARTESIAN_POINT ( 'NONE',  ( -6.972266317189433020E-16, -49.24999999999999289, -5.000000000000000000 ) ) ;
#5158=CARTESIAN_POINT ( 'NONE',  ( -4.458734124999999437, 23.35416666803226349, -2.574251347313719407 ) ) ;
#5159=ORIENTED_EDGE ( 'NONE', *, *, #57455, .F. ) ;
#5160=CARTESIAN_POINT ( 'NONE',  ( 4.458734124999999437, -98.81249999863440792, -5.460374474430324690E-16 ) ) ;
#5163=CARTESIAN_POINT ( 'NONE',  ( -4.458734124999999437, -13.31249999863440259, 0.000000000000000000 ) ) ;
#5164=CARTESIAN_POINT ( 'NONE',  ( -6.972266317189433020E-16, -110.1249999972688158, -5.000000000000000000 ) ) ;
#5168=CARTESIAN_POINT ( 'NONE',  ( -4.999999999999999112, -42.79166666393548013, 2.886751345948131764 ) ) ;
#5170=CARTESIAN_POINT ( 'NONE',  ( -4.458734124999997661, 11.77083333469892601, 2.574251347313722516 ) ) ;
#5175=CARTESIAN_POINT ( 'NONE',  ( -4.458734124999999437, -64.39583333196772230, -2.574251347313719407 ) ) ;
#5176=EDGE_LOOP ( 'NONE', ( #57452, #32675, #25731, #15825 ) ) ;
#5179=CARTESIAN_POINT ( 'NONE',  ( 2.500000000000002220, 6.333333333333333037, 4.330127018922192761 ) ) ;
#5181=FACE_OUTER_BOUND ( 'NONE', #38865, .T. ) ;
#5183=AXIS2_PLACEMENT_3D ( 'NONE', #63256, #44573, #39422 ) ;
#5184=CARTESIAN_POINT ( 'NONE',  ( -4.458734124999999437, -52.31249999863440792, 0.000000000000000000 ) ) ;
#5185=CARTESIAN_POINT ( 'NONE',  ( 5.000000000000000000, -91.29166666393547303, -2.886751345948129988 ) ) ;
#5186=CARTESIAN_POINT ( 'NONE',  ( -3.152548672688508926E-16, -33.56249999863440792, -5.148502694627439702 ) ) ;
#5188=CARTESIAN_POINT ( 'NONE',  ( 5.000000000000000000, 25.62500000273118417, -6.123233995736766282E-16 ) ) ;
#5191=CARTESIAN_POINT ( 'NONE',  ( -3.535250795749689387E-16, -43.24999999999999289, -5.773502691896257311 ) ) ;
#5193=ORIENTED_EDGE ( 'NONE', *, *, #9420, .F. ) ;
#5194=CARTESIAN_POINT ( 'NONE',  ( -4.458734124999998549, -100.2291666653010509, 2.574251347313722516 ) ) ;
#5195=CARTESIAN_POINT ( 'NONE',  ( -2.229367062499996610, 5.604166668032261711, 3.861377020970582219 ) ) ;
#5202=ORIENTED_EDGE ( 'NONE', *, *, #13548, .T. ) ;
#5204=DIRECTION ( 'NONE',  ( -0.000000000000000000, 1.000000000000000000, -0.000000000000000000 ) ) ;
#5205=VERTEX_POINT ( 'NONE', #36860 ) ;
#5207=CYLINDRICAL_SURFACE ( 'NONE', #34656, 5.000000000000000000 ) ;
#5208=CARTESIAN_POINT ( 'NONE',  ( -2.229367062499996610, -24.39583333196773651, 3.861377020970582219 ) ) ;
#5209=CARTESIAN_POINT ( 'NONE',  ( -6.972266317189433020E-16, -81.24999999999998579, -5.000000000000000000 ) ) ;
#5214=( BOUNDED_CURVE ( )  B_SPLINE_CURVE ( 2, ( #32754, #57215, #12814, #57529, #47540, #56894, #42080, #13451, #23104 ),
 .UNSPECIFIED., .F., .F. ) 
 B_SPLINE_CURVE_WITH_KNOTS ( ( 3, 2, 2, 2, 3 ),
 ( 0.5982142857142856984, 0.5988095238095237915, 0.5999999999999999778, 0.6011904761904761640, 0.6017857142857142572 ),
 .UNSPECIFIED. ) 
 CURVE ( )  GEOMETRIC_REPRESENTATION_ITEM ( )  RATIONAL_B_SPLINE_CURVE ( ( 0.9330127018922194093, 0.9330127018922194093, 1.000000000000000000, 0.8660254037844387076, 1.000000000000000000, 0.8660254037844387076, 1.000000000000000000, 0.9330127018922194093, 0.9330127018922194093 ) ) 
 REPRESENTATION_ITEM ( '' )  );
#5218=DIRECTION ( 'NONE',  ( -0.000000000000000000, 1.000000000000000000, -0.000000000000000000 ) ) ;
#5220=CARTESIAN_POINT ( 'NONE',  ( -2.229367062499996610, -72.39583333196773651, 3.861377020970582219 ) ) ;
#5223=EDGE_LOOP ( 'NONE', ( #33673, #19911, #54933, #8223 ) ) ;
#5227=CARTESIAN_POINT ( 'NONE',  ( 4.458734124999998549, -2.979166665301069994, -2.574251347313721627 ) ) ;
#5229=( BOUNDED_CURVE ( )  B_SPLINE_CURVE ( 2, ( #36501, #6602, #46476, #36192, #61279, #31993, #7251, #55813, #37150 ),
 .UNSPECIFIED., .F., .F. ) 
 B_SPLINE_CURVE_WITH_KNOTS ( ( 3, 2, 2, 2, 3 ),
 ( 0.6482142857142857428, 0.6488095238095238360, 0.6500000000000000222, 0.6511904761904762085, 0.6517857142857143016 ),
 .UNSPECIFIED. ) 
 CURVE ( )  GEOMETRIC_REPRESENTATION_ITEM ( )  RATIONAL_B_SPLINE_CURVE ( ( 0.9330127018922194093, 0.9330127018922194093, 1.000000000000000000, 0.8660254037844387076, 1.000000000000000000, 0.8660254037844387076, 1.000000000000000000, 0.9330127018922194093, 0.9330127018922194093 ) ) 
 REPRESENTATION_ITEM ( '' )  );
#5230=ADVANCED_FACE ( 'NONE', ( #37181 ), #37808, .T. ) ;
#5237=VERTEX_POINT ( 'NONE', #17235 ) ;
#5238=CARTESIAN_POINT ( 'NONE',  ( -2.229367062499996610, -83.14583333196773651, 3.861377020970582219 ) ) ;
#5240=CARTESIAN_POINT ( 'NONE',  ( 4.458734125000001214, 4.104166668032260823, 2.574251347313718519 ) ) ;
#5241=CARTESIAN_POINT ( 'NONE',  ( 2.500000000000002220, -84.66666666666667140, 4.330127018922192761 ) ) ;
#5242=CARTESIAN_POINT ( 'NONE',  ( 4.458734124999999437, -67.06249999863440792, -5.460374474430324690E-16 ) ) ;
#5243=CARTESIAN_POINT ( 'NONE',  ( -2.499999999999996447, -24.70833333060214443, 4.330127018922195425 ) ) ;
#5245=CARTESIAN_POINT ( 'NONE',  ( 4.458734125000000326, 28.10416666803225993, 2.574251347313718519 ) ) ;
#5246=CARTESIAN_POINT ( 'NONE',  ( -1.339745962155613812, -65.08034179853029855, -5.000000000000000000 ) ) ;
#5247=CARTESIAN_POINT ( 'NONE',  ( 6.158835246850667461E-14, -3.124999997268814944, -4.999999999999999112 ) ) ;
#5248=EDGE_CURVE ( 'NONE', #27379, #22002, #36533, .T. ) ;
#5249=CARTESIAN_POINT ( 'NONE',  ( -4.458734124999999437, -47.39583333196774362, -2.574251347313719407 ) ) ;
#5251=CARTESIAN_POINT ( 'NONE',  ( 4.458734125000000326, -34.14583333196772941, 2.574251347313718519 ) ) ;
#5254=CARTESIAN_POINT ( 'NONE',  ( 1.060575238724906964E-15, 21.24999999999999645, 5.773502691896257311 ) ) ;
#5255=EDGE_CURVE ( 'NONE', #61639, #47219, #12249, .T. ) ;
#5257=CARTESIAN_POINT ( 'NONE',  ( 5.000000000000000000, -54.29166666393549434, -2.886751345948130876 ) ) ;
#5258=CARTESIAN_POINT ( 'NONE',  ( 4.458734124999999437, -34.81249999863440792, -5.460374474430324690E-16 ) ) ;
#5259=CARTESIAN_POINT ( 'NONE',  ( -4.999999999999999112, -72.79166666393547303, 2.886751345948131764 ) ) ;
#5264=CARTESIAN_POINT ( 'NONE',  ( 4.458734124999998549, -78.97916666530106511, -2.574251347313721627 ) ) ;
#5268=CARTESIAN_POINT ( 'NONE',  ( 5.000000000000000000, -23.50000000000000000, -6.123233995736766282E-16 ) ) ;
#5274=CARTESIAN_POINT ( 'NONE',  ( -3.535250795749689387E-16, 19.87500000273118417, -5.773502691896257311 ) ) ;
#5275=CARTESIAN_POINT ( 'NONE',  ( -6.972266317189433020E-16, -48.12499999726880873, -5.000000000000000000 ) ) ;
#5277=VECTOR ( 'NONE', #27237, 1000.000000000000000 ) ;
#5280=CARTESIAN_POINT ( 'NONE',  ( -1.339745962155613812, 3.794658198738521282, -5.000000000000000000 ) ) ;
#5284=VECTOR ( 'NONE', #17882, 1000.000000000000000 ) ;
#5287=CARTESIAN_POINT ( 'NONE',  ( 2.229367062500001939, -21.97916666530107221, 3.861377020970579999 ) ) ;
#5295=ORIENTED_EDGE ( 'NONE', *, *, #1204, .T. ) ;
#5297=CARTESIAN_POINT ( 'NONE',  ( 3.044556291839386294E-14, 11.87500000273118417, -5.000000000000000000 ) ) ;
#5302=CARTESIAN_POINT ( 'NONE',  ( 0.000000000000000000, -120.0000000000000000, 0.000000000000000000 ) ) ;
#5306=CARTESIAN_POINT ( 'NONE',  ( 2.229367062499998831, 12.35416666803226171, -3.861377020970580887 ) ) ;
#5311=FACE_OUTER_BOUND ( 'NONE', #50057, .T. ) ;
#5313=( BOUNDED_CURVE ( )  B_SPLINE_CURVE ( 2, ( #59547, #24249, #33591, #20946, #15482, #19096, #14281, #9144, #13659 ),
 .UNSPECIFIED., .F., .F. ) 
 B_SPLINE_CURVE_WITH_KNOTS ( ( 3, 2, 2, 2, 3 ),
 ( 0.5625000000000000000, 0.5630952380952380931, 0.5642857142857142794, 0.5654761904761904656, 0.5660714285714285587 ),
 .UNSPECIFIED. ) 
 CURVE ( )  GEOMETRIC_REPRESENTATION_ITEM ( )  RATIONAL_B_SPLINE_CURVE ( ( 0.9330127018922194093, 0.9330127018922194093, 1.000000000000000000, 0.8660254037844387076, 1.000000000000000000, 0.8660254037844387076, 1.000000000000000000, 0.9330127018922194093, 0.9330127018922194093 ) ) 
 REPRESENTATION_ITEM ( '' )  );
#5315=CARTESIAN_POINT ( 'NONE',  ( -4.458734124999999437, -66.39583333196773651, -2.574251347313719407 ) ) ;
#5317=CARTESIAN_POINT ( 'NONE',  ( -4.458734124999999437, 19.60416666803225993, -2.574251347313719407 ) ) ;
#5319=CARTESIAN_POINT ( 'NONE',  ( -2.229367062499996610, -47.39583333196774362, 3.861377020970582219 ) ) ;
#5320=CARTESIAN_POINT ( 'NONE',  ( 2.499999999999998668, -8.208333330602144429, -4.330127018922193649 ) ) ;
#5324=CARTESIAN_POINT ( 'NONE',  ( 4.458734124999999437, -107.8124999986343937, -5.460374474430324690E-16 ) ) ;
#5326=CARTESIAN_POINT ( 'NONE',  ( -2.229367062500000163, -13.72916666530107221, -3.861377020970580443 ) ) ;
#5328=( BOUNDED_CURVE ( )  B_SPLINE_CURVE ( 2, ( #12991, #46777, #32614, #2723, #56760, #47717, #12682, #52240, #22345 ),
 .UNSPECIFIED., .F., .F. ) 
 B_SPLINE_CURVE_WITH_KNOTS ( ( 3, 2, 2, 2, 3 ),
 ( 0.2803571428571428603, 0.2809523809523809534, 0.2821428571428571397, 0.2833333333333333259, 0.2839285714285714191 ),
 .UNSPECIFIED. ) 
 CURVE ( )  GEOMETRIC_REPRESENTATION_ITEM ( )  RATIONAL_B_SPLINE_CURVE ( ( 0.9330127018922194093, 0.9330127018922194093, 1.000000000000000000, 0.8660254037844387076, 1.000000000000000000, 0.8660254037844387076, 1.000000000000000000, 0.9330127018922194093, 0.9330127018922194093 ) ) 
 REPRESENTATION_ITEM ( '' )  );
#5329=CARTESIAN_POINT ( 'NONE',  ( -1.339745962155613812, -47.08034179853029144, -5.000000000000000000 ) ) ;
#5330=CARTESIAN_POINT ( 'NONE',  ( -4.458734124999998549, -100.2291666653010509, 2.574251347313722516 ) ) ;
#5332=CARTESIAN_POINT ( 'NONE',  ( -2.229367062499996610, -97.39583333196773651, 3.861377020970582219 ) ) ;
#5334=CARTESIAN_POINT ( 'NONE',  ( 5.000000000000000888, -57.45833333060214443, 2.886751345948126879 ) ) ;
#5335=DIRECTION ( 'NONE',  ( -0.000000000000000000, 1.000000000000000000, -0.000000000000000000 ) ) ;
#5338=CARTESIAN_POINT ( 'NONE',  ( -2.229367062500000163, -19.47916666530106866, -3.861377020970580443 ) ) ;
#5339=CARTESIAN_POINT ( 'NONE',  ( -4.458734124999999437, 6.437500001365593860, 0.000000000000000000 ) ) ;
#5340=CARTESIAN_POINT ( 'NONE',  ( -4.458734124999997661, -58.47916666530106511, 2.574251347313722516 ) ) ;
#5345=CARTESIAN_POINT ( 'NONE',  ( 5.000000000000000000, -4.499999999999997335, -6.123233995736766282E-16 ) ) ;
#5349=CARTESIAN_POINT ( 'NONE',  ( 5.000000000000000888, -66.58333333333332860, 2.886751345948126879 ) ) ;
#5351=CARTESIAN_POINT ( 'NONE',  ( 4.458734124999999437, -91.81249999863440792, -5.460374474430324690E-16 ) ) ;
#5352=CARTESIAN_POINT ( 'NONE',  ( -2.229367062500000163, 17.27083333469892779, -3.861377020970580443 ) ) ;
#5354=CARTESIAN_POINT ( 'NONE',  ( -6.972266317189433020E-16, -48.24999999999999289, -5.000000000000000000 ) ) ;
#5357=CARTESIAN_POINT ( 'NONE',  ( 5.000000000000000888, -77.58333333333334281, 2.886751345948126879 ) ) ;
#5360=DIRECTION ( 'NONE',  ( -0.000000000000000000, 1.000000000000000000, -0.000000000000000000 ) ) ;
#5361=ORIENTED_EDGE ( 'NONE', *, *, #55412, .T. ) ;
#5366=ORIENTED_EDGE ( 'NONE', *, *, #26102, .T. ) ;
#5373=CARTESIAN_POINT ( 'NONE',  ( -2.229367062500000163, -64.72916666530106511, -3.861377020970580443 ) ) ;
#5380=ORIENTED_EDGE ( 'NONE', *, *, #29018, .F. ) ;
#5383=CARTESIAN_POINT ( 'NONE',  ( 9.457646018065525792E-16, -105.3124999986344221, 5.148502694627439702 ) ) ;
#5384=CARTESIAN_POINT ( 'NONE',  ( 1.339745962155612702, 20.70534180126147916, -5.000000000000000000 ) ) ;
#5389=CARTESIAN_POINT ( 'NONE',  ( 9.457646018065525792E-16, -42.06249999863440081, 5.148502694627439702 ) ) ;
#5393=CARTESIAN_POINT ( 'NONE',  ( 4.458734124999999437, -10.81249999863440792, -5.460374474430324690E-16 ) ) ;
#5394=CARTESIAN_POINT ( 'NONE',  ( -5.000000000000000000, -103.0833333333333428, -2.886751345948128211 ) ) ;
#5397=CARTESIAN_POINT ( 'NONE',  ( 4.458734124999999437, -33.06249999863440792, -5.460374474430324690E-16 ) ) ;
#5398=CARTESIAN_POINT ( 'NONE',  ( -4.999999999999999112, 7.208333336064517205, 2.886751345948131764 ) ) ;
#5404=CARTESIAN_POINT ( 'NONE',  ( -4.458734124999999437, 1.354166668032261933, -2.574251347313719407 ) ) ;
#5406=CARTESIAN_POINT ( 'NONE',  ( 5.000000000000000000, -30.50000000000000000, -6.123233995736766282E-16 ) ) ;
#5407=CARTESIAN_POINT ( 'NONE',  ( 1.339745962155612702, -57.29465819873851729, -5.000000000000000000 ) ) ;
#5408=CARTESIAN_POINT ( 'NONE',  ( 5.000000000000000000, -94.50000000000000000, -6.123233995736766282E-16 ) ) ;
#5409=CARTESIAN_POINT ( 'NONE',  ( 4.458734125000001214, -31.89583333196773651, 2.574251347313718519 ) ) ;
#5410=CARTESIAN_POINT ( 'NONE',  ( 4.458734124999998549, -79.97916666530107932, -2.574251347313721627 ) ) ;
#5412=CARTESIAN_POINT ( 'NONE',  ( -6.972266317189433020E-16, -63.12499999726880873, -5.000000000000000000 ) ) ;
#5413=( BOUNDED_CURVE ( )  B_SPLINE_CURVE ( 2, ( #22723, #7299, #16618, #27220, #13057, #42321, #3106, #41051, #16936 ),
 .UNSPECIFIED., .F., .F. ) 
 B_SPLINE_CURVE_WITH_KNOTS ( ( 3, 2, 2, 2, 3 ),
 ( 0.04107142857142857123, 0.04166666666666666435, 0.04285714285714285754, 0.04404761904761905073, 0.04464285714285714385 ),
 .UNSPECIFIED. ) 
 CURVE ( )  GEOMETRIC_REPRESENTATION_ITEM ( )  RATIONAL_B_SPLINE_CURVE ( ( 0.9330127018922194093, 0.9330127018922194093, 1.000000000000000000, 0.8660254037844387076, 1.000000000000000000, 0.8660254037844387076, 1.000000000000000000, 0.9330127018922194093, 0.9330127018922194093 ) ) 
 REPRESENTATION_ITEM ( '' )  );
#5415=CARTESIAN_POINT ( 'NONE',  ( 2.229367062499998831, -2.645833331967738289, -3.861377020970580887 ) ) ;
#5416=CARTESIAN_POINT ( 'NONE',  ( -4.458734124999999437, 22.35416666803225638, -2.574251347313719407 ) ) ;
#5417=CARTESIAN_POINT ( 'NONE',  ( -4.458734124999999437, -41.56249999863440081, 0.000000000000000000 ) ) ;
#5418=FACE_OUTER_BOUND ( 'NONE', #40906, .T. ) ;
#5422=CARTESIAN_POINT ( 'NONE',  ( 2.229367062500001939, -75.97916666530106511, 3.861377020970579999 ) ) ;
#5423=CARTESIAN_POINT ( 'NONE',  ( 2.499999999999998668, -107.2083333306021444, -4.330127018922193649 ) ) ;
#5425=CARTESIAN_POINT ( 'NONE',  ( 1.975475456537005874E-15, -64.74999999999998579, 5.000000000000000000 ) ) ;
#5426=CARTESIAN_POINT ( 'NONE',  ( -4.458734124999999437, -109.6458333319677365, -2.574251347313719407 ) ) ;
#5428=CARTESIAN_POINT ( 'NONE',  ( -5.000000000000000000, -60.00000000000000000, 0.000000000000000000 ) ) ;
#5429=CARTESIAN_POINT ( 'NONE',  ( 2.500000000000002220, -36.54166666393547303, 4.330127018922192761 ) ) ;
#5431=ORIENTED_EDGE ( 'NONE', *, *, #47833, .T. ) ;
#5432=DIRECTION ( 'NONE',  ( -0.000000000000000000, 1.000000000000000000, -0.000000000000000000 ) ) ;
#5433=CARTESIAN_POINT ( 'NONE',  ( 5.000000000000000888, -67.58333333333332860, 2.886751345948126879 ) ) ;
#5436=EDGE_CURVE ( 'NONE', #10376, #41255, #21756, .T. ) ;
#5440=VERTEX_POINT ( 'NONE', #28143 ) ;
#5441=CARTESIAN_POINT ( 'NONE',  ( 2.499999999999998668, -35.20833333060213732, -4.330127018922193649 ) ) ;
#5448=CARTESIAN_POINT ( 'NONE',  ( 4.458734124999999437, -42.06249999863440081, -5.460374474430324690E-16 ) ) ;
#5449=CARTESIAN_POINT ( 'NONE',  ( 1.339745962155615144, -68.58034179853028434, 4.999999999999999112 ) ) ;
#5455=EDGE_CURVE ( 'NONE', #16461, #59581, #51700, .T. ) ;
#5458=EDGE_CURVE ( 'NONE', #29318, #50188, #38121, .T. ) ;
#5459=CARTESIAN_POINT ( 'NONE',  ( 9.457646018065525792E-16, -91.31249999863440792, 5.148502694627439702 ) ) ;
#5460=CARTESIAN_POINT ( 'NONE',  ( -6.972266317189433020E-16, -107.2499999999999858, -5.000000000000000000 ) ) ;
#5462=ORIENTED_EDGE ( 'NONE', *, *, #3884, .F. ) ;
#5463=CARTESIAN_POINT ( 'NONE',  ( -4.999999999999998224, -31.91666666666666430, 2.886751345948131764 ) ) ;
#5469=CARTESIAN_POINT ( 'NONE',  ( 2.229367062500001939, 4.020833334698926009, 3.861377020970579999 ) ) ;
#5470=CARTESIAN_POINT ( 'NONE',  ( -6.972266317189433020E-16, -50.12499999726881583, -5.000000000000000000 ) ) ;
#5471=CARTESIAN_POINT ( 'NONE',  ( 9.457646018065525792E-16, -19.31249999863440792, 5.148502694627439702 ) ) ;
#5472=CARTESIAN_POINT ( 'NONE',  ( -1.339745962155610925, -100.6696581960073331, 5.000000000000000000 ) ) ;
#5476=CARTESIAN_POINT ( 'NONE',  ( -2.229367062499996610, 23.60416666803225993, 3.861377020970582219 ) ) ;
#5477=ORIENTED_EDGE ( 'NONE', *, *, #18788, .T. ) ;
#5478=CARTESIAN_POINT ( 'NONE',  ( 4.458734125000000326, -96.89583333196773651, 2.574251347313718519 ) ) ;
#5479=FACE_OUTER_BOUND ( 'NONE', #12056, .T. ) ;
#5480=CARTESIAN_POINT ( 'NONE',  ( -5.000000000000000000, -20.99999999999999645, 0.000000000000000000 ) ) ;
#5481=CARTESIAN_POINT ( 'NONE',  ( -4.458734124999998549, -15.22916666530107754, 2.574251347313722516 ) ) ;
#5483=DIRECTION ( 'NONE',  ( -0.000000000000000000, 1.000000000000000000, -0.000000000000000000 ) ) ;
#5486=CARTESIAN_POINT ( 'NONE',  ( 5.000000000000000888, -40.45833333060214443, 2.886751345948126879 ) ) ;
#5488=CARTESIAN_POINT ( 'NONE',  ( 2.229367062499998831, 12.35416666803226171, -3.861377020970580887 ) ) ;
#5492=CARTESIAN_POINT ( 'NONE',  ( -4.458734124999998549, -60.22916666530106511, 2.574251347313722516 ) ) ;
#5495=CARTESIAN_POINT ( 'NONE',  ( -2.499999999999996447, 5.166666666666666963, 4.330127018922195425 ) ) ;
#5498=CARTESIAN_POINT ( 'NONE',  ( -3.152548672688508926E-16, -53.56249999863439371, -5.148502694627439702 ) ) ;
#5499=CARTESIAN_POINT ( 'NONE',  ( -2.499999999999996447, -89.70833333060214443, 4.330127018922195425 ) ) ;
#5500=CARTESIAN_POINT ( 'NONE',  ( 2.229367062500001939, -32.97916666530106511, 3.861377020970579999 ) ) ;
#5501=DIRECTION ( 'NONE',  ( 0.000000000000000000, 0.000000000000000000, 1.000000000000000000 ) ) ;
#5503=CARTESIAN_POINT ( 'NONE',  ( -5.000000000000000000, -41.99999999999999289, 0.000000000000000000 ) ) ;
#5504=CARTESIAN_POINT ( 'NONE',  ( -5.000000000000000000, -110.8749999972688016, 0.000000000000000000 ) ) ;
#5507=CARTESIAN_POINT ( 'NONE',  ( 4.458734125000001214, -98.89583333196775072, 2.574251347313718519 ) ) ;
#5508=CARTESIAN_POINT ( 'NONE',  ( 9.457646018065525792E-16, 1.687500001365593194, 5.148502694627439702 ) ) ;
#5510=CARTESIAN_POINT ( 'NONE',  ( 0.000000000000000000, -120.0000000000000000, 0.000000000000000000 ) ) ;
#5512=EDGE_CURVE ( 'NONE', #6430, #63596, #49614, .T. ) ;
#5519=EDGE_LOOP ( 'NONE', ( #51401, #36659, #50820, #39465 ) ) ;
#5524=DIRECTION ( 'NONE',  ( -0.000000000000000000, 1.000000000000000000, -0.000000000000000000 ) ) ;
#5525=CARTESIAN_POINT ( 'NONE',  ( -4.458734124999999437, -27.64583333196774007, -2.574251347313719407 ) ) ;
#5535=CARTESIAN_POINT ( 'NONE',  ( 2.500000000000002220, -20.54166666393548013, 4.330127018922192761 ) ) ;
#5538=CARTESIAN_POINT ( 'NONE',  ( -2.229367062500000163, -73.72916666530106511, -3.861377020970580443 ) ) ;
#5539=DIRECTION ( 'NONE',  ( -0.000000000000000000, 1.000000000000000000, -0.000000000000000000 ) ) ;
#5541=ORIENTED_EDGE ( 'NONE', *, *, #48776, .T. ) ;
#5545=CARTESIAN_POINT ( 'NONE',  ( 4.458734124999999437, -6.062499998634403475, -5.460374474430324690E-16 ) ) ;
#5547=CARTESIAN_POINT ( 'NONE',  ( -2.500000000000000444, -20.16666666666666430, -4.330127018922193649 ) ) ;
#5555=CARTESIAN_POINT ( 'NONE',  ( 4.458734124999998549, -83.72916666530106511, -2.574251347313721627 ) ) ;
#5556=CARTESIAN_POINT ( 'NONE',  ( 5.000000000000000000, -0.2916666639354824619, -2.886751345948130876 ) ) ;
#5557=CARTESIAN_POINT ( 'NONE',  ( -2.229367062500000163, 0.5208333346989266754, -3.861377020970580443 ) ) ;
#5558=CYLINDRICAL_SURFACE ( 'NONE', #63274, 5.000000000000000000 ) ;
#5559=CARTESIAN_POINT ( 'NONE',  ( -2.500000000000000444, -84.16666666666667140, -4.330127018922193649 ) ) ;
#5561=CARTESIAN_POINT ( 'NONE',  ( -4.458734124999999437, -66.64583333196773651, -2.574251347313719407 ) ) ;
#5562=CARTESIAN_POINT ( 'NONE',  ( -3.535250795749689387E-16, -23.12499999726881228, -5.773502691896257311 ) ) ;
#5563=CARTESIAN_POINT ( 'NONE',  ( -5.000000000000000000, -41.08333333333333570, -2.886751345948128211 ) ) ;
#5564=CARTESIAN_POINT ( 'NONE',  ( -2.499999999999996447, -37.70833333060213732, 4.330127018922195425 ) ) ;
#5565=CARTESIAN_POINT ( 'NONE',  ( 2.500000000000002220, -43.54166666393548013, 4.330127018922192761 ) ) ;
#5566=CARTESIAN_POINT ( 'NONE',  ( 9.457646018065525792E-16, -44.06249999863439371, 5.148502694627439702 ) ) ;
#5567=CARTESIAN_POINT ( 'NONE',  ( -2.229367062499996610, -33.39583333196772941, 3.861377020970582219 ) ) ;
#5570=CARTESIAN_POINT ( 'NONE',  ( -2.499999999999996447, 18.16666666666666430, 4.330127018922195425 ) ) ;
#5573=CARTESIAN_POINT ( 'NONE',  ( -4.458734124999999437, -38.31249999863439371, 0.000000000000000000 ) ) ;
#5574=CARTESIAN_POINT ( 'NONE',  ( 5.000000000000000000, -75.29166666393547303, -2.886751345948129988 ) ) ;
#5577=CARTESIAN_POINT ( 'NONE',  ( 0.000000000000000000, -120.0000000000000000, 5.000000000000000000 ) ) ;
#5578=CARTESIAN_POINT ( 'NONE',  ( 2.229367062499998831, -82.89583333196773651, -3.861377020970580887 ) ) ;
#5582=CARTESIAN_POINT ( 'NONE',  ( -5.000000000000000000, -27.99999999999999645, 0.000000000000000000 ) ) ;
#5588=CARTESIAN_POINT ( 'NONE',  ( -2.500000000000000444, 21.95833333606451987, -4.330127018922193649 ) ) ;
#5589=CARTESIAN_POINT ( 'NONE',  ( -5.000000000000000000, -60.95833333060214443, -2.886751345948128211 ) ) ;
#5592=( BOUNDED_CURVE ( )  B_SPLINE_CURVE ( 2, ( #49355, #63526, #28785, #15264, #34888, #43565, #58691, #49030, #39691 ),
 .UNSPECIFIED., .F., .F. ) 
 B_SPLINE_CURVE_WITH_KNOTS ( ( 3, 2, 2, 2, 3 ),
 ( 0.3732142857142857206, 0.3738095238095238138, 0.3750000000000000000, 0.3761904761904761862, 0.3767857142857142794 ),
 .UNSPECIFIED. ) 
 CURVE ( )  GEOMETRIC_REPRESENTATION_ITEM ( )  RATIONAL_B_SPLINE_CURVE ( ( 0.9330127018922194093, 0.9330127018922194093, 1.000000000000000000, 0.8660254037844387076, 1.000000000000000000, 0.8660254037844387076, 1.000000000000000000, 0.9330127018922194093, 0.9330127018922194093 ) ) 
 REPRESENTATION_ITEM ( '' )  );
#5596=EDGE_CURVE ( 'NONE', #1202, #31117, #8488, .T. ) ;
#5597=CARTESIAN_POINT ( 'NONE',  ( 1.975475456537005874E-15, -22.62499999726880873, 5.000000000000000000 ) ) ;
#5599=CARTESIAN_POINT ( 'NONE',  ( -1.339745962155610925, -79.66965819600731891, 5.000000000000000000 ) ) ;
#5600=CARTESIAN_POINT ( 'NONE',  ( 1.339745962155615144, -74.70534180126148271, 4.999999999999999112 ) ) ;
#5602=CARTESIAN_POINT ( 'NONE',  ( -4.458734124999999437, -22.31249999863440436, 0.000000000000000000 ) ) ;
#5604=CARTESIAN_POINT ( 'NONE',  ( -5.000000000000000000, -77.95833333060214443, -2.886751345948128211 ) ) ;
#5609=( BOUNDED_CURVE ( )  B_SPLINE_CURVE ( 2, ( #30992, #39996, #21352, #1116, #11684, #40957, #16523, #20722, #55453 ),
 .UNSPECIFIED., .F., .F. ) 
 B_SPLINE_CURVE_WITH_KNOTS ( ( 3, 2, 2, 2, 3 ),
 ( 0.6553571428571428603, 0.6559523809523809534, 0.6571428571428571397, 0.6583333333333333259, 0.6589285714285714191 ),
 .UNSPECIFIED. ) 
 CURVE ( )  GEOMETRIC_REPRESENTATION_ITEM ( )  RATIONAL_B_SPLINE_CURVE ( ( 0.9330127018922194093, 0.9330127018922194093, 1.000000000000000000, 0.8660254037844387076, 1.000000000000000000, 0.8660254037844387076, 1.000000000000000000, 0.9330127018922194093, 0.9330127018922194093 ) ) 
 REPRESENTATION_ITEM ( '' )  );
#5612=CARTESIAN_POINT ( 'NONE',  ( 1.339745962155612702, 13.70534180126148094, -5.000000000000000000 ) ) ;
#5614=ORIENTED_EDGE ( 'NONE', *, *, #35780, .T. ) ;
#5615=CARTESIAN_POINT ( 'NONE',  ( 5.000000000000000888, -21.58333333333332860, 2.886751345948126879 ) ) ;
#5616=DIRECTION ( 'NONE',  ( 0.000000000000000000, 0.000000000000000000, 1.000000000000000000 ) ) ;
#5618=EDGE_CURVE ( 'NONE', #33683, #29077, #21354, .T. ) ;
#5620=ADVANCED_FACE ( 'NONE', ( #39675 ), #59311, .T. ) ;
#5621=CARTESIAN_POINT ( 'NONE',  ( -2.499999999999996447, 11.16666666666666430, 4.330127018922195425 ) ) ;
#5623=CARTESIAN_POINT ( 'NONE',  ( 1.339745962155615144, -86.70534180126148271, 4.999999999999999112 ) ) ;
#5625=ORIENTED_EDGE ( 'NONE', *, *, #19746, .F. ) ;
#5628=CARTESIAN_POINT ( 'NONE',  ( -2.229367062499996610, 13.85416666803226171, 3.861377020970582219 ) ) ;
#5631=CARTESIAN_POINT ( 'NONE',  ( 2.499999999999998668, 12.79166666939785379, -4.330127018922193649 ) ) ;
#5634=CARTESIAN_POINT ( 'NONE',  ( 4.458734124999998549, -67.72916666530106511, -2.574251347313721627 ) ) ;
#5636=CARTESIAN_POINT ( 'NONE',  ( 4.458734125000001214, 19.10416666803225638, 2.574251347313718519 ) ) ;
#5637=CARTESIAN_POINT ( 'NONE',  ( 4.458734124999999437, -50.06249999863440792, -5.460374474430324690E-16 ) ) ;
#5638=CARTESIAN_POINT ( 'NONE',  ( 1.060575238724906964E-15, -8.624999997268814056, 5.773502691896257311 ) ) ;
#5641=DIRECTION ( 'NONE',  ( -0.000000000000000000, 1.000000000000000000, -0.000000000000000000 ) ) ;
#5642=CARTESIAN_POINT ( 'NONE',  ( 1.339745962155615144, -64.58034179853029855, 4.999999999999999112 ) ) ;
#5643=CARTESIAN_POINT ( 'NONE',  ( -4.458734124999997661, -18.47916666530106511, 2.574251347313722516 ) ) ;
#5645=CARTESIAN_POINT ( 'NONE',  ( 5.000000000000000000, 23.50000000000000000, -6.123233995736766282E-16 ) ) ;
#5646=CARTESIAN_POINT ( 'NONE',  ( -4.458734124999999437, -102.3958333319677365, -2.574251347313719407 ) ) ;
#5648=ORIENTED_EDGE ( 'NONE', *, *, #47152, .T. ) ;
#5649=CARTESIAN_POINT ( 'NONE',  ( 2.229367062500001939, -97.22916666530105090, 3.861377020970579999 ) ) ;
#5651=CARTESIAN_POINT ( 'NONE',  ( -5.000000000000000000, -54.87499999726880162, 0.000000000000000000 ) ) ;
#5656=CARTESIAN_POINT ( 'NONE',  ( -3.152548672688508926E-16, -17.56249999863440792, -5.148502694627439702 ) ) ;
#5657=CARTESIAN_POINT ( 'NONE',  ( -4.458734124999998549, 8.520833334698926009, 2.574251347313722516 ) ) ;
#5658=CARTESIAN_POINT ( 'NONE',  ( -2.229367062500000163, -65.72916666530106511, -3.861377020970580443 ) ) ;
#5659=DIRECTION ( 'NONE',  ( -0.000000000000000000, -1.000000000000000000, -0.000000000000000000 ) ) ;
#5663=CARTESIAN_POINT ( 'NONE',  ( 5.000000000000000000, -9.416666666666662522, -2.886751345948129988 ) ) ;
#5669=CARTESIAN_POINT ( 'NONE',  ( -5.000000000000000000, -9.083333333333333925, -2.886751345948128211 ) ) ;
#5671=CARTESIAN_POINT ( 'NONE',  ( 2.229367062500001939, -89.97916666530106511, 3.861377020970579999 ) ) ;
#5673=CARTESIAN_POINT ( 'NONE',  ( 5.000000000000000888, -0.5833333333333350357, 2.886751345948126879 ) ) ;
#5675=CARTESIAN_POINT ( 'NONE',  ( 5.000000000000000888, 20.54166666939784847, 2.886751345948126879 ) ) ;
#5677=CARTESIAN_POINT ( 'NONE',  ( 2.500000000000002220, -76.66666666666665719, 4.330127018922192761 ) ) ;
#5682=CARTESIAN_POINT ( 'NONE',  ( 5.000000000000000000, 26.58333333333333215, -2.886751345948130876 ) ) ;
#5685=ORIENTED_EDGE ( 'NONE', *, *, #21379, .F. ) ;
#5691=CARTESIAN_POINT ( 'NONE',  ( 2.229367062500001939, -61.22916666530106511, 3.861377020970579999 ) ) ;
#5699=ORIENTED_EDGE ( 'NONE', *, *, #44705, .T. ) ;
#5700=VECTOR ( 'NONE', #12295, 1000.000000000000000 ) ;
#5702=CARTESIAN_POINT ( 'NONE',  ( 4.458734125000001214, 28.10416666803225993, 2.574251347313718519 ) ) ;
#5708=CARTESIAN_POINT ( 'NONE',  ( 4.458734124999998549, -41.72916666530107932, -2.574251347313721627 ) ) ;
#5711=CARTESIAN_POINT ( 'NONE',  ( 2.229367062500001939, -47.97916666530106511, 3.861377020970579999 ) ) ;
#5712=CARTESIAN_POINT ( 'NONE',  ( 1.975475456537005874E-15, -70.75000000000000000, 5.000000000000000000 ) ) ;
#5713=CARTESIAN_POINT ( 'NONE',  ( 4.458734124999999437, -15.81249999863440436, -5.460374474430324690E-16 ) ) ;
#5714=CARTESIAN_POINT ( 'NONE',  ( 5.000000000000000888, -101.5833333333333286, 2.886751345948126879 ) ) ;
#5716=CARTESIAN_POINT ( 'NONE',  ( 4.458734125000001214, -32.14583333196773651, 2.574251347313718519 ) ) ;
#5717=CARTESIAN_POINT ( 'NONE',  ( 2.499999999999998668, 7.791666669397852019, -4.330127018922193649 ) ) ;
#5721=CARTESIAN_POINT ( 'NONE',  ( 0.000000000000000000, -120.0000000000000000, 0.000000000000000000 ) ) ;
#5724=CARTESIAN_POINT ( 'NONE',  ( 2.229367062500001939, -2.229166665301068662, 3.861377020970579999 ) ) ;
#5726=CARTESIAN_POINT ( 'NONE',  ( 5.000000000000000000, 16.62500000273118417, -6.123233995736766282E-16 ) ) ;
#5728=CARTESIAN_POINT ( 'NONE',  ( -4.458734124999999437, -88.39583333196773651, -2.574251347313719407 ) ) ;
#5729=CARTESIAN_POINT ( 'NONE',  ( 2.229367062500001939, -37.97916666530107221, 3.861377020970579999 ) ) ;
#5730=CARTESIAN_POINT ( 'NONE',  ( -1.339745962155613812, -36.20534180126147561, -5.000000000000000000 ) ) ;
#5731=CARTESIAN_POINT ( 'NONE',  ( -2.229367062499996610, -79.39583333196773651, 3.861377020970582219 ) ) ;
#5735=CARTESIAN_POINT ( 'NONE',  ( 4.458734124999998549, 0.2708333346989263979, -2.574251347313721627 ) ) ;
#5736=CARTESIAN_POINT ( 'NONE',  ( -2.229367062499996610, 19.60416666803225993, 3.861377020970582219 ) ) ;
#5737=CARTESIAN_POINT ( 'NONE',  ( 2.229367062500001939, -47.22916666530106511, 3.861377020970579999 ) ) ;
#5738=CARTESIAN_POINT ( 'NONE',  ( 5.000000000000000000, -15.41666666666666963, -2.886751345948130876 ) ) ;
#5742=CARTESIAN_POINT ( 'NONE',  ( -2.229367062499996610, -76.14583333196773651, 3.861377020970582219 ) ) ;
#5743=CARTESIAN_POINT ( 'NONE',  ( -5.000000000000000000, -105.9583333306021586, -2.886751345948128211 ) ) ;
#5747=CARTESIAN_POINT ( 'NONE',  ( -2.229367062499996610, -109.3958333319677365, 3.861377020970582219 ) ) ;
#5749=CARTESIAN_POINT ( 'NONE',  ( 2.500000000000002220, -61.66666666666666430, 4.330127018922192761 ) ) ;
#5750=CYLINDRICAL_SURFACE ( 'NONE', #54165, 5.000000000000000000 ) ;
#5761=CARTESIAN_POINT ( 'NONE',  ( -1.339745962155613812, -76.08034179853028434, -5.000000000000000000 ) ) ;
#5768=CARTESIAN_POINT ( 'NONE',  ( -3.152548672688508926E-16, -48.81249999863440792, -5.148502694627439702 ) ) ;
#5769=LINE ( 'NONE', #30523, #9089 ) ;
#5776=CARTESIAN_POINT ( 'NONE',  ( 2.229367062500001939, -93.22916666530106511, 3.861377020970579999 ) ) ;
#5777=CARTESIAN_POINT ( 'NONE',  ( 1.975475456537005874E-15, 4.375000002731185056, 5.000000000000000000 ) ) ;
#5782=AXIS2_PLACEMENT_3D ( 'NONE', #31949, #11687, #57048 ) ;
#5786=CARTESIAN_POINT ( 'NONE',  ( 9.457646018065525792E-16, 1.937500001365593416, 5.148502694627439702 ) ) ;
#5788=( BOUNDED_CURVE ( )  B_SPLINE_CURVE ( 2, ( #47931, #62748, #18355, #47621, #8701, #13538, #47319, #43107, #28316 ),
 .UNSPECIFIED., .F., .F. ) 
 B_SPLINE_CURVE_WITH_KNOTS ( ( 3, 2, 2, 2, 3 ),
 ( 0.6017857142857142572, 0.6023809523809523503, 0.6035714285714285365, 0.6047619047619047228, 0.6053571428571428159 ),
 .UNSPECIFIED. ) 
 CURVE ( )  GEOMETRIC_REPRESENTATION_ITEM ( )  RATIONAL_B_SPLINE_CURVE ( ( 0.9330127018922194093, 0.9330127018922194093, 1.000000000000000000, 0.8660254037844387076, 1.000000000000000000, 0.8660254037844387076, 1.000000000000000000, 0.9330127018922194093, 0.9330127018922194093 ) ) 
 REPRESENTATION_ITEM ( '' )  );
#5789=CARTESIAN_POINT ( 'NONE',  ( 1.975475456537005874E-15, -1.624999997268813834, 5.000000000000000000 ) ) ;
#5790=CARTESIAN_POINT ( 'NONE',  ( -4.458734124999999437, -16.64583333196773651, -2.574251347313719407 ) ) ;
#5793=CARTESIAN_POINT ( 'NONE',  ( -2.499999999999996447, -73.70833333060214443, 4.330127018922195425 ) ) ;
#5795=CARTESIAN_POINT ( 'NONE',  ( -4.458734124999997661, 16.52083333469892779, 2.574251347313722516 ) ) ;
#5796=ORIENTED_EDGE ( 'NONE', *, *, #47579, .F. ) ;
#5797=CARTESIAN_POINT ( 'NONE',  ( -5.000000000000000000, -13.87499999726881228, 0.000000000000000000 ) ) ;
#5799=CARTESIAN_POINT ( 'NONE',  ( -2.229367062499996610, -20.14583333196774007, 3.861377020970582219 ) ) ;
#5800=EDGE_CURVE ( 'NONE', #58830, #45091, #15052, .T. ) ;
#5802=CARTESIAN_POINT ( 'NONE',  ( 6.123233995736766282E-16, -120.0000000000000000, -5.000000000000000000 ) ) ;
#5804=CARTESIAN_POINT ( 'NONE',  ( -5.000000000000000000, -45.95833333060214443, -2.886751345948128211 ) ) ;
#5806=CARTESIAN_POINT ( 'NONE',  ( -4.458734124999999437, 15.68750000136559564, 0.000000000000000000 ) ) ;
#5807=FACE_OUTER_BOUND ( 'NONE', #9168, .T. ) ;
#5810=CARTESIAN_POINT ( 'NONE',  ( -2.229367062499996610, -60.14583333196774362, 3.861377020970582219 ) ) ;
#5811=EDGE_LOOP ( 'NONE', ( #46094, #27357, #2845, #56498 ) ) ;
#5813=CARTESIAN_POINT ( 'NONE',  ( -3.535250795749689387E-16, 4.750000000000000888, -5.773502691896257311 ) ) ;
#5816=CARTESIAN_POINT ( 'NONE',  ( 4.458734124999998549, -59.72916666530106511, -2.574251347313721627 ) ) ;
#5817=CARTESIAN_POINT ( 'NONE',  ( -2.500000000000000444, -92.04166666393547303, -4.330127018922193649 ) ) ;
#5818=CARTESIAN_POINT ( 'NONE',  ( -4.458734124999999437, -32.39583333196773651, -2.574251347313719407 ) ) ;
#5819=CARTESIAN_POINT ( 'NONE',  ( -6.972266317189433020E-16, -9.250000000000000000, -5.000000000000000000 ) ) ;
#5824=CARTESIAN_POINT ( 'NONE',  ( 1.339745962155615144, 1.294658198738520172, 4.999999999999999112 ) ) ;
#5826=CARTESIAN_POINT ( 'NONE',  ( -5.000000000000000000, -45.08333333333333570, -2.886751345948128211 ) ) ;
#5828=FACE_OUTER_BOUND ( 'NONE', #991, .T. ) ;
#5829=ORIENTED_EDGE ( 'NONE', *, *, #57324, .F. ) ;
#5830=CARTESIAN_POINT ( 'NONE',  ( 2.229367062499998831, -99.64583333196773651, -3.861377020970580887 ) ) ;
#5831=CARTESIAN_POINT ( 'NONE',  ( -2.229367062500000163, 4.270833334698926897, -3.861377020970580443 ) ) ;
#5832=VECTOR ( 'NONE', #14664, 1000.000000000000000 ) ;
#5835=VECTOR ( 'NONE', #27828, 1000.000000000000000 ) ;
#5837=VECTOR ( 'NONE', #57469, 1000.000000000000000 ) ;
#5841=VERTEX_POINT ( 'NONE', #16206 ) ;
#5843=CARTESIAN_POINT ( 'NONE',  ( 1.975475456537005874E-15, -33.75000000000000000, 5.000000000000000000 ) ) ;
#5845=ORIENTED_EDGE ( 'NONE', *, *, #2776, .T. ) ;
#5846=( BOUNDED_CURVE ( )  B_SPLINE_CURVE ( 2, ( #39289, #4888, #4263, #23881, #54088, #53771, #44113, #18730, #76 ),
 .UNSPECIFIED., .F., .F. ) 
 B_SPLINE_CURVE_WITH_KNOTS ( ( 3, 2, 2, 2, 3 ),
 ( 0.04821428571428571647, 0.04880952380952380959, 0.05000000000000000278, 0.05119047619047618902, 0.05178571428571428908 ),
 .UNSPECIFIED. ) 
 CURVE ( )  GEOMETRIC_REPRESENTATION_ITEM ( )  RATIONAL_B_SPLINE_CURVE ( ( 0.9330127018922194093, 0.9330127018922197424, 1.000000000000000000, 0.8660254037844387076, 1.000000000000000000, 0.8660254037844387076, 1.000000000000000000, 0.9330127018922189652, 0.9330127018922194093 ) ) 
 REPRESENTATION_ITEM ( '' )  );
#5847=CARTESIAN_POINT ( 'NONE',  ( -5.000000000000000000, -48.87499999726880873, 0.000000000000000000 ) ) ;
#5851=CARTESIAN_POINT ( 'NONE',  ( -4.458734124999999437, -29.56249999863440436, 0.000000000000000000 ) ) ;
#5852=FACE_OUTER_BOUND ( 'NONE', #56182, .T. ) ;
#5860=CARTESIAN_POINT ( 'NONE',  ( 0.000000000000000000, -120.0000000000000000, 5.000000000000000000 ) ) ;
#5862=CARTESIAN_POINT ( 'NONE',  ( 4.458734125000001214, -72.14583333196773651, 2.574251347313718519 ) ) ;
#5865=CARTESIAN_POINT ( 'NONE',  ( 1.975475456537005874E-15, -16.74999999999999645, 5.000000000000000000 ) ) ;
#5868=CARTESIAN_POINT ( 'NONE',  ( -4.458734124999998549, -2.479166665301069550, 2.574251347313722516 ) ) ;
#5869=ORIENTED_EDGE ( 'NONE', *, *, #23163, .F. ) ;
#5871=CARTESIAN_POINT ( 'NONE',  ( 5.000000000000000888, -27.58333333333333570, 2.886751345948126879 ) ) ;
#5875=CARTESIAN_POINT ( 'NONE',  ( 1.975475456537005874E-15, -47.62499999726880873, 5.000000000000000000 ) ) ;
#5880=CARTESIAN_POINT ( 'NONE',  ( 4.458734125000000326, -81.89583333196773651, 2.574251347313718519 ) ) ;
#5881=FACE_OUTER_BOUND ( 'NONE', #33937, .T. ) ;
#5882=CARTESIAN_POINT ( 'NONE',  ( 4.458734124999998549, -4.729166665301071326, -2.574251347313721627 ) ) ;
#5886=CYLINDRICAL_SURFACE ( 'NONE', #51068, 5.000000000000000000 ) ;
#5887=CARTESIAN_POINT ( 'NONE',  ( -3.152548672688508926E-16, -69.81249999863439371, -5.148502694627439702 ) ) ;
#5888=CARTESIAN_POINT ( 'NONE',  ( 5.000000000000000000, -26.37499999726881583, -6.123233995736766282E-16 ) ) ;
#5890=CARTESIAN_POINT ( 'NONE',  ( 4.458734124999999437, 29.18750000136559208, -5.460374474430324690E-16 ) ) ;
#5891=CARTESIAN_POINT ( 'NONE',  ( -1.339745962155606929, 22.79465819873851729, -5.000000000000004441 ) ) ;
#5893=CARTESIAN_POINT ( 'NONE',  ( 4.458734125000001214, -47.89583333196775072, 2.574251347313718519 ) ) ;
#5894=CARTESIAN_POINT ( 'NONE',  ( 4.458734124999998549, -29.97916666530107221, -2.574251347313721627 ) ) ;
#5898=CARTESIAN_POINT ( 'NONE',  ( -5.000000000000000000, 21.91666666666666785, -2.886751345948128211 ) ) ;
#5901=CARTESIAN_POINT ( 'NONE',  ( 4.458734124999999437, -43.81249999863440081, -5.460374474430324690E-16 ) ) ;
#5902=CARTESIAN_POINT ( 'NONE',  ( 2.500000000000002220, -72.54166666393548724, 4.330127018922192761 ) ) ;
#5905=CARTESIAN_POINT ( 'NONE',  ( 1.975475456537005874E-15, -37.74999999999999289, 5.000000000000000000 ) ) ;
#5907=CARTESIAN_POINT ( 'NONE',  ( -4.458734124999997661, -82.47916666530106511, 2.574251347313722516 ) ) ;
#5911=CARTESIAN_POINT ( 'NONE',  ( 2.500000000000002220, -28.66666666666666785, 4.330127018922192761 ) ) ;
#5913=ORIENTED_EDGE ( 'NONE', *, *, #1944, .F. ) ;
#5916=EDGE_CURVE ( 'NONE', #8062, #45518, #32583, .T. ) ;
#5918=CARTESIAN_POINT ( 'NONE',  ( -5.000000000000000000, 24.04166666939785202, -2.886751345948128211 ) ) ;
#5928=CARTESIAN_POINT ( 'NONE',  ( -3.152548672688508926E-16, -19.56249999863440081, -5.148502694627439702 ) ) ;
#5929=VECTOR ( 'NONE', #48890, 1000.000000000000000 ) ;
#5930=CARTESIAN_POINT ( 'NONE',  ( 2.493747252781420335E-13, -78.12499999726881583, -5.000000000000000000 ) ) ;
#5934=VECTOR ( 'NONE', #43303, 1000.000000000000000 ) ;
#5937=CARTESIAN_POINT ( 'NONE',  ( 5.000000000000000000, 13.58333333333333215, -2.886751345948130876 ) ) ;
#5944=CARTESIAN_POINT ( 'NONE',  ( 1.339745962155612702, -99.29465819873853150, -5.000000000000000000 ) ) ;
#5946=CARTESIAN_POINT ( 'NONE',  ( 1.339745962155615144, 15.29465819873851906, 4.999999999999999112 ) ) ;
#5950=CARTESIAN_POINT ( 'NONE',  ( 2.229367062500001939, 13.02083333469892779, 3.861377020970579999 ) ) ;
#5953=CARTESIAN_POINT ( 'NONE',  ( 0.000000000000000000, -120.0000000000000000, 0.000000000000000000 ) ) ;
#5955=CARTESIAN_POINT ( 'NONE',  ( 0.000000000000000000, -120.0000000000000000, 0.000000000000000000 ) ) ;
#5956=CARTESIAN_POINT ( 'NONE',  ( 2.229367062500001939, -67.97916666530106511, 3.861377020970579999 ) ) ;
#5957=LINE ( 'NONE', #40993, #25349 ) ;
#5958=CARTESIAN_POINT ( 'NONE',  ( 9.457646018065525792E-16, 18.93750000136559208, 5.148502694627439702 ) ) ;
#5962=EDGE_CURVE ( 'NONE', #35597, #28144, #52076, .T. ) ;
#5963=CARTESIAN_POINT ( 'NONE',  ( 4.458734124999999437, -48.06249999863440792, -5.460374474430324690E-16 ) ) ;
#5964=CARTESIAN_POINT ( 'NONE',  ( 5.000000000000000000, -8.291666663935481907, -2.886751345948129988 ) ) ;
#5965=CARTESIAN_POINT ( 'NONE',  ( -5.000000000000000000, -108.9999999999999858, 0.000000000000000000 ) ) ;
#5968=EDGE_CURVE ( 'NONE', #62355, #55212, #41352, .T. ) ;
#5969=CARTESIAN_POINT ( 'NONE',  ( 5.000000000000000000, -64.29166666393547303, -2.886751345948130876 ) ) ;
#5970=CARTESIAN_POINT ( 'NONE',  ( 4.458734125000000326, -16.14583333196773651, 2.574251347313718519 ) ) ;
#5972=VERTEX_POINT ( 'NONE', #27128 ) ;
#5974=CARTESIAN_POINT ( 'NONE',  ( 2.229367062499998831, -104.6458333319677365, -3.861377020970580887 ) ) ;
#5976=ORIENTED_EDGE ( 'NONE', *, *, #8142, .T. ) ;
#5977=CARTESIAN_POINT ( 'NONE',  ( -2.229367062499996610, -95.39583333196773651, 3.861377020970582219 ) ) ;
#5979=CARTESIAN_POINT ( 'NONE',  ( -4.999999999999998224, -7.916666666666668739, 2.886751345948131764 ) ) ;
#5980=CARTESIAN_POINT ( 'NONE',  ( -2.500000000000000444, -60.04166666393547303, -4.330127018922193649 ) ) ;
#5983=EDGE_CURVE ( 'NONE', #28793, #28403, #23250, .T. ) ;
#5987=CARTESIAN_POINT ( 'NONE',  ( 4.458734125000000326, -20.89583333196774007, 2.574251347313718519 ) ) ;
#5988=CARTESIAN_POINT ( 'NONE',  ( 2.229367062499998831, 7.104166668032259935, -3.861377020970580887 ) ) ;
#5990=CARTESIAN_POINT ( 'NONE',  ( -4.458734124999997661, -63.47916666530106511, 2.574251347313722516 ) ) ;
#5993=CARTESIAN_POINT ( 'NONE',  ( -2.499999999999996447, -32.83333333333332860, 4.330127018922195425 ) ) ;
#5995=CARTESIAN_POINT ( 'NONE',  ( 2.500000000000002220, -13.66666666666666785, 4.330127018922192761 ) ) ;
#5996=EDGE_CURVE ( 'NONE', #43569, #38517, #19171, .T. ) ;
#6000=CARTESIAN_POINT ( 'NONE',  ( 0.000000000000000000, -120.0000000000000000, 0.000000000000000000 ) ) ;
#6007=CARTESIAN_POINT ( 'NONE',  ( 0.000000000000000000, -120.0000000000000000, 0.000000000000000000 ) ) ;
#6010=CARTESIAN_POINT ( 'NONE',  ( -4.999999999999999112, -72.91666666666665719, 2.886751345948131764 ) ) ;
#6014=VERTEX_POINT ( 'NONE', #28070 ) ;
#6015=CARTESIAN_POINT ( 'NONE',  ( -1.339745962155610925, -53.66965819600733312, 5.000000000000000000 ) ) ;
#6023=AXIS2_PLACEMENT_3D ( 'NONE', #38676, #58315, #24210 ) ;
#6026=VERTEX_POINT ( 'NONE', #3638 ) ;
#6030=CARTESIAN_POINT ( 'NONE',  ( -2.500000000000000444, -84.16666666666667140, -4.330127018922193649 ) ) ;
#6031=ORIENTED_EDGE ( 'NONE', *, *, #18172, .F. ) ;
#6034=CARTESIAN_POINT ( 'NONE',  ( -2.229367062500000163, 27.52083333469892779, -3.861377020970580443 ) ) ;
#6039=CARTESIAN_POINT ( 'NONE',  ( 4.458734125000000326, -42.89583333196773651, 2.574251347313718519 ) ) ;
#6042=CARTESIAN_POINT ( 'NONE',  ( 4.458734124999999437, -46.81249999863440792, -5.460374474430324690E-16 ) ) ;
#6044=CARTESIAN_POINT ( 'NONE',  ( -2.229367062499996610, -16.14583333196773651, 3.861377020970582219 ) ) ;
#6045=CARTESIAN_POINT ( 'NONE',  ( 5.000000000000000888, -103.5833333333333428, 2.886751345948126879 ) ) ;
#6047=CARTESIAN_POINT ( 'NONE',  ( 2.229367062500001939, -35.22916666530107221, 3.861377020970579999 ) ) ;
#6048=CARTESIAN_POINT ( 'NONE',  ( 2.500000000000002220, 6.458333336064519870, 4.330127018922192761 ) ) ;
#6054=CARTESIAN_POINT ( 'NONE',  ( -3.152548672688508926E-16, 2.187500001365593416, -5.148502694627439702 ) ) ;
#6059=CARTESIAN_POINT ( 'NONE',  ( -2.229367062500000163, -88.47916666530106511, -3.861377020970580443 ) ) ;
#6060=CARTESIAN_POINT ( 'NONE',  ( -4.458734124999998549, -33.22916666530107221, 2.574251347313722516 ) ) ;
#6061=CARTESIAN_POINT ( 'NONE',  ( 2.229367062500001939, -82.22916666530106511, 3.861377020970579999 ) ) ;
#6064=CARTESIAN_POINT ( 'NONE',  ( 4.458734125000000326, -3.895833331967739177, 2.574251347313718519 ) ) ;
#6065=CARTESIAN_POINT ( 'NONE',  ( -4.458734124999999437, 23.35416666803226349, -2.574251347313719407 ) ) ;
#6066=CARTESIAN_POINT ( 'NONE',  ( -2.229367062500000163, -45.72916666530106511, -3.861377020970580443 ) ) ;
#6070=EDGE_CURVE ( 'NONE', #29896, #2056, #23333, .T. ) ;
#6071=ORIENTED_EDGE ( 'NONE', *, *, #30714, .F. ) ;
#6074=CARTESIAN_POINT ( 'NONE',  ( 2.229367062499998831, -76.64583333196773651, -3.861377020970580887 ) ) ;
#6075=CARTESIAN_POINT ( 'NONE',  ( 4.458734125000001214, 28.85416666803225993, 2.574251347313718519 ) ) ;
#6078=EDGE_CURVE ( 'NONE', #2252, #14226, #25775, .T. ) ;
#6082=CARTESIAN_POINT ( 'NONE',  ( -5.000000000000000000, -57.08333333333333570, -2.886751345948128211 ) ) ;
#6084=ORIENTED_EDGE ( 'NONE', *, *, #7605, .F. ) ;
#6092=ORIENTED_EDGE ( 'NONE', *, *, #29563, .F. ) ;
#6094=CARTESIAN_POINT ( 'NONE',  ( -6.972266317189433020E-16, -59.12499999726880873, -5.000000000000000000 ) ) ;
#6096=ORIENTED_EDGE ( 'NONE', *, *, #9100, .T. ) ;
#6100=CARTESIAN_POINT ( 'NONE',  ( -4.458734124999999437, -45.64583333196774362, -2.574251347313719407 ) ) ;
#6101=CARTESIAN_POINT ( 'NONE',  ( 2.500000000000002220, -23.66666666666666785, 4.330127018922192761 ) ) ;
#6107=CARTESIAN_POINT ( 'NONE',  ( 1.339745962155615144, -89.70534180126146850, 4.999999999999999112 ) ) ;
#6109=CARTESIAN_POINT ( 'NONE',  ( -2.229367062500000163, -95.72916666530107932, -3.861377020970580443 ) ) ;
#6111=ORIENTED_EDGE ( 'NONE', *, *, #3135, .T. ) ;
#6112=CARTESIAN_POINT ( 'NONE',  ( -1.339745962155610259, 26.91965820146970501, -5.000000000000002665 ) ) ;
#6118=CARTESIAN_POINT ( 'NONE',  ( 2.229367062499998831, -2.645833331967738289, -3.861377020970580887 ) ) ;
#6119=EDGE_CURVE ( 'NONE', #17008, #41671, #14761, .T. ) ;
#6120=CARTESIAN_POINT ( 'NONE',  ( 1.339745962155612702, -106.2946581987385173, -5.000000000000000000 ) ) ;
#6121=CARTESIAN_POINT ( 'NONE',  ( 2.229367062499998831, -19.89583333196774007, -3.861377020970580887 ) ) ;
#6125=CARTESIAN_POINT ( 'NONE',  ( -3.152548672688508926E-16, 15.18750000136559564, -5.148502694627439702 ) ) ;
#6126=ORIENTED_EDGE ( 'NONE', *, *, #31958, .F. ) ;
#6127=CARTESIAN_POINT ( 'NONE',  ( -5.000000000000000000, -13.95833333060214976, -2.886751345948128211 ) ) ;
#6128=CARTESIAN_POINT ( 'NONE',  ( 6.123233995736766282E-16, -120.0000000000000000, -5.000000000000000000 ) ) ;
#6129=CARTESIAN_POINT ( 'NONE',  ( -3.152548672688508926E-16, -19.56249999863440081, -5.148502694627439702 ) ) ;
#6133=CARTESIAN_POINT ( 'NONE',  ( -5.000000000000000000, -45.87499999726880873, 0.000000000000000000 ) ) ;
#6134=CARTESIAN_POINT ( 'NONE',  ( -6.972266317189433020E-16, 20.87500000273118062, -5.000000000000000000 ) ) ;
#6135=CARTESIAN_POINT ( 'NONE',  ( 2.229367062499998831, 15.35416666803225993, -3.861377020970580887 ) ) ;
#6139=CARTESIAN_POINT ( 'NONE',  ( -4.458734124999999437, -67.39583333196773651, -2.574251347313719407 ) ) ;
#6142=CARTESIAN_POINT ( 'NONE',  ( 5.000000000000000888, 2.416666666666667851, 2.886751345948126879 ) ) ;
#6144=CARTESIAN_POINT ( 'NONE',  ( -5.000000000000000000, 21.91666666666666785, -2.886751345948128211 ) ) ;
#6145=CARTESIAN_POINT ( 'NONE',  ( 2.229367062499998831, -59.64583333196774362, -3.861377020970580887 ) ) ;
#6146=CARTESIAN_POINT ( 'NONE',  ( 5.000000000000000888, -95.45833333060213022, 2.886751345948126879 ) ) ;
#6147=CARTESIAN_POINT ( 'NONE',  ( 4.458734125000000326, -34.89583333196772941, 2.574251347313718519 ) ) ;
#6148=CARTESIAN_POINT ( 'NONE',  ( -4.999999999999998224, -41.79166666393548013, 2.886751345948131764 ) ) ;
#6149=CARTESIAN_POINT ( 'NONE',  ( 1.339745962155616255, 25.83034180399265622, -4.999999999999997335 ) ) ;
#6151=CARTESIAN_POINT ( 'NONE',  ( -6.972266317189433020E-16, -18.12499999726881228, -5.000000000000000000 ) ) ;
#6153=CARTESIAN_POINT ( 'NONE',  ( 5.000000000000000888, -43.58333333333333570, 2.886751345948126879 ) ) ;
#6154=CARTESIAN_POINT ( 'NONE',  ( -5.000000000000000000, 19.00000000000000000, 0.000000000000000000 ) ) ;
#6155=CARTESIAN_POINT ( 'NONE',  ( 1.339745962155615144, -86.58034179853028434, 4.999999999999999112 ) ) ;
#6157=CARTESIAN_POINT ( 'NONE',  ( 4.458734124999999437, -104.8124999986344079, -5.460374474430324690E-16 ) ) ;
#6158=CARTESIAN_POINT ( 'NONE',  ( 2.229367062499998831, 2.104166668032262599, -3.861377020970580887 ) ) ;
#6161=VECTOR ( 'NONE', #8598, 1000.000000000000000 ) ;
#6165=VERTEX_POINT ( 'NONE', #34379 ) ;
#6166=CARTESIAN_POINT ( 'NONE',  ( -6.972266317189433020E-16, -33.24999999999999289, -5.000000000000000000 ) ) ;
#6169=ORIENTED_EDGE ( 'NONE', *, *, #35440, .T. ) ;
#6172=CARTESIAN_POINT ( 'NONE',  ( -4.458734124999999437, -32.56249999863440792, 0.000000000000000000 ) ) ;
#6173=LINE ( 'NONE', #59898, #18364 ) ;
#6177=EDGE_CURVE ( 'NONE', #19698, #15898, #32346, .T. ) ;
#6181=( BOUNDED_CURVE ( )  B_SPLINE_CURVE ( 2, ( #50341, #25577, #15611, #20438, #24941, #35229, #30067, #30391, #60002 ),
 .UNSPECIFIED., .F., .F. ) 
 B_SPLINE_CURVE_WITH_KNOTS ( ( 3, 2, 2, 2, 3 ),
 ( 0.6767857142857143238, 0.6773809523809524169, 0.6785714285714286031, 0.6797619047619047894, 0.6803571428571428825 ),
 .UNSPECIFIED. ) 
 CURVE ( )  GEOMETRIC_REPRESENTATION_ITEM ( )  RATIONAL_B_SPLINE_CURVE ( ( 0.9330127018922194093, 0.9330127018922194093, 1.000000000000000000, 0.8660254037844387076, 1.000000000000000000, 0.8660254037844387076, 1.000000000000000000, 0.9330127018922194093, 0.9330127018922194093 ) ) 
 REPRESENTATION_ITEM ( '' )  );
#6182=ORIENTED_EDGE ( 'NONE', *, *, #11770, .T. ) ;
#6183=CARTESIAN_POINT ( 'NONE',  ( 8.660254037844342889, 45.00000000000000000, 0.000000000000000000 ) ) ;
#6185=CARTESIAN_POINT ( 'NONE',  ( -4.458734124999999437, -76.64583333196775072, -2.574251347313719407 ) ) ;
#6188=CYLINDRICAL_SURFACE ( 'NONE', #1883, 5.000000000000000000 ) ;
#6191=CARTESIAN_POINT ( 'NONE',  ( -4.458734124999999437, -3.562499998634407916, 0.000000000000000000 ) ) ;
#6192=ORIENTED_EDGE ( 'NONE', *, *, #29090, .T. ) ;
#6199=EDGE_LOOP ( 'NONE', ( #49567, #694, #63153, #44672 ) ) ;
#6200=CARTESIAN_POINT ( 'NONE',  ( 9.457646018065525792E-16, -80.06249999863440792, 5.148502694627439702 ) ) ;
#6202=CARTESIAN_POINT ( 'NONE',  ( -4.458734124999998549, -1.229166665301071326, 2.574251347313722516 ) ) ;
#6206=CARTESIAN_POINT ( 'NONE',  ( 9.457646018065525792E-16, -68.31249999863442213, 5.148502694627439702 ) ) ;
#6207=CARTESIAN_POINT ( 'NONE',  ( 5.000000000000000000, -33.29166666393547303, -2.886751345948129988 ) ) ;
#6209=CARTESIAN_POINT ( 'NONE',  ( -2.229367062500000163, 29.52083333469892779, -3.861377020970580443 ) ) ;
#6212=CARTESIAN_POINT ( 'NONE',  ( -4.458734124999999437, -51.39583333196772941, -2.574251347313719407 ) ) ;
#6213=CARTESIAN_POINT ( 'NONE',  ( 4.458734124999999437, -33.06249999863440792, -5.460374474430324690E-16 ) ) ;
#6216=CARTESIAN_POINT ( 'NONE',  ( -2.499999999999996447, 21.16666666666666785, 4.330127018922195425 ) ) ;
#6218=FACE_OUTER_BOUND ( 'NONE', #42278, .T. ) ;
#6219=CARTESIAN_POINT ( 'NONE',  ( -4.458734124999999437, -41.31249999863440081, 0.000000000000000000 ) ) ;
#6220=CARTESIAN_POINT ( 'NONE',  ( -4.999999999999999112, -78.79166666393547303, 2.886751345948131764 ) ) ;
#6224=CARTESIAN_POINT ( 'NONE',  ( -4.458734124999999437, -79.64583333196773651, -2.574251347313719407 ) ) ;
#6229=CARTESIAN_POINT ( 'NONE',  ( -4.999999999999999112, -24.91666666666666075, 2.886751345948131764 ) ) ;
#6235=( BOUNDED_CURVE ( )  B_SPLINE_CURVE ( 2, ( #22534, #8669, #63031, #42130, #62084, #18000, #13507, #3852, #48214 ),
 .UNSPECIFIED., .F., .F. ) 
 B_SPLINE_CURVE_WITH_KNOTS ( ( 3, 2, 2, 2, 3 ),
 ( 0.5089285714285713969, 0.5095238095238094900, 0.5107142857142856762, 0.5119047619047618625, 0.5124999999999999556 ),
 .UNSPECIFIED. ) 
 CURVE ( )  GEOMETRIC_REPRESENTATION_ITEM ( )  RATIONAL_B_SPLINE_CURVE ( ( 0.9330127018922194093, 0.9330127018922194093, 1.000000000000000000, 0.8660254037844387076, 1.000000000000000000, 0.8660254037844387076, 1.000000000000000000, 0.9330127018922194093, 0.9330127018922194093 ) ) 
 REPRESENTATION_ITEM ( '' )  );
#6236=CARTESIAN_POINT ( 'NONE',  ( -3.535250795749689387E-16, 20.87500000273118417, -5.773502691896257311 ) ) ;
#6242=CARTESIAN_POINT ( 'NONE',  ( 5.000000000000000888, -99.45833333060214443, 2.886751345948126879 ) ) ;
#6248=CARTESIAN_POINT ( 'NONE',  ( 9.457646018065525792E-16, -12.31249999863440259, 5.148502694627439702 ) ) ;
#6254=ADVANCED_FACE ( 'NONE', ( #50474 ), #10900, .T. ) ;
#6256=VERTEX_POINT ( 'NONE', #31156 ) ;
#6257=CARTESIAN_POINT ( 'NONE',  ( -6.972266317189433020E-16, 13.74999999999999822, -5.000000000000000000 ) ) ;
#6261=CARTESIAN_POINT ( 'NONE',  ( -1.339745962155613812, -28.20534180126147916, -5.000000000000000000 ) ) ;
#6266=CARTESIAN_POINT ( 'NONE',  ( -1.339745962155610925, -7.669658196007332229, 5.000000000000000000 ) ) ;
#6270=EDGE_LOOP ( 'NONE', ( #20058, #30046, #61888, #24145 ) ) ;
#6273=CARTESIAN_POINT ( 'NONE',  ( 4.458734125000001214, 15.10416666803225993, 2.574251347313718519 ) ) ;
#6276=DIRECTION ( 'NONE',  ( -0.000000000000000000, 1.000000000000000000, -0.000000000000000000 ) ) ;
#6277=CARTESIAN_POINT ( 'NONE',  ( 5.000000000000000000, -25.41666666666666430, -2.886751345948130876 ) ) ;
#6278=( BOUNDED_CURVE ( )  B_SPLINE_CURVE ( 2, ( #59878, #15799, #35739, #25120, #50205, #20634, #49566, #6155, #45705 ),
 .UNSPECIFIED., .F., .F. ) 
 B_SPLINE_CURVE_WITH_KNOTS ( ( 3, 2, 2, 2, 3 ),
 ( 0.8232142857142856762, 0.8238095238095237693, 0.8249999999999999556, 0.8261904761904761418, 0.8267857142857142350 ),
 .UNSPECIFIED. ) 
 CURVE ( )  GEOMETRIC_REPRESENTATION_ITEM ( )  RATIONAL_B_SPLINE_CURVE ( ( 0.9330127018922194093, 0.9330127018922194093, 1.000000000000000000, 0.8660254037844387076, 1.000000000000000000, 0.8660254037844387076, 1.000000000000000000, 0.9330127018922194093, 0.9330127018922194093 ) ) 
 REPRESENTATION_ITEM ( '' )  );
#6279=CARTESIAN_POINT ( 'NONE',  ( -4.458734124999999437, -65.31249999863440792, 0.000000000000000000 ) ) ;
#6281=CARTESIAN_POINT ( 'NONE',  ( 2.229367062500001939, 15.02083333469892779, 3.861377020970579999 ) ) ;
#6285=CARTESIAN_POINT ( 'NONE',  ( 4.458734124999998549, -55.97916666530107932, -2.574251347313721627 ) ) ;
#6286=CARTESIAN_POINT ( 'NONE',  ( 1.060575238724906964E-15, -13.62499999726881050, 5.773502691896257311 ) ) ;
#6287=CARTESIAN_POINT ( 'NONE',  ( -4.999999999999998224, -108.9166666666666572, 2.886751345948131764 ) ) ;
#6289=DIRECTION ( 'NONE',  ( -0.000000000000000000, 1.000000000000000000, -0.000000000000000000 ) ) ;
#6291=CARTESIAN_POINT ( 'NONE',  ( 4.458734124999998549, -16.97916666530107577, -2.574251347313721627 ) ) ;
#6293=CARTESIAN_POINT ( 'NONE',  ( -6.972266317189433020E-16, 23.75000000000000000, -5.000000000000000000 ) ) ;
#6294=CARTESIAN_POINT ( 'NONE',  ( -4.458734124999998549, -103.2291666653010509, 2.574251347313722516 ) ) ;
#6297=CARTESIAN_POINT ( 'NONE',  ( 9.457646018065525792E-16, -105.3124999986344221, 5.148502694627439702 ) ) ;
#6298=CARTESIAN_POINT ( 'NONE',  ( -2.229367062500000163, -24.47916666530106866, -3.861377020970580443 ) ) ;
#6299=CARTESIAN_POINT ( 'NONE',  ( 2.499999999999998668, -56.20833333060214443, -4.330127018922193649 ) ) ;
#6303=CARTESIAN_POINT ( 'NONE',  ( -4.458734124999999437, -21.31249999863440436, 0.000000000000000000 ) ) ;
#6304=CARTESIAN_POINT ( 'NONE',  ( -3.152548672688508926E-16, -64.81249999863440792, -5.148502694627439702 ) ) ;
#6305=PLANE ( 'NONE',  #50048 ) ;
#6307=DIRECTION ( 'NONE',  ( 0.000000000000000000, 0.000000000000000000, 1.000000000000000000 ) ) ;
#6309=CARTESIAN_POINT ( 'NONE',  ( 2.499999999999998668, -12.33333333333333570, -4.330127018922193649 ) ) ;
#6314=CARTESIAN_POINT ( 'NONE',  ( 1.339745962155615144, -90.70534180126146850, 4.999999999999999112 ) ) ;
#6317=CARTESIAN_POINT ( 'NONE',  ( -6.972266317189433020E-16, 1.875000002731185722, -5.000000000000000000 ) ) ;
#6319=CARTESIAN_POINT ( 'NONE',  ( 1.339745962155615144, 20.41965820146970501, 4.999999999999999112 ) ) ;
#6321=CARTESIAN_POINT ( 'NONE',  ( 1.060575238724906964E-15, -79.74999999999998579, 5.773502691896257311 ) ) ;
#6324=CARTESIAN_POINT ( 'NONE',  ( -5.000000000000000000, -98.00000000000000000, 0.000000000000000000 ) ) ;
#6325=ORIENTED_EDGE ( 'NONE', *, *, #26107, .F. ) ;
#6326=CARTESIAN_POINT ( 'NONE',  ( -5.000000000000000000, -53.87499999726880162, 0.000000000000000000 ) ) ;
#6331=EDGE_CURVE ( 'NONE', #3031, #48295, #35677, .T. ) ;
#6339=VERTEX_POINT ( 'NONE', #55933 ) ;
#6345=ORIENTED_EDGE ( 'NONE', *, *, #52295, .T. ) ;
#6347=CARTESIAN_POINT ( 'NONE',  ( -4.458734124999998549, -78.22916666530106511, 2.574251347313722516 ) ) ;
#6349=CARTESIAN_POINT ( 'NONE',  ( 4.458734124999998549, -108.9791666653010651, -2.574251347313721627 ) ) ;
#6352=FACE_OUTER_BOUND ( 'NONE', #5519, .T. ) ;
#6356=CARTESIAN_POINT ( 'NONE',  ( -2.229367062500000163, -41.47916666530107932, -3.861377020970580443 ) ) ;
#6359=CARTESIAN_POINT ( 'NONE',  ( 4.458734125000000326, -51.89583333196773651, 2.574251347313718519 ) ) ;
#6362=CARTESIAN_POINT ( 'NONE',  ( 2.229367062500001939, -16.97916666530106866, 3.861377020970579999 ) ) ;
#6364=CARTESIAN_POINT ( 'NONE',  ( -2.500000000000000444, -99.16666666666665719, -4.330127018922193649 ) ) ;
#6366=CARTESIAN_POINT ( 'NONE',  ( -2.229367062500000163, -36.72916666530107221, -3.861377020970580443 ) ) ;
#6367=CARTESIAN_POINT ( 'NONE',  ( 5.000000000000000000, 6.625000002731185944, -6.123233995736766282E-16 ) ) ;
#6370=CYLINDRICAL_SURFACE ( 'NONE', #50747, 5.000000000000000000 ) ;
#6372=CARTESIAN_POINT ( 'NONE',  ( 2.229367062500001939, 1.770833334698927786, 3.861377020970579999 ) ) ;
#6374=CARTESIAN_POINT ( 'NONE',  ( 2.499999999999998668, 24.79166666939785202, -4.330127018922193649 ) ) ;
#6376=CARTESIAN_POINT ( 'NONE',  ( -4.458734124999999437, -87.31249999863439371, 0.000000000000000000 ) ) ;
#6377=CARTESIAN_POINT ( 'NONE',  ( -2.229367062500000163, -37.47916666530107221, -3.861377020970580443 ) ) ;
#6378=FACE_OUTER_BOUND ( 'NONE', #1014, .T. ) ;
#6379=CARTESIAN_POINT ( 'NONE',  ( -4.458734124999999437, -80.56249999863440792, 0.000000000000000000 ) ) ;
#6381=CARTESIAN_POINT ( 'NONE',  ( 1.975475456537005874E-15, -49.74999999999999289, 5.000000000000000000 ) ) ;
#6383=( BOUNDED_CURVE ( )  B_SPLINE_CURVE ( 2, ( #36773, #8454, #17780, #32251, #37399, #32573, #52194, #56404, #57351 ),
 .UNSPECIFIED., .F., .F. ) 
 B_SPLINE_CURVE_WITH_KNOTS ( ( 3, 2, 2, 2, 3 ),
 ( 0.4124999999999999778, 0.4130952380952380709, 0.4142857142857143127, 0.4154761904761904989, 0.4160714285714285920 ),
 .UNSPECIFIED. ) 
 CURVE ( )  GEOMETRIC_REPRESENTATION_ITEM ( )  RATIONAL_B_SPLINE_CURVE ( ( 0.9330127018922194093, 0.9330127018922194093, 1.000000000000000000, 0.8660254037844387076, 1.000000000000000000, 0.8660254037844387076, 1.000000000000000000, 0.9330127018922194093, 0.9330127018922194093 ) ) 
 REPRESENTATION_ITEM ( '' )  );
#6384=CARTESIAN_POINT ( 'NONE',  ( 9.457646018065525792E-16, -10.06249999863440614, 5.148502694627439702 ) ) ;
#6385=CARTESIAN_POINT ( 'NONE',  ( -4.458734124999999437, 19.43750000136559208, 0.000000000000000000 ) ) ;
#6386=CARTESIAN_POINT ( 'NONE',  ( 4.458734125000000326, -47.14583333196774362, 2.574251347313718519 ) ) ;
#6387=CARTESIAN_POINT ( 'NONE',  ( 1.339745962155615144, -105.7053418012614685, 4.999999999999999112 ) ) ;
#6394=CARTESIAN_POINT ( 'NONE',  ( 4.458734125000001214, -74.89583333196773651, 2.574251347313718519 ) ) ;
#6395=CARTESIAN_POINT ( 'NONE',  ( 9.457646018065525792E-16, 27.68750000136559208, 5.148502694627439702 ) ) ;
#6400=CARTESIAN_POINT ( 'NONE',  ( -5.000000000000000000, -62.08333333333332860, -2.886751345948128211 ) ) ;
#6401=CARTESIAN_POINT ( 'NONE',  ( 1.339745962155612702, -90.16965819600733312, -5.000000000000000000 ) ) ;
#6412=ORIENTED_EDGE ( 'NONE', *, *, #48712, .T. ) ;
#6420=CARTESIAN_POINT ( 'NONE',  ( 4.458734125000001214, -48.14583333196773651, 2.574251347313718519 ) ) ;
#6426=CARTESIAN_POINT ( 'NONE',  ( -5.000000000000000000, 1.000000000000000888, 0.000000000000000000 ) ) ;
#6428=CARTESIAN_POINT ( 'NONE',  ( -2.229367062499996610, -93.39583333196773651, 3.861377020970582219 ) ) ;
#6430=VERTEX_POINT ( 'NONE', #15296 ) ;
#6437=CARTESIAN_POINT ( 'NONE',  ( -6.972266317189433020E-16, -63.25000000000000000, -5.000000000000000000 ) ) ;
#6438=EDGE_LOOP ( 'NONE', ( #8572, #17535, #31971, #23025 ) ) ;
#6439=CARTESIAN_POINT ( 'NONE',  ( -2.229367062500000163, -2.479166665301069106, -3.861377020970580443 ) ) ;
#6440=EDGE_CURVE ( 'NONE', #14985, #43493, #63560, .T. ) ;
#6441=CARTESIAN_POINT ( 'NONE',  ( 5.000000000000000000, -1.374999997268814500, -6.123233995736766282E-16 ) ) ;
#6442=CARTESIAN_POINT ( 'NONE',  ( 4.458734125000001214, -18.14583333196773651, 2.574251347313718519 ) ) ;
#6447=CARTESIAN_POINT ( 'NONE',  ( 4.458734124999998549, 15.02083333469892779, -2.574251347313721627 ) ) ;
#6448=ORIENTED_EDGE ( 'NONE', *, *, #8391, .T. ) ;
#6451=CARTESIAN_POINT ( 'NONE',  ( 2.229367062500001939, -18.97916666530106866, 3.861377020970579999 ) ) ;
#6452=DIRECTION ( 'NONE',  ( -0.000000000000000000, 1.000000000000000000, -0.000000000000000000 ) ) ;
#6455=CARTESIAN_POINT ( 'NONE',  ( 5.000000000000000888, -45.45833333060214443, 2.886751345948126879 ) ) ;
#6456=CARTESIAN_POINT ( 'NONE',  ( 5.000000000000000000, -67.37499999726881583, -6.123233995736766282E-16 ) ) ;
#6457=CARTESIAN_POINT ( 'NONE',  ( -4.458734124999999437, 7.687500001365594748, 0.000000000000000000 ) ) ;
#6459=DIRECTION ( 'NONE',  ( 0.000000000000000000, 0.000000000000000000, 1.000000000000000000 ) ) ;
#6461=CARTESIAN_POINT ( 'NONE',  ( -3.152548672688508926E-16, -67.56249999863440792, -5.148502694627439702 ) ) ;
#6463=( BOUNDED_CURVE ( )  B_SPLINE_CURVE ( 2, ( #22984, #12050, #37146, #56770, #51932, #37770, #57401, #22031, #57084 ),
 .UNSPECIFIED., .F., .F. ) 
 B_SPLINE_CURVE_WITH_KNOTS ( ( 3, 2, 2, 2, 3 ),
 ( 0.8053571428571428825, 0.8059523809523809756, 0.8071428571428571619, 0.8083333333333333481, 0.8089285714285714413 ),
 .UNSPECIFIED. ) 
 CURVE ( )  GEOMETRIC_REPRESENTATION_ITEM ( )  RATIONAL_B_SPLINE_CURVE ( ( 0.9330127018922194093, 0.9330127018922194093, 1.000000000000000000, 0.8660254037844387076, 1.000000000000000000, 0.8660254037844387076, 1.000000000000000000, 0.9330127018922194093, 0.9330127018922194093 ) ) 
 REPRESENTATION_ITEM ( '' )  );
#6464=CARTESIAN_POINT ( 'NONE',  ( -5.000000000000000000, 4.916666666666666075, -2.886751345948128211 ) ) ;
#6466=CARTESIAN_POINT ( 'NONE',  ( -4.999999999999998224, 22.08333333333333215, 2.886751345948131764 ) ) ;
#6467=CARTESIAN_POINT ( 'NONE',  ( 4.458734124999999437, -56.81249999863440081, -5.460374474430324690E-16 ) ) ;
#6468=CARTESIAN_POINT ( 'NONE',  ( -2.499999999999996447, -95.70833333060213022, 4.330127018922195425 ) ) ;
#6470=CARTESIAN_POINT ( 'NONE',  ( -5.000000000000000000, -80.08333333333332860, -2.886751345948128211 ) ) ;
#6471=DIRECTION ( 'NONE',  ( 0.000000000000000000, 0.000000000000000000, 1.000000000000000000 ) ) ;
#6474=CARTESIAN_POINT ( 'NONE',  ( 1.060575238724906964E-15, -41.74999999999999289, 5.773502691896257311 ) ) ;
#6476=DIRECTION ( 'NONE',  ( -0.000000000000000000, 1.000000000000000000, -0.000000000000000000 ) ) ;
#6477=ORIENTED_EDGE ( 'NONE', *, *, #36714, .F. ) ;
#6478=CARTESIAN_POINT ( 'NONE',  ( -2.229367062500000163, -104.4791666653010651, -3.861377020970580443 ) ) ;
#6479=CARTESIAN_POINT ( 'NONE',  ( -2.229367062499996610, -2.395833331967737845, 3.861377020970582219 ) ) ;
#6480=FACE_OUTER_BOUND ( 'NONE', #27499, .T. ) ;
#6486=ORIENTED_EDGE ( 'NONE', *, *, #58534, .T. ) ;
#6487=CARTESIAN_POINT ( 'NONE',  ( 5.000000000000000888, -22.45833333060214443, 2.886751345948126879 ) ) ;
#6490=DIRECTION ( 'NONE',  ( -0.000000000000000000, 1.000000000000000000, -0.000000000000000000 ) ) ;
#6492=CARTESIAN_POINT ( 'NONE',  ( 4.458734124999999437, -29.06249999863440436, -5.460374474430324690E-16 ) ) ;
#6493=DIRECTION ( 'NONE',  ( -0.000000000000000000, 1.000000000000000000, -0.000000000000000000 ) ) ;
#6499=ORIENTED_EDGE ( 'NONE', *, *, #23952, .T. ) ;
#6500=CARTESIAN_POINT ( 'NONE',  ( 2.499999999999998668, -70.20833333060214443, -4.330127018922193649 ) ) ;
#6502=CARTESIAN_POINT ( 'NONE',  ( -2.229367062499996610, -79.39583333196773651, 3.861377020970582219 ) ) ;
#6505=DIRECTION ( 'NONE',  ( -0.000000000000000000, 1.000000000000000000, -0.000000000000000000 ) ) ;
#6508=CARTESIAN_POINT ( 'NONE',  ( 9.457646018065525792E-16, -5.312499998634402587, 5.148502694627439702 ) ) ;
#6509=ORIENTED_EDGE ( 'NONE', *, *, #18968, .F. ) ;
#6511=DIRECTION ( 'NONE',  ( -0.000000000000000000, 1.000000000000000000, -0.000000000000000000 ) ) ;
#6512=ORIENTED_EDGE ( 'NONE', *, *, #41590, .T. ) ;
#6513=CARTESIAN_POINT ( 'NONE',  ( 2.499999999999998668, -91.33333333333334281, -4.330127018922193649 ) ) ;
#6519=CARTESIAN_POINT ( 'NONE',  ( -4.458734124999997661, -83.22916666530106511, 2.574251347313722516 ) ) ;
#6521=CARTESIAN_POINT ( 'NONE',  ( 4.458734124999999437, -3.812499998634408360, -5.460374474430324690E-16 ) ) ;
#6524=CARTESIAN_POINT ( 'NONE',  ( -2.499999999999996447, -30.70833333060214443, 4.330127018922195425 ) ) ;
#6525=CARTESIAN_POINT ( 'NONE',  ( 2.229367062500001939, 24.02083333469892779, 3.861377020970579999 ) ) ;
#6526=CARTESIAN_POINT ( 'NONE',  ( 1.339745962155612702, -104.2946581987385315, -5.000000000000000000 ) ) ;
#6527=CARTESIAN_POINT ( 'NONE',  ( 2.229367062499998831, -53.64583333196773651, -3.861377020970580887 ) ) ;
#6528=CARTESIAN_POINT ( 'NONE',  ( -2.229367062499996610, -36.39583333196773651, 3.861377020970582219 ) ) ;
#6530=CARTESIAN_POINT ( 'NONE',  ( -4.999999999999998224, -17.91666666666666430, 2.886751345948131764 ) ) ;
#6531=CARTESIAN_POINT ( 'NONE',  ( -5.000000000000000000, 22.00000000000000000, 0.000000000000000000 ) ) ;
#6534=CARTESIAN_POINT ( 'NONE',  ( 2.229367062499998831, -43.64583333196773651, -3.861377020970580887 ) ) ;
#6535=CARTESIAN_POINT ( 'NONE',  ( 5.000000000000000000, -76.29166666393547303, -2.886751345948129988 ) ) ;
#6540=CARTESIAN_POINT ( 'NONE',  ( 2.229367062499998831, -80.89583333196773651, -3.861377020970580887 ) ) ;
#6542=CARTESIAN_POINT ( 'NONE',  ( 1.060575238724906964E-15, -27.74999999999999645, 5.773502691896257311 ) ) ;
#6547=CARTESIAN_POINT ( 'NONE',  ( 4.458734124999998549, 13.02083333469892779, -2.574251347313721627 ) ) ;
#6548=CARTESIAN_POINT ( 'NONE',  ( 5.000000000000000000, 16.62500000273118417, -6.123233995736766282E-16 ) ) ;
#6549=CARTESIAN_POINT ( 'NONE',  ( -2.480964764533239819E-13, -60.62499999726880873, 5.000000000000000000 ) ) ;
#6555=CARTESIAN_POINT ( 'NONE',  ( 1.975475456537005874E-15, -109.7499999999999858, 5.000000000000000000 ) ) ;
#6556=CYLINDRICAL_SURFACE ( 'NONE', #11753, 5.000000000000000000 ) ;
#6561=CARTESIAN_POINT ( 'NONE',  ( 4.458734125000001214, -13.14583333196774184, 2.574251347313718519 ) ) ;
#6562=CARTESIAN_POINT ( 'NONE',  ( 2.499999999999998668, 17.79166666939785557, -4.330127018922193649 ) ) ;
#6569=ORIENTED_EDGE ( 'NONE', *, *, #40160, .T. ) ;
#6570=CARTESIAN_POINT ( 'NONE',  ( -4.999999999999998224, 25.20833333606451987, 2.886751345948131764 ) ) ;
#6573=CARTESIAN_POINT ( 'NONE',  ( 5.000000000000000000, -103.5000000000000142, -6.123233995736766282E-16 ) ) ;
#6575=VERTEX_POINT ( 'NONE', #29755 ) ;
#6578=CARTESIAN_POINT ( 'NONE',  ( 0.000000000000000000, -120.0000000000000000, 0.000000000000000000 ) ) ;
#6582=CARTESIAN_POINT ( 'NONE',  ( -4.458734124999999437, 14.60416666803226171, -2.574251347313719407 ) ) ;
#6585=CARTESIAN_POINT ( 'NONE',  ( -1.339745962155613812, -24.08034179853029499, -5.000000000000000000 ) ) ;
#6588=CARTESIAN_POINT ( 'NONE',  ( -4.458734124999997661, -65.22916666530106511, 2.574251347313722516 ) ) ;
#6589=CARTESIAN_POINT ( 'NONE',  ( -6.972266317189433020E-16, -19.12499999726880873, -5.000000000000000000 ) ) ;
#6590=CARTESIAN_POINT ( 'NONE',  ( 4.458734124999999437, 15.18750000136559564, -5.460374474430324690E-16 ) ) ;
#6593=CARTESIAN_POINT ( 'NONE',  ( -2.229367062500000163, -52.72916666530107221, -3.861377020970580443 ) ) ;
#6594=CARTESIAN_POINT ( 'NONE',  ( 5.000000000000000888, -16.45833333060214443, 2.886751345948126879 ) ) ;
#6595=CARTESIAN_POINT ( 'NONE',  ( 0.000000000000000000, -120.0000000000000000, 0.000000000000000000 ) ) ;
#6598=CARTESIAN_POINT ( 'NONE',  ( 1.339745962155612702, -64.16965819600731891, -5.000000000000000000 ) ) ;
#6599=CARTESIAN_POINT ( 'NONE',  ( -4.458734124999997661, -15.47916666530107399, 2.574251347313722516 ) ) ;
#6601=VERTEX_POINT ( 'NONE', #34265 ) ;
#6602=CARTESIAN_POINT ( 'NONE',  ( -1.339745962155610925, -60.79465819873851729, 5.000000000000000000 ) ) ;
#6603=CARTESIAN_POINT ( 'NONE',  ( 4.458734124999999437, -105.8124999986344221, -5.460374474430324690E-16 ) ) ;
#6606=CARTESIAN_POINT ( 'NONE',  ( -2.229367062499996610, -103.3958333319677365, 3.861377020970582219 ) ) ;
#6607=ADVANCED_FACE ( 'NONE', ( #199 ), #9510, .T. ) ;
#6608=CARTESIAN_POINT ( 'NONE',  ( 4.458734125000001214, -28.89583333196774007, 2.574251347313718519 ) ) ;
#6609=CARTESIAN_POINT ( 'NONE',  ( -2.500000000000000444, -62.04166666393547303, -4.330127018922193649 ) ) ;
#6612=CARTESIAN_POINT ( 'NONE',  ( -4.458734124999997661, -24.22916666530107577, 2.574251347313722516 ) ) ;
#6613=CARTESIAN_POINT ( 'NONE',  ( 2.229367062500001939, -65.22916666530106511, 3.861377020970579999 ) ) ;
#6616=DIRECTION ( 'NONE',  ( 0.000000000000000000, 0.000000000000000000, 1.000000000000000000 ) ) ;
#6618=CARTESIAN_POINT ( 'NONE',  ( -3.535250795749689387E-16, -12.24999999999999645, -5.773502691896257311 ) ) ;
#6620=ORIENTED_EDGE ( 'NONE', *, *, #63624, .F. ) ;
#6622=CARTESIAN_POINT ( 'NONE',  ( 2.500000000000002220, 21.45833333606451987, 4.330127018922192761 ) ) ;
#6627=EDGE_CURVE ( 'NONE', #61600, #26190, #59691, .T. ) ;
#6629=EDGE_CURVE ( 'NONE', #4186, #12980, #4904, .T. ) ;
#6633=CARTESIAN_POINT ( 'NONE',  ( -5.000000000000000000, -80.00000000000000000, 0.000000000000000000 ) ) ;
#6637=ORIENTED_EDGE ( 'NONE', *, *, #2863, .T. ) ;
#6648=( BOUNDED_CURVE ( )  B_SPLINE_CURVE ( 2, ( #13559, #41541, #47338, #41866, #61193, #61513, #17442, #37060, #22590 ),
 .UNSPECIFIED., .F., .F. ) 
 B_SPLINE_CURVE_WITH_KNOTS ( ( 3, 2, 2, 2, 3 ),
 ( 0.7696428571428571841, 0.7702380952380952772, 0.7714285714285714635, 0.7726190476190476497, 0.7732142857142857428 ),
 .UNSPECIFIED. ) 
 CURVE ( )  GEOMETRIC_REPRESENTATION_ITEM ( )  RATIONAL_B_SPLINE_CURVE ( ( 0.9330127018922194093, 0.9330127018922194093, 1.000000000000000000, 0.8660254037844387076, 1.000000000000000000, 0.8660254037844387076, 1.000000000000000000, 0.9330127018922194093, 0.9330127018922194093 ) ) 
 REPRESENTATION_ITEM ( '' )  );
#6650=CARTESIAN_POINT ( 'NONE',  ( 1.975475456537005874E-15, -75.74999999999998579, 5.000000000000000000 ) ) ;
#6651=VERTEX_POINT ( 'NONE', #48034 ) ;
#6655=ORIENTED_EDGE ( 'NONE', *, *, #2082, .F. ) ;
#6657=CARTESIAN_POINT ( 'NONE',  ( 4.458734124999998549, -75.72916666530106511, -2.574251347313721627 ) ) ;
#6658=CARTESIAN_POINT ( 'NONE',  ( -4.458734124999999437, -110.5624999986343937, 0.000000000000000000 ) ) ;
#6659=CARTESIAN_POINT ( 'NONE',  ( 5.000000000000000000, -18.50000000000000355, -6.123233995736766282E-16 ) ) ;
#6665=CARTESIAN_POINT ( 'NONE',  ( -3.152548672688508926E-16, -45.56249999863439371, -5.148502694627439702 ) ) ;
#6668=CARTESIAN_POINT ( 'NONE',  ( 9.457646018065525792E-16, -48.06249999863440792, 5.148502694627439702 ) ) ;
#6670=CARTESIAN_POINT ( 'NONE',  ( 4.458734124999998549, 29.27083333469892423, -2.574251347313721627 ) ) ;
#6671=CARTESIAN_POINT ( 'NONE',  ( -4.999999999999999112, -103.9166666666666430, 2.886751345948131764 ) ) ;
#6674=CARTESIAN_POINT ( 'NONE',  ( 2.229367062500001939, -37.22916666530107221, 3.861377020970579999 ) ) ;
#6675=CARTESIAN_POINT ( 'NONE',  ( 5.000000000000000000, -0.2916666639354824619, -2.886751345948129988 ) ) ;
#6676=LINE ( 'NONE', #34663, #50977 ) ;
#6680=CARTESIAN_POINT ( 'NONE',  ( -3.152548672688508926E-16, -95.56249999863439371, -5.148502694627439702 ) ) ;
#6682=CARTESIAN_POINT ( 'NONE',  ( 2.229367062499998831, 2.104166668032262599, -3.861377020970580887 ) ) ;
#6683=ORIENTED_EDGE ( 'NONE', *, *, #39433, .F. ) ;
#6684=CARTESIAN_POINT ( 'NONE',  ( 1.339745962155612702, 24.83034180399266333, -5.000000000000000000 ) ) ;
#6686=CARTESIAN_POINT ( 'NONE',  ( -3.152548672688508926E-16, -87.56249999863440792, -5.148502694627439702 ) ) ;
#6688=CARTESIAN_POINT ( 'NONE',  ( -2.229367062500000163, -87.72916666530107932, -3.861377020970580443 ) ) ;
#6693=EDGE_CURVE ( 'NONE', #35135, #9375, #28418, .T. ) ;
#6694=CARTESIAN_POINT ( 'NONE',  ( -3.152548672688508926E-16, -6.562499998634404363, -5.148502694627439702 ) ) ;
#6695=CARTESIAN_POINT ( 'NONE',  ( 4.458734124999998549, 16.02083333469892423, -2.574251347313721627 ) ) ;
#6696=CARTESIAN_POINT ( 'NONE',  ( 4.458734124999998549, -45.97916666530106511, -2.574251347313721627 ) ) ;
#6704=CARTESIAN_POINT ( 'NONE',  ( -4.458734124999998549, -76.22916666530107932, 2.574251347313722516 ) ) ;
#6705=CARTESIAN_POINT ( 'NONE',  ( 2.229367062499998831, 27.10416666803225993, -3.861377020970580887 ) ) ;
#6707=DIRECTION ( 'NONE',  ( -0.000000000000000000, 1.000000000000000000, -0.000000000000000000 ) ) ;
#6711=CARTESIAN_POINT ( 'NONE',  ( -2.500000000000000444, -67.16666666666667140, -4.330127018922193649 ) ) ;
#6712=CARTESIAN_POINT ( 'NONE',  ( 1.975475456537005874E-15, -103.6249999972688016, 5.000000000000000000 ) ) ;
#6715=CARTESIAN_POINT ( 'NONE',  ( -1.339745962155610925, -72.66965819600733312, 5.000000000000000000 ) ) ;
#6716=CARTESIAN_POINT ( 'NONE',  ( -2.499999999999996447, -106.7083333306021444, 4.330127018922195425 ) ) ;
#6723=EDGE_LOOP ( 'NONE', ( #29423, #58239, #51661, #15930 ) ) ;
#6727=VERTEX_POINT ( 'NONE', #14559 ) ;
#6730=CARTESIAN_POINT ( 'NONE',  ( 2.229367062500001939, -45.22916666530106511, 3.861377020970579999 ) ) ;
#6741=CARTESIAN_POINT ( 'NONE',  ( -3.152548672688508926E-16, -92.81249999863439371, -5.148502694627439702 ) ) ;
#6744=CARTESIAN_POINT ( 'NONE',  ( 6.123233995736766282E-16, -120.0000000000000000, -5.000000000000000000 ) ) ;
#6747=DIRECTION ( 'NONE',  ( -0.000000000000000000, 1.000000000000000000, -0.000000000000000000 ) ) ;
#6748=CARTESIAN_POINT ( 'NONE',  ( -2.229367062500000163, -0.4791666653010707710, -3.861377020970580443 ) ) ;
#6749=CARTESIAN_POINT ( 'NONE',  ( 6.123233995736766282E-16, -120.0000000000000000, -5.000000000000000000 ) ) ;
#6750=CARTESIAN_POINT ( 'NONE',  ( 4.458734124999999437, -24.06249999863440436, -5.460374474430324690E-16 ) ) ;
#6752=DIRECTION ( 'NONE',  ( -0.000000000000000000, 1.000000000000000000, -0.000000000000000000 ) ) ;
#6756=CARTESIAN_POINT ( 'NONE',  ( -4.458734124999997661, 15.52083333469892779, 2.574251347313722516 ) ) ;
#6757=ORIENTED_EDGE ( 'NONE', *, *, #44391, .F. ) ;
#6758=LINE ( 'NONE', #26371, #63417 ) ;
#6759=CARTESIAN_POINT ( 'NONE',  ( 5.000000000000000000, -71.29166666393547303, -2.886751345948130876 ) ) ;
#6760=CARTESIAN_POINT ( 'NONE',  ( -3.535250795749689387E-16, -84.24999999999998579, -5.773502691896257311 ) ) ;
#6761=CARTESIAN_POINT ( 'NONE',  ( 9.457646018065525792E-16, -19.06249999863440792, 5.148502694627439702 ) ) ;
#6763=CARTESIAN_POINT ( 'NONE',  ( 1.975475456537005874E-15, -3.750000000000001776, 5.000000000000000000 ) ) ;
#6764=AXIS2_PLACEMENT_3D ( 'NONE', #48268, #9348, #63397 ) ;
#6766=EDGE_CURVE ( 'NONE', #26829, #43493, #2482, .T. ) ;
#6768=CARTESIAN_POINT ( 'NONE',  ( 5.000000000000000000, -46.29166666393547303, -2.886751345948129988 ) ) ;
#6769=CARTESIAN_POINT ( 'NONE',  ( -1.339745962155610925, -1.669658196007333784, 5.000000000000000000 ) ) ;
#6770=CARTESIAN_POINT ( 'NONE',  ( 4.458734125000000326, 11.10416666803225993, 2.574251347313718519 ) ) ;
#6775=CARTESIAN_POINT ( 'NONE',  ( 9.457646018065525792E-16, -69.06249999863439371, 5.148502694627439702 ) ) ;
#6777=EDGE_CURVE ( 'NONE', #13925, #63218, #50045, .T. ) ;
#6778=CARTESIAN_POINT ( 'NONE',  ( 5.000000000000000000, -1.416666666666663188, -2.886751345948129988 ) ) ;
#6780=CARTESIAN_POINT ( 'NONE',  ( 4.458734124999999437, -58.81249999863440081, -5.460374474430324690E-16 ) ) ;
#6781=CARTESIAN_POINT ( 'NONE',  ( -5.000000000000000000, -96.95833333060213022, -2.886751345948128211 ) ) ;
#6785=CYLINDRICAL_SURFACE ( 'NONE', #22423, 5.000000000000000000 ) ;
#6788=CARTESIAN_POINT ( 'NONE',  ( 2.500000000000002220, -49.66666666666666430, 4.330127018922192761 ) ) ;
#6789=CARTESIAN_POINT ( 'NONE',  ( 5.000000000000000000, -13.49999999999999822, -6.123233995736766282E-16 ) ) ;
#6792=ORIENTED_EDGE ( 'NONE', *, *, #48143, .F. ) ;
#6793=CARTESIAN_POINT ( 'NONE',  ( -2.229367062500000163, -105.4791666653010651, -3.861377020970580443 ) ) ;
#6794=CARTESIAN_POINT ( 'NONE',  ( -3.152548672688508926E-16, -1.812499998634406362, -5.148502694627439702 ) ) ;
#6795=DIRECTION ( 'NONE',  ( 0.000000000000000000, 0.000000000000000000, 1.000000000000000000 ) ) ;
#6804=CARTESIAN_POINT ( 'NONE',  ( -5.000000000000000000, -16.95833333060214443, -2.886751345948128211 ) ) ;
#6807=CARTESIAN_POINT ( 'NONE',  ( -1.339745962155610925, -55.66965819600732601, 5.000000000000000000 ) ) ;
#6809=CARTESIAN_POINT ( 'NONE',  ( 9.457646018065525792E-16, -28.31249999863440081, 5.148502694627439702 ) ) ;
#6821=CARTESIAN_POINT ( 'NONE',  ( -4.458734124999998549, -77.47916666530106511, 2.574251347313722516 ) ) ;
#6822=CARTESIAN_POINT ( 'NONE',  ( -2.499999999999996447, 13.29166666939785379, 4.330127018922195425 ) ) ;
#6824=DIRECTION ( 'NONE',  ( -0.000000000000000000, 1.000000000000000000, -0.000000000000000000 ) ) ;
#6827=CARTESIAN_POINT ( 'NONE',  ( 2.229367062499998831, -6.895833331967741842, -3.861377020970580887 ) ) ;
#6829=CARTESIAN_POINT ( 'NONE',  ( -1.975475456537005874E-15, 27.37500000273118417, 5.000000000000000000 ) ) ;
#6830=CARTESIAN_POINT ( 'NONE',  ( -5.000000000000000000, 3.125000002731185944, 0.000000000000000000 ) ) ;
#6832=CARTESIAN_POINT ( 'NONE',  ( 9.457646018065525792E-16, -7.312499998634405252, 5.148502694627439702 ) ) ;
#6839=CARTESIAN_POINT ( 'NONE',  ( -2.229367062499996610, -87.14583333196773651, 3.861377020970582219 ) ) ;
#6841=CARTESIAN_POINT ( 'NONE',  ( 4.458734124999999437, -2.812499998634407472, -5.460374474430324690E-16 ) ) ;
#6842=CARTESIAN_POINT ( 'NONE',  ( 5.000000000000000000, -28.37499999726881228, -6.123233995736766282E-16 ) ) ;
#6844=CARTESIAN_POINT ( 'NONE',  ( 9.457646018065525792E-16, 26.93750000136559564, 5.148502694627439702 ) ) ;
#6845=CARTESIAN_POINT ( 'NONE',  ( 1.464175926609780648E-14, 22.74999999999999645, -5.000000000000000000 ) ) ;
#6847=CARTESIAN_POINT ( 'NONE',  ( 4.458734125000001214, -48.89583333196772941, 2.574251347313718519 ) ) ;
#6848=CARTESIAN_POINT ( 'NONE',  ( -4.458734124999999437, -36.64583333196773651, -2.574251347313719407 ) ) ;
#6850=CARTESIAN_POINT ( 'NONE',  ( -1.339745962155585168, 8.919658201469705006, -5.000000000000015987 ) ) ;
#6851=CARTESIAN_POINT ( 'NONE',  ( -2.499999999999996447, 16.16666666666666430, 4.330127018922195425 ) ) ;
#6854=CARTESIAN_POINT ( 'NONE',  ( 4.458734124999998549, -44.72916666530106511, -2.574251347313721627 ) ) ;
#6855=CARTESIAN_POINT ( 'NONE',  ( -4.999999999999999112, -77.79166666393547303, 2.886751345948131764 ) ) ;
#6860=CARTESIAN_POINT ( 'NONE',  ( 2.229367062500001939, -84.22916666530107932, 3.861377020970579999 ) ) ;
#6863=CARTESIAN_POINT ( 'NONE',  ( 2.499999999999998668, -25.33333333333333215, -4.330127018922193649 ) ) ;
#6867=ORIENTED_EDGE ( 'NONE', *, *, #23901, .T. ) ;
#6868=CARTESIAN_POINT ( 'NONE',  ( 4.458734124999999437, -88.81249999863439371, -5.460374474430324690E-16 ) ) ;
#6869=CARTESIAN_POINT ( 'NONE',  ( 4.458734124999998549, 12.02083333469892601, -2.574251347313721627 ) ) ;
#6870=CARTESIAN_POINT ( 'NONE',  ( 1.060575238724906964E-15, 17.37500000273118417, 5.773502691896257311 ) ) ;
#6879=DIRECTION ( 'NONE',  ( -0.000000000000000000, 1.000000000000000000, -0.000000000000000000 ) ) ;
#6880=CARTESIAN_POINT ( 'NONE',  ( -6.972266317189433020E-16, -11.12499999726881406, -5.000000000000000000 ) ) ;
#6884=CARTESIAN_POINT ( 'NONE',  ( 4.458734124999999437, -17.06249999863440792, -5.460374474430324690E-16 ) ) ;
#6892=ORIENTED_EDGE ( 'NONE', *, *, #42758, .F. ) ;
#6894=ORIENTED_EDGE ( 'NONE', *, *, #41762, .T. ) ;
#6895=CARTESIAN_POINT ( 'NONE',  ( 4.458734125000001214, -64.14583333196773651, 2.574251347313718519 ) ) ;
#6896=CARTESIAN_POINT ( 'NONE',  ( 1.975475456537005874E-15, 11.37500000273118239, 5.000000000000000000 ) ) ;
#6898=VERTEX_POINT ( 'NONE', #15537 ) ;
#6899=AXIS2_PLACEMENT_3D ( 'NONE', #61335, #2476, #60062 ) ;
#6900=CARTESIAN_POINT ( 'NONE',  ( -2.500000000000000444, -8.041666663935481907, -4.330127018922193649 ) ) ;
#6902=DIRECTION ( 'NONE',  ( -0.000000000000000000, 1.000000000000000000, -0.000000000000000000 ) ) ;
#6904=AXIS2_PLACEMENT_3D ( 'NONE', #9613, #24414, #53996 ) ;
#6908=CARTESIAN_POINT ( 'NONE',  ( 4.458734124999999437, 6.187500001365593860, -5.460374474430324690E-16 ) ) ;
#6911=CARTESIAN_POINT ( 'NONE',  ( 5.000000000000000000, -108.3749999972688016, -6.123233995736766282E-16 ) ) ;
#6912=CARTESIAN_POINT ( 'NONE',  ( 2.499999999999998668, -25.33333333333333215, -4.330127018922193649 ) ) ;
#6913=ORIENTED_EDGE ( 'NONE', *, *, #28761, .F. ) ;
#6914=CARTESIAN_POINT ( 'NONE',  ( 4.458734125000000326, -72.89583333196775072, 2.574251347313718519 ) ) ;
#6915=LINE ( 'NONE', #35540, #12994 ) ;
#6916=CARTESIAN_POINT ( 'NONE',  ( -3.152548672688508926E-16, 13.43750000136559386, -5.148502694627439702 ) ) ;
#6920=CARTESIAN_POINT ( 'NONE',  ( -2.229367062499996610, -56.39583333196773651, 3.861377020970582219 ) ) ;
#6921=CARTESIAN_POINT ( 'NONE',  ( -5.000000000000000000, -13.95833333060215153, -2.886751345948128211 ) ) ;
#6922=DIRECTION ( 'NONE',  ( -0.000000000000000000, 1.000000000000000000, -0.000000000000000000 ) ) ;
#6925=CARTESIAN_POINT ( 'NONE',  ( -3.152548672688508926E-16, -21.81249999863440436, -5.148502694627439702 ) ) ;
#6926=ORIENTED_EDGE ( 'NONE', *, *, #26360, .F. ) ;
#6928=CARTESIAN_POINT ( 'NONE',  ( 2.229367062499998831, -107.6458333319677365, -3.861377020970580887 ) ) ;
#6931=CARTESIAN_POINT ( 'NONE',  ( 2.229367062500001939, -103.2291666653010651, 3.861377020970579999 ) ) ;
#6932=CARTESIAN_POINT ( 'NONE',  ( 2.229367062499998831, -27.64583333196774007, -3.861377020970580887 ) ) ;
#6933=CARTESIAN_POINT ( 'NONE',  ( -4.999999999999999112, -61.79166666393546592, 2.886751345948131764 ) ) ;
#6937=CARTESIAN_POINT ( 'NONE',  ( 4.458734124999998549, -22.72916666530107221, -2.574251347313721627 ) ) ;
#6938=CARTESIAN_POINT ( 'NONE',  ( -4.458734124999999437, -71.64583333196773651, -2.574251347313719407 ) ) ;
#6941=LINE ( 'NONE', #51001, #60502 ) ;
#6943=CARTESIAN_POINT ( 'NONE',  ( 5.000000000000000000, -12.41666666666666607, -2.886751345948129988 ) ) ;
#6945=ORIENTED_EDGE ( 'NONE', *, *, #33776, .T. ) ;
#6948=CARTESIAN_POINT ( 'NONE',  ( 1.975475456537005874E-15, -2.624999997268813168, 5.000000000000000000 ) ) ;
#6949=CARTESIAN_POINT ( 'NONE',  ( 2.499999999999998668, -92.33333333333334281, -4.330127018922193649 ) ) ;
#6951=VECTOR ( 'NONE', #299, 1000.000000000000000 ) ;
#6964=CARTESIAN_POINT ( 'NONE',  ( -5.926426369611017623E-15, 26.25000000000000000, 5.000000000000000000 ) ) ;
#6970=ORIENTED_EDGE ( 'NONE', *, *, #36265, .T. ) ;
#6974=ORIENTED_EDGE ( 'NONE', *, *, #32342, .T. ) ;
#6976=ADVANCED_FACE ( 'NONE', ( #25819 ), #5886, .T. ) ;
#6979=ORIENTED_EDGE ( 'NONE', *, *, #15409, .T. ) ;
#6980=CARTESIAN_POINT ( 'NONE',  ( -3.152548672688508926E-16, -77.56249999863440792, -5.148502694627439702 ) ) ;
#6981=CARTESIAN_POINT ( 'NONE',  ( 2.229367062500001939, 29.02083333469892779, 3.861377020970579999 ) ) ;
#6988=CARTESIAN_POINT ( 'NONE',  ( 0.000000000000000000, -120.0000000000000000, 0.000000000000000000 ) ) ;
#6990=( BOUNDED_CURVE ( )  B_SPLINE_CURVE ( 2, ( #19561, #39173, #25026, #45281, #25344, #53976, #15060, #44315, #49471 ),
 .UNSPECIFIED., .F., .F. ) 
 B_SPLINE_CURVE_WITH_KNOTS ( ( 3, 2, 2, 2, 3 ),
 ( 0.8946428571428571841, 0.8952380952380952772, 0.8964285714285714635, 0.8976190476190476497, 0.8982142857142857428 ),
 .UNSPECIFIED. ) 
 CURVE ( )  GEOMETRIC_REPRESENTATION_ITEM ( )  RATIONAL_B_SPLINE_CURVE ( ( 0.9330127018922194093, 0.9330127018922194093, 1.000000000000000000, 0.8660254037844387076, 1.000000000000000000, 0.8660254037844387076, 1.000000000000000000, 0.9330127018922194093, 0.9330127018922194093 ) ) 
 REPRESENTATION_ITEM ( '' )  );
#6993=CARTESIAN_POINT ( 'NONE',  ( 4.458734124999999437, -53.81249999863439371, -5.460374474430324690E-16 ) ) ;
#6995=CARTESIAN_POINT ( 'NONE',  ( 4.458734125000001214, 29.10416666803225993, 2.574251347313718519 ) ) ;
#6996=CARTESIAN_POINT ( 'NONE',  ( 2.499999999999998668, -107.3333333333333428, -4.330127018922193649 ) ) ;
#6998=CARTESIAN_POINT ( 'NONE',  ( -2.229367062499996610, -41.39583333196773651, 3.861377020970582219 ) ) ;
#6999=CARTESIAN_POINT ( 'NONE',  ( -5.000000000000000000, 2.041666669397854239, -2.886751345948128211 ) ) ;
#7003=CARTESIAN_POINT ( 'NONE',  ( -5.000000000000000000, 5.916666666666666963, -2.886751345948128211 ) ) ;
#7004=CARTESIAN_POINT ( 'NONE',  ( 2.229367062500001939, -94.97916666530106511, 3.861377020970579999 ) ) ;
#7005=CARTESIAN_POINT ( 'NONE',  ( -2.229367062499996610, -7.395833331967735624, 3.861377020970582219 ) ) ;
#7009=CARTESIAN_POINT ( 'NONE',  ( -3.152548672688508926E-16, -88.56249999863439371, -5.148502694627439702 ) ) ;
#7010=CARTESIAN_POINT ( 'NONE',  ( 5.000000000000000000, 27.50000000000000000, -6.123233995736766282E-16 ) ) ;
#7011=CARTESIAN_POINT ( 'NONE',  ( -4.458734124999999437, -88.56249999863439371, 0.000000000000000000 ) ) ;
#7013=CARTESIAN_POINT ( 'NONE',  ( 6.123233995736766282E-16, -120.0000000000000000, -5.000000000000000000 ) ) ;
#7015=CARTESIAN_POINT ( 'NONE',  ( 4.458734125000000326, -5.895833331967740953, 2.574251347313718519 ) ) ;
#7016=CARTESIAN_POINT ( 'NONE',  ( 4.458734124999999437, 18.93750000136559564, -5.460374474430324690E-16 ) ) ;
#7017=CARTESIAN_POINT ( 'NONE',  ( -4.458734124999999437, -50.64583333196773651, -2.574251347313719407 ) ) ;
#7018=FACE_OUTER_BOUND ( 'NONE', #47108, .T. ) ;
#7021=CARTESIAN_POINT ( 'NONE',  ( 1.339745962155612702, -84.29465819873850307, -5.000000000000000000 ) ) ;
#7022=VERTEX_POINT ( 'NONE', #35472 ) ;
#7025=CARTESIAN_POINT ( 'NONE',  ( -2.229367062499996610, -79.14583333196773651, 3.861377020970582219 ) ) ;
#7026=CARTESIAN_POINT ( 'NONE',  ( -2.229367062500000163, 28.27083333469892779, -3.861377020970580443 ) ) ;
#7028=CARTESIAN_POINT ( 'NONE',  ( -5.000000000000000000, -94.00000000000000000, 0.000000000000000000 ) ) ;
#7029=CARTESIAN_POINT ( 'NONE',  ( 0.000000000000000000, -120.0000000000000000, 5.000000000000000000 ) ) ;
#7031=CARTESIAN_POINT ( 'NONE',  ( -2.500000000000000444, -63.16666666666666430, -4.330127018922193649 ) ) ;
#7036=CARTESIAN_POINT ( 'NONE',  ( 1.339745962155615144, 7.294658198738519950, 4.999999999999999112 ) ) ;
#7037=( BOUNDED_CURVE ( )  B_SPLINE_CURVE ( 2, ( #51336, #36213, #57117, #8218, #56481, #12404, #32652, #26886, #60988 ),
 .UNSPECIFIED., .F., .F. ) 
 B_SPLINE_CURVE_WITH_KNOTS ( ( 3, 2, 2, 2, 3 ),
 ( 0.7517857142857142794, 0.7523809523809523725, 0.7535714285714285587, 0.7547619047619047450, 0.7553571428571428381 ),
 .UNSPECIFIED. ) 
 CURVE ( )  GEOMETRIC_REPRESENTATION_ITEM ( )  RATIONAL_B_SPLINE_CURVE ( ( 0.9330127018922194093, 0.9330127018922194093, 1.000000000000000000, 0.8660254037844387076, 1.000000000000000000, 0.8660254037844387076, 1.000000000000000000, 0.9330127018922194093, 0.9330127018922194093 ) ) 
 REPRESENTATION_ITEM ( '' )  );
#7047=ORIENTED_EDGE ( 'NONE', *, *, #58246, .T. ) ;
#7050=CARTESIAN_POINT ( 'NONE',  ( -3.152548672688508926E-16, -44.81249999863440792, -5.148502694627439702 ) ) ;
#7053=CARTESIAN_POINT ( 'NONE',  ( -1.339745962155613812, -22.08034179853029855, -5.000000000000000000 ) ) ;
#7057=AXIS2_PLACEMENT_3D ( 'NONE', #35794, #34833, #44470 ) ;
#7059=CARTESIAN_POINT ( 'NONE',  ( -4.999999999999998224, -58.79166666393546592, 2.886751345948131764 ) ) ;
#7061=CARTESIAN_POINT ( 'NONE',  ( 4.458734125000001214, -95.14583333196772230, 2.574251347313718519 ) ) ;
#7069=CARTESIAN_POINT ( 'NONE',  ( -4.458734124999998549, -1.229166665301071326, 2.574251347313722516 ) ) ;
#7070=CARTESIAN_POINT ( 'NONE',  ( 2.229367062499998831, -97.89583333196773651, -3.861377020970580887 ) ) ;
#7072=CARTESIAN_POINT ( 'NONE',  ( -3.152548672688508926E-16, -24.81249999863440436, -5.148502694627439702 ) ) ;
#7076=CARTESIAN_POINT ( 'NONE',  ( 1.975475456537005874E-15, -70.75000000000000000, 5.000000000000000000 ) ) ;
#7079=AXIS2_PLACEMENT_3D ( 'NONE', #8521, #31696, #46808 ) ;
#7080=CARTESIAN_POINT ( 'NONE',  ( -2.229367062499996610, 13.60416666803226171, 3.861377020970582219 ) ) ;
#7081=EDGE_LOOP ( 'NONE', ( #54082, #49054, #26434, #5050 ) ) ;
#7083=CARTESIAN_POINT ( 'NONE',  ( -2.499999999999996447, -84.83333333333332860, 4.330127018922195425 ) ) ;
#7084=CARTESIAN_POINT ( 'NONE',  ( 2.229367062500001939, -19.97916666530107221, 3.861377020970579999 ) ) ;
#7086=CARTESIAN_POINT ( 'NONE',  ( -6.972266317189433020E-16, -3.250000000000001332, -5.000000000000000000 ) ) ;
#7089=CARTESIAN_POINT ( 'NONE',  ( 1.060575238724906964E-15, -46.62499999726880873, 5.773502691896257311 ) ) ;
#7090=CARTESIAN_POINT ( 'NONE',  ( -2.500000000000000444, -2.041666663935480575, -4.330127018922193649 ) ) ;
#7091=CARTESIAN_POINT ( 'NONE',  ( -2.229367062499996610, 7.854166668032260823, 3.861377020970582219 ) ) ;
#7095=CARTESIAN_POINT ( 'NONE',  ( 2.229367062499998831, -66.64583333196773651, -3.861377020970580887 ) ) ;
#7097=CARTESIAN_POINT ( 'NONE',  ( 1.060575238724906964E-15, -0.7500000000000007772, 5.773502691896257311 ) ) ;
#7099=CARTESIAN_POINT ( 'NONE',  ( -1.336351044127974539E-14, 22.24999999999999645, 5.000000000000000000 ) ) ;
#7100=CARTESIAN_POINT ( 'NONE',  ( 2.229367062499998831, -57.64583333196773651, -3.861377020970580887 ) ) ;
#7101=CARTESIAN_POINT ( 'NONE',  ( 5.000000000000000000, -92.37499999726880162, -6.123233995736766282E-16 ) ) ;
#7103=CARTESIAN_POINT ( 'NONE',  ( -2.500000000000000444, -80.16666666666665719, -4.330127018922193649 ) ) ;
#7106=CARTESIAN_POINT ( 'NONE',  ( -1.339745962155610925, -90.66965819600733312, 5.000000000000000000 ) ) ;
#7107=CARTESIAN_POINT ( 'NONE',  ( -5.000000000000000000, -51.00000000000000711, 0.000000000000000000 ) ) ;
#7108=DIRECTION ( 'NONE',  ( -0.000000000000000000, 1.000000000000000000, -0.000000000000000000 ) ) ;
#7109=ORIENTED_EDGE ( 'NONE', *, *, #23709, .T. ) ;
#7110=CARTESIAN_POINT ( 'NONE',  ( 9.457646018065525792E-16, -109.0624999986344221, 5.148502694627439702 ) ) ;
#7111=CARTESIAN_POINT ( 'NONE',  ( 9.457646018065525792E-16, -0.3124999986344051961, 5.148502694627439702 ) ) ;
#7115=( BOUNDED_CURVE ( )  B_SPLINE_CURVE ( 2, ( #57774, #14004, #13695, #37514, #23675, #28487, #3430, #33007, #51996 ),
 .UNSPECIFIED., .F., .F. ) 
 B_SPLINE_CURVE_WITH_KNOTS ( ( 3, 2, 2, 2, 3 ),
 ( 0.1803571428571428548, 0.1809523809523809479, 0.1821428571428571341, 0.1833333333333333204, 0.1839285714285714413 ),
 .UNSPECIFIED. ) 
 CURVE ( )  GEOMETRIC_REPRESENTATION_ITEM ( )  RATIONAL_B_SPLINE_CURVE ( ( 0.9330127018922194093, 0.9330127018922194093, 1.000000000000000000, 0.8660254037844387076, 1.000000000000000000, 0.8660254037844387076, 1.000000000000000000, 0.9330127018922178550, 0.9330127018922194093 ) ) 
 REPRESENTATION_ITEM ( '' )  );
#7116=CARTESIAN_POINT ( 'NONE',  ( -5.000000000000000000, -26.08333333333332860, -2.886751345948128211 ) ) ;
#7119=ORIENTED_EDGE ( 'NONE', *, *, #52826, .F. ) ;
#7120=CARTESIAN_POINT ( 'NONE',  ( -2.500000000000000444, 27.95833333606451987, -4.330127018922193649 ) ) ;
#7126=CARTESIAN_POINT ( 'NONE',  ( 4.458734124999998549, -31.97916666530107577, -2.574251347313721627 ) ) ;
#7133=EDGE_CURVE ( 'NONE', #7022, #25814, #18624, .T. ) ;
#7134=EDGE_CURVE ( 'NONE', #9564, #32043, #18051, .T. ) ;
#7135=CARTESIAN_POINT ( 'NONE',  ( 5.000000000000000000, -83.37499999726881583, -6.123233995736766282E-16 ) ) ;
#7136=ORIENTED_EDGE ( 'NONE', *, *, #12788, .T. ) ;
#7137=CARTESIAN_POINT ( 'NONE',  ( -4.458734124999998549, -78.47916666530107932, 2.574251347313722516 ) ) ;
#7139=EDGE_CURVE ( 'NONE', #57442, #9470, #33280, .T. ) ;
#7142=DIRECTION ( 'NONE',  ( 0.000000000000000000, 0.000000000000000000, 1.000000000000000000 ) ) ;
#7144=CARTESIAN_POINT ( 'NONE',  ( 4.458734124999998549, -6.979166665301073103, -2.574251347313721627 ) ) ;
#7145=ORIENTED_EDGE ( 'NONE', *, *, #28761, .T. ) ;
#7146=EDGE_CURVE ( 'NONE', #60305, #27444, #38164, .T. ) ;
#7149=CARTESIAN_POINT ( 'NONE',  ( -5.000000000000000000, -92.95833333060214443, -2.886751345948128211 ) ) ;
#7150=ORIENTED_EDGE ( 'NONE', *, *, #21762, .F. ) ;
#7151=CARTESIAN_POINT ( 'NONE',  ( 2.229367062500001939, -8.229166665301073991, 3.861377020970579999 ) ) ;
#7152=EDGE_CURVE ( 'NONE', #11069, #32964, #37297, .T. ) ;
#7153=FACE_OUTER_BOUND ( 'NONE', #24183, .T. ) ;
#7159=CARTESIAN_POINT ( 'NONE',  ( 4.458734124999998549, -84.72916666530106511, -2.574251347313721627 ) ) ;
#7161=DIRECTION ( 'NONE',  ( 0.000000000000000000, 0.000000000000000000, 1.000000000000000000 ) ) ;
#7162=CARTESIAN_POINT ( 'NONE',  ( -4.458734124999999437, -1.395833331967737179, -2.574251347313719407 ) ) ;
#7163=CARTESIAN_POINT ( 'NONE',  ( 5.000000000000000888, -51.58333333333332149, 2.886751345948126879 ) ) ;
#7164=CARTESIAN_POINT ( 'NONE',  ( -3.535250795749689387E-16, -29.12499999726881228, -5.773502691896257311 ) ) ;
#7166=CARTESIAN_POINT ( 'NONE',  ( 2.229367062499998831, 26.35416666803225993, -3.861377020970580887 ) ) ;
#7167=CARTESIAN_POINT ( 'NONE',  ( -5.000000000000000000, -20.95833333060214798, -2.886751345948128211 ) ) ;
#7168=( BOUNDED_CURVE ( )  B_SPLINE_CURVE ( 2, ( #61930, #8208, #32008, #57106, #37790, #18780, #23316, #12393, #62868 ),
 .UNSPECIFIED., .F., .F. ) 
 B_SPLINE_CURVE_WITH_KNOTS ( ( 3, 2, 2, 2, 3 ),
 ( 0.2446428571428571341, 0.2452380952380952273, 0.2464285714285714413, 0.2476190476190476275, 0.2482142857142857206 ),
 .UNSPECIFIED. ) 
 CURVE ( )  GEOMETRIC_REPRESENTATION_ITEM ( )  RATIONAL_B_SPLINE_CURVE ( ( 0.9330127018922194093, 0.9330127018922194093, 1.000000000000000000, 0.8660254037844387076, 1.000000000000000000, 0.8660254037844387076, 1.000000000000000000, 0.9330127018922194093, 0.9330127018922194093 ) ) 
 REPRESENTATION_ITEM ( '' )  );
#7170=CARTESIAN_POINT ( 'NONE',  ( 2.229367062500001939, -53.97916666530107221, 3.861377020970579999 ) ) ;
#7171=CARTESIAN_POINT ( 'NONE',  ( 2.229367062500001939, -39.22916666530107221, 3.861377020970579999 ) ) ;
#7174=CARTESIAN_POINT ( 'NONE',  ( 2.499999999999998668, 17.66666666666666430, -4.330127018922193649 ) ) ;
#7176=CYLINDRICAL_SURFACE ( 'NONE', #32549, 5.000000000000000000 ) ;
#7178=CARTESIAN_POINT ( 'NONE',  ( -4.458734124999999437, -45.31249999863440081, 0.000000000000000000 ) ) ;
#7179=CARTESIAN_POINT ( 'NONE',  ( 5.000000000000000000, -80.37499999726881583, -6.123233995736766282E-16 ) ) ;
#7181=CARTESIAN_POINT ( 'NONE',  ( 1.339745962155612702, -65.16965819600733312, -5.000000000000000000 ) ) ;
#7183=CARTESIAN_POINT ( 'NONE',  ( 4.458734125000000326, -88.14583333196773651, 2.574251347313718519 ) ) ;
#7185=CARTESIAN_POINT ( 'NONE',  ( -6.972266317189433020E-16, 13.87500000273118594, -5.000000000000000000 ) ) ;
#7186=CARTESIAN_POINT ( 'NONE',  ( 2.500000000000002220, -30.66666666666666785, 4.330127018922192761 ) ) ;
#7191=CARTESIAN_POINT ( 'NONE',  ( -3.152548672688508926E-16, -88.56249999863439371, -5.148502694627439702 ) ) ;
#7192=CARTESIAN_POINT ( 'NONE',  ( -4.458734124999999437, 11.43750000136559564, 0.000000000000000000 ) ) ;
#7193=CARTESIAN_POINT ( 'NONE',  ( 2.500000000000002220, 14.45833333606451809, 4.330127018922192761 ) ) ;
#7194=CARTESIAN_POINT ( 'NONE',  ( 1.975475456537005874E-15, -101.6249999972688158, 5.000000000000000000 ) ) ;
#7201=CARTESIAN_POINT ( 'NONE',  ( -2.500000000000000444, 17.95833333606451632, -4.330127018922193649 ) ) ;
#7203=CARTESIAN_POINT ( 'NONE',  ( 1.339745962155499015, -107.7053418012614543, 5.000000000000065725 ) ) ;
#7205=CARTESIAN_POINT ( 'NONE',  ( -2.229367062499996610, -14.39583333196774184, 3.861377020970582219 ) ) ;
#7213=EDGE_CURVE ( 'NONE', #32181, #39986, #13487, .T. ) ;
#7214=ORIENTED_EDGE ( 'NONE', *, *, #4813, .F. ) ;
#7215=DIRECTION ( 'NONE',  ( 0.000000000000000000, 0.000000000000000000, 1.000000000000000000 ) ) ;
#7217=CARTESIAN_POINT ( 'NONE',  ( -3.152548672688508926E-16, -60.81249999863440081, -5.148502694627439702 ) ) ;
#7219=CARTESIAN_POINT ( 'NONE',  ( 5.000000000000000888, -8.583333333333332149, 2.886751345948126879 ) ) ;
#7222=( BOUNDED_CURVE ( )  B_SPLINE_CURVE ( 2, ( #20987, #40590, #16154, #30299, #49919, #5871, #42015, #32048, #7310 ),
 .UNSPECIFIED., .F., .F. ) 
 B_SPLINE_CURVE_WITH_KNOTS ( ( 3, 2, 2, 2, 3 ),
 ( 0.4089285714285714191, 0.4095238095238095122, 0.4107142857142856984, 0.4119047619047618847, 0.4124999999999999778 ),
 .UNSPECIFIED. ) 
 CURVE ( )  GEOMETRIC_REPRESENTATION_ITEM ( )  RATIONAL_B_SPLINE_CURVE ( ( 0.9330127018922194093, 0.9330127018922194093, 1.000000000000000000, 0.8660254037844387076, 1.000000000000000000, 0.8660254037844387076, 1.000000000000000000, 0.9330127018922194093, 0.9330127018922194093 ) ) 
 REPRESENTATION_ITEM ( '' )  );
#7229=CARTESIAN_POINT ( 'NONE',  ( 1.975475456537005874E-15, -77.75000000000000000, 5.000000000000000000 ) ) ;
#7230=CARTESIAN_POINT ( 'NONE',  ( -3.152548672688508926E-16, 6.437500001365592972, -5.148502694627439702 ) ) ;
#7231=EDGE_CURVE ( 'NONE', #21367, #721, #49236, .T. ) ;
#7234=CYLINDRICAL_SURFACE ( 'NONE', #30532, 5.000000000000000000 ) ;
#7236=EDGE_CURVE ( 'NONE', #41687, #27676, #7375, .T. ) ;
#7237=CARTESIAN_POINT ( 'NONE',  ( -2.229367062499996610, -68.14583333196773651, 3.861377020970582219 ) ) ;
#7238=LINE ( 'NONE', #2110, #54078 ) ;
#7239=CARTESIAN_POINT ( 'NONE',  ( 4.458734124999999437, 14.18750000136559386, -5.460374474430324690E-16 ) ) ;
#7242=EDGE_CURVE ( 'NONE', #42402, #17975, #6990, .T. ) ;
#7244=CARTESIAN_POINT ( 'NONE',  ( 4.458734124999999437, -54.06249999863440081, -5.460374474430324690E-16 ) ) ;
#7245=CARTESIAN_POINT ( 'NONE',  ( 1.060575238724906964E-15, -15.62499999726881406, 5.773502691896257311 ) ) ;
#7246=CARTESIAN_POINT ( 'NONE',  ( -2.499999999999996447, -99.83333333333332860, 4.330127018922195425 ) ) ;
#7247=LINE ( 'NONE', #15690, #15188 ) ;
#7249=CARTESIAN_POINT ( 'NONE',  ( -2.229367062500000163, -20.72916666530107221, -3.861377020970580443 ) ) ;
#7250=VERTEX_POINT ( 'NONE', #44637 ) ;
#7251=CARTESIAN_POINT ( 'NONE',  ( -2.500000000000000444, -61.16666666666666430, -4.330127018922193649 ) ) ;
#7252=CARTESIAN_POINT ( 'NONE',  ( -3.152548672688508926E-16, -108.5624999986343937, -5.148502694627439702 ) ) ;
#7254=VERTEX_POINT ( 'NONE', #39808 ) ;
#7255=CARTESIAN_POINT ( 'NONE',  ( -3.152548672688508926E-16, -100.8124999986343937, -5.148502694627439702 ) ) ;
#7256=CARTESIAN_POINT ( 'NONE',  ( -4.458734124999999437, -25.39583333196773651, -2.574251347313719407 ) ) ;
#7257=CARTESIAN_POINT ( 'NONE',  ( -5.000000000000000000, -61.87499999726880873, 0.000000000000000000 ) ) ;
#7260=CARTESIAN_POINT ( 'NONE',  ( -3.152548672688508926E-16, -25.56249999863440792, -5.148502694627439702 ) ) ;
#7261=CARTESIAN_POINT ( 'NONE',  ( 2.229367062499998831, -71.89583333196773651, -3.861377020970580887 ) ) ;
#7262=CARTESIAN_POINT ( 'NONE',  ( -2.499999999999996447, -39.70833333060214443, 4.330127018922195425 ) ) ;
#7264=DIRECTION ( 'NONE',  ( -0.000000000000000000, 1.000000000000000000, -0.000000000000000000 ) ) ;
#7266=CARTESIAN_POINT ( 'NONE',  ( -4.999999999999999112, -14.91666666666666785, 2.886751345948131764 ) ) ;
#7272=CARTESIAN_POINT ( 'NONE',  ( -2.499999999999996447, -110.7083333306021444, 4.330127018922195425 ) ) ;
#7275=DIRECTION ( 'NONE',  ( -0.000000000000000000, 1.000000000000000000, 0.000000000000000000 ) ) ;
#7279=DIRECTION ( 'NONE',  ( -0.000000000000000000, 1.000000000000000000, -0.000000000000000000 ) ) ;
#7282=ORIENTED_EDGE ( 'NONE', *, *, #53511, .T. ) ;
#7288=EDGE_CURVE ( 'NONE', #62194, #4978, #15992, .T. ) ;
#7299=CARTESIAN_POINT ( 'NONE',  ( -1.339745962155610925, 23.33034180399266333, 5.000000000000000000 ) ) ;
#7300=ORIENTED_EDGE ( 'NONE', *, *, #3671, .T. ) ;
#7302=CARTESIAN_POINT ( 'NONE',  ( 4.458734125000001214, -75.89583333196775072, 2.574251347313718519 ) ) ;
#7303=CARTESIAN_POINT ( 'NONE',  ( 4.458734125000001214, 24.10416666803226349, 2.574251347313718519 ) ) ;
#7304=CARTESIAN_POINT ( 'NONE',  ( -4.999999999999998224, -53.91666666666667140, 2.886751345948131764 ) ) ;
#7310=CARTESIAN_POINT ( 'NONE',  ( 1.975475456537005874E-15, -27.74999999999999645, 5.000000000000000000 ) ) ;
#7313=CARTESIAN_POINT ( 'NONE',  ( -4.458734124999997661, -52.22916666530107932, 2.574251347313722516 ) ) ;
#7316=CARTESIAN_POINT ( 'NONE',  ( 4.458734124999999437, 26.18750000136559564, -5.460374474430324690E-16 ) ) ;
#7317=CARTESIAN_POINT ( 'NONE',  ( -5.000000000000000000, -105.0833333333333286, -2.886751345948128211 ) ) ;
#7320=CARTESIAN_POINT ( 'NONE',  ( -4.458734124999998549, -40.47916666530107221, 2.574251347313722516 ) ) ;
#7321=CARTESIAN_POINT ( 'NONE',  ( -3.535250795749689387E-16, 1.875000002731185056, -5.773502691896257311 ) ) ;
#7325=CARTESIAN_POINT ( 'NONE',  ( -2.499999999999996447, 6.166666666666667851, 4.330127018922195425 ) ) ;
#7326=CARTESIAN_POINT ( 'NONE',  ( -3.152548672688508926E-16, -100.5624999986344079, -5.148502694627439702 ) ) ;
#7327=CARTESIAN_POINT ( 'NONE',  ( -3.152548672688508926E-16, -7.812499998634405252, -5.148502694627439702 ) ) ;
#7328=ORIENTED_EDGE ( 'NONE', *, *, #60224, .T. ) ;
#7329=CARTESIAN_POINT ( 'NONE',  ( 0.000000000000000000, -120.0000000000000000, 0.000000000000000000 ) ) ;
#7330=CARTESIAN_POINT ( 'NONE',  ( 1.975475456537005874E-15, -35.62499999726880162, 5.000000000000000000 ) ) ;
#7331=CARTESIAN_POINT ( 'NONE',  ( -4.458734124999999437, -93.31249999863440792, 0.000000000000000000 ) ) ;
#7333=CARTESIAN_POINT ( 'NONE',  ( -2.229367062499996610, -87.39583333196773651, 3.861377020970582219 ) ) ;
#7335=LINE ( 'NONE', #56539, #62325 ) ;
#7337=CARTESIAN_POINT ( 'NONE',  ( -3.152548672688508926E-16, -9.562499998634409692, -5.148502694627439702 ) ) ;
#7338=CARTESIAN_POINT ( 'NONE',  ( -4.458734124999998549, 15.52083333469892779, 2.574251347313722516 ) ) ;
#7339=CARTESIAN_POINT ( 'NONE',  ( 4.458734125000000326, -54.14583333196773651, 2.574251347313718519 ) ) ;
#7342=CARTESIAN_POINT ( 'NONE',  ( 2.500000000000002220, -84.66666666666667140, 4.330127018922192761 ) ) ;
#7346=CARTESIAN_POINT ( 'NONE',  ( 2.229367062499998831, -80.64583333196773651, -3.861377020970580887 ) ) ;
#7347=CARTESIAN_POINT ( 'NONE',  ( 4.458734124999998549, 23.02083333469892423, -2.574251347313721627 ) ) ;
#7351=CARTESIAN_POINT ( 'NONE',  ( -4.999999999999998224, -57.79166666393548013, 2.886751345948131764 ) ) ;
#7354=CARTESIAN_POINT ( 'NONE',  ( 2.500000000000002220, -62.66666666666666430, 4.330127018922192761 ) ) ;
#7359=CARTESIAN_POINT ( 'NONE',  ( -2.499999999999996447, 28.16666666666666785, 4.330127018922195425 ) ) ;
#7360=CARTESIAN_POINT ( 'NONE',  ( -5.000000000000000000, -106.9583333306021444, -2.886751345948128211 ) ) ;
#7373=CARTESIAN_POINT ( 'NONE',  ( -4.458734124999998549, -54.47916666530107932, 2.574251347313722516 ) ) ;
#7375=( BOUNDED_CURVE ( )  B_SPLINE_CURVE ( 2, ( #30155, #49145, #5091, #279, #35318, #29839, #20204, #5730, #29201 ),
 .UNSPECIFIED., .F., .F. ) 
 B_SPLINE_CURVE_WITH_KNOTS ( ( 3, 2, 2, 2, 3 ),
 ( 0.4696428571428571397, 0.4702380952380952328, 0.4714285714285714191, 0.4726190476190476053, 0.4732142857142856984 ),
 .UNSPECIFIED. ) 
 CURVE ( )  GEOMETRIC_REPRESENTATION_ITEM ( )  RATIONAL_B_SPLINE_CURVE ( ( 0.9330127018922194093, 0.9330127018922194093, 1.000000000000000000, 0.8660254037844387076, 1.000000000000000000, 0.8660254037844387076, 1.000000000000000000, 0.9330127018922194093, 0.9330127018922194093 ) ) 
 REPRESENTATION_ITEM ( '' )  );
#7380=DIRECTION ( 'NONE',  ( 0.000000000000000000, 0.000000000000000000, 1.000000000000000000 ) ) ;
#7383=CARTESIAN_POINT ( 'NONE',  ( -4.458734124999998549, -97.47916666530106511, 2.574251347313722516 ) ) ;
#7389=CARTESIAN_POINT ( 'NONE',  ( 4.458734124999998549, -0.7291666653010709931, -2.574251347313721627 ) ) ;
#7390=CARTESIAN_POINT ( 'NONE',  ( 9.457646018065525792E-16, -97.31249999863440792, 5.148502694627439702 ) ) ;
#7392=CARTESIAN_POINT ( 'NONE',  ( -2.229367062499996610, -25.39583333196773651, 3.861377020970582219 ) ) ;
#7393=CARTESIAN_POINT ( 'NONE',  ( 1.339745962155612702, -46.29465819873851729, -5.000000000000000000 ) ) ;
#7399=CARTESIAN_POINT ( 'NONE',  ( -4.458734124999997661, 8.520833334698926009, 2.574251347313722516 ) ) ;
#7401=CARTESIAN_POINT ( 'NONE',  ( -1.339745962155613812, -81.20534180126146850, -5.000000000000000000 ) ) ;
#7402=CARTESIAN_POINT ( 'NONE',  ( 5.000000000000000888, -66.45833333060213022, 2.886751345948126879 ) ) ;
#7403=CARTESIAN_POINT ( 'NONE',  ( -3.535250795749689387E-16, -89.25000000000000000, -5.773502691896257311 ) ) ;
#7404=CARTESIAN_POINT ( 'NONE',  ( 2.229367062499998831, -23.64583333196773651, -3.861377020970580887 ) ) ;
#7405=CARTESIAN_POINT ( 'NONE',  ( -2.229367062499996610, -71.39583333196773651, 3.861377020970582219 ) ) ;
#7409=CARTESIAN_POINT ( 'NONE',  ( 5.000000000000000888, -51.45833333060214443, 2.886751345948126879 ) ) ;
#7410=CARTESIAN_POINT ( 'NONE',  ( 2.229367062499998831, 8.354166668032261711, -3.861377020970580887 ) ) ;
#7414=CARTESIAN_POINT ( 'NONE',  ( -2.229367062499996610, -69.14583333196773651, 3.861377020970582219 ) ) ;
#7417=CARTESIAN_POINT ( 'NONE',  ( -3.535250795749689387E-16, 0.7500000000000007772, -5.773502691896257311 ) ) ;
#7419=CARTESIAN_POINT ( 'NONE',  ( -6.972266317189433020E-16, -31.24999999999999645, -5.000000000000000000 ) ) ;
#7420=CARTESIAN_POINT ( 'NONE',  ( 2.229367062499998831, -63.64583333196772941, -3.861377020970580887 ) ) ;
#7421=CARTESIAN_POINT ( 'NONE',  ( -2.499999999999996447, -94.70833333060213022, 4.330127018922195425 ) ) ;
#7422=ADVANCED_FACE ( 'NONE', ( #54938 ), #63640, .T. ) ;
#7423=CARTESIAN_POINT ( 'NONE',  ( 6.123233995736766282E-16, -120.0000000000000000, -5.000000000000000000 ) ) ;
#7427=CARTESIAN_POINT ( 'NONE',  ( 5.000000000000000000, -48.50000000000000000, -6.123233995736766282E-16 ) ) ;
#7428=CARTESIAN_POINT ( 'NONE',  ( -2.500000000000000444, 15.83333333333333037, -4.330127018922193649 ) ) ;
#7429=VERTEX_POINT ( 'NONE', #54620 ) ;
#7431=CARTESIAN_POINT ( 'NONE',  ( -4.458734124999998549, -2.479166665301069550, 2.574251347313722516 ) ) ;
#7435=CARTESIAN_POINT ( 'NONE',  ( 0.000000000000000000, -120.0000000000000000, 0.000000000000000000 ) ) ;
#7447=CARTESIAN_POINT ( 'NONE',  ( 4.458734124999999437, -37.06249999863440792, -5.460374474430324690E-16 ) ) ;
#7454=ADVANCED_FACE ( 'NONE', ( #6378 ), #16650, .T. ) ;
#7457=CARTESIAN_POINT ( 'NONE',  ( 9.457646018065525792E-16, -77.31249999863440792, 5.148502694627439702 ) ) ;
#7459=ORIENTED_EDGE ( 'NONE', *, *, #34461, .F. ) ;
#7461=FACE_OUTER_BOUND ( 'NONE', #2999, .T. ) ;
#7463=CARTESIAN_POINT ( 'NONE',  ( 9.457646018065525792E-16, -7.312499998634405252, 5.148502694627439702 ) ) ;
#7464=VERTEX_POINT ( 'NONE', #41710 ) ;
#7465=ADVANCED_FACE ( 'NONE', ( #55898 ), #30806, .T. ) ;
#7466=CARTESIAN_POINT ( 'NONE',  ( 4.458734124999998549, -8.979166665301073991, -2.574251347313721627 ) ) ;
#7471=CARTESIAN_POINT ( 'NONE',  ( -2.229367062500000163, 26.27083333469892779, -3.861377020970580443 ) ) ;
#7472=ORIENTED_EDGE ( 'NONE', *, *, #43238, .T. ) ;
#7473=CARTESIAN_POINT ( 'NONE',  ( -3.152548672688508926E-16, -85.56249999863439371, -5.148502694627439702 ) ) ;
#7474=CARTESIAN_POINT ( 'NONE',  ( 4.458734125000001214, -8.895833331967736513, 2.574251347313718519 ) ) ;
#7476=CARTESIAN_POINT ( 'NONE',  ( -4.999999999999999112, -32.79166666393547303, 2.886751345948131764 ) ) ;
#7477=DIRECTION ( 'NONE',  ( -0.000000000000000000, 0.000000000000000000, -1.000000000000000000 ) ) ;
#7478=CARTESIAN_POINT ( 'NONE',  ( -4.458734124999999437, 23.68750000136559564, 0.000000000000000000 ) ) ;
#7479=CARTESIAN_POINT ( 'NONE',  ( 5.000000000000000000, -7.416666666666667851, -2.886751345948130876 ) ) ;
#7481=CARTESIAN_POINT ( 'NONE',  ( -4.458734124999998549, -51.22916666530107221, 2.574251347313722516 ) ) ;
#7482=CARTESIAN_POINT ( 'NONE',  ( 4.458734124999998549, -35.97916666530107221, -2.574251347313721627 ) ) ;
#7485=CARTESIAN_POINT ( 'NONE',  ( 1.060575238724906964E-15, 16.25000000000000000, 5.773502691896257311 ) ) ;
#7488=CARTESIAN_POINT ( 'NONE',  ( 9.457646018065525792E-16, -47.06249999863440792, 5.148502694627439702 ) ) ;
#7489=CARTESIAN_POINT ( 'NONE',  ( -3.535250795749689387E-16, -76.12499999726881583, -5.773502691896257311 ) ) ;
#7490=EDGE_CURVE ( 'NONE', #20484, #35996, #24622, .T. ) ;
#7495=CARTESIAN_POINT ( 'NONE',  ( -2.499999999999996447, -63.70833333060215153, 4.330127018922195425 ) ) ;
#7497=CARTESIAN_POINT ( 'NONE',  ( 4.458734125000000326, -83.14583333196773651, 2.574251347313718519 ) ) ;
#7499=CARTESIAN_POINT ( 'NONE',  ( 5.000000000000000000, -35.41666666666667140, -2.886751345948129988 ) ) ;
#7504=CARTESIAN_POINT ( 'NONE',  ( -4.458734124999998549, -91.22916666530106511, 2.574251347313722516 ) ) ;
#7505=CARTESIAN_POINT ( 'NONE',  ( -3.152548672688508926E-16, 15.18750000136559386, -5.148502694627439702 ) ) ;
#7506=CARTESIAN_POINT ( 'NONE',  ( 5.000000000000000888, 16.54166666939785202, 2.886751345948126879 ) ) ;
#7507=CARTESIAN_POINT ( 'NONE',  ( -6.972266317189433020E-16, -35.12499999726880873, -5.000000000000000000 ) ) ;
#7511=CARTESIAN_POINT ( 'NONE',  ( -5.000000000000000000, 15.12500000273118417, 0.000000000000000000 ) ) ;
#7512=CARTESIAN_POINT ( 'NONE',  ( 1.975475456537005874E-15, -45.62499999726880873, 5.000000000000000000 ) ) ;
#7514=CARTESIAN_POINT ( 'NONE',  ( -6.972266317189433020E-16, -26.12499999726881583, -5.000000000000000000 ) ) ;
#7516=DIRECTION ( 'NONE',  ( -0.000000000000000000, 1.000000000000000000, -0.000000000000000000 ) ) ;
#7520=CARTESIAN_POINT ( 'NONE',  ( -2.229367062500000163, -21.72916666530107221, -3.861377020970580443 ) ) ;
#7530=ORIENTED_EDGE ( 'NONE', *, *, #27611, .T. ) ;
#7531=CARTESIAN_POINT ( 'NONE',  ( -4.458734124999999437, -62.56249999863440792, 0.000000000000000000 ) ) ;
#7541=CARTESIAN_POINT ( 'NONE',  ( -4.458734124999998549, 6.770833334698928674, 2.574251347313722516 ) ) ;
#7542=( BOUNDED_CURVE ( )  B_SPLINE_CURVE ( 2, ( #49728, #53913, #58743, #9839, #14670, #5673, #48763, #49084, #536 ),
 .UNSPECIFIED., .F., .F. ) 
 B_SPLINE_CURVE_WITH_KNOTS ( ( 3, 2, 2, 2, 3 ),
 ( 0.2160714285714285809, 0.2166666666666666741, 0.2178571428571428603, 0.2190476190476190466, 0.2196428571428571397 ),
 .UNSPECIFIED. ) 
 CURVE ( )  GEOMETRIC_REPRESENTATION_ITEM ( )  RATIONAL_B_SPLINE_CURVE ( ( 0.9330127018922194093, 0.9330127018922194093, 1.000000000000000000, 0.8660254037844387076, 1.000000000000000000, 0.8660254037844387076, 1.000000000000000000, 0.9330127018922194093, 0.9330127018922194093 ) ) 
 REPRESENTATION_ITEM ( '' )  );
#7545=CARTESIAN_POINT ( 'NONE',  ( 2.500000000000002220, -77.66666666666665719, 4.330127018922192761 ) ) ;
#7548=CARTESIAN_POINT ( 'NONE',  ( 2.229367062499998831, -68.64583333196773651, -3.861377020970580887 ) ) ;
#7549=CARTESIAN_POINT ( 'NONE',  ( 2.499999999999998668, 14.79166666939785202, -4.330127018922193649 ) ) ;
#7550=CARTESIAN_POINT ( 'NONE',  ( -4.458734124999999437, 14.68750000136559386, 0.000000000000000000 ) ) ;
#7553=CARTESIAN_POINT ( 'NONE',  ( 2.229367062500001939, -56.22916666530107221, 3.861377020970579999 ) ) ;
#7554=CARTESIAN_POINT ( 'NONE',  ( 2.499999999999998668, -16.20833333060214443, -4.330127018922193649 ) ) ;
#7555=CARTESIAN_POINT ( 'NONE',  ( -5.000000000000000000, -100.0833333333333144, -2.886751345948128211 ) ) ;
#7557=CARTESIAN_POINT ( 'NONE',  ( -4.769696007084728073, -120.0000000000000000, -1.500000000000000000 ) ) ;
#7558=CARTESIAN_POINT ( 'NONE',  ( 4.458734125000001214, -33.89583333196773651, 2.574251347313718519 ) ) ;
#7559=CARTESIAN_POINT ( 'NONE',  ( 4.458734124999998549, -22.97916666530107221, -2.574251347313721627 ) ) ;
#7562=CARTESIAN_POINT ( 'NONE',  ( 9.457646018065525792E-16, -110.0624999986343795, 5.148502694627439702 ) ) ;
#7565=CARTESIAN_POINT ( 'NONE',  ( -4.458734124999998549, -101.4791666653010651, 2.574251347313722516 ) ) ;
#7566=CARTESIAN_POINT ( 'NONE',  ( -3.152548672688508926E-16, -28.56249999863440436, -5.148502694627439702 ) ) ;
#7567=CARTESIAN_POINT ( 'NONE',  ( -4.999999999999999112, -62.79166666393546592, 2.886751345948131764 ) ) ;
#7571=CARTESIAN_POINT ( 'NONE',  ( 2.229367062499998831, -26.64583333196774007, -3.861377020970580887 ) ) ;
#7572=CARTESIAN_POINT ( 'NONE',  ( -3.152548672688508926E-16, -68.81249999863439371, -5.148502694627439702 ) ) ;
#7573=CARTESIAN_POINT ( 'NONE',  ( 1.975475456537005874E-15, 8.249999999999998224, 5.000000000000000000 ) ) ;
#7575=CARTESIAN_POINT ( 'NONE',  ( -6.972266317189433020E-16, -32.12499999726880873, -5.000000000000000000 ) ) ;
#7577=CARTESIAN_POINT ( 'NONE',  ( 1.060575238724906964E-15, -16.75000000000000355, 5.773502691896257311 ) ) ;
#7579=ORIENTED_EDGE ( 'NONE', *, *, #51779, .T. ) ;
#7580=CYLINDRICAL_SURFACE ( 'NONE', #7079, 5.000000000000000000 ) ;
#7582=ADVANCED_FACE ( 'NONE', ( #3935 ), #42210, .T. ) ;
#7583=CARTESIAN_POINT ( 'NONE',  ( -5.000000000000000000, -86.87499999726880162, 0.000000000000000000 ) ) ;
#7584=CARTESIAN_POINT ( 'NONE',  ( 0.000000000000000000, -120.0000000000000000, 0.000000000000000000 ) ) ;
#7587=EDGE_CURVE ( 'NONE', #58058, #25203, #37796, .T. ) ;
#7592=CARTESIAN_POINT ( 'NONE',  ( -2.500000000000000444, -81.04166666393547303, -4.330127018922193649 ) ) ;
#7597=EDGE_LOOP ( 'NONE', ( #55390, #56950, #21620, #62267 ) ) ;
#7604=AXIS2_PLACEMENT_3D ( 'NONE', #9971, #34740, #45349 ) ;
#7605=EDGE_CURVE ( 'NONE', #37393, #59890, #22963, .T. ) ;
#7612=CARTESIAN_POINT ( 'NONE',  ( -4.999999999999998224, -50.79166666393547303, 2.886751345948131764 ) ) ;
#7617=CARTESIAN_POINT ( 'NONE',  ( -2.229367062499996610, -77.14583333196773651, 3.861377020970582219 ) ) ;
#7618=CARTESIAN_POINT ( 'NONE',  ( -3.152548672688508926E-16, 22.43750000136559208, -5.148502694627439702 ) ) ;
#7620=ORIENTED_EDGE ( 'NONE', *, *, #10529, .T. ) ;
#7621=CARTESIAN_POINT ( 'NONE',  ( 1.339745962155615144, 14.29465819873852084, 4.999999999999999112 ) ) ;
#7625=PLANE ( 'NONE',  #49014 ) ;
#7628=CARTESIAN_POINT ( 'NONE',  ( -2.229367062500000163, -55.47916666530107221, -3.861377020970580443 ) ) ;
#7631=CARTESIAN_POINT ( 'NONE',  ( -5.000000000000000000, -108.9999999999999858, 0.000000000000000000 ) ) ;
#7633=CARTESIAN_POINT ( 'NONE',  ( 2.229367062500001939, -39.22916666530107221, 3.861377020970579999 ) ) ;
#7634=CARTESIAN_POINT ( 'NONE',  ( -2.499999999999996447, 2.291666669397850686, 4.330127018922195425 ) ) ;
#7638=FACE_OUTER_BOUND ( 'NONE', #18358, .T. ) ;
#7639=CARTESIAN_POINT ( 'NONE',  ( 4.458734125000000326, -101.8958333319677365, 2.574251347313718519 ) ) ;
#7640=CARTESIAN_POINT ( 'NONE',  ( 4.458734124999999437, -3.062499998634407472, -5.460374474430324690E-16 ) ) ;
#7643=CARTESIAN_POINT ( 'NONE',  ( -2.229367062499996610, -92.14583333196773651, 3.861377020970582219 ) ) ;
#7644=DIRECTION ( 'NONE',  ( 0.000000000000000000, 0.000000000000000000, 1.000000000000000000 ) ) ;
#7645=CARTESIAN_POINT ( 'NONE',  ( 2.229367062500001939, -84.22916666530107932, 3.861377020970579999 ) ) ;
#7650=CARTESIAN_POINT ( 'NONE',  ( 9.457646018065525792E-16, -11.06249999863440969, 5.148502694627439702 ) ) ;
#7651=CARTESIAN_POINT ( 'NONE',  ( 9.457646018065525792E-16, 15.68750000136559386, 5.148502694627439702 ) ) ;
#7652=CARTESIAN_POINT ( 'NONE',  ( 4.458734124999999437, -51.06249999863440792, -5.460374474430324690E-16 ) ) ;
#7656=CARTESIAN_POINT ( 'NONE',  ( 2.499999999999998668, -84.33333333333332860, -4.330127018922193649 ) ) ;
#7660=CARTESIAN_POINT ( 'NONE',  ( -6.972266317189433020E-16, -76.24999999999998579, -5.000000000000000000 ) ) ;
#7661=CARTESIAN_POINT ( 'NONE',  ( 4.458734124999999437, -81.81249999863440792, -5.460374474430324690E-16 ) ) ;
#7662=CARTESIAN_POINT ( 'NONE',  ( -4.458734124999999437, 23.35416666803226349, -2.574251347313719407 ) ) ;
#7668=CARTESIAN_POINT ( 'NONE',  ( 2.500000000000002220, -63.66666666666666430, 4.330127018922192761 ) ) ;
#7669=DIRECTION ( 'NONE',  ( 0.000000000000000000, 0.000000000000000000, 1.000000000000000000 ) ) ;
#7672=CARTESIAN_POINT ( 'NONE',  ( -5.000000000000000000, -61.95833333060213732, -2.886751345948128211 ) ) ;
#7673=CARTESIAN_POINT ( 'NONE',  ( 1.975475456537005874E-15, 9.250000000000000000, 5.000000000000000000 ) ) ;
#7674=CARTESIAN_POINT ( 'NONE',  ( -2.499999999999996447, -108.7083333306021444, 4.330127018922195425 ) ) ;
#7679=EDGE_CURVE ( 'NONE', #43327, #11325, #44337, .T. ) ;
#7688=CARTESIAN_POINT ( 'NONE',  ( -4.458734124999999437, -52.64583333196773651, -2.574251347313719407 ) ) ;
#7695=VECTOR ( 'NONE', #640, 1000.000000000000000 ) ;
#7700=CARTESIAN_POINT ( 'NONE',  ( 2.229367062499998831, -100.8958333319677365, -3.861377020970580887 ) ) ;
#7701=CARTESIAN_POINT ( 'NONE',  ( 5.000000000000000000, -2.500000000000002220, -6.123233995736766282E-16 ) ) ;
#7706=CARTESIAN_POINT ( 'NONE',  ( 4.458734124999998549, -6.729166665301073103, -2.574251347313721627 ) ) ;
#7707=CARTESIAN_POINT ( 'NONE',  ( 4.458734125000000326, -94.14583333196772230, 2.574251347313718519 ) ) ;
#7709=CARTESIAN_POINT ( 'NONE',  ( 4.458734124999999437, -21.06249999863440436, -5.460374474430324690E-16 ) ) ;
#7714=CARTESIAN_POINT ( 'NONE',  ( -2.499999999999996447, 17.16666666666666430, 4.330127018922195425 ) ) ;
#7716=CARTESIAN_POINT ( 'NONE',  ( 4.458734124999998549, 10.02083333469892779, -2.574251347313721627 ) ) ;
#7718=CARTESIAN_POINT ( 'NONE',  ( 1.975475456537005874E-15, -80.74999999999998579, 5.000000000000000000 ) ) ;
#7719=FACE_OUTER_BOUND ( 'NONE', #31648, .T. ) ;
#7720=CARTESIAN_POINT ( 'NONE',  ( 2.499999999999998668, -92.33333333333334281, -4.330127018922193649 ) ) ;
#7721=CARTESIAN_POINT ( 'NONE',  ( -2.229367062500000163, -23.47916666530107221, -3.861377020970580443 ) ) ;
#7722=CARTESIAN_POINT ( 'NONE',  ( 4.458734124999999437, -72.06249999863439371, -5.460374474430324690E-16 ) ) ;
#7725=CARTESIAN_POINT ( 'NONE',  ( -5.000000000000000000, -1.958333330602145983, -2.886751345948128211 ) ) ;
#7726=CARTESIAN_POINT ( 'NONE',  ( 4.458734124999998549, 6.270833334698928674, -2.574251347313721627 ) ) ;
#7730=CARTESIAN_POINT ( 'NONE',  ( -3.152548672688508926E-16, -71.56249999863440792, -5.148502694627439702 ) ) ;
#7732=CARTESIAN_POINT ( 'NONE',  ( -4.999999999999999112, -1.916666666666663854, 2.886751345948131764 ) ) ;
#7734=CARTESIAN_POINT ( 'NONE',  ( 1.975475456537005874E-15, -61.62499999726880162, 5.000000000000000000 ) ) ;
#7735=CARTESIAN_POINT ( 'NONE',  ( 2.229367062499998831, -65.64583333196773651, -3.861377020970580887 ) ) ;
#7736=CARTESIAN_POINT ( 'NONE',  ( -5.000000000000000000, -98.87499999726881583, 0.000000000000000000 ) ) ;
#7741=CARTESIAN_POINT ( 'NONE',  ( -4.999999999999999112, -48.91666666666666430, 2.886751345948131764 ) ) ;
#7742=CARTESIAN_POINT ( 'NONE',  ( 7.204675194429079505E-15, 25.87500000273118062, -5.000000000000000000 ) ) ;
#7748=DIRECTION ( 'NONE',  ( 0.000000000000000000, 0.000000000000000000, 1.000000000000000000 ) ) ;
#7754=VERTEX_POINT ( 'NONE', #10007 ) ;
#7758=CARTESIAN_POINT ( 'NONE',  ( 9.457646018065525792E-16, -33.31249999863440792, 5.148502694627439702 ) ) ;
#7759=CARTESIAN_POINT ( 'NONE',  ( 2.500000000000002220, -10.66666666666666430, 4.330127018922192761 ) ) ;
#7767=CARTESIAN_POINT ( 'NONE',  ( 4.458734124999999437, -85.06249999863439371, -5.460374474430324690E-16 ) ) ;
#7770=( BOUNDED_CURVE ( )  B_SPLINE_CURVE ( 2, ( #52851, #42873, #12974, #8785, #17502, #27449, #23589, #43184, #57374 ),
 .UNSPECIFIED., .F., .F. ) 
 B_SPLINE_CURVE_WITH_KNOTS ( ( 3, 2, 2, 2, 3 ),
 ( 0.2482142857142857206, 0.2488095238095238138, 0.2500000000000000000, 0.2511904761904761862, 0.2517857142857142794 ),
 .UNSPECIFIED. ) 
 CURVE ( )  GEOMETRIC_REPRESENTATION_ITEM ( )  RATIONAL_B_SPLINE_CURVE ( ( 0.9330127018922194093, 0.9330127018922194093, 1.000000000000000000, 0.8660254037844387076, 1.000000000000000000, 0.8660254037844387076, 1.000000000000000000, 0.9330127018922194093, 0.9330127018922194093 ) ) 
 REPRESENTATION_ITEM ( '' )  );
#7773=ADVANCED_FACE ( 'NONE', ( #44412 ), #19656, .T. ) ;
#7774=CARTESIAN_POINT ( 'NONE',  ( 9.457646018065525792E-16, -37.06249999863440792, 5.148502694627439702 ) ) ;
#7775=CARTESIAN_POINT ( 'NONE',  ( -2.229367062500000163, -10.72916666530106866, -3.861377020970580443 ) ) ;
#7778=LINE ( 'NONE', #17740, #12268 ) ;
#7779=CARTESIAN_POINT ( 'NONE',  ( 3.044556291839386294E-14, 17.75000000000000355, -5.000000000000000000 ) ) ;
#7780=CARTESIAN_POINT ( 'NONE',  ( -2.229367062500000163, -7.729166665301073991, -3.861377020970580443 ) ) ;
#7781=CYLINDRICAL_SURFACE ( 'NONE', #34289, 5.000000000000000000 ) ;
#7785=CARTESIAN_POINT ( 'NONE',  ( 2.229367062500001939, 27.77083333469892779, 3.861377020970579999 ) ) ;
#7786=ORIENTED_EDGE ( 'NONE', *, *, #39305, .T. ) ;
#7787=CARTESIAN_POINT ( 'NONE',  ( -4.458734124999999437, -84.39583333196773651, -2.574251347313719407 ) ) ;
#7789=CARTESIAN_POINT ( 'NONE',  ( 4.458734124999998549, -10.72916666530106866, -2.574251347313721627 ) ) ;
#7790=CARTESIAN_POINT ( 'NONE',  ( 1.339745962155612702, -51.29465819873851729, -5.000000000000000000 ) ) ;
#7791=CARTESIAN_POINT ( 'NONE',  ( 5.000000000000000000, -48.41666666666666430, -2.886751345948130876 ) ) ;
#7794=CARTESIAN_POINT ( 'NONE',  ( -5.000000000000000000, -33.87499999726880873, 0.000000000000000000 ) ) ;
#7796=CARTESIAN_POINT ( 'NONE',  ( 1.975475456537005874E-15, -16.74999999999999645, 5.000000000000000000 ) ) ;
#7797=CARTESIAN_POINT ( 'NONE',  ( 2.229367062500001939, 25.02083333469892779, 3.861377020970579999 ) ) ;
#7800=CARTESIAN_POINT ( 'NONE',  ( 2.229367062499998831, -56.64583333196773651, -3.861377020970580887 ) ) ;
#7802=CARTESIAN_POINT ( 'NONE',  ( -1.339745962155610925, -17.79465819873852439, 5.000000000000000000 ) ) ;
#7803=CARTESIAN_POINT ( 'NONE',  ( 5.000000000000000888, 17.41666666666666430, 2.886751345948126879 ) ) ;
#7806=VECTOR ( 'NONE', #32542, 1000.000000000000000 ) ;
#7807=CARTESIAN_POINT ( 'NONE',  ( 4.458734124999998549, -48.72916666530107221, -2.574251347313721627 ) ) ;
#7808=CARTESIAN_POINT ( 'NONE',  ( 1.060575238724906964E-15, -81.62499999726881583, 5.773502691896257311 ) ) ;
#7811=CARTESIAN_POINT ( 'NONE',  ( 2.500000000000002220, -36.66666666666666430, 4.330127018922192761 ) ) ;
#7812=CARTESIAN_POINT ( 'NONE',  ( -2.229367062499996610, -85.39583333196773651, 3.861377020970582219 ) ) ;
#7814=CARTESIAN_POINT ( 'NONE',  ( -5.000000000000000000, -32.00000000000000000, 0.000000000000000000 ) ) ;
#7815=ORIENTED_EDGE ( 'NONE', *, *, #31398, .F. ) ;
#7818=CARTESIAN_POINT ( 'NONE',  ( 4.458734124999999437, -97.81249999863440792, -5.460374474430324690E-16 ) ) ;
#7819=CARTESIAN_POINT ( 'NONE',  ( -4.458734124999999437, 15.43750000136559386, 0.000000000000000000 ) ) ;
#7820=CARTESIAN_POINT ( 'NONE',  ( 2.500000000000002220, 18.45833333606451632, 4.330127018922192761 ) ) ;
#7821=DIRECTION ( 'NONE',  ( -0.000000000000000000, 1.000000000000000000, -0.000000000000000000 ) ) ;
#7825=CARTESIAN_POINT ( 'NONE',  ( 5.000000000000000000, -61.29166666393548013, -2.886751345948130876 ) ) ;
#7826=CARTESIAN_POINT ( 'NONE',  ( 5.000000000000000000, -82.41666666666665719, -2.886751345948129988 ) ) ;
#7828=CARTESIAN_POINT ( 'NONE',  ( 1.975475456537005874E-15, -40.62499999726879452, 5.000000000000000000 ) ) ;
#7829=CARTESIAN_POINT ( 'NONE',  ( 2.499999999999998668, -63.33333333333332149, -4.330127018922193649 ) ) ;
#7830=CARTESIAN_POINT ( 'NONE',  ( -1.339745962155599601, 17.91965820146970501, -5.000000000000007994 ) ) ;
#7833=CARTESIAN_POINT ( 'NONE',  ( -1.339745962155613812, -43.20534180126148271, -5.000000000000000000 ) ) ;
#7834=CARTESIAN_POINT ( 'NONE',  ( -3.152548672688508926E-16, -19.81249999863440436, -5.148502694627439702 ) ) ;
#7835=CARTESIAN_POINT ( 'NONE',  ( 1.339745962155612702, -107.1696581960073189, -5.000000000000000000 ) ) ;
#7844=VERTEX_POINT ( 'NONE', #5504 ) ;
#7845=CARTESIAN_POINT ( 'NONE',  ( 9.457646018065525792E-16, -66.31249999863440792, 5.148502694627439702 ) ) ;
#7848=ORIENTED_EDGE ( 'NONE', *, *, #43115, .T. ) ;
#7854=ORIENTED_EDGE ( 'NONE', *, *, #10968, .F. ) ;
#7855=CARTESIAN_POINT ( 'NONE',  ( 5.000000000000000000, -45.41666666666665719, -2.886751345948130876 ) ) ;
#7856=CARTESIAN_POINT ( 'NONE',  ( 4.458734125000001214, 10.10416666803226171, 2.574251347313718519 ) ) ;
#7861=EDGE_LOOP ( 'NONE', ( #46627, #11784, #26267, #6913, #29257, #27467 ) ) ;
#7862=CARTESIAN_POINT ( 'NONE',  ( 2.229367062500001939, -69.97916666530107932, 3.861377020970579999 ) ) ;
#7863=EDGE_CURVE ( 'NONE', #41928, #19133, #42663, .T. ) ;
#7865=CARTESIAN_POINT ( 'NONE',  ( -2.229367062499996610, 9.854166668032261711, 3.861377020970582219 ) ) ;
#7866=( BOUNDED_CURVE ( )  B_SPLINE_CURVE ( 2, ( #36668, #6769, #16417, #31200, #61444, #7725, #7090, #1639, #56297 ),
 .UNSPECIFIED., .F., .F. ) 
 B_SPLINE_CURVE_WITH_KNOTS ( ( 3, 2, 2, 2, 3 ),
 ( 0.2196428571428571397, 0.2202380952380952328, 0.2214285714285714191, 0.2226190476190476053, 0.2232142857142857262 ),
 .UNSPECIFIED. ) 
 CURVE ( )  GEOMETRIC_REPRESENTATION_ITEM ( )  RATIONAL_B_SPLINE_CURVE ( ( 0.9330127018922194093, 0.9330127018922194093, 1.000000000000000000, 0.8660254037844387076, 1.000000000000000000, 0.8660254037844387076, 1.000000000000000000, 0.9330127018922178550, 0.9330127018922194093 ) ) 
 REPRESENTATION_ITEM ( '' )  );
#7867=CARTESIAN_POINT ( 'NONE',  ( -4.999999999999998224, -88.91666666666667140, 2.886751345948131764 ) ) ;
#7868=CARTESIAN_POINT ( 'NONE',  ( -4.458734124999998549, -61.47916666530107221, 2.574251347313722516 ) ) ;
#7869=CARTESIAN_POINT ( 'NONE',  ( -4.999999999999999112, -20.79166666393548013, 2.886751345948131764 ) ) ;
#7871=FACE_OUTER_BOUND ( 'NONE', #44717, .T. ) ;
#7873=CARTESIAN_POINT ( 'NONE',  ( 2.499999999999998668, -65.33333333333332860, -4.330127018922193649 ) ) ;
#7874=CARTESIAN_POINT ( 'NONE',  ( 2.229367062500001939, -39.97916666530107221, 3.861377020970579999 ) ) ;
#7875=EDGE_CURVE ( 'NONE', #52469, #4573, #44719, .T. ) ;
#7876=CARTESIAN_POINT ( 'NONE',  ( 2.229367062500001939, -19.22916666530106866, 3.861377020970579999 ) ) ;
#7878=CARTESIAN_POINT ( 'NONE',  ( -2.499999999999996447, -101.8333333333333286, 4.330127018922195425 ) ) ;
#7879=CARTESIAN_POINT ( 'NONE',  ( -2.229367062499996610, -110.1458333319677365, 3.861377020970582219 ) ) ;
#7881=VERTEX_POINT ( 'NONE', #20949 ) ;
#7882=CARTESIAN_POINT ( 'NONE',  ( -2.229367062500000163, -108.7291666653010651, -3.861377020970580443 ) ) ;
#7883=CARTESIAN_POINT ( 'NONE',  ( -4.458734124999999437, -33.39583333196772941, -2.574251347313719407 ) ) ;
#7884=CARTESIAN_POINT ( 'NONE',  ( -5.000000000000000000, -60.95833333060214443, -2.886751345948128211 ) ) ;
#7887=CARTESIAN_POINT ( 'NONE',  ( -4.458734124999997661, -28.22916666530107221, 2.574251347313722516 ) ) ;
#7888=CARTESIAN_POINT ( 'NONE',  ( 4.458734124999999437, -67.06249999863440792, -5.460374474430324690E-16 ) ) ;
#7892=CARTESIAN_POINT ( 'NONE',  ( -2.499999999999996447, -18.83333333333333215, 4.330127018922195425 ) ) ;
#7894=ORIENTED_EDGE ( 'NONE', *, *, #55866, .F. ) ;
#7898=DIRECTION ( 'NONE',  ( -0.000000000000000000, 1.000000000000000000, -0.000000000000000000 ) ) ;
#7901=CARTESIAN_POINT ( 'NONE',  ( 1.339745962155612702, 25.70534180126147916, -5.000000000000000000 ) ) ;
#7903=CARTESIAN_POINT ( 'NONE',  ( -6.972266317189433020E-16, -52.12499999726880873, -5.000000000000000000 ) ) ;
#7905=CARTESIAN_POINT ( 'NONE',  ( 1.975475456537005874E-15, -60.75000000000000000, 5.000000000000000000 ) ) ;
#7909=ORIENTED_EDGE ( 'NONE', *, *, #37702, .T. ) ;
#7910=CARTESIAN_POINT ( 'NONE',  ( 0.000000000000000000, -120.0000000000000000, 0.000000000000000000 ) ) ;
#7914=VECTOR ( 'NONE', #41713, 1000.000000000000000 ) ;
#7916=ORIENTED_EDGE ( 'NONE', *, *, #37869, .F. ) ;
#7920=CARTESIAN_POINT ( 'NONE',  ( -1.339745962155610925, -11.79465819873851906, 5.000000000000000000 ) ) ;
#7928=EDGE_CURVE ( 'NONE', #13658, #49915, #21257, .T. ) ;
#7929=CARTESIAN_POINT ( 'NONE',  ( 4.458734124999999437, -82.81249999863440792, -5.460374474430324690E-16 ) ) ;
#7930=CARTESIAN_POINT ( 'NONE',  ( 4.458734124999999437, 24.18750000136559564, -5.460374474430324690E-16 ) ) ;
#7933=VERTEX_POINT ( 'NONE', #59876 ) ;
#7939=CARTESIAN_POINT ( 'NONE',  ( 4.458734125000000326, -54.89583333196774362, 2.574251347313718519 ) ) ;
#7940=CARTESIAN_POINT ( 'NONE',  ( 1.339745962155612702, 10.70534180126147739, -5.000000000000000000 ) ) ;
#7941=CARTESIAN_POINT ( 'NONE',  ( 4.458734125000001214, 21.10416666803226349, 2.574251347313718519 ) ) ;
#7943=CARTESIAN_POINT ( 'NONE',  ( 2.500000000000002220, -106.6666666666666572, 4.330127018922192761 ) ) ;
#7945=CARTESIAN_POINT ( 'NONE',  ( -3.152548672688508926E-16, -45.81249999863440081, -5.148502694627439702 ) ) ;
#7946=CARTESIAN_POINT ( 'NONE',  ( -5.000000000000000000, 0.1250000027311869155, 0.000000000000000000 ) ) ;
#7947=LINE ( 'NONE', #27550, #16077 ) ;
#7948=EDGE_CURVE ( 'NONE', #51032, #3809, #50848, .T. ) ;
#7949=DIRECTION ( 'NONE',  ( 0.000000000000000000, 0.000000000000000000, 1.000000000000000000 ) ) ;
#7952=CARTESIAN_POINT ( 'NONE',  ( -2.229367062499996610, -100.1458333319677365, 3.861377020970582219 ) ) ;
#7953=CARTESIAN_POINT ( 'NONE',  ( -2.229367062499996610, -6.395833331967741842, 3.861377020970582219 ) ) ;
#7955=CARTESIAN_POINT ( 'NONE',  ( -5.000000000000000000, -85.95833333060214443, -2.886751345948128211 ) ) ;
#7956=CARTESIAN_POINT ( 'NONE',  ( 2.229367062499998831, -92.64583333196773651, -3.861377020970580887 ) ) ;
#7957=EDGE_CURVE ( 'NONE', #34574, #52846, #53739, .T. ) ;
#7959=CARTESIAN_POINT ( 'NONE',  ( 9.457646018065525792E-16, -86.31249999863440792, 5.148502694627439702 ) ) ;
#7962=AXIS2_PLACEMENT_3D ( 'NONE', #30879, #20276, #1955 ) ;
#7965=CARTESIAN_POINT ( 'NONE',  ( 4.458734124999998549, -10.72916666530106866, -2.574251347313721627 ) ) ;
#7966=CARTESIAN_POINT ( 'NONE',  ( 4.458734124999998549, 15.02083333469892601, -2.574251347313721627 ) ) ;
#7967=CARTESIAN_POINT ( 'NONE',  ( 4.458734124999998549, -54.97916666530107221, -2.574251347313721627 ) ) ;
#7970=CARTESIAN_POINT ( 'NONE',  ( -5.000000000000000000, -39.08333333333332860, -2.886751345948128211 ) ) ;
#7975=DIRECTION ( 'NONE',  ( -0.000000000000000000, 1.000000000000000000, -0.000000000000000000 ) ) ;
#7976=CARTESIAN_POINT ( 'NONE',  ( -2.229367062499996610, -78.14583333196773651, 3.861377020970582219 ) ) ;
#7977=CARTESIAN_POINT ( 'NONE',  ( 4.458734124999999437, 26.93750000136559564, -5.460374474430324690E-16 ) ) ;
#7981=CARTESIAN_POINT ( 'NONE',  ( 6.123233995736766282E-16, -120.0000000000000000, -5.000000000000000000 ) ) ;
#7983=CARTESIAN_POINT ( 'NONE',  ( -2.499999999999996447, -64.83333333333332860, 4.330127018922195425 ) ) ;
#7986=ORIENTED_EDGE ( 'NONE', *, *, #53178, .T. ) ;
#7994=ORIENTED_EDGE ( 'NONE', *, *, #3657, .T. ) ;
#7997=EDGE_LOOP ( 'NONE', ( #47229, #56548, #6979, #55844 ) ) ;
#8000=CARTESIAN_POINT ( 'NONE',  ( -2.229367062500000163, -50.72916666530107221, -3.861377020970580443 ) ) ;
#8004=ORIENTED_EDGE ( 'NONE', *, *, #14116, .T. ) ;
#8006=VECTOR ( 'NONE', #19017, 1000.000000000000000 ) ;
#8009=DIRECTION ( 'NONE',  ( -0.000000000000000000, 1.000000000000000000, -0.000000000000000000 ) ) ;
#8012=CARTESIAN_POINT ( 'NONE',  ( 9.457646018065525792E-16, -101.3124999986344079, 5.148502694627439702 ) ) ;
#8017=CARTESIAN_POINT ( 'NONE',  ( -2.229367062500000163, -6.479166665301072214, -3.861377020970580443 ) ) ;
#8019=CARTESIAN_POINT ( 'NONE',  ( -2.229367062500000163, -95.72916666530107932, -3.861377020970580443 ) ) ;
#8021=CARTESIAN_POINT ( 'NONE',  ( -2.229367062500000163, -22.72916666530107221, -3.861377020970580443 ) ) ;
#8026=FACE_OUTER_BOUND ( 'NONE', #10163, .T. ) ;
#8028=CARTESIAN_POINT ( 'NONE',  ( -2.229367062499996610, 8.604166668032261711, 3.861377020970582219 ) ) ;
#8029=ORIENTED_EDGE ( 'NONE', *, *, #60224, .F. ) ;
#8030=CARTESIAN_POINT ( 'NONE',  ( -6.972266317189433020E-16, -58.12499999726880162, -5.000000000000000000 ) ) ;
#8031=EDGE_CURVE ( 'NONE', #34574, #62346, #36367, .T. ) ;
#8033=CARTESIAN_POINT ( 'NONE',  ( -3.535250795749689387E-16, -91.25000000000000000, -5.773502691896257311 ) ) ;
#8034=CARTESIAN_POINT ( 'NONE',  ( -4.458734124999998549, -25.22916666530106866, 2.574251347313722516 ) ) ;
#8035=CARTESIAN_POINT ( 'NONE',  ( 1.975475456537005874E-15, -73.75000000000000000, 5.000000000000000000 ) ) ;
#8036=CARTESIAN_POINT ( 'NONE',  ( -2.229367062500000163, -72.72916666530107932, -3.861377020970580443 ) ) ;
#8040=EDGE_CURVE ( 'NONE', #42363, #2855, #51332, .T. ) ;
#8041=CARTESIAN_POINT ( 'NONE',  ( -2.229367062500000163, 1.520833334698927564, -3.861377020970580443 ) ) ;
#8042=CARTESIAN_POINT ( 'NONE',  ( 6.123233995736766282E-16, -120.0000000000000000, -5.000000000000000000 ) ) ;
#8043=DIRECTION ( 'NONE',  ( -0.000000000000000000, 1.000000000000000000, -0.000000000000000000 ) ) ;
#8045=CARTESIAN_POINT ( 'NONE',  ( -2.229367062499996610, -74.14583333196773651, 3.861377020970582219 ) ) ;
#8048=CARTESIAN_POINT ( 'NONE',  ( 2.500000000000002220, -3.666666666666665186, 4.330127018922192761 ) ) ;
#8051=CARTESIAN_POINT ( 'NONE',  ( 4.458734124999999437, -62.81249999863440792, -5.460374474430324690E-16 ) ) ;
#8052=CARTESIAN_POINT ( 'NONE',  ( -2.499999999999996447, -98.70833333060214443, 4.330127018922195425 ) ) ;
#8053=VECTOR ( 'NONE', #36163, 1000.000000000000000 ) ;
#8054=( BOUNDED_CURVE ( )  B_SPLINE_CURVE ( 2, ( #49891, #25455, #10975, #51188, #16448, #6487, #59892, #55376, #40879 ),
 .UNSPECIFIED., .F., .F. ) 
 B_SPLINE_CURVE_WITH_KNOTS ( ( 3, 2, 2, 2, 3 ),
 ( 0.3660714285714285476, 0.3666666666666666408, 0.3678571428571428825, 0.3690476190476190688, 0.3696428571428571619 ),
 .UNSPECIFIED. ) 
 CURVE ( )  GEOMETRIC_REPRESENTATION_ITEM ( )  RATIONAL_B_SPLINE_CURVE ( ( 0.9330127018922194093, 0.9330127018922194093, 1.000000000000000000, 0.8660254037844387076, 1.000000000000000000, 0.8660254037844387076, 1.000000000000000000, 0.9330127018922194093, 0.9330127018922194093 ) ) 
 REPRESENTATION_ITEM ( '' )  );
#8057=CARTESIAN_POINT ( 'NONE',  ( -2.229367062500000163, -104.7291666653010651, -3.861377020970580443 ) ) ;
#8059=CARTESIAN_POINT ( 'NONE',  ( -2.500000000000000444, -51.16666666666666430, -4.330127018922193649 ) ) ;
#8060=CARTESIAN_POINT ( 'NONE',  ( -4.999999999999998224, 27.08333333333333215, 2.886751345948131764 ) ) ;
#8062=VERTEX_POINT ( 'NONE', #3857 ) ;
#8063=CARTESIAN_POINT ( 'NONE',  ( -2.229367062499996610, -110.1458333319677365, 3.861377020970582219 ) ) ;
#8064=CARTESIAN_POINT ( 'NONE',  ( -6.972266317189433020E-16, -100.1249999972688016, -5.000000000000000000 ) ) ;
#8068=( BOUNDED_CURVE ( )  B_SPLINE_CURVE ( 2, ( #60282, #55128, #60917, #2071, #35194, #11055, #10741, #30349, #30678 ),
 .UNSPECIFIED., .F., .F. ) 
 B_SPLINE_CURVE_WITH_KNOTS ( ( 3, 2, 2, 2, 3 ),
 ( 0.001785714285714286092, 0.002380952380952381167, 0.003571428571428571317, 0.004761904761904762334, 0.005357142857142858060 ),
 .UNSPECIFIED. ) 
 CURVE ( )  GEOMETRIC_REPRESENTATION_ITEM ( )  RATIONAL_B_SPLINE_CURVE ( ( 0.9330127018922194093, 0.9330127018922194093, 1.000000000000000000, 0.8660254037844387076, 1.000000000000000000, 0.8660254037844387076, 1.000000000000000000, 0.9330127018922191873, 0.9330127018922192983 ) ) 
 REPRESENTATION_ITEM ( '' )  );
#8072=ORIENTED_EDGE ( 'NONE', *, *, #17948, .T. ) ;
#8079=CARTESIAN_POINT ( 'NONE',  ( 4.458734124999999437, -38.06249999863440792, -5.460374474430324690E-16 ) ) ;
#8080=CARTESIAN_POINT ( 'NONE',  ( -2.499999999999996447, -10.70833333060214621, 4.330127018922195425 ) ) ;
#8083=CARTESIAN_POINT ( 'NONE',  ( -1.339745962155610925, -29.79465819873851729, 5.000000000000000000 ) ) ;
#8087=CARTESIAN_POINT ( 'NONE',  ( -6.972266317189433020E-16, -47.25000000000000000, -5.000000000000000000 ) ) ;
#8088=CARTESIAN_POINT ( 'NONE',  ( -4.458734124999999437, -85.64583333196773651, -2.574251347313719407 ) ) ;
#8092=AXIS2_PLACEMENT_3D ( 'NONE', #59387, #53604, #54563 ) ;
#8095=CARTESIAN_POINT ( 'NONE',  ( -4.458734124999999437, -7.645833331967735624, -2.574251347313719407 ) ) ;
#8096=ORIENTED_EDGE ( 'NONE', *, *, #14246, .T. ) ;
#8098=DIRECTION ( 'NONE',  ( 0.000000000000000000, 0.000000000000000000, 1.000000000000000000 ) ) ;
#8099=CARTESIAN_POINT ( 'NONE',  ( -3.152548672688508926E-16, -5.812499998634404363, -5.148502694627439702 ) ) ;
#8104=CARTESIAN_POINT ( 'NONE',  ( -2.229367062499996610, 25.60416666803225993, 3.861377020970582219 ) ) ;
#8106=CARTESIAN_POINT ( 'NONE',  ( -2.229367062499996610, -90.14583333196773651, 3.861377020970582219 ) ) ;
#8108=CARTESIAN_POINT ( 'NONE',  ( -2.229367062500000163, -8.479166665301073991, -3.861377020970580443 ) ) ;
#8110=DIRECTION ( 'NONE',  ( -0.000000000000000000, 1.000000000000000000, -0.000000000000000000 ) ) ;
#8111=DIRECTION ( 'NONE',  ( 0.000000000000000000, 0.000000000000000000, 1.000000000000000000 ) ) ;
#8112=CARTESIAN_POINT ( 'NONE',  ( 1.060575238724906964E-15, -37.62499999726881583, 5.773502691896257311 ) ) ;
#8113=CARTESIAN_POINT ( 'NONE',  ( 0.000000000000000000, -120.0000000000000000, 0.000000000000000000 ) ) ;
#8114=CARTESIAN_POINT ( 'NONE',  ( -2.229367062499996610, 19.85416666803225993, 3.861377020970582219 ) ) ;
#8115=CARTESIAN_POINT ( 'NONE',  ( -2.499999999999996447, -97.70833333060213022, 4.330127018922195425 ) ) ;
#8117=CARTESIAN_POINT ( 'NONE',  ( 4.458734124999998549, -56.72916666530107932, -2.574251347313721627 ) ) ;
#8119=( BOUNDED_CURVE ( )  B_SPLINE_CURVE ( 2, ( #62410, #56642, #12556, #13516, #8678, #32814, #56951, #46980, #2928 ),
 .UNSPECIFIED., .F., .F. ) 
 B_SPLINE_CURVE_WITH_KNOTS ( ( 3, 2, 2, 2, 3 ),
 ( 0.8874999999999999556, 0.8880952380952380487, 0.8892857142857142350, 0.8904761904761904212, 0.8910714285714286254 ),
 .UNSPECIFIED. ) 
 CURVE ( )  GEOMETRIC_REPRESENTATION_ITEM ( )  RATIONAL_B_SPLINE_CURVE ( ( 0.9330127018922194093, 0.9330127018922194093, 1.000000000000000000, 0.8660254037844387076, 1.000000000000000000, 0.8660254037844387076, 1.000000000000000000, 0.9330127018922130810, 0.9330127018922194093 ) ) 
 REPRESENTATION_ITEM ( '' )  );
#8121=CARTESIAN_POINT ( 'NONE',  ( -2.500000000000000444, 12.83333333333333215, -4.330127018922193649 ) ) ;
#8124=CARTESIAN_POINT ( 'NONE',  ( -4.458734124999998549, -50.22916666530107221, 2.574251347313722516 ) ) ;
#8125=CARTESIAN_POINT ( 'NONE',  ( -5.000000000000000000, -83.87499999726880162, 0.000000000000000000 ) ) ;
#8129=CARTESIAN_POINT ( 'NONE',  ( -4.458734124999999437, -85.56249999863439371, 0.000000000000000000 ) ) ;
#8131=CARTESIAN_POINT ( 'NONE',  ( -2.499999999999996447, -33.83333333333332860, 4.330127018922195425 ) ) ;
#8136=CARTESIAN_POINT ( 'NONE',  ( 2.229367062500001939, -93.97916666530106511, 3.861377020970579999 ) ) ;
#8137=CARTESIAN_POINT ( 'NONE',  ( -4.458734124999999437, 7.437500001365594748, 0.000000000000000000 ) ) ;
#8139=CARTESIAN_POINT ( 'NONE',  ( -2.500000000000000444, 11.95833333606451809, -4.330127018922193649 ) ) ;
#8140=CARTESIAN_POINT ( 'NONE',  ( -1.339745962155610925, -43.66965819600732601, 5.000000000000000000 ) ) ;
#8142=EDGE_CURVE ( 'NONE', #35996, #18224, #60348, .T. ) ;
#8143=AXIS2_PLACEMENT_3D ( 'NONE', #43885, #39069, #58698 ) ;
#8146=CARTESIAN_POINT ( 'NONE',  ( -3.535250795749689387E-16, -79.25000000000000000, -5.773502691896257311 ) ) ;
#8149=CARTESIAN_POINT ( 'NONE',  ( -2.499999999999996447, -12.70833333060214798, 4.330127018922195425 ) ) ;
#8152=CARTESIAN_POINT ( 'NONE',  ( 1.339745962155612702, -107.2946581987385315, -5.000000000000000000 ) ) ;
#8155=CARTESIAN_POINT ( 'NONE',  ( -2.229367062499996610, -22.39583333196773651, 3.861377020970582219 ) ) ;
#8163=ORIENTED_EDGE ( 'NONE', *, *, #20453, .F. ) ;
#8166=CARTESIAN_POINT ( 'NONE',  ( -4.458734124999998549, -66.47916666530106511, 2.574251347313722516 ) ) ;
#8169=ORIENTED_EDGE ( 'NONE', *, *, #43621, .T. ) ;
#8175=CARTESIAN_POINT ( 'NONE',  ( 4.458734124999998549, 7.270833334698928674, -2.574251347313721627 ) ) ;
#8179=ORIENTED_EDGE ( 'NONE', *, *, #36256, .F. ) ;
#8180=CARTESIAN_POINT ( 'NONE',  ( -4.458734124999997661, -72.22916666530107932, 2.574251347313722516 ) ) ;
#8182=CARTESIAN_POINT ( 'NONE',  ( -4.458734124999999437, 5.687500001365592972, 0.000000000000000000 ) ) ;
#8185=CARTESIAN_POINT ( 'NONE',  ( 4.458734125000001214, -62.14583333196774362, 2.574251347313718519 ) ) ;
#8186=CARTESIAN_POINT ( 'NONE',  ( -3.535250795749689387E-16, -21.12499999726881228, -5.773502691896257311 ) ) ;
#8188=LINE ( 'NONE', #46155, #22418 ) ;
#8191=CARTESIAN_POINT ( 'NONE',  ( 4.458734124999998549, -42.72916666530107221, -2.574251347313721627 ) ) ;
#8192=CARTESIAN_POINT ( 'NONE',  ( -4.458734124999999437, -22.56249999863440436, 0.000000000000000000 ) ) ;
#8195=CARTESIAN_POINT ( 'NONE',  ( 4.458734124999998549, -108.7291666653010651, -2.574251347313721627 ) ) ;
#8198=CARTESIAN_POINT ( 'NONE',  ( 4.458734124999999437, -109.0624999986343937, -5.460374474430324690E-16 ) ) ;
#8199=CARTESIAN_POINT ( 'NONE',  ( 9.457646018065525792E-16, -32.06249999863440792, 5.148502694627439702 ) ) ;
#8200=CARTESIAN_POINT ( 'NONE',  ( 5.000000000000000888, -68.45833333060214443, 2.886751345948126879 ) ) ;
#8203=CARTESIAN_POINT ( 'NONE',  ( 2.229367062499998831, -27.64583333196774007, -3.861377020970580887 ) ) ;
#8204=CARTESIAN_POINT ( 'NONE',  ( 2.229367062499998831, -70.89583333196773651, -3.861377020970580887 ) ) ;
#8208=CARTESIAN_POINT ( 'NONE',  ( 1.339745962155612702, -5.169658196007333117, -5.000000000000000000 ) ) ;
#8209=CARTESIAN_POINT ( 'NONE',  ( 2.500000000000002220, -16.66666666666666430, 4.330127018922192761 ) ) ;
#8212=LINE ( 'NONE', #37170, #54307 ) ;
#8214=CARTESIAN_POINT ( 'NONE',  ( -2.500000000000000444, -3.041666663935477910, -4.330127018922193649 ) ) ;
#8215=CARTESIAN_POINT ( 'NONE',  ( -2.500000000000000444, -1.166666666666666519, -4.330127018922193649 ) ) ;
#8218=CARTESIAN_POINT ( 'NONE',  ( 5.000000000000000000, -76.29166666393547303, -2.886751345948130876 ) ) ;
#8220=CARTESIAN_POINT ( 'NONE',  ( 1.975475456537005874E-15, -51.62499999726880873, 5.000000000000000000 ) ) ;
#8221=CARTESIAN_POINT ( 'NONE',  ( 5.000000000000000000, -14.41666666666666785, -2.886751345948130876 ) ) ;
#8223=ORIENTED_EDGE ( 'NONE', *, *, #10605, .T. ) ;
#8224=ORIENTED_EDGE ( 'NONE', *, *, #42758, .T. ) ;
#8229=VECTOR ( 'NONE', #45713, 1000.000000000000000 ) ;
#8232=ORIENTED_EDGE ( 'NONE', *, *, #2887, .T. ) ;
#8234=EDGE_CURVE ( 'NONE', #37866, #31992, #42295, .T. ) ;
#8236=CARTESIAN_POINT ( 'NONE',  ( 1.339745962155612702, -53.29465819873850307, -5.000000000000000000 ) ) ;
#8242=ORIENTED_EDGE ( 'NONE', *, *, #4501, .F. ) ;
#8245=CARTESIAN_POINT ( 'NONE',  ( 9.457646018065525792E-16, -85.06249999863440792, 5.148502694627439702 ) ) ;
#8246=CARTESIAN_POINT ( 'NONE',  ( -2.229367062499996610, 23.85416666803225993, 3.861377020970582219 ) ) ;
#8248=ORIENTED_EDGE ( 'NONE', *, *, #20126, .T. ) ;
#8253=DIRECTION ( 'NONE',  ( -0.000000000000000000, 1.000000000000000000, -0.000000000000000000 ) ) ;
#8256=CARTESIAN_POINT ( 'NONE',  ( -4.458734124999999437, -52.39583333196773651, -2.574251347313719407 ) ) ;
#8257=CARTESIAN_POINT ( 'NONE',  ( 2.229367062499998831, 23.35416666803225993, -3.861377020970580887 ) ) ;
#8258=CARTESIAN_POINT ( 'NONE',  ( -2.499999999999996447, -107.8333333333333428, 4.330127018922195425 ) ) ;
#8259=CARTESIAN_POINT ( 'NONE',  ( -5.000000000000000000, -44.08333333333333570, -2.886751345948128211 ) ) ;
#8260=CARTESIAN_POINT ( 'NONE',  ( 9.457646018065525792E-16, -43.31249999863440792, 5.148502694627439702 ) ) ;
#8262=CARTESIAN_POINT ( 'NONE',  ( -5.000000000000000000, -5.874999997268811391, 0.000000000000000000 ) ) ;
#8266=CARTESIAN_POINT ( 'NONE',  ( -4.458734124999999437, -103.3124999986344079, 0.000000000000000000 ) ) ;
#8267=CARTESIAN_POINT ( 'NONE',  ( 4.458734125000000326, -5.145833331967740065, 2.574251347313718519 ) ) ;
#8268=ORIENTED_EDGE ( 'NONE', *, *, #7152, .F. ) ;
#8269=CARTESIAN_POINT ( 'NONE',  ( -2.229367062500000163, -91.47916666530106511, -3.861377020970580443 ) ) ;
#8271=CARTESIAN_POINT ( 'NONE',  ( -3.152548672688508926E-16, -90.81249999863440792, -5.148502694627439702 ) ) ;
#8275=CARTESIAN_POINT ( 'NONE',  ( 4.458734124999998549, -13.72916666530107399, -2.574251347313721627 ) ) ;
#8276=CARTESIAN_POINT ( 'NONE',  ( 4.458734125000001214, 13.85416666803226171, 2.574251347313718519 ) ) ;
#8277=CARTESIAN_POINT ( 'NONE',  ( 4.458734124999999437, -56.06249999863440081, -5.460374474430324690E-16 ) ) ;
#8278=CYLINDRICAL_SURFACE ( 'NONE', #24380, 5.000000000000000000 ) ;
#8281=CARTESIAN_POINT ( 'NONE',  ( -6.972266317189433020E-16, -84.24999999999998579, -5.000000000000000000 ) ) ;
#8282=ORIENTED_EDGE ( 'NONE', *, *, #6766, .F. ) ;
#8285=CARTESIAN_POINT ( 'NONE',  ( 2.500000000000002220, 26.45833333606451632, 4.330127018922192761 ) ) ;
#8286=LINE ( 'NONE', #21893, #25476 ) ;
#8287=CARTESIAN_POINT ( 'NONE',  ( -3.152548672688508926E-16, -78.56249999863440792, -5.148502694627439702 ) ) ;
#8288=CARTESIAN_POINT ( 'NONE',  ( -3.152548672688508926E-16, 25.18750000136558853, -5.148502694627439702 ) ) ;
#8289=EDGE_CURVE ( 'NONE', #29366, #24051, #59970, .T. ) ;
#8293=CARTESIAN_POINT ( 'NONE',  ( -1.339745962155613812, 6.794658198738520838, -5.000000000000000000 ) ) ;
#8296=CARTESIAN_POINT ( 'NONE',  ( -5.000000000000000000, -68.08333333333332860, -2.886751345948128211 ) ) ;
#8297=( BOUNDED_CURVE ( )  B_SPLINE_CURVE ( 2, ( #21604, #27682, #27056, #17089, #42159, #36710, #18027, #11931, #32186 ),
 .UNSPECIFIED., .F., .F. ) 
 B_SPLINE_CURVE_WITH_KNOTS ( ( 3, 2, 2, 2, 3 ),
 ( 0.8339285714285714635, 0.8345238095238095566, 0.8357142857142857428, 0.8369047619047619291, 0.8375000000000000222 ),
 .UNSPECIFIED. ) 
 CURVE ( )  GEOMETRIC_REPRESENTATION_ITEM ( )  RATIONAL_B_SPLINE_CURVE ( ( 0.9330127018922194093, 0.9330127018922194093, 1.000000000000000000, 0.8660254037844387076, 1.000000000000000000, 0.8660254037844387076, 1.000000000000000000, 0.9330127018922194093, 0.9330127018922194093 ) ) 
 REPRESENTATION_ITEM ( '' )  );
#8300=CARTESIAN_POINT ( 'NONE',  ( 0.000000000000000000, -120.0000000000000000, 0.000000000000000000 ) ) ;
#8301=( BOUNDED_CURVE ( )  B_SPLINE_CURVE ( 2, ( #19496, #38790, #57807, #54229, #39111, #43311, #23399, #18860, #4701 ),
 .UNSPECIFIED., .F., .F. ) 
 B_SPLINE_CURVE_WITH_KNOTS ( ( 3, 2, 2, 2, 3 ),
 ( 0.6839285714285714413, 0.6845238095238095344, 0.6857142857142857206, 0.6869047619047619069, 0.6875000000000000000 ),
 .UNSPECIFIED. ) 
 CURVE ( )  GEOMETRIC_REPRESENTATION_ITEM ( )  RATIONAL_B_SPLINE_CURVE ( ( 0.9330127018922194093, 0.9330127018922194093, 1.000000000000000000, 0.8660254037844387076, 1.000000000000000000, 0.8660254037844387076, 1.000000000000000000, 0.9330127018922194093, 0.9330127018922194093 ) ) 
 REPRESENTATION_ITEM ( '' )  );
#8302=FACE_OUTER_BOUND ( 'NONE', #42062, .T. ) ;
#8303=DIRECTION ( 'NONE',  ( -0.000000000000000000, 1.000000000000000000, -0.000000000000000000 ) ) ;
#8306=EDGE_CURVE ( 'NONE', #35972, #37904, #3245, .T. ) ;
#8309=ORIENTED_EDGE ( 'NONE', *, *, #27600, .T. ) ;
#8311=ADVANCED_FACE ( 'NONE', ( #34058 ), #44333, .F. ) ;
#8316=VECTOR ( 'NONE', #18699, 1000.000000000000000 ) ;
#8317=CARTESIAN_POINT ( 'NONE',  ( 4.458734125000001214, -53.14583333196773651, 2.574251347313718519 ) ) ;
#8319=ORIENTED_EDGE ( 'NONE', *, *, #60942, .F. ) ;
#8327=CARTESIAN_POINT ( 'NONE',  ( -4.458734124999999437, -98.56249999863440792, 0.000000000000000000 ) ) ;
#8328=CARTESIAN_POINT ( 'NONE',  ( -1.339745962155610925, -68.66965819600733312, 5.000000000000000000 ) ) ;
#8329=( BOUNDED_CURVE ( )  B_SPLINE_CURVE ( 2, ( #12623, #32237, #27412, #47043, #2993, #22610, #28355, #13881, #23224 ),
 .UNSPECIFIED., .F., .F. ) 
 B_SPLINE_CURVE_WITH_KNOTS ( ( 3, 2, 2, 2, 3 ),
 ( 0.4732142857142856984, 0.4738095238095237915, 0.4749999999999999778, 0.4761904761904761640, 0.4767857142857143127 ),
 .UNSPECIFIED. ) 
 CURVE ( )  GEOMETRIC_REPRESENTATION_ITEM ( )  RATIONAL_B_SPLINE_CURVE ( ( 0.9330127018922194093, 0.9330127018922194093, 1.000000000000000000, 0.8660254037844387076, 1.000000000000000000, 0.8660254037844387076, 1.000000000000000000, 0.9330127018922163007, 0.9330127018922194093 ) ) 
 REPRESENTATION_ITEM ( '' )  );
#8333=CARTESIAN_POINT ( 'NONE',  ( -5.000000000000000000, 1.041666669397853351, -2.886751345948128211 ) ) ;
#8334=CARTESIAN_POINT ( 'NONE',  ( 2.229367062499998831, -9.645833331967738289, -3.861377020970580887 ) ) ;
#8335=CARTESIAN_POINT ( 'NONE',  ( 4.458734125000000326, -95.14583333196772230, 2.574251347313718519 ) ) ;
#8337=CARTESIAN_POINT ( 'NONE',  ( 2.229367062500001939, -27.22916666530106866, 3.861377020970579999 ) ) ;
#8341=CARTESIAN_POINT ( 'NONE',  ( 1.975475456537005874E-15, -21.62499999726880873, 5.000000000000000000 ) ) ;
#8342=DIRECTION ( 'NONE',  ( 0.000000000000000000, 0.000000000000000000, 1.000000000000000000 ) ) ;
#8344=( BOUNDED_CURVE ( )  B_SPLINE_CURVE ( 2, ( #26235, #59060, #31058, #50680, #35254, #54874, #6622, #49722, #20140 ),
 .UNSPECIFIED., .F., .F. ) 
 B_SPLINE_CURVE_WITH_KNOTS ( ( 3, 2, 2, 2, 3 ),
 ( 0.05178571428571428908, 0.05238095238095238221, 0.05357142857142856845, 0.05476190476190476164, 0.05535714285714286170 ),
 .UNSPECIFIED. ) 
 CURVE ( )  GEOMETRIC_REPRESENTATION_ITEM ( )  RATIONAL_B_SPLINE_CURVE ( ( 0.9330127018922194093, 0.9330127018922197424, 1.000000000000000000, 0.8660254037844387076, 1.000000000000000000, 0.8660254037844387076, 1.000000000000000000, 0.9330127018922189652, 0.9330127018922194093 ) ) 
 REPRESENTATION_ITEM ( '' )  );
#8345=CARTESIAN_POINT ( 'NONE',  ( -4.458734124999999437, 12.35416666803226171, -2.574251347313719407 ) ) ;
#8349=CARTESIAN_POINT ( 'NONE',  ( 5.000000000000000888, -90.58333333333334281, 2.886751345948126879 ) ) ;
#8350=CARTESIAN_POINT ( 'NONE',  ( -2.229367062500000163, -24.47916666530106866, -3.861377020970580443 ) ) ;
#8351=CARTESIAN_POINT ( 'NONE',  ( -4.458734124999998549, -78.47916666530107932, 2.574251347313722516 ) ) ;
#8355=CARTESIAN_POINT ( 'NONE',  ( -3.152548672688508926E-16, 2.437500001365593860, -5.148502694627439702 ) ) ;
#8357=FACE_OUTER_BOUND ( 'NONE', #53938, .T. ) ;
#8359=CARTESIAN_POINT ( 'NONE',  ( -4.458734124999999437, -70.31249999863439371, 0.000000000000000000 ) ) ;
#8361=CARTESIAN_POINT ( 'NONE',  ( 5.000000000000000888, -4.583333333333334814, 2.886751345948126879 ) ) ;
#8364=AXIS2_PLACEMENT_3D ( 'NONE', #23248, #7516, #52526 ) ;
#8365=CARTESIAN_POINT ( 'NONE',  ( -4.458734124999998549, -64.22916666530107932, 2.574251347313722516 ) ) ;
#8366=CARTESIAN_POINT ( 'NONE',  ( 2.500000000000002220, -99.54166666393545881, 4.330127018922192761 ) ) ;
#8370=CARTESIAN_POINT ( 'NONE',  ( 5.000000000000000888, 9.541666669397852019, 2.886751345948126879 ) ) ;
#8371=CARTESIAN_POINT ( 'NONE',  ( -4.458734124999999437, -108.6458333319677365, -2.574251347313719407 ) ) ;
#8373=CARTESIAN_POINT ( 'NONE',  ( -2.500000000000000444, -54.16666666666667140, -4.330127018922193649 ) ) ;
#8374=CARTESIAN_POINT ( 'NONE',  ( 1.339745962155612702, -72.16965819600733312, -5.000000000000000000 ) ) ;
#8376=ORIENTED_EDGE ( 'NONE', *, *, #7957, .F. ) ;
#8383=CARTESIAN_POINT ( 'NONE',  ( -1.339745962155610925, -5.794658198738521726, 5.000000000000000000 ) ) ;
#8388=ORIENTED_EDGE ( 'NONE', *, *, #2963, .T. ) ;
#8391=EDGE_CURVE ( 'NONE', #46887, #26939, #38877, .T. ) ;
#8393=CARTESIAN_POINT ( 'NONE',  ( -4.458734124999998549, -37.47916666530107221, 2.574251347313722516 ) ) ;
#8397=ADVANCED_FACE ( 'NONE', ( #44015 ), #49172, .T. ) ;
#8402=EDGE_CURVE ( 'NONE', #15905, #1425, #48850, .T. ) ;
#8403=CARTESIAN_POINT ( 'NONE',  ( -2.500000000000000444, -25.04166666393547658, -4.330127018922193649 ) ) ;
#8404=CARTESIAN_POINT ( 'NONE',  ( -4.458734124999999437, -82.56249999863440792, 0.000000000000000000 ) ) ;
#8407=CARTESIAN_POINT ( 'NONE',  ( 5.000000000000000000, -43.50000000000000000, -6.123233995736766282E-16 ) ) ;
#8412=DIRECTION ( 'NONE',  ( -0.000000000000000000, 1.000000000000000000, -0.000000000000000000 ) ) ;
#8413=CARTESIAN_POINT ( 'NONE',  ( -4.458734124999999437, -14.64583333196773474, -2.574251347313719407 ) ) ;
#8417=CARTESIAN_POINT ( 'NONE',  ( 2.229367062500001939, 25.77083333469892779, 3.861377020970579999 ) ) ;
#8419=CARTESIAN_POINT ( 'NONE',  ( -2.229367062500000163, -94.47916666530106511, -3.861377020970580443 ) ) ;
#8420=CARTESIAN_POINT ( 'NONE',  ( 1.975475456537005874E-15, -30.74999999999999645, 5.000000000000000000 ) ) ;
#8422=CARTESIAN_POINT ( 'NONE',  ( 2.229367062500001939, -8.979166665301075767, 3.861377020970579999 ) ) ;
#8424=LINE ( 'NONE', #45831, #45826 ) ;
#8425=( BOUNDED_CURVE ( )  B_SPLINE_CURVE ( 2, ( #6094, #60450, #15734, #11848, #31467, #1917, #11221, #35351, #20884 ),
 .UNSPECIFIED., .F., .F. ) 
 B_SPLINE_CURVE_WITH_KNOTS ( ( 3, 2, 2, 2, 3 ),
 ( 0.6303571428571428381, 0.6309523809523809312, 0.6321428571428571175, 0.6333333333333333037, 0.6339285714285713969 ),
 .UNSPECIFIED. ) 
 CURVE ( )  GEOMETRIC_REPRESENTATION_ITEM ( )  RATIONAL_B_SPLINE_CURVE ( ( 0.9330127018922194093, 0.9330127018922194093, 1.000000000000000000, 0.8660254037844387076, 1.000000000000000000, 0.8660254037844387076, 1.000000000000000000, 0.9330127018922194093, 0.9330127018922194093 ) ) 
 REPRESENTATION_ITEM ( '' )  );
#8426=CARTESIAN_POINT ( 'NONE',  ( -5.000000000000000000, 14.91666666666666607, -2.886751345948128211 ) ) ;
#8427=CARTESIAN_POINT ( 'NONE',  ( 2.499999999999998668, -35.20833333060213732, -4.330127018922193649 ) ) ;
#8428=CARTESIAN_POINT ( 'NONE',  ( -6.972266317189433020E-16, -49.12499999726880162, -5.000000000000000000 ) ) ;
#8429=CARTESIAN_POINT ( 'NONE',  ( -2.229367062500000163, 16.52083333469892779, -3.861377020970580443 ) ) ;
#8432=CARTESIAN_POINT ( 'NONE',  ( -3.152548672688508926E-16, -55.56249999863440081, -5.148502694627439702 ) ) ;
#8435=CARTESIAN_POINT ( 'NONE',  ( -2.499999999999996447, 11.16666666666666430, 4.330127018922195425 ) ) ;
#8438=CARTESIAN_POINT ( 'NONE',  ( 4.458734124999998549, -47.72916666530106511, -2.574251347313721627 ) ) ;
#8439=CARTESIAN_POINT ( 'NONE',  ( 2.499999999999998668, -84.20833333060214443, -4.330127018922193649 ) ) ;
#8441=DIRECTION ( 'NONE',  ( 0.000000000000000000, 0.000000000000000000, 1.000000000000000000 ) ) ;
#8442=ADVANCED_FACE ( 'NONE', ( #40789 ), #5750, .T. ) ;
#8444=CARTESIAN_POINT ( 'NONE',  ( 2.229367062499998831, -90.89583333196773651, -3.861377020970580887 ) ) ;
#8446=CARTESIAN_POINT ( 'NONE',  ( 1.060575238724906964E-15, -34.75000000000000711, 5.773502691896257311 ) ) ;
#8448=ORIENTED_EDGE ( 'NONE', *, *, #12788, .F. ) ;
#8451=CARTESIAN_POINT ( 'NONE',  ( 4.458734124999999437, -94.81249999863440792, -5.460374474430324690E-16 ) ) ;
#8452=CARTESIAN_POINT ( 'NONE',  ( -2.229367062500000163, 8.270833334698926009, -3.861377020970580443 ) ) ;
#8453=CARTESIAN_POINT ( 'NONE',  ( -5.000000000000000000, 10.04166666939785202, -2.886751345948128211 ) ) ;
#8454=CARTESIAN_POINT ( 'NONE',  ( -1.339745962155610925, -28.66965819600733312, 5.000000000000000000 ) ) ;
#8457=CARTESIAN_POINT ( 'NONE',  ( 1.339745962155615144, -61.58034179853027723, 4.999999999999999112 ) ) ;
#8460=CARTESIAN_POINT ( 'NONE',  ( -4.999999999999998224, -25.79166666393547658, 2.886751345948131764 ) ) ;
#8462=CARTESIAN_POINT ( 'NONE',  ( -2.499999999999996447, -75.70833333060214443, 4.330127018922195425 ) ) ;
#8464=CARTESIAN_POINT ( 'NONE',  ( -4.458734124999999437, -17.64583333196773651, -2.574251347313719407 ) ) ;
#8474=ORIENTED_EDGE ( 'NONE', *, *, #24306, .F. ) ;
#8475=CARTESIAN_POINT ( 'NONE',  ( 4.458734125000001214, -70.14583333196773651, 2.574251347313718519 ) ) ;
#8480=CARTESIAN_POINT ( 'NONE',  ( -4.458734124999998549, 0.5208333346989265644, 2.574251347313722516 ) ) ;
#8482=CARTESIAN_POINT ( 'NONE',  ( -1.339745962155497683, -55.20534180126147561, -5.000000000000066613 ) ) ;
#8483=CARTESIAN_POINT ( 'NONE',  ( 4.458734124999998549, 2.270833334698928230, -2.574251347313721627 ) ) ;
#8486=CARTESIAN_POINT ( 'NONE',  ( 1.975475456537005874E-15, 16.24999999999999645, 5.000000000000000000 ) ) ;
#8488=( BOUNDED_CURVE ( )  B_SPLINE_CURVE ( 2, ( #39360, #48389, #14291, #49975, #15577, #45152, #11371, #1117, #16525 ),
 .UNSPECIFIED., .F., .F. ) 
 B_SPLINE_CURVE_WITH_KNOTS ( ( 3, 2, 2, 2, 3 ),
 ( 0.6089285714285714857, 0.6095238095238095788, 0.6107142857142857650, 0.6119047619047619513, 0.6125000000000000444 ),
 .UNSPECIFIED. ) 
 CURVE ( )  GEOMETRIC_REPRESENTATION_ITEM ( )  RATIONAL_B_SPLINE_CURVE ( ( 0.9330127018922194093, 0.9330127018922256266, 1.000000000000000000, 0.8660254037844387076, 1.000000000000000000, 0.8660254037844387076, 1.000000000000000000, 0.9330127018922194093, 0.9330127018922194093 ) ) 
 REPRESENTATION_ITEM ( '' )  );
#8490=CARTESIAN_POINT ( 'NONE',  ( 2.229367062499998831, -77.64583333196773651, -3.861377020970580887 ) ) ;
#8492=CARTESIAN_POINT ( 'NONE',  ( 4.458734124999998549, 7.270833334698928674, -2.574251347313721627 ) ) ;
#8493=CARTESIAN_POINT ( 'NONE',  ( -1.339745962155610925, -88.79465819873851729, 5.000000000000000000 ) ) ;
#8494=CARTESIAN_POINT ( 'NONE',  ( -2.229367062500000163, -62.72916666530106511, -3.861377020970580443 ) ) ;
#8495=CARTESIAN_POINT ( 'NONE',  ( 1.060575238724906964E-15, -22.62499999726881228, 5.773502691896257311 ) ) ;
#8496=FACE_OUTER_BOUND ( 'NONE', #9398, .T. ) ;
#8497=CARTESIAN_POINT ( 'NONE',  ( 1.339745962155612702, -42.16965819600732601, -5.000000000000000000 ) ) ;
#8501=CARTESIAN_POINT ( 'NONE',  ( -4.458734124999999437, -39.39583333196773651, -2.574251347313719407 ) ) ;
#8502=CARTESIAN_POINT ( 'NONE',  ( 4.458734125000000326, -28.14583333196774007, 2.574251347313718519 ) ) ;
#8504=CARTESIAN_POINT ( 'NONE',  ( 2.500000000000002220, 24.33333333333333215, 4.330127018922192761 ) ) ;
#8506=ORIENTED_EDGE ( 'NONE', *, *, #13449, .T. ) ;
#8507=CARTESIAN_POINT ( 'NONE',  ( 4.458734124999998549, -109.9791666653010793, -2.574251347313721627 ) ) ;
#8508=CARTESIAN_POINT ( 'NONE',  ( 4.458734124999999437, -31.81249999863440436, -5.460374474430324690E-16 ) ) ;
#8509=CARTESIAN_POINT ( 'NONE',  ( 2.499999999999998668, -70.20833333060214443, -4.330127018922193649 ) ) ;
#8512=CARTESIAN_POINT ( 'NONE',  ( 4.458734124999998549, -27.72916666530107221, -2.574251347313721627 ) ) ;
#8513=CARTESIAN_POINT ( 'NONE',  ( -4.458734124999999437, -75.56249999863440792, 0.000000000000000000 ) ) ;
#8518=CARTESIAN_POINT ( 'NONE',  ( 5.000000000000000000, -15.41666666666666963, -2.886751345948129988 ) ) ;
#8520=ORIENTED_EDGE ( 'NONE', *, *, #63627, .T. ) ;
#8521=CARTESIAN_POINT ( 'NONE',  ( 0.000000000000000000, -120.0000000000000000, 0.000000000000000000 ) ) ;
#8524=CARTESIAN_POINT ( 'NONE',  ( -2.499999999999996447, 25.29166666939785202, 4.330127018922195425 ) ) ;
#8532=ORIENTED_EDGE ( 'NONE', *, *, #1374, .F. ) ;
#8533=CARTESIAN_POINT ( 'NONE',  ( 5.000000000000000000, -12.49999999999999645, -6.123233995736766282E-16 ) ) ;
#8539=VERTEX_POINT ( 'NONE', #30175 ) ;
#8542=CARTESIAN_POINT ( 'NONE',  ( -6.972266317189433020E-16, -0.1249999972688142363, -5.000000000000000000 ) ) ;
#8543=CARTESIAN_POINT ( 'NONE',  ( -4.999999999999998224, -102.7916666639354730, 2.886751345948131764 ) ) ;
#8549=CARTESIAN_POINT ( 'NONE',  ( -3.152548672688508926E-16, -83.56249999863440792, -5.148502694627439702 ) ) ;
#8550=CARTESIAN_POINT ( 'NONE',  ( 9.457646018065525792E-16, 22.93750000136559919, 5.148502694627439702 ) ) ;
#8551=CARTESIAN_POINT ( 'NONE',  ( 2.499999999999998668, -12.20833333060214798, -4.330127018922193649 ) ) ;
#8552=ORIENTED_EDGE ( 'NONE', *, *, #13887, .F. ) ;
#8556=CARTESIAN_POINT ( 'NONE',  ( 5.000000000000000000, -88.41666666666665719, -2.886751345948130876 ) ) ;
#8559=CARTESIAN_POINT ( 'NONE',  ( -4.458734124999999437, -57.39583333196773651, -2.574251347313719407 ) ) ;
#8561=CARTESIAN_POINT ( 'NONE',  ( -4.458734124999998549, 25.77083333469892779, 2.574251347313722516 ) ) ;
#8565=CARTESIAN_POINT ( 'NONE',  ( -4.458734124999999437, -44.64583333196773651, -2.574251347313719407 ) ) ;
#8566=CARTESIAN_POINT ( 'NONE',  ( -4.999999999999999112, -2.791666663935477466, 2.886751345948131764 ) ) ;
#8567=CARTESIAN_POINT ( 'NONE',  ( 5.000000000000000000, -31.50000000000000000, -6.123233995736766282E-16 ) ) ;
#8570=CARTESIAN_POINT ( 'NONE',  ( 9.457646018065525792E-16, -101.0624999986344079, 5.148502694627439702 ) ) ;
#8571=CARTESIAN_POINT ( 'NONE',  ( 2.229367062500001939, -12.22916666530107044, 3.861377020970579999 ) ) ;
#8572=ORIENTED_EDGE ( 'NONE', *, *, #60231, .F. ) ;
#8574=CARTESIAN_POINT ( 'NONE',  ( -4.458734124999998549, -94.22916666530106511, 2.574251347313722516 ) ) ;
#8576=CARTESIAN_POINT ( 'NONE',  ( 2.229367062499998831, -89.89583333196773651, -3.861377020970580887 ) ) ;
#8577=CARTESIAN_POINT ( 'NONE',  ( -5.000000000000000000, -50.87499999726881583, 0.000000000000000000 ) ) ;
#8581=CARTESIAN_POINT ( 'NONE',  ( 9.457646018065525792E-16, -15.06249999863440259, 5.148502694627439702 ) ) ;
#8582=CARTESIAN_POINT ( 'NONE',  ( 2.229367062500001939, 12.77083333469892779, 3.861377020970579999 ) ) ;
#8583=EDGE_CURVE ( 'NONE', #45091, #8062, #55457, .T. ) ;
#8584=CARTESIAN_POINT ( 'NONE',  ( -2.229367062500000163, -54.72916666530107221, -3.861377020970580443 ) ) ;
#8589=VERTEX_POINT ( 'NONE', #6712 ) ;
#8594=CARTESIAN_POINT ( 'NONE',  ( 2.229367062499998831, -84.64583333196773651, -3.861377020970580887 ) ) ;
#8595=CARTESIAN_POINT ( 'NONE',  ( 4.458734125000001214, 24.85416666803225993, 2.574251347313718519 ) ) ;
#8596=EDGE_CURVE ( 'NONE', #49029, #53577, #52992, .T. ) ;
#8598=DIRECTION ( 'NONE',  ( 1.000000000000000000, 0.000000000000000000, -1.061635649774262664E-14 ) ) ;
#8601=CARTESIAN_POINT ( 'NONE',  ( -2.500000000000000444, -69.16666666666667140, -4.330127018922193649 ) ) ;
#8606=CARTESIAN_POINT ( 'NONE',  ( -6.972266317189433020E-16, -109.1249999972688016, -5.000000000000000000 ) ) ;
#8612=EDGE_CURVE ( 'NONE', #51084, #29252, #62032, .T. ) ;
#8620=CARTESIAN_POINT ( 'NONE',  ( -2.229367062500000163, -56.72916666530107221, -3.861377020970580443 ) ) ;
#8627=ORIENTED_EDGE ( 'NONE', *, *, #6629, .T. ) ;
#8629=CARTESIAN_POINT ( 'NONE',  ( 4.458734125000001214, -102.1458333319677365, 2.574251347313718519 ) ) ;
#8634=DIRECTION ( 'NONE',  ( -0.000000000000000000, 1.000000000000000000, -0.000000000000000000 ) ) ;
#8636=CARTESIAN_POINT ( 'NONE',  ( 4.458734124999998549, -9.729166665301068662, -2.574251347313721627 ) ) ;
#8637=CARTESIAN_POINT ( 'NONE',  ( 4.458734124999999437, -100.0624999986344079, -5.460374474430324690E-16 ) ) ;
#8639=CARTESIAN_POINT ( 'NONE',  ( -4.458734124999998549, -28.47916666530107221, 2.574251347313722516 ) ) ;
#8643=CARTESIAN_POINT ( 'NONE',  ( -1.339745962155610925, -90.79465819873853150, 5.000000000000000000 ) ) ;
#8644=CARTESIAN_POINT ( 'NONE',  ( 1.975475456537005874E-15, -33.75000000000000000, 5.000000000000000000 ) ) ;
#8646=CARTESIAN_POINT ( 'NONE',  ( -4.458734124999999437, 11.35416666803225993, -2.574251347313719407 ) ) ;
#8648=CARTESIAN_POINT ( 'NONE',  ( -5.926426369611017623E-15, 26.25000000000000000, 5.000000000000000000 ) ) ;
#8649=CARTESIAN_POINT ( 'NONE',  ( 5.000000000000000000, 2.583333333333333481, -2.886751345948130876 ) ) ;
#8650=CARTESIAN_POINT ( 'NONE',  ( 1.060575238724906964E-15, -90.75000000000000000, 5.773502691896257311 ) ) ;
#8651=CARTESIAN_POINT ( 'NONE',  ( 2.229367062500001939, -23.97916666530107577, 3.861377020970579999 ) ) ;
#8652=CARTESIAN_POINT ( 'NONE',  ( -4.999999999999998224, 7.208333336064517205, 2.886751345948131764 ) ) ;
#8653=CARTESIAN_POINT ( 'NONE',  ( 4.458734125000001214, -76.14583333196773651, 2.574251347313718519 ) ) ;
#8655=CARTESIAN_POINT ( 'NONE',  ( 5.000000000000000888, -79.45833333060213022, 2.886751345948126879 ) ) ;
#8657=CARTESIAN_POINT ( 'NONE',  ( 9.457646018065525792E-16, 4.937500001365595637, 5.148502694627439702 ) ) ;
#8658=EDGE_CURVE ( 'NONE', #47006, #50188, #50942, .T. ) ;
#8659=CARTESIAN_POINT ( 'NONE',  ( -4.458734124999999437, -35.64583333196772941, -2.574251347313719407 ) ) ;
#8661=DIRECTION ( 'NONE',  ( 0.000000000000000000, 0.000000000000000000, 1.000000000000000000 ) ) ;
#8663=CARTESIAN_POINT ( 'NONE',  ( -2.229367062500000163, -73.47916666530106511, -3.861377020970580443 ) ) ;
#8665=( BOUNDED_CURVE ( )  B_SPLINE_CURVE ( 2, ( #52364, #42693, #7674, #3476, #37560, #2848, #38197, #22469, #8606 ),
 .UNSPECIFIED., .F., .F. ) 
 B_SPLINE_CURVE_WITH_KNOTS ( ( 3, 2, 2, 2, 3 ),
 ( 0.9839285714285714857, 0.9845238095238095788, 0.9857142857142857650, 0.9869047619047619513, 0.9875000000000000444 ),
 .UNSPECIFIED. ) 
 CURVE ( )  GEOMETRIC_REPRESENTATION_ITEM ( )  RATIONAL_B_SPLINE_CURVE ( ( 0.9330127018922194093, 0.9330127018922256266, 1.000000000000000000, 0.8660254037844387076, 1.000000000000000000, 0.8660254037844387076, 1.000000000000000000, 0.9330127018922194093, 0.9330127018922194093 ) ) 
 REPRESENTATION_ITEM ( '' )  );
#8667=CARTESIAN_POINT ( 'NONE',  ( -2.229367062500000163, -64.47916666530106511, -3.861377020970580443 ) ) ;
#8668=CARTESIAN_POINT ( 'NONE',  ( 2.499999999999998668, -99.20833333060214443, -4.330127018922193649 ) ) ;
#8669=CARTESIAN_POINT ( 'NONE',  ( 1.339745962155612702, -41.29465819873852439, -5.000000000000000000 ) ) ;
#8672=CARTESIAN_POINT ( 'NONE',  ( 4.458734124999998549, -105.9791666653010651, -2.574251347313721627 ) ) ;
#8674=CARTESIAN_POINT ( 'NONE',  ( 1.060575238724906964E-15, -56.74999999999999289, 5.773502691896257311 ) ) ;
#8675=CARTESIAN_POINT ( 'NONE',  ( 5.000000000000000000, -72.29166666393548724, -2.886751345948130876 ) ) ;
#8677=ORIENTED_EDGE ( 'NONE', *, *, #59480, .T. ) ;
#8678=CARTESIAN_POINT ( 'NONE',  ( 5.000000000000000000, -94.50000000000000000, -6.123233995736766282E-16 ) ) ;
#8688=CARTESIAN_POINT ( 'NONE',  ( 0.000000000000000000, -120.0000000000000000, 0.000000000000000000 ) ) ;
#8694=CARTESIAN_POINT ( 'NONE',  ( -2.229367062499996610, -34.39583333196772941, 3.861377020970582219 ) ) ;
#8701=CARTESIAN_POINT ( 'NONE',  ( 5.000000000000000000, -54.49999999999999289, -6.123233995736766282E-16 ) ) ;
#8703=CARTESIAN_POINT ( 'NONE',  ( -4.458734124999998549, -82.47916666530106511, 2.574251347313722516 ) ) ;
#8707=( BOUNDED_CURVE ( )  B_SPLINE_CURVE ( 2, ( #55727, #49927, #11642, #60559, #16481, #36102, #50577, #16798, #35468 ),
 .UNSPECIFIED., .F., .F. ) 
 B_SPLINE_CURVE_WITH_KNOTS ( ( 3, 2, 2, 2, 3 ),
 ( 0.4160714285714285920, 0.4166666666666666852, 0.4178571428571428714, 0.4190476190476190577, 0.4196428571428571508 ),
 .UNSPECIFIED. ) 
 CURVE ( )  GEOMETRIC_REPRESENTATION_ITEM ( )  RATIONAL_B_SPLINE_CURVE ( ( 0.9330127018922194093, 0.9330127018922194093, 1.000000000000000000, 0.8660254037844387076, 1.000000000000000000, 0.8660254037844387076, 1.000000000000000000, 0.9330127018922194093, 0.9330127018922194093 ) ) 
 REPRESENTATION_ITEM ( '' )  );
#8708=CARTESIAN_POINT ( 'NONE',  ( -1.339745962155613812, -105.2053418012614827, -5.000000000000000000 ) ) ;
#8712=ADVANCED_FACE ( 'NONE', ( #2526 ), #26965, .T. ) ;
#8715=CARTESIAN_POINT ( 'NONE',  ( -4.458734124999999437, -10.64583333196773829, -2.574251347313719407 ) ) ;
#8716=ADVANCED_FACE ( 'NONE', ( #36610 ), #17931, .T. ) ;
#8721=ADVANCED_FACE ( 'NONE', ( #27276 ), #32414, .T. ) ;
#8722=CARTESIAN_POINT ( 'NONE',  ( 4.458734125000000326, 24.85416666803225993, 2.574251347313718519 ) ) ;
#8724=CARTESIAN_POINT ( 'NONE',  ( -3.152548672688508926E-16, -89.56249999863439371, -5.148502694627439702 ) ) ;
#8725=CARTESIAN_POINT ( 'NONE',  ( -5.000000000000000000, -68.08333333333332860, -2.886751345948128211 ) ) ;
#8726=CARTESIAN_POINT ( 'NONE',  ( 5.000000000000000888, 7.541666669397851130, 2.886751345948126879 ) ) ;
#8727=CARTESIAN_POINT ( 'NONE',  ( -2.229367062500000163, -6.479166665301072214, -3.861377020970580443 ) ) ;
#8730=EDGE_CURVE ( 'NONE', #10267, #5205, #57527, .T. ) ;
#8732=AXIS2_PLACEMENT_3D ( 'NONE', #54348, #35051, #44357 ) ;
#8734=CARTESIAN_POINT ( 'NONE',  ( -4.999999999999999112, -37.79166666393547303, 2.886751345948131764 ) ) ;
#8735=CARTESIAN_POINT ( 'NONE',  ( 1.339745962155615144, -29.70534180126147561, 4.999999999999999112 ) ) ;
#8736=CARTESIAN_POINT ( 'NONE',  ( 2.229367062500001939, 20.02083333469892779, 3.861377020970579999 ) ) ;
#8737=CARTESIAN_POINT ( 'NONE',  ( 1.975475456537005874E-15, -51.62499999726880873, 5.000000000000000000 ) ) ;
#8740=CARTESIAN_POINT ( 'NONE',  ( -4.458734124999999437, -57.31249999863440081, 0.000000000000000000 ) ) ;
#8742=CARTESIAN_POINT ( 'NONE',  ( 2.500000000000002220, 11.33333333333333393, 4.330127018922192761 ) ) ;
#8746=ADVANCED_FACE ( 'NONE', ( #55806 ), #20752, .T. ) ;
#8747=CARTESIAN_POINT ( 'NONE',  ( 2.229367062499998831, -50.64583333196772941, -3.861377020970580887 ) ) ;
#8748=CARTESIAN_POINT ( 'NONE',  ( 2.500000000000002220, -82.54166666393547303, 4.330127018922192761 ) ) ;
#8750=DIRECTION ( 'NONE',  ( 0.000000000000000000, 0.000000000000000000, 1.000000000000000000 ) ) ;
#8751=LINE ( 'NONE', #43148, #63459 ) ;
#8752=CARTESIAN_POINT ( 'NONE',  ( -4.458734124999997661, -92.47916666530106511, 2.574251347313722516 ) ) ;
#8754=CARTESIAN_POINT ( 'NONE',  ( 2.499999999999998668, -40.33333333333332860, -4.330127018922193649 ) ) ;
#8758=CARTESIAN_POINT ( 'NONE',  ( -2.229367062499996610, -94.14583333196772230, 3.861377020970582219 ) ) ;
#8759=CARTESIAN_POINT ( 'NONE',  ( -4.458734124999998549, 6.520833334698930450, 2.574251347313722516 ) ) ;
#8760=CARTESIAN_POINT ( 'NONE',  ( -3.535250795749689387E-16, 11.87500000273118594, -5.773502691896257311 ) ) ;
#8764=CARTESIAN_POINT ( 'NONE',  ( -2.499999999999996447, 15.29166666939785202, 4.330127018922195425 ) ) ;
#8768=CARTESIAN_POINT ( 'NONE',  ( 5.000000000000000888, -63.58333333333332860, 2.886751345948126879 ) ) ;
#8771=CARTESIAN_POINT ( 'NONE',  ( 1.464175926609780648E-14, 23.87500000273118417, -5.000000000000000000 ) ) ;
#8772=CARTESIAN_POINT ( 'NONE',  ( -4.458734124999998549, -20.47916666530107577, 2.574251347313722516 ) ) ;
#8783=CARTESIAN_POINT ( 'NONE',  ( 4.458734124999998549, -68.97916666530106511, -2.574251347313721627 ) ) ;
#8785=CARTESIAN_POINT ( 'NONE',  ( -4.999999999999998224, -5.791666663935480130, 2.886751345948131764 ) ) ;
#8786=VERTEX_POINT ( 'NONE', #25572 ) ;
#8789=CARTESIAN_POINT ( 'NONE',  ( -4.458734124999999437, 1.437500001365592972, 0.000000000000000000 ) ) ;
#8791=( BOUNDED_CURVE ( )  B_SPLINE_CURVE ( 2, ( #40810, #12500, #22162, #21531, #60775, #51116, #61092, #7053, #21204 ),
 .UNSPECIFIED., .F., .F. ) 
 B_SPLINE_CURVE_WITH_KNOTS ( ( 3, 2, 2, 2, 3 ),
 ( 0.3624999999999999889, 0.3630952380952380820, 0.3642857142857142683, 0.3654761904761904545, 0.3660714285714285476 ),
 .UNSPECIFIED. ) 
 CURVE ( )  GEOMETRIC_REPRESENTATION_ITEM ( )  RATIONAL_B_SPLINE_CURVE ( ( 0.9330127018922194093, 0.9330127018922194093, 1.000000000000000000, 0.8660254037844387076, 1.000000000000000000, 0.8660254037844387076, 1.000000000000000000, 0.9330127018922194093, 0.9330127018922194093 ) ) 
 REPRESENTATION_ITEM ( '' )  );
#8792=FACE_OUTER_BOUND ( 'NONE', #44632, .T. ) ;
#8793=CARTESIAN_POINT ( 'NONE',  ( 4.458734124999998549, 1.270833334698927342, -2.574251347313721627 ) ) ;
#8796=CARTESIAN_POINT ( 'NONE',  ( 2.500000000000002220, 16.33333333333333215, 4.330127018922192761 ) ) ;
#8798=ORIENTED_EDGE ( 'NONE', *, *, #4031, .T. ) ;
#8799=CARTESIAN_POINT ( 'NONE',  ( -2.229367062499996610, -78.14583333196773651, 3.861377020970582219 ) ) ;
#8801=CARTESIAN_POINT ( 'NONE',  ( 2.229367062499998831, 9.354166668032261711, -3.861377020970580887 ) ) ;
#8804=CARTESIAN_POINT ( 'NONE',  ( 9.457646018065525792E-16, -58.31249999863440792, 5.148502694627439702 ) ) ;
#8805=CARTESIAN_POINT ( 'NONE',  ( 5.000000000000000000, -20.29166666393548368, -2.886751345948129988 ) ) ;
#8807=FACE_OUTER_BOUND ( 'NONE', #59150, .T. ) ;
#8809=CARTESIAN_POINT ( 'NONE',  ( 1.975475456537005874E-15, -105.6249999972688016, 5.000000000000000000 ) ) ;
#8812=CARTESIAN_POINT ( 'NONE',  ( 2.229367062500001939, -40.97916666530107221, 3.861377020970579999 ) ) ;
#8813=CARTESIAN_POINT ( 'NONE',  ( 4.458734125000000326, -29.14583333196774007, 2.574251347313718519 ) ) ;
#8815=CARTESIAN_POINT ( 'NONE',  ( 5.000000000000000888, 24.41666666666666785, 2.886751345948126879 ) ) ;
#8817=ORIENTED_EDGE ( 'NONE', *, *, #18172, .T. ) ;
#8818=CARTESIAN_POINT ( 'NONE',  ( -4.458734124999999437, -105.6458333319677507, -2.574251347313719407 ) ) ;
#8819=CARTESIAN_POINT ( 'NONE',  ( -2.229367062499996610, -32.14583333196773651, 3.861377020970582219 ) ) ;
#8820=CARTESIAN_POINT ( 'NONE',  ( 5.000000000000000888, -66.45833333060214443, 2.886751345948126879 ) ) ;
#8825=CARTESIAN_POINT ( 'NONE',  ( -4.458734124999999437, -29.31249999863440436, 0.000000000000000000 ) ) ;
#8826=CARTESIAN_POINT ( 'NONE',  ( -2.229367062500000163, -76.72916666530106511, -3.861377020970580443 ) ) ;
#8830=DIRECTION ( 'NONE',  ( -0.000000000000000000, 1.000000000000000000, -0.000000000000000000 ) ) ;
#8831=CARTESIAN_POINT ( 'NONE',  ( -4.999999999999999112, -19.91666666666666785, 2.886751345948131764 ) ) ;
#8834=CARTESIAN_POINT ( 'NONE',  ( -6.972266317189433020E-16, 1.750000000000000444, -5.000000000000000000 ) ) ;
#8836=CARTESIAN_POINT ( 'NONE',  ( -5.000000000000000000, 26.04166666939784847, -2.886751345948128211 ) ) ;
#8839=LINE ( 'NONE', #57739, #34495 ) ;
#8841=CARTESIAN_POINT ( 'NONE',  ( 3.253724281355068545E-15, 28.75000000000000000, -5.000000000000000000 ) ) ;
#8842=CARTESIAN_POINT ( 'NONE',  ( 6.123233995736766282E-16, -120.0000000000000000, -5.000000000000000000 ) ) ;
#8845=ORIENTED_EDGE ( 'NONE', *, *, #2516, .T. ) ;
#8850=ORIENTED_EDGE ( 'NONE', *, *, #51213, .F. ) ;
#8862=VERTEX_POINT ( 'NONE', #55170 ) ;
#8863=CARTESIAN_POINT ( 'NONE',  ( -4.458734124999999437, -83.31249999863439371, 0.000000000000000000 ) ) ;
#8864=CARTESIAN_POINT ( 'NONE',  ( -4.458734124999999437, 19.60416666803225993, -2.574251347313719407 ) ) ;
#8870=CARTESIAN_POINT ( 'NONE',  ( 1.975475456537005874E-15, -88.74999999999998579, 5.000000000000000000 ) ) ;
#8873=CARTESIAN_POINT ( 'NONE',  ( 2.229367062500001939, -61.97916666530106511, 3.861377020970579999 ) ) ;
#8875=CARTESIAN_POINT ( 'NONE',  ( -3.152548672688508926E-16, 24.43750000136559564, -5.148502694627439702 ) ) ;
#8876=CARTESIAN_POINT ( 'NONE',  ( 5.000000000000000000, -97.41666666666665719, -2.886751345948130876 ) ) ;
#8878=CARTESIAN_POINT ( 'NONE',  ( 2.229367062500001939, -44.22916666530106511, 3.861377020970579999 ) ) ;
#8879=CARTESIAN_POINT ( 'NONE',  ( 1.060575238724906964E-15, -4.624999997268816720, 5.773502691896257311 ) ) ;
#8883=CARTESIAN_POINT ( 'NONE',  ( 4.458734124999998549, -109.7291666653010651, -2.574251347313721627 ) ) ;
#8885=CARTESIAN_POINT ( 'NONE',  ( -4.458734124999997661, -11.47916666530107044, 2.574251347313722516 ) ) ;
#8886=VERTEX_POINT ( 'NONE', #45505 ) ;
#8887=CARTESIAN_POINT ( 'NONE',  ( 5.000000000000000000, -52.50000000000000711, -6.123233995736766282E-16 ) ) ;
#8888=CARTESIAN_POINT ( 'NONE',  ( -4.458734124999999437, -100.3958333319677365, -2.574251347313719407 ) ) ;
#8890=CARTESIAN_POINT ( 'NONE',  ( 2.229367062499998831, -92.89583333196773651, -3.861377020970580887 ) ) ;
#8891=CARTESIAN_POINT ( 'NONE',  ( -3.535250795749689387E-16, -54.12499999726880162, -5.773502691896257311 ) ) ;
#8895=CARTESIAN_POINT ( 'NONE',  ( -4.458734124999997661, -12.22916666530106866, 2.574251347313722516 ) ) ;
#8896=CARTESIAN_POINT ( 'NONE',  ( 9.457646018065525792E-16, 10.68750000136559386, 5.148502694627439702 ) ) ;
#8897=CARTESIAN_POINT ( 'NONE',  ( -4.458734124999999437, -57.56249999863440081, 0.000000000000000000 ) ) ;
#8901=ORIENTED_EDGE ( 'NONE', *, *, #24677, .F. ) ;
#8903=VECTOR ( 'NONE', #6289, 1000.000000000000000 ) ;
#8905=DIRECTION ( 'NONE',  ( 0.000000000000000000, 0.000000000000000000, 1.000000000000000000 ) ) ;
#8907=CARTESIAN_POINT ( 'NONE',  ( 4.458734124999999437, -84.81249999863439371, -5.460374474430324690E-16 ) ) ;
#8908=CARTESIAN_POINT ( 'NONE',  ( -2.229367062500000163, 20.27083333469892779, -3.861377020970580443 ) ) ;
#8910=VECTOR ( 'NONE', #19243, 1000.000000000000000 ) ;
#8912=CARTESIAN_POINT ( 'NONE',  ( -4.999999999999998224, -47.91666666666667140, 2.886751345948131764 ) ) ;
#8916=CARTESIAN_POINT ( 'NONE',  ( 5.000000000000000000, -72.50000000000000000, -6.123233995736766282E-16 ) ) ;
#8918=VERTEX_POINT ( 'NONE', #1468 ) ;
#8919=CARTESIAN_POINT ( 'NONE',  ( -6.972266317189433020E-16, -28.12499999726880873, -5.000000000000000000 ) ) ;
#8932=CARTESIAN_POINT ( 'NONE',  ( -2.229367062499996610, -56.39583333196773651, 3.861377020970582219 ) ) ;
#8934=CARTESIAN_POINT ( 'NONE',  ( -2.499999999999996447, 10.29166666939785024, 4.330127018922195425 ) ) ;
#8935=EDGE_LOOP ( 'NONE', ( #43647, #49100, #63636, #10125 ) ) ;
#8941=CARTESIAN_POINT ( 'NONE',  ( -2.229367062500000163, -104.7291666653010651, -3.861377020970580443 ) ) ;
#8946=CARTESIAN_POINT ( 'NONE',  ( 2.229367062500001939, -37.97916666530107221, 3.861377020970579999 ) ) ;
#8950=CARTESIAN_POINT ( 'NONE',  ( 4.458734125000001214, -7.895833331967735624, 2.574251347313718519 ) ) ;
#8952=CARTESIAN_POINT ( 'NONE',  ( -4.458734124999999437, -101.6458333319677365, -2.574251347313719407 ) ) ;
#8954=CARTESIAN_POINT ( 'NONE',  ( 2.229367062500001939, -26.22916666530106866, 3.861377020970579999 ) ) ;
#8955=AXIS2_PLACEMENT_3D ( 'NONE', #57466, #61340, #28169 ) ;
#8956=DIRECTION ( 'NONE',  ( 0.000000000000000000, 0.000000000000000000, 1.000000000000000000 ) ) ;
#8959=CARTESIAN_POINT ( 'NONE',  ( -5.000000000000000000, -16.08333333333333215, -2.886751345948128211 ) ) ;
#8960=CARTESIAN_POINT ( 'NONE',  ( -1.339745962155613812, -34.20534180126147561, -5.000000000000000000 ) ) ;
#8962=CARTESIAN_POINT ( 'NONE',  ( 2.229367062500001939, 3.770833334698926009, 3.861377020970579999 ) ) ;
#8965=CARTESIAN_POINT ( 'NONE',  ( 1.339745962155641346, 9.705341801261479162, -4.999999999999983125 ) ) ;
#8966=CARTESIAN_POINT ( 'NONE',  ( -2.499999999999996447, -93.83333333333332860, 4.330127018922195425 ) ) ;
#8967=CARTESIAN_POINT ( 'NONE',  ( 2.229367062500001939, -30.97916666530107221, 3.861377020970579999 ) ) ;
#8969=CARTESIAN_POINT ( 'NONE',  ( 2.229367062500001939, -76.22916666530106511, 3.861377020970579999 ) ) ;
#8971=DIRECTION ( 'NONE',  ( -0.000000000000000000, 1.000000000000000000, -0.000000000000000000 ) ) ;
#8974=CARTESIAN_POINT ( 'NONE',  ( 4.458734125000000326, 5.104166668032261711, 2.574251347313718519 ) ) ;
#8975=CARTESIAN_POINT ( 'NONE',  ( 4.458734124999999437, 28.93750000136559208, -5.460374474430324690E-16 ) ) ;
#8976=CARTESIAN_POINT ( 'NONE',  ( -4.458734124999997661, -43.47916666530106511, 2.574251347313722516 ) ) ;
#8977=CARTESIAN_POINT ( 'NONE',  ( -2.499999999999996447, -3.708333330602147537, 4.330127018922195425 ) ) ;
#8981=CARTESIAN_POINT ( 'NONE',  ( 2.229367062500001939, -70.97916666530107932, 3.861377020970579999 ) ) ;
#8982=CARTESIAN_POINT ( 'NONE',  ( -3.535250795749689387E-16, -102.1249999972688158, -5.773502691896257311 ) ) ;
#8985=CARTESIAN_POINT ( 'NONE',  ( -4.999999999999998224, -63.91666666666666430, 2.886751345948131764 ) ) ;
#8986=CARTESIAN_POINT ( 'NONE',  ( -4.458734124999997661, -104.4791666653010651, 2.574251347313722516 ) ) ;
#8988=CARTESIAN_POINT ( 'NONE',  ( 5.000000000000000000, -53.49999999999999289, -6.123233995736766282E-16 ) ) ;
#8996=ADVANCED_FACE ( 'NONE', ( #21714 ), #41307, .T. ) ;
#8998=AXIS2_PLACEMENT_3D ( 'NONE', #63163, #44793, #44150 ) ;
#9002=ORIENTED_EDGE ( 'NONE', *, *, #29089, .T. ) ;
#9005=ORIENTED_EDGE ( 'NONE', *, *, #23458, .T. ) ;
#9009=CARTESIAN_POINT ( 'NONE',  ( 2.229367062500001939, -42.22916666530107932, 3.861377020970579999 ) ) ;
#9013=LINE ( 'NONE', #53388, #4586 ) ;
#9017=CARTESIAN_POINT ( 'NONE',  ( -6.972266317189433020E-16, -25.12499999726881228, -5.000000000000000000 ) ) ;
#9020=CARTESIAN_POINT ( 'NONE',  ( 4.458734125000001214, -86.14583333196775072, 2.574251347313718519 ) ) ;
#9023=CARTESIAN_POINT ( 'NONE',  ( 1.975475456537005874E-15, -99.74999999999998579, 5.000000000000000000 ) ) ;
#9029=CARTESIAN_POINT ( 'NONE',  ( 2.229367062499998831, -10.89583333196773829, -3.861377020970580887 ) ) ;
#9035=CARTESIAN_POINT ( 'NONE',  ( -4.458734124999999437, 22.43750000136559564, 0.000000000000000000 ) ) ;
#9037=CARTESIAN_POINT ( 'NONE',  ( -2.229367062500000163, -92.47916666530106511, -3.861377020970580443 ) ) ;
#9039=CARTESIAN_POINT ( 'NONE',  ( 0.000000000000000000, -120.0000000000000000, 5.000000000000000000 ) ) ;
#9040=CARTESIAN_POINT ( 'NONE',  ( 4.458734124999999437, -15.81249999863440436, -5.460374474430324690E-16 ) ) ;
#9044=DIRECTION ( 'NONE',  ( -0.000000000000000000, 1.000000000000000000, -0.000000000000000000 ) ) ;
#9046=CARTESIAN_POINT ( 'NONE',  ( 1.060575238724906964E-15, -36.62499999726880873, 5.773502691896257311 ) ) ;
#9047=CARTESIAN_POINT ( 'NONE',  ( 2.499999999999998668, -49.20833333060213732, -4.330127018922193649 ) ) ;
#9048=CARTESIAN_POINT ( 'NONE',  ( 4.458734125000000326, 21.10416666803226704, 2.574251347313718519 ) ) ;
#9050=CARTESIAN_POINT ( 'NONE',  ( 4.458734124999999437, -56.81249999863440081, -5.460374474430324690E-16 ) ) ;
#9053=CARTESIAN_POINT ( 'NONE',  ( -5.000000000000000000, 9.999999999999998224, 0.000000000000000000 ) ) ;
#9055=CARTESIAN_POINT ( 'NONE',  ( 4.458734125000001214, -55.89583333196773651, 2.574251347313718519 ) ) ;
#9056=CARTESIAN_POINT ( 'NONE',  ( -5.000000000000000000, -81.87499999726881583, 0.000000000000000000 ) ) ;
#9060=CARTESIAN_POINT ( 'NONE',  ( -4.999999999999998224, -104.7916666639354730, 2.886751345948131764 ) ) ;
#9061=CARTESIAN_POINT ( 'NONE',  ( -4.458734124999999437, -90.64583333196773651, -2.574251347313719407 ) ) ;
#9063=CARTESIAN_POINT ( 'NONE',  ( -5.000000000000000000, -36.08333333333332860, -2.886751345948128211 ) ) ;
#9064=CARTESIAN_POINT ( 'NONE',  ( 1.243387493232115550E-13, -20.12499999726881228, -5.000000000000000000 ) ) ;
#9067=CARTESIAN_POINT ( 'NONE',  ( 2.229367062500001939, -96.97916666530105090, 3.861377020970579999 ) ) ;
#9068=CARTESIAN_POINT ( 'NONE',  ( -2.229367062500000163, 7.270833334698929562, -3.861377020970580443 ) ) ;
#9069=CARTESIAN_POINT ( 'NONE',  ( -2.499999999999996447, 11.29166666939785202, 4.330127018922195425 ) ) ;
#9073=CARTESIAN_POINT ( 'NONE',  ( -2.499999999999996447, 3.166666666666664742, 4.330127018922195425 ) ) ;
#9082=CARTESIAN_POINT ( 'NONE',  ( 1.975475456537005874E-15, -39.62499999726880162, 5.000000000000000000 ) ) ;
#9083=CARTESIAN_POINT ( 'NONE',  ( -4.458734124999998549, -25.47916666530106866, 2.574251347313722516 ) ) ;
#9086=( BOUNDED_CURVE ( )  B_SPLINE_CURVE ( 2, ( #54040, #345, #43126, #62766, #57940, #13858, #33482, #53103, #43439 ),
 .UNSPECIFIED., .F., .F. ) 
 B_SPLINE_CURVE_WITH_KNOTS ( ( 3, 2, 2, 2, 3 ),
 ( 0.5517857142857143238, 0.5523809523809524169, 0.5535714285714286031, 0.5547619047619047894, 0.5553571428571428825 ),
 .UNSPECIFIED. ) 
 CURVE ( )  GEOMETRIC_REPRESENTATION_ITEM ( )  RATIONAL_B_SPLINE_CURVE ( ( 0.9330127018922194093, 0.9330127018922194093, 1.000000000000000000, 0.8660254037844387076, 1.000000000000000000, 0.8660254037844387076, 1.000000000000000000, 0.9330127018922194093, 0.9330127018922194093 ) ) 
 REPRESENTATION_ITEM ( '' )  );
#9089=VECTOR ( 'NONE', #16697, 1000.000000000000000 ) ;
#9091=EDGE_CURVE ( 'NONE', #3482, #31783, #47187, .T. ) ;
#9095=CARTESIAN_POINT ( 'NONE',  ( 4.769696007084728073, -120.0000000000000000, -1.500000000000000444 ) ) ;
#9097=EDGE_LOOP ( 'NONE', ( #37180, #52059, #27354, #36577 ) ) ;
#9098=CARTESIAN_POINT ( 'NONE',  ( 9.457646018065525792E-16, -69.31249999863440792, 5.148502694627439702 ) ) ;
#9099=ORIENTED_EDGE ( 'NONE', *, *, #29978, .T. ) ;
#9100=EDGE_CURVE ( 'NONE', #6898, #3623, #16382, .T. ) ;
#9103=CARTESIAN_POINT ( 'NONE',  ( -2.229367062500000163, -0.7291666653010709931, -3.861377020970580443 ) ) ;
#9105=VECTOR ( 'NONE', #26533, 1000.000000000000000 ) ;
#9112=CARTESIAN_POINT ( 'NONE',  ( 2.229367062499998831, -76.64583333196773651, -3.861377020970580887 ) ) ;
#9114=CARTESIAN_POINT ( 'NONE',  ( -2.229367062500000163, 6.520833334698928674, -3.861377020970580443 ) ) ;
#9116=CARTESIAN_POINT ( 'NONE',  ( 4.458734124999998549, -59.97916666530107221, -2.574251347313721627 ) ) ;
#9117=CARTESIAN_POINT ( 'NONE',  ( -5.000000000000000000, -20.95833333060214798, -2.886751345948128211 ) ) ;
#9119=CARTESIAN_POINT ( 'NONE',  ( 5.000000000000000000, -44.37499999726880873, -6.123233995736766282E-16 ) ) ;
#9120=CARTESIAN_POINT ( 'NONE',  ( 1.339745962155612702, -49.29465819873851018, -5.000000000000000000 ) ) ;
#9123=CARTESIAN_POINT ( 'NONE',  ( -4.458734124999999437, -42.39583333196773651, -2.574251347313719407 ) ) ;
#9124=CARTESIAN_POINT ( 'NONE',  ( 9.457646018065525792E-16, -29.31249999863440436, 5.148502694627439702 ) ) ;
#9125=VECTOR ( 'NONE', #41654, 1000.000000000000000 ) ;
#9127=CARTESIAN_POINT ( 'NONE',  ( 5.000000000000000000, 23.58333333333333215, -2.886751345948129988 ) ) ;
#9129=CARTESIAN_POINT ( 'NONE',  ( -2.229367062499996610, -107.3958333319677365, 3.861377020970582219 ) ) ;
#9131=CARTESIAN_POINT ( 'NONE',  ( -3.152548672688508926E-16, -30.56249999863440436, -5.148502694627439702 ) ) ;
#9132=CARTESIAN_POINT ( 'NONE',  ( 2.499999999999998668, -69.20833333060214443, -4.330127018922193649 ) ) ;
#9135=CARTESIAN_POINT ( 'NONE',  ( -2.229367062500000163, -73.72916666530106511, -3.861377020970580443 ) ) ;
#9140=CARTESIAN_POINT ( 'NONE',  ( 1.060575238724906964E-15, -24.75000000000000355, 5.773502691896257311 ) ) ;
#9144=CARTESIAN_POINT ( 'NONE',  ( -1.339745962155613812, -49.20534180126148271, -5.000000000000000000 ) ) ;
#9146=CARTESIAN_POINT ( 'NONE',  ( 5.000000000000000888, 24.54166666939784847, 2.886751345948126879 ) ) ;
#9147=CARTESIAN_POINT ( 'NONE',  ( 5.000000000000000888, -48.45833333060215153, 2.886751345948126879 ) ) ;
#9152=EDGE_CURVE ( 'NONE', #59111, #38517, #22025, .T. ) ;
#9159=( BOUNDED_CURVE ( )  B_SPLINE_CURVE ( 2, ( #41074, #36574, #7325, #32061, #35951, #7003, #25976, #12128, #46552 ),
 .UNSPECIFIED., .F., .F. ) 
 B_SPLINE_CURVE_WITH_KNOTS ( ( 3, 2, 2, 2, 3 ),
 ( 0.1696428571428571508, 0.1702380952380952439, 0.1714285714285714302, 0.1726190476190476164, 0.1732142857142857095 ),
 .UNSPECIFIED. ) 
 CURVE ( )  GEOMETRIC_REPRESENTATION_ITEM ( )  RATIONAL_B_SPLINE_CURVE ( ( 0.9330127018922194093, 0.9330127018922194093, 1.000000000000000000, 0.8660254037844387076, 1.000000000000000000, 0.8660254037844387076, 1.000000000000000000, 0.9330127018922194093, 0.9330127018922194093 ) ) 
 REPRESENTATION_ITEM ( '' )  );
#9163=ORIENTED_EDGE ( 'NONE', *, *, #62993, .F. ) ;
#9165=CARTESIAN_POINT ( 'NONE',  ( -5.000000000000000000, -102.9583333306021586, -2.886751345948128211 ) ) ;
#9168=EDGE_LOOP ( 'NONE', ( #46129, #6031, #52218, #5845 ) ) ;
#9170=EDGE_CURVE ( 'NONE', #60689, #13643, #29490, .T. ) ;
#9173=CARTESIAN_POINT ( 'NONE',  ( -6.972266317189433020E-16, -82.24999999999998579, -5.000000000000000000 ) ) ;
#9178=CARTESIAN_POINT ( 'NONE',  ( -2.229367062499996610, -80.14583333196773651, 3.861377020970582219 ) ) ;
#9179=CARTESIAN_POINT ( 'NONE',  ( 4.458734125000001214, 21.10416666803226349, 2.574251347313718519 ) ) ;
#9181=ORIENTED_EDGE ( 'NONE', *, *, #21310, .T. ) ;
#9186=CARTESIAN_POINT ( 'NONE',  ( -6.972266317189433020E-16, -13.12499999726881050, -5.000000000000000000 ) ) ;
#9187=CARTESIAN_POINT ( 'NONE',  ( -4.458734124999997661, -60.22916666530105800, 2.574251347313722516 ) ) ;
#9189=CARTESIAN_POINT ( 'NONE',  ( -2.229367062499996610, 23.85416666803225993, 3.861377020970582219 ) ) ;
#9192=CARTESIAN_POINT ( 'NONE',  ( 2.229367062499998831, -44.89583333196774362, -3.861377020970580887 ) ) ;
#9193=CARTESIAN_POINT ( 'NONE',  ( 2.499999999999998668, -3.208333330602147093, -4.330127018922193649 ) ) ;
#9195=DIRECTION ( 'NONE',  ( -0.000000000000000000, 1.000000000000000000, -0.000000000000000000 ) ) ;
#9197=DIRECTION ( 'NONE',  ( -0.000000000000000000, 1.000000000000000000, -0.000000000000000000 ) ) ;
#9198=CARTESIAN_POINT ( 'NONE',  ( -3.152548672688508926E-16, -8.812499998634406140, -5.148502694627439702 ) ) ;
#9200=CARTESIAN_POINT ( 'NONE',  ( -4.458734124999999437, 29.56250000136559208, 0.000000000000000000 ) ) ;
#9201=CARTESIAN_POINT ( 'NONE',  ( -3.152548672688508926E-16, -96.56249999863439371, -5.148502694627439702 ) ) ;
#9203=CARTESIAN_POINT ( 'NONE',  ( -2.229367062500000163, -90.72916666530106511, -3.861377020970580443 ) ) ;
#9204=CARTESIAN_POINT ( 'NONE',  ( -5.000000000000000000, -51.95833333060213732, -2.886751345948128211 ) ) ;
#9208=CARTESIAN_POINT ( 'NONE',  ( 4.458734124999999437, -19.81249999863440081, -5.460374474430324690E-16 ) ) ;
#9209=CARTESIAN_POINT ( 'NONE',  ( -4.458734124999999437, 10.35416666803225816, -2.574251347313719407 ) ) ;
#9210=CARTESIAN_POINT ( 'NONE',  ( 2.229367062499998831, -60.89583333196774362, -3.861377020970580887 ) ) ;
#9219=CARTESIAN_POINT ( 'NONE',  ( -5.000000000000000000, -25.08333333333333215, -2.886751345948128211 ) ) ;
#9220=CARTESIAN_POINT ( 'NONE',  ( -4.458734124999999437, -86.31249999863439371, 0.000000000000000000 ) ) ;
#9221=CARTESIAN_POINT ( 'NONE',  ( 9.457646018065525792E-16, 20.68750000136559564, 5.148502694627439702 ) ) ;
#9224=CARTESIAN_POINT ( 'NONE',  ( -5.000000000000000000, -6.999999999999999112, 0.000000000000000000 ) ) ;
#9226=CARTESIAN_POINT ( 'NONE',  ( -4.999999999999999112, -67.91666666666667140, 2.886751345948131764 ) ) ;
#9228=ORIENTED_EDGE ( 'NONE', *, *, #63627, .F. ) ;
#9229=FACE_OUTER_BOUND ( 'NONE', #26917, .T. ) ;
#9230=ORIENTED_EDGE ( 'NONE', *, *, #48437, .F. ) ;
#9241=ORIENTED_EDGE ( 'NONE', *, *, #787, .F. ) ;
#9244=CARTESIAN_POINT ( 'NONE',  ( -2.229367062500000163, -54.72916666530107221, -3.861377020970580443 ) ) ;
#9247=EDGE_LOOP ( 'NONE', ( #39630, #8506, #12086, #29650 ) ) ;
#9251=ORIENTED_EDGE ( 'NONE', *, *, #57044, .T. ) ;
#9254=CARTESIAN_POINT ( 'NONE',  ( -4.458734124999998549, -106.4791666653010651, 2.574251347313722516 ) ) ;
#9255=CARTESIAN_POINT ( 'NONE',  ( -5.000000000000000000, -26.95833333060214798, -2.886751345948128211 ) ) ;
#9259=CARTESIAN_POINT ( 'NONE',  ( -4.458734124999999437, -40.31249999863440081, 0.000000000000000000 ) ) ;
#9260=( BOUNDED_CURVE ( )  B_SPLINE_CURVE ( 2, ( #31188, #51143, #46308, #26366, #2569, #17039, #50502, #55654, #2265 ),
 .UNSPECIFIED., .F., .F. ) 
 B_SPLINE_CURVE_WITH_KNOTS ( ( 3, 2, 2, 2, 3 ),
 ( 0.03750000000000000555, 0.03809523809523809867, 0.03928571428571428492, 0.04047619047619047811, 0.04107142857142857123 ),
 .UNSPECIFIED. ) 
 CURVE ( )  GEOMETRIC_REPRESENTATION_ITEM ( )  RATIONAL_B_SPLINE_CURVE ( ( 0.9330127018922194093, 0.9330127018922197424, 1.000000000000000000, 0.8660254037844387076, 1.000000000000000000, 0.8660254037844387076, 1.000000000000000000, 0.9330127018922194093, 0.9330127018922194093 ) ) 
 REPRESENTATION_ITEM ( '' )  );
#9261=CARTESIAN_POINT ( 'NONE',  ( 0.000000000000000000, -120.0000000000000000, 0.000000000000000000 ) ) ;
#9262=CARTESIAN_POINT ( 'NONE',  ( -4.458734124999998549, -10.22916666530106866, 2.574251347313722516 ) ) ;
#9263=CARTESIAN_POINT ( 'NONE',  ( -3.152548672688508926E-16, -101.8124999986344079, -5.148502694627439702 ) ) ;
#9265=CARTESIAN_POINT ( 'NONE',  ( 9.457646018065525792E-16, -29.31249999863440436, 5.148502694627439702 ) ) ;
#9269=CARTESIAN_POINT ( 'NONE',  ( -5.000000000000000000, -91.00000000000000000, 0.000000000000000000 ) ) ;
#9271=CARTESIAN_POINT ( 'NONE',  ( -4.458734124999999437, 7.354166668032259047, -2.574251347313719407 ) ) ;
#9274=CARTESIAN_POINT ( 'NONE',  ( 1.975475456537005874E-15, 9.250000000000000000, 5.000000000000000000 ) ) ;
#9275=CARTESIAN_POINT ( 'NONE',  ( 2.500000000000002220, -94.66666666666665719, 4.330127018922192761 ) ) ;
#9276=CARTESIAN_POINT ( 'NONE',  ( -4.458734124999999437, -27.39583333196773651, -2.574251347313719407 ) ) ;
#9278=CARTESIAN_POINT ( 'NONE',  ( -4.458734124999999437, -74.56249999863440792, 0.000000000000000000 ) ) ;
#9283=CARTESIAN_POINT ( 'NONE',  ( 2.229367062499998831, 5.354166668032261711, -3.861377020970580887 ) ) ;
#9284=CARTESIAN_POINT ( 'NONE',  ( 2.229367062500001939, 25.77083333469892779, 3.861377020970579999 ) ) ;
#9285=CARTESIAN_POINT ( 'NONE',  ( 4.458734125000000326, -41.14583333196773651, 2.574251347313718519 ) ) ;
#9290=CARTESIAN_POINT ( 'NONE',  ( -4.458734124999999437, -70.39583333196773651, -2.574251347313719407 ) ) ;
#9291=CARTESIAN_POINT ( 'NONE',  ( 5.000000000000000000, -106.3749999972688158, -6.123233995736766282E-16 ) ) ;
#9293=CARTESIAN_POINT ( 'NONE',  ( 0.000000000000000000, -120.0000000000000000, 5.000000000000000000 ) ) ;
#9294=CARTESIAN_POINT ( 'NONE',  ( -4.458734124999999437, -105.6458333319677365, -2.574251347313719407 ) ) ;
#9296=CARTESIAN_POINT ( 'NONE',  ( 2.500000000000002220, -52.66666666666666430, 4.330127018922192761 ) ) ;
#9301=AXIS2_PLACEMENT_3D ( 'NONE', #62150, #58260, #33810 ) ;
#9310=ORIENTED_EDGE ( 'NONE', *, *, #15253, .T. ) ;
#9311=LINE ( 'NONE', #59161, #16908 ) ;
#9317=CARTESIAN_POINT ( 'NONE',  ( 4.458734124999999437, -40.06249999863440081, -5.460374474430324690E-16 ) ) ;
#9326=CARTESIAN_POINT ( 'NONE',  ( -2.229367062500000163, -91.72916666530106511, -3.861377020970580443 ) ) ;
#9327=CARTESIAN_POINT ( 'NONE',  ( 1.975475456537005874E-15, -34.62499999726880873, 5.000000000000000000 ) ) ;
#9328=ORIENTED_EDGE ( 'NONE', *, *, #21593, .T. ) ;
#9332=CARTESIAN_POINT ( 'NONE',  ( 0.000000000000000000, -120.0000000000000000, 0.000000000000000000 ) ) ;
#9336=CARTESIAN_POINT ( 'NONE',  ( -4.458734124999998549, -10.47916666530107044, 2.574251347313722516 ) ) ;
#9339=CARTESIAN_POINT ( 'NONE',  ( -5.000000000000000000, -11.95833333060214798, -2.886751345948128211 ) ) ;
#9341=CARTESIAN_POINT ( 'NONE',  ( -4.458734124999997661, 19.52083333469893134, 2.574251347313722516 ) ) ;
#9343=CARTESIAN_POINT ( 'NONE',  ( -4.458734124999997661, -94.22916666530106511, 2.574251347313722516 ) ) ;
#9344=CARTESIAN_POINT ( 'NONE',  ( -6.972266317189433020E-16, -104.1249999972688016, -5.000000000000000000 ) ) ;
#9345=CARTESIAN_POINT ( 'NONE',  ( -4.458734124999999437, -14.39583333196773474, -2.574251347313719407 ) ) ;
#9348=DIRECTION ( 'NONE',  ( -0.000000000000000000, 1.000000000000000000, -0.000000000000000000 ) ) ;
#9350=( BOUNDED_CURVE ( )  B_SPLINE_CURVE ( 2, ( #57319, #35866, #13236, #55491, #42816, #32859, #26529, #52488, #46149 ),
 .UNSPECIFIED., .F., .F. ) 
 B_SPLINE_CURVE_WITH_KNOTS ( ( 3, 2, 2, 2, 3 ),
 ( 0.6624999999999999778, 0.6630952380952380709, 0.6642857142857142572, 0.6654761904761904434, 0.6660714285714285365 ),
 .UNSPECIFIED. ) 
 CURVE ( )  GEOMETRIC_REPRESENTATION_ITEM ( )  RATIONAL_B_SPLINE_CURVE ( ( 0.9330127018922194093, 0.9330127018922194093, 1.000000000000000000, 0.8660254037844387076, 1.000000000000000000, 0.8660254037844387076, 1.000000000000000000, 0.9330127018922194093, 0.9330127018922194093 ) ) 
 REPRESENTATION_ITEM ( '' )  );
#9352=CARTESIAN_POINT ( 'NONE',  ( 1.060575238724906964E-15, -41.62499999726880162, 5.773502691896257311 ) ) ;
#9354=CARTESIAN_POINT ( 'NONE',  ( -4.458734124999999437, 21.68750000136559208, 0.000000000000000000 ) ) ;
#9355=CARTESIAN_POINT ( 'NONE',  ( -5.000000000000000000, 12.12500000273118772, 0.000000000000000000 ) ) ;
#9358=CARTESIAN_POINT ( 'NONE',  ( 2.229367062499998831, -62.64583333196774362, -3.861377020970580887 ) ) ;
#9361=CARTESIAN_POINT ( 'NONE',  ( -2.499999999999996447, 12.16666666666666607, 4.330127018922195425 ) ) ;
#9364=CARTESIAN_POINT ( 'NONE',  ( -2.229367062499996610, -52.14583333196773651, 3.861377020970582219 ) ) ;
#9365=CARTESIAN_POINT ( 'NONE',  ( 5.000000000000000000, -89.29166666393545881, -2.886751345948129988 ) ) ;
#9368=EDGE_CURVE ( 'NONE', #45662, #49599, #22208, .T. ) ;
#9369=LINE ( 'NONE', #33198, #8006 ) ;
#9371=CARTESIAN_POINT ( 'NONE',  ( 9.457646018065525792E-16, -89.31249999863440792, 5.148502694627439702 ) ) ;
#9373=CARTESIAN_POINT ( 'NONE',  ( -2.499999999999996447, -38.83333333333332860, 4.330127018922195425 ) ) ;
#9375=VERTEX_POINT ( 'NONE', #17919 ) ;
#9376=CARTESIAN_POINT ( 'NONE',  ( -4.458734124999998549, -101.2291666653010651, 2.574251347313722516 ) ) ;
#9377=CARTESIAN_POINT ( 'NONE',  ( -4.458734124999998549, 8.520833334698926009, 2.574251347313722516 ) ) ;
#9382=DIRECTION ( 'NONE',  ( -0.000000000000000000, 1.000000000000000000, -0.000000000000000000 ) ) ;
#9385=DIRECTION ( 'NONE',  ( -0.000000000000000000, 1.000000000000000000, -0.000000000000000000 ) ) ;
#9389=CARTESIAN_POINT ( 'NONE',  ( -5.000000000000000000, -89.87499999726880162, 0.000000000000000000 ) ) ;
#9390=CARTESIAN_POINT ( 'NONE',  ( 4.458734124999999437, -23.06249999863440436, -5.460374474430324690E-16 ) ) ;
#9393=AXIS2_PLACEMENT_3D ( 'NONE', #17679, #47569, #37602 ) ;
#9398=EDGE_LOOP ( 'NONE', ( #48431, #16615, #47457, #33617 ) ) ;
#9402=CARTESIAN_POINT ( 'NONE',  ( 4.458734124999999437, -72.06249999863439371, -5.460374474430324690E-16 ) ) ;
#9409=CARTESIAN_POINT ( 'NONE',  ( 9.457646018065525792E-16, -0.3124999986344051961, 5.148502694627439702 ) ) ;
#9411=CARTESIAN_POINT ( 'NONE',  ( 5.000000000000000000, -69.29166666393547303, -2.886751345948130876 ) ) ;
#9414=CARTESIAN_POINT ( 'NONE',  ( 5.000000000000000000, 16.50000000000000000, -6.123233995736766282E-16 ) ) ;
#9417=CARTESIAN_POINT ( 'NONE',  ( -4.458734124999999437, -75.31249999863440792, 0.000000000000000000 ) ) ;
#9419=CARTESIAN_POINT ( 'NONE',  ( -4.458734124999998549, 0.7708333346989267865, 2.574251347313722516 ) ) ;
#9420=EDGE_CURVE ( 'NONE', #12555, #42937, #58970, .T. ) ;
#9423=EDGE_CURVE ( 'NONE', #49599, #10376, #61657, .T. ) ;
#9424=CARTESIAN_POINT ( 'NONE',  ( 9.457646018065525792E-16, -65.31249999863440792, 5.148502694627439702 ) ) ;
#9425=CARTESIAN_POINT ( 'NONE',  ( -2.499999999999996447, -26.70833333060214798, 4.330127018922195425 ) ) ;
#9426=CARTESIAN_POINT ( 'NONE',  ( 5.000000000000000888, -96.45833333060213022, 2.886751345948126879 ) ) ;
#9427=CARTESIAN_POINT ( 'NONE',  ( -6.972266317189433020E-16, -59.25000000000000000, -5.000000000000000000 ) ) ;
#9429=FACE_OUTER_BOUND ( 'NONE', #59719, .T. ) ;
#9430=CARTESIAN_POINT ( 'NONE',  ( 4.458734125000001214, -43.89583333196775072, 2.574251347313718519 ) ) ;
#9431=CARTESIAN_POINT ( 'NONE',  ( 4.458734125000000326, -27.14583333196774717, 2.574251347313718519 ) ) ;
#9433=DIRECTION ( 'NONE',  ( 0.000000000000000000, 0.000000000000000000, 1.000000000000000000 ) ) ;
#9434=CARTESIAN_POINT ( 'NONE',  ( 5.000000000000000000, 27.50000000000000000, -6.123233995736766282E-16 ) ) ;
#9437=CARTESIAN_POINT ( 'NONE',  ( -2.229367062499996610, -39.14583333196773651, 3.861377020970582219 ) ) ;
#9438=CARTESIAN_POINT ( 'NONE',  ( 5.000000000000000000, -67.29166666393547303, -2.886751345948129988 ) ) ;
#9442=CARTESIAN_POINT ( 'NONE',  ( 9.457646018065525792E-16, -76.31249999863440792, 5.148502694627439702 ) ) ;
#9446=CARTESIAN_POINT ( 'NONE',  ( 2.500000000000002220, 22.45833333606451987, 4.330127018922192761 ) ) ;
#9447=CARTESIAN_POINT ( 'NONE',  ( -2.499999999999996447, -20.83333333333333570, 4.330127018922195425 ) ) ;
#9451=CARTESIAN_POINT ( 'NONE',  ( 1.339745962155612702, 1.705341801261480272, -5.000000000000000000 ) ) ;
#9453=CARTESIAN_POINT ( 'NONE',  ( -4.999999999999999112, 28.20833333606451632, 2.886751345948131764 ) ) ;
#9460=CARTESIAN_POINT ( 'NONE',  ( 1.975475456537005874E-15, -40.62499999726879452, 5.000000000000000000 ) ) ;
#9461=CARTESIAN_POINT ( 'NONE',  ( -6.972266317189433020E-16, -89.12499999726880162, -5.000000000000000000 ) ) ;
#9462=CARTESIAN_POINT ( 'NONE',  ( -4.999999999999998224, -87.79166666393547303, 2.886751345948131764 ) ) ;
#9463=CARTESIAN_POINT ( 'NONE',  ( -2.229367062500000163, -22.47916666530107221, -3.861377020970580443 ) ) ;
#9464=CARTESIAN_POINT ( 'NONE',  ( 1.339745962155615144, 0.2946581987385212820, 4.999999999999999112 ) ) ;
#9470=VERTEX_POINT ( 'NONE', #48132 ) ;
#9471=CARTESIAN_POINT ( 'NONE',  ( 2.500000000000002220, -87.66666666666667140, 4.330127018922192761 ) ) ;
#9472=CARTESIAN_POINT ( 'NONE',  ( -5.000000000000000000, -67.87499999726881583, 0.000000000000000000 ) ) ;
#9475=CARTESIAN_POINT ( 'NONE',  ( 0.000000000000000000, -120.0000000000000000, 5.000000000000000000 ) ) ;
#9479=ORIENTED_EDGE ( 'NONE', *, *, #12296, .T. ) ;
#9481=CARTESIAN_POINT ( 'NONE',  ( -4.458734124999998549, 18.77083333469893134, 2.574251347313722516 ) ) ;
#9482=CARTESIAN_POINT ( 'NONE',  ( 5.000000000000000000, -12.29166666393547835, -2.886751345948130876 ) ) ;
#9483=VERTEX_POINT ( 'NONE', #21016 ) ;
#9486=CARTESIAN_POINT ( 'NONE',  ( 1.339745962155612702, -88.29465819873851729, -5.000000000000000000 ) ) ;
#9487=CARTESIAN_POINT ( 'NONE',  ( 0.000000000000000000, -120.0000000000000000, 5.000000000000000000 ) ) ;
#9488=CARTESIAN_POINT ( 'NONE',  ( -5.000000000000000000, -103.0833333333333286, -2.886751345948128211 ) ) ;
#9489=CARTESIAN_POINT ( 'NONE',  ( 4.458734124999999437, -61.81249999863440081, -5.460374474430324690E-16 ) ) ;
#9491=CARTESIAN_POINT ( 'NONE',  ( 9.457646018065525792E-16, 16.93750000136559564, 5.148502694627439702 ) ) ;
#9494=EDGE_CURVE ( 'NONE', #2754, #6651, #48481, .T. ) ;
#9495=EDGE_CURVE ( 'NONE', #45662, #29252, #49640, .T. ) ;
#9496=CARTESIAN_POINT ( 'NONE',  ( 4.458734125000001214, -48.14583333196773651, 2.574251347313718519 ) ) ;
#9497=CARTESIAN_POINT ( 'NONE',  ( -3.535250795749689387E-16, -3.124999997268815832, -5.773502691896257311 ) ) ;
#9502=CARTESIAN_POINT ( 'NONE',  ( 9.457646018065525792E-16, -107.0624999986343937, 5.148502694627439702 ) ) ;
#9503=CARTESIAN_POINT ( 'NONE',  ( 2.229367062499998831, -11.89583333196774007, -3.861377020970580887 ) ) ;
#9505=ORIENTED_EDGE ( 'NONE', *, *, #10671, .F. ) ;
#9506=CARTESIAN_POINT ( 'NONE',  ( 1.339745962155612702, -52.29465819873851729, -5.000000000000000000 ) ) ;
#9507=CARTESIAN_POINT ( 'NONE',  ( 2.229367062500001939, -99.97916666530106511, 3.861377020970579999 ) ) ;
#9509=CARTESIAN_POINT ( 'NONE',  ( 4.458734124999999437, -91.06249999863440792, -5.460374474430324690E-16 ) ) ;
#9510=CYLINDRICAL_SURFACE ( 'NONE', #51023, 5.000000000000000000 ) ;
#9511=CARTESIAN_POINT ( 'NONE',  ( -2.500000000000000444, -50.04166666393547303, -4.330127018922193649 ) ) ;
#9513=CARTESIAN_POINT ( 'NONE',  ( 1.339745962155615144, -5.705341801261479162, 4.999999999999999112 ) ) ;
#9514=EDGE_CURVE ( 'NONE', #50188, #30770, #28755, .T. ) ;
#9517=CARTESIAN_POINT ( 'NONE',  ( 2.229367062500001939, -19.97916666530107221, 3.861377020970579999 ) ) ;
#9518=CARTESIAN_POINT ( 'NONE',  ( 9.457646018065525792E-16, 12.68750000136559208, 5.148502694627439702 ) ) ;
#9519=CARTESIAN_POINT ( 'NONE',  ( 9.457646018065525792E-16, -60.31249999863441502, 5.148502694627439702 ) ) ;
#9524=CARTESIAN_POINT ( 'NONE',  ( -2.500000000000000444, -7.166666666666668739, -4.330127018922193649 ) ) ;
#9528=CARTESIAN_POINT ( 'NONE',  ( -6.972266317189433020E-16, -103.1249999972688158, -5.000000000000000000 ) ) ;
#9530=CARTESIAN_POINT ( 'NONE',  ( -2.500000000000000444, -9.166666666666662522, -4.330127018922193649 ) ) ;
#9532=CARTESIAN_POINT ( 'NONE',  ( 2.229367062500001939, -86.97916666530107932, 3.861377020970579999 ) ) ;
#9533=CARTESIAN_POINT ( 'NONE',  ( 2.229367062500001939, 17.77083333469892779, 3.861377020970579999 ) ) ;
#9541=CARTESIAN_POINT ( 'NONE',  ( 1.060575238724906964E-15, -72.74999999999998579, 5.773502691896257311 ) ) ;
#9543=ORIENTED_EDGE ( 'NONE', *, *, #33801, .F. ) ;
#9551=ORIENTED_EDGE ( 'NONE', *, *, #39672, .T. ) ;
#9555=ORIENTED_EDGE ( 'NONE', *, *, #3544, .T. ) ;
#9558=CARTESIAN_POINT ( 'NONE',  ( 4.458734124999999437, -56.06249999863440081, -5.460374474430324690E-16 ) ) ;
#9560=CARTESIAN_POINT ( 'NONE',  ( 5.000000000000000000, 3.625000002731186388, -6.123233995736766282E-16 ) ) ;
#9561=VERTEX_POINT ( 'NONE', #41886 ) ;
#9564=VERTEX_POINT ( 'NONE', #17138 ) ;
#9567=CARTESIAN_POINT ( 'NONE',  ( -2.229367062499996610, -107.3958333319677365, 3.861377020970582219 ) ) ;
#9569=ORIENTED_EDGE ( 'NONE', *, *, #13449, .F. ) ;
#9572=CARTESIAN_POINT ( 'NONE',  ( -4.458734124999999437, -36.39583333196773651, -2.574251347313719407 ) ) ;
#9575=CARTESIAN_POINT ( 'NONE',  ( 2.229367062500001939, -10.97916666530107044, 3.861377020970579999 ) ) ;
#9576=CARTESIAN_POINT ( 'NONE',  ( 2.229367062500001939, -98.22916666530105090, 3.861377020970579999 ) ) ;
#9578=VERTEX_POINT ( 'NONE', #45771 ) ;
#9580=CARTESIAN_POINT ( 'NONE',  ( 4.458734124999999437, -35.06249999863440792, -5.460374474430324690E-16 ) ) ;
#9581=CARTESIAN_POINT ( 'NONE',  ( -6.972266317189433020E-16, 11.74999999999999645, -5.000000000000000000 ) ) ;
#9585=CARTESIAN_POINT ( 'NONE',  ( 5.000000000000000888, -17.58333333333333215, 2.886751345948126879 ) ) ;
#9588=CARTESIAN_POINT ( 'NONE',  ( 9.457646018065525792E-16, 4.687500001365595637, 5.148502694627439702 ) ) ;
#9589=VERTEX_POINT ( 'NONE', #2048 ) ;
#9591=CARTESIAN_POINT ( 'NONE',  ( -2.500000000000000444, -94.16666666666665719, -4.330127018922193649 ) ) ;
#9592=CARTESIAN_POINT ( 'NONE',  ( -4.458734124999999437, -32.39583333196773651, -2.574251347313719407 ) ) ;
#9594=CARTESIAN_POINT ( 'NONE',  ( -2.229367062500000163, -77.72916666530106511, -3.861377020970580443 ) ) ;
#9596=CARTESIAN_POINT ( 'NONE',  ( -1.339745962155613812, -102.0803417985302843, -5.000000000000000000 ) ) ;
#9598=CARTESIAN_POINT ( 'NONE',  ( -3.152548672688508926E-16, -4.562499998634401699, -5.148502694627439702 ) ) ;
#9599=CARTESIAN_POINT ( 'NONE',  ( -3.152548672688508926E-16, 27.18750000136559564, -5.148502694627439702 ) ) ;
#9600=CARTESIAN_POINT ( 'NONE',  ( -3.152548672688508926E-16, -43.81249999863440081, -5.148502694627439702 ) ) ;
#9603=ORIENTED_EDGE ( 'NONE', *, *, #1931, .F. ) ;
#9605=CARTESIAN_POINT ( 'NONE',  ( 4.458734125000001214, -69.89583333196773651, 2.574251347313718519 ) ) ;
#9606=CARTESIAN_POINT ( 'NONE',  ( 2.500000000000002220, -104.5416666639354730, 4.330127018922192761 ) ) ;
#9608=EDGE_CURVE ( 'NONE', #14094, #50477, #21655, .T. ) ;
#9609=CARTESIAN_POINT ( 'NONE',  ( -2.500000000000000444, -64.16666666666665719, -4.330127018922193649 ) ) ;
#9610=LINE ( 'NONE', #10562, #31677 ) ;
#9612=CARTESIAN_POINT ( 'NONE',  ( 2.500000000000002220, -54.66666666666667140, 4.330127018922192761 ) ) ;
#9613=CARTESIAN_POINT ( 'NONE',  ( -4.330127018922101279, 45.00000000000000000, 7.500000000000002665 ) ) ;
#9625=CARTESIAN_POINT ( 'NONE',  ( -1.339745962155610925, -23.79465819873851729, 5.000000000000000000 ) ) ;
#9628=ORIENTED_EDGE ( 'NONE', *, *, #24758, .T. ) ;
#9632=CARTESIAN_POINT ( 'NONE',  ( 2.229367062499998831, -40.89583333196773651, -3.861377020970580887 ) ) ;
#9639=VECTOR ( 'NONE', #40028, 1000.000000000000000 ) ;
#9642=CARTESIAN_POINT ( 'NONE',  ( 2.229367062500001939, -89.22916666530106511, 3.861377020970579999 ) ) ;
#9645=CARTESIAN_POINT ( 'NONE',  ( -1.339745962155610925, -46.79465819873852439, 5.000000000000000000 ) ) ;
#9650=CARTESIAN_POINT ( 'NONE',  ( 4.458734124999999437, -14.06249999863440436, -5.460374474430324690E-16 ) ) ;
#9655=CARTESIAN_POINT ( 'NONE',  ( 4.458734125000000326, 19.85416666803226349, 2.574251347313718519 ) ) ;
#9657=CARTESIAN_POINT ( 'NONE',  ( 4.458734124999998549, -98.72916666530105090, -2.574251347313721627 ) ) ;
#9658=CARTESIAN_POINT ( 'NONE',  ( -1.339745962155610925, -33.66965819600732601, 5.000000000000000000 ) ) ;
#9660=CARTESIAN_POINT ( 'NONE',  ( 2.229367062500001939, -11.97916666530107044, 3.861377020970579999 ) ) ;
#9661=CARTESIAN_POINT ( 'NONE',  ( 2.499999999999998668, -39.20833333060214443, -4.330127018922193649 ) ) ;
#9663=CARTESIAN_POINT ( 'NONE',  ( 1.975475456537005874E-15, -90.74999999999998579, 5.000000000000000000 ) ) ;
#9664=CARTESIAN_POINT ( 'NONE',  ( 2.499999999999998668, -42.20833333060214443, -4.330127018922193649 ) ) ;
#9665=CARTESIAN_POINT ( 'NONE',  ( 5.000000000000000888, -29.58333333333332860, 2.886751345948126879 ) ) ;
#9666=CARTESIAN_POINT ( 'NONE',  ( -4.458734124999999437, 15.60416666803225993, -2.574251347313719407 ) ) ;
#9667=CARTESIAN_POINT ( 'NONE',  ( 5.000000000000000000, -46.37499999726880873, -6.123233995736766282E-16 ) ) ;
#9670=CARTESIAN_POINT ( 'NONE',  ( -2.229367062500000163, -61.47916666530106511, -3.861377020970580443 ) ) ;
#9672=CARTESIAN_POINT ( 'NONE',  ( -6.972266317189433020E-16, -109.1249999972688016, -5.000000000000000000 ) ) ;
#9673=CARTESIAN_POINT ( 'NONE',  ( -5.000000000000000000, 7.916666666666665186, -2.886751345948128211 ) ) ;
#9675=CARTESIAN_POINT ( 'NONE',  ( 1.975475456537005874E-15, -98.62499999726880162, 5.000000000000000000 ) ) ;
#9676=CARTESIAN_POINT ( 'NONE',  ( 4.458734124999999437, -50.81249999863440792, -5.460374474430324690E-16 ) ) ;
#9677=CARTESIAN_POINT ( 'NONE',  ( -2.499999999999996447, -91.70833333060214443, 4.330127018922195425 ) ) ;
#9683=CARTESIAN_POINT ( 'NONE',  ( -2.499999999999996447, -37.83333333333332860, 4.330127018922195425 ) ) ;
#9685=CARTESIAN_POINT ( 'NONE',  ( 2.499999999999998668, -22.33333333333332860, -4.330127018922193649 ) ) ;
#9687=CARTESIAN_POINT ( 'NONE',  ( -4.458734124999999437, -100.3124999986344079, 0.000000000000000000 ) ) ;
#9688=CARTESIAN_POINT ( 'NONE',  ( 2.229367062499998831, 5.104166668032261711, -3.861377020970580887 ) ) ;
#9693=CARTESIAN_POINT ( 'NONE',  ( -6.972266317189433020E-16, 2.750000000000000000, -5.000000000000000000 ) ) ;
#9702=CARTESIAN_POINT ( 'NONE',  ( 2.229367062500001939, -24.22916666530107577, 3.861377020970579999 ) ) ;
#9713=CARTESIAN_POINT ( 'NONE',  ( 0.000000000000000000, -120.0000000000000000, 0.000000000000000000 ) ) ;
#9715=CARTESIAN_POINT ( 'NONE',  ( -2.229367062500000163, -74.72916666530106511, -3.861377020970580443 ) ) ;
#9716=CARTESIAN_POINT ( 'NONE',  ( -4.999999999999998224, 29.08333333333333215, 2.886751345948131764 ) ) ;
#9718=CARTESIAN_POINT ( 'NONE',  ( 2.499999999999998668, -20.20833333060214798, -4.330127018922193649 ) ) ;
#9721=CARTESIAN_POINT ( 'NONE',  ( -4.458734124999999437, 0.4375000013655955255, 0.000000000000000000 ) ) ;
#9722=ORIENTED_EDGE ( 'NONE', *, *, #55429, .F. ) ;
#9724=EDGE_CURVE ( 'NONE', #27676, #45662, #58811, .T. ) ;
#9732=CARTESIAN_POINT ( 'NONE',  ( 4.458734125000000326, -76.89583333196773651, 2.574251347313718519 ) ) ;
#9734=CARTESIAN_POINT ( 'NONE',  ( 2.229367062499998831, 4.354166668032260823, -3.861377020970580887 ) ) ;
#9735=CARTESIAN_POINT ( 'NONE',  ( 0.000000000000000000, -114.9999999999999858, 0.000000000000000000 ) ) ;
#9736=CARTESIAN_POINT ( 'NONE',  ( -3.152548672688508926E-16, -64.81249999863440792, -5.148502694627439702 ) ) ;
#9737=CARTESIAN_POINT ( 'NONE',  ( 2.500000000000002220, -24.54166666393548368, 4.330127018922192761 ) ) ;
#9738=CARTESIAN_POINT ( 'NONE',  ( 0.000000000000000000, -120.0000000000000000, 0.000000000000000000 ) ) ;
#9739=CARTESIAN_POINT ( 'NONE',  ( 5.000000000000000000, -28.37499999726881228, -6.123233995736766282E-16 ) ) ;
#9740=CARTESIAN_POINT ( 'NONE',  ( 0.000000000000000000, -120.0000000000000000, 5.000000000000000000 ) ) ;
#9741=CARTESIAN_POINT ( 'NONE',  ( 2.229367062499998831, -45.64583333196774362, -3.861377020970580887 ) ) ;
#9742=CARTESIAN_POINT ( 'NONE',  ( -2.229367062500000163, -24.72916666530106866, -3.861377020970580443 ) ) ;
#9745=CARTESIAN_POINT ( 'NONE',  ( 2.500000000000002220, 27.33333333333333215, 4.330127018922192761 ) ) ;
#9748=CARTESIAN_POINT ( 'NONE',  ( 4.458734124999998549, -38.72916666530106511, -2.574251347313721627 ) ) ;
#9749=CARTESIAN_POINT ( 'NONE',  ( -4.999999999999999112, -70.79166666393548724, 2.886751345948131764 ) ) ;
#9752=CARTESIAN_POINT ( 'NONE',  ( 2.229367062500001939, -77.22916666530106511, 3.861377020970579999 ) ) ;
#9755=CARTESIAN_POINT ( 'NONE',  ( 0.000000000000000000, -120.0000000000000000, 0.000000000000000000 ) ) ;
#9757=CARTESIAN_POINT ( 'NONE',  ( -2.500000000000000444, -23.16666666666666785, -4.330127018922193649 ) ) ;
#9759=ORIENTED_EDGE ( 'NONE', *, *, #33908, .T. ) ;
#9763=CARTESIAN_POINT ( 'NONE',  ( 5.000000000000000000, 26.62500000273118772, -6.123233995736766282E-16 ) ) ;
#9765=CARTESIAN_POINT ( 'NONE',  ( -5.000000000000000000, 8.125000002731187720, 0.000000000000000000 ) ) ;
#9766=VECTOR ( 'NONE', #29395, 1000.000000000000000 ) ;
#9770=CARTESIAN_POINT ( 'NONE',  ( 2.493747252781420335E-13, -91.12499999726880162, -5.000000000000000000 ) ) ;
#9772=CARTESIAN_POINT ( 'NONE',  ( 5.000000000000000000, 18.58333333333333215, -2.886751345948130876 ) ) ;
#9774=CARTESIAN_POINT ( 'NONE',  ( 4.458734124999998549, -21.72916666530107221, -2.574251347313721627 ) ) ;
#9775=CARTESIAN_POINT ( 'NONE',  ( 2.499999999999998668, -97.20833333060213022, -4.330127018922193649 ) ) ;
#9782=ORIENTED_EDGE ( 'NONE', *, *, #28330, .T. ) ;
#9786=EDGE_CURVE ( 'NONE', #54905, #6256, #41150, .T. ) ;
#9787=CARTESIAN_POINT ( 'NONE',  ( -1.339745962155610925, 11.20534180126147739, 5.000000000000000000 ) ) ;
#9794=CARTESIAN_POINT ( 'NONE',  ( 4.458734124999998549, 18.27083333469893134, -2.574251347313721627 ) ) ;
#9796=VERTEX_POINT ( 'NONE', #57022 ) ;
#9802=CARTESIAN_POINT ( 'NONE',  ( -2.229367062499996610, -62.14583333196774362, 3.861377020970582219 ) ) ;
#9803=CARTESIAN_POINT ( 'NONE',  ( -4.458734124999999437, 15.68750000136559564, 0.000000000000000000 ) ) ;
#9804=VECTOR ( 'NONE', #25286, 1000.000000000000000 ) ;
#9805=CARTESIAN_POINT ( 'NONE',  ( 0.000000000000000000, -120.0000000000000000, 0.000000000000000000 ) ) ;
#9806=CARTESIAN_POINT ( 'NONE',  ( -4.458734124999999437, -51.64583333196773651, -2.574251347313719407 ) ) ;
#9807=CARTESIAN_POINT ( 'NONE',  ( -5.000000000000000000, -10.87499999726881583, 0.000000000000000000 ) ) ;
#9808=CARTESIAN_POINT ( 'NONE',  ( 1.975475456537005874E-15, -92.74999999999998579, 5.000000000000000000 ) ) ;
#9811=CARTESIAN_POINT ( 'NONE',  ( -2.229367062500000163, -107.4791666653010651, -3.861377020970580443 ) ) ;
#9812=CARTESIAN_POINT ( 'NONE',  ( -4.458734124999999437, -8.645833331967736513, -2.574251347313719407 ) ) ;
#9814=CARTESIAN_POINT ( 'NONE',  ( 9.457646018065525792E-16, -96.06249999863440792, 5.148502694627439702 ) ) ;
#9816=CARTESIAN_POINT ( 'NONE',  ( 4.458734124999999437, -98.06249999863440792, -5.460374474430324690E-16 ) ) ;
#9818=CARTESIAN_POINT ( 'NONE',  ( 1.975475456537005874E-15, -7.750000000000000000, 5.000000000000000000 ) ) ;
#9819=CARTESIAN_POINT ( 'NONE',  ( 2.500000000000002220, -55.54166666393548013, 4.330127018922192761 ) ) ;
#9820=CARTESIAN_POINT ( 'NONE',  ( 5.000000000000000000, -5.499999999999998224, -6.123233995736766282E-16 ) ) ;
#9823=CARTESIAN_POINT ( 'NONE',  ( 4.458734124999998549, -19.72916666530107221, -2.574251347313721627 ) ) ;
#9824=CARTESIAN_POINT ( 'NONE',  ( -4.458734124999999437, 4.437500001365595637, 0.000000000000000000 ) ) ;
#9825=CARTESIAN_POINT ( 'NONE',  ( 4.458734124999999437, -58.06249999863440081, -5.460374474430324690E-16 ) ) ;
#9826=CARTESIAN_POINT ( 'NONE',  ( 1.975475456537005874E-15, -94.62499999726880162, 5.000000000000000000 ) ) ;
#9830=CARTESIAN_POINT ( 'NONE',  ( -2.500000000000000444, -6.166666666666667851, -4.330127018922193649 ) ) ;
#9835=DIRECTION ( 'NONE',  ( 0.000000000000000000, 0.000000000000000000, 1.000000000000000000 ) ) ;
#9836=CARTESIAN_POINT ( 'NONE',  ( 2.229367062500001939, -85.97916666530107932, 3.861377020970579999 ) ) ;
#9837=CARTESIAN_POINT ( 'NONE',  ( 4.458734125000001214, 18.85416666803226349, 2.574251347313718519 ) ) ;
#9839=CARTESIAN_POINT ( 'NONE',  ( 5.000000000000000000, -0.4166666666666659080, -2.886751345948130876 ) ) ;
#9843=CARTESIAN_POINT ( 'NONE',  ( -2.499999999999996447, -77.83333333333334281, 4.330127018922195425 ) ) ;
#9848=CARTESIAN_POINT ( 'NONE',  ( -2.500000000000000444, -104.1666666666666572, -4.330127018922193649 ) ) ;
#9851=AXIS2_PLACEMENT_3D ( 'NONE', #45942, #21512, #54644 ) ;
#9865=CARTESIAN_POINT ( 'NONE',  ( -2.229367062500000163, -58.72916666530106511, -3.861377020970580443 ) ) ;
#9868=ORIENTED_EDGE ( 'NONE', *, *, #20699, .F. ) ;
#9871=ADVANCED_FACE ( 'NONE', ( #28046 ), #33817, .T. ) ;
#9875=EDGE_CURVE ( 'NONE', #7933, #44977, #9369, .T. ) ;
#9876=CARTESIAN_POINT ( 'NONE',  ( 4.458734125000001214, -103.1458333319677365, 2.574251347313718519 ) ) ;
#9878=ORIENTED_EDGE ( 'NONE', *, *, #37254, .T. ) ;
#9879=EDGE_CURVE ( 'NONE', #35341, #36804, #8751, .T. ) ;
#9882=CARTESIAN_POINT ( 'NONE',  ( -4.458734124999999437, -39.31249999863440081, 0.000000000000000000 ) ) ;
#9884=EDGE_CURVE ( 'NONE', #6339, #38436, #37414, .T. ) ;
#9885=LINE ( 'NONE', #59752, #61052 ) ;
#9886=CARTESIAN_POINT ( 'NONE',  ( 1.339745962155586056, 2.419658201469705894, 5.000000000000015987 ) ) ;
#9887=CARTESIAN_POINT ( 'NONE',  ( -3.152548672688508926E-16, -12.56249999863440081, -5.148502694627439702 ) ) ;
#9888=CARTESIAN_POINT ( 'NONE',  ( 4.458734124999999437, -102.0624999986344079, -5.460374474430324690E-16 ) ) ;
#9891=CARTESIAN_POINT ( 'NONE',  ( -4.458734124999999437, -32.56249999863440792, 0.000000000000000000 ) ) ;
#9892=CARTESIAN_POINT ( 'NONE',  ( 2.499999999999998668, 5.791666669397853795, -4.330127018922193649 ) ) ;
#9899=CARTESIAN_POINT ( 'NONE',  ( 2.229367062500001939, 4.770833334698926897, 3.861377020970579999 ) ) ;
#9901=CARTESIAN_POINT ( 'NONE',  ( 2.500000000000002220, 9.333333333333332149, 4.330127018922192761 ) ) ;
#9902=CARTESIAN_POINT ( 'NONE',  ( -5.000000000000000000, -98.00000000000000000, 0.000000000000000000 ) ) ;
#9903=CARTESIAN_POINT ( 'NONE',  ( 4.458734124999998549, -28.72916666530107221, -2.574251347313721627 ) ) ;
#9905=CARTESIAN_POINT ( 'NONE',  ( -2.229367062499996610, -82.39583333196773651, 3.861377020970582219 ) ) ;
#9908=AXIS2_PLACEMENT_3D ( 'NONE', #54860, #5335, #29757 ) ;
#9911=CARTESIAN_POINT ( 'NONE',  ( -3.152548672688508926E-16, -2.562499998634407028, -5.148502694627439702 ) ) ;
#9912=CARTESIAN_POINT ( 'NONE',  ( -4.458734124999999437, 29.35416666803225993, -2.574251347313719407 ) ) ;
#9913=CARTESIAN_POINT ( 'NONE',  ( -3.152548672688508926E-16, -44.81249999863439371, -5.148502694627439702 ) ) ;
#9916=CARTESIAN_POINT ( 'NONE',  ( -3.152548672688508926E-16, -70.56249999863439371, -5.148502694627439702 ) ) ;
#9917=CARTESIAN_POINT ( 'NONE',  ( -5.000000000000000000, -103.9583333306021444, -2.886751345948128211 ) ) ;
#9922=CARTESIAN_POINT ( 'NONE',  ( -3.535250795749689387E-16, -59.25000000000000000, -5.773502691896257311 ) ) ;
#9927=CARTESIAN_POINT ( 'NONE',  ( -5.000000000000000000, -26.99999999999999645, 0.000000000000000000 ) ) ;
#9928=CARTESIAN_POINT ( 'NONE',  ( 1.975475456537005874E-15, -67.74999999999998579, 5.000000000000000000 ) ) ;
#9937=CARTESIAN_POINT ( 'NONE',  ( 6.123233995736766282E-16, -120.0000000000000000, -5.000000000000000000 ) ) ;
#9944=CARTESIAN_POINT ( 'NONE',  ( 4.458734124999999437, -43.06249999863440081, -5.460374474430324690E-16 ) ) ;
#9948=DIRECTION ( 'NONE',  ( 0.000000000000000000, 0.000000000000000000, 1.000000000000000000 ) ) ;
#9950=VECTOR ( 'NONE', #1830, 1000.000000000000000 ) ;
#9954=CARTESIAN_POINT ( 'NONE',  ( 0.000000000000000000, -120.0000000000000000, 5.000000000000000000 ) ) ;
#9956=CARTESIAN_POINT ( 'NONE',  ( 4.458734124999999437, -88.06249999863439371, -5.460374474430324690E-16 ) ) ;
#9958=( BOUNDED_CURVE ( )  B_SPLINE_CURVE ( 2, ( #39115, #10173, #44579, #54879, #34942, #54562, #39744, #30421, #43934 ),
 .UNSPECIFIED., .F., .F. ) 
 B_SPLINE_CURVE_WITH_KNOTS ( ( 3, 2, 2, 2, 3 ),
 ( 0.8017857142857143238, 0.8023809523809524169, 0.8035714285714286031, 0.8047619047619047894, 0.8053571428571428825 ),
 .UNSPECIFIED. ) 
 CURVE ( )  GEOMETRIC_REPRESENTATION_ITEM ( )  RATIONAL_B_SPLINE_CURVE ( ( 0.9330127018922194093, 0.9330127018922194093, 1.000000000000000000, 0.8660254037844387076, 1.000000000000000000, 0.8660254037844387076, 1.000000000000000000, 0.9330127018922194093, 0.9330127018922194093 ) ) 
 REPRESENTATION_ITEM ( '' )  );
#9960=EDGE_CURVE ( 'NONE', #17569, #16469, #4518, .T. ) ;
#9962=CARTESIAN_POINT ( 'NONE',  ( 4.330127018922258486, 45.00000000000000000, 7.499999999999910294 ) ) ;
#9966=ORIENTED_EDGE ( 'NONE', *, *, #23259, .T. ) ;
#9967=CARTESIAN_POINT ( 'NONE',  ( -2.229367062500000163, 2.520833334698928230, -3.861377020970580443 ) ) ;
#9970=CARTESIAN_POINT ( 'NONE',  ( 4.458734125000001214, -15.14583333196773651, 2.574251347313718519 ) ) ;
#9971=CARTESIAN_POINT ( 'NONE',  ( 0.000000000000000000, -120.0000000000000000, 0.000000000000000000 ) ) ;
#9975=CARTESIAN_POINT ( 'NONE',  ( -3.152548672688508926E-16, 22.18750000136559564, -5.148502694627439702 ) ) ;
#9977=CARTESIAN_POINT ( 'NONE',  ( 2.229367062499998831, -95.64583333196773651, -3.861377020970580887 ) ) ;
#9979=CARTESIAN_POINT ( 'NONE',  ( -5.000000000000000000, -103.8749999972688158, 0.000000000000000000 ) ) ;
#9980=CARTESIAN_POINT ( 'NONE',  ( 4.458734125000001214, -12.89583333196774184, 2.574251347313718519 ) ) ;
#9981=CARTESIAN_POINT ( 'NONE',  ( -1.339745962155613812, -85.08034179853028434, -5.000000000000000000 ) ) ;
#9984=CARTESIAN_POINT ( 'NONE',  ( -4.999999999999999112, -39.79166666393547303, 2.886751345948131764 ) ) ;
#9986=CARTESIAN_POINT ( 'NONE',  ( 4.458734125000000326, 12.10416666803226171, 2.574251347313718519 ) ) ;
#9990=CARTESIAN_POINT ( 'NONE',  ( 2.229367062500001939, -61.97916666530106511, 3.861377020970579999 ) ) ;
#9991=ORIENTED_EDGE ( 'NONE', *, *, #26810, .F. ) ;
#9993=CARTESIAN_POINT ( 'NONE',  ( 5.000000000000000000, -109.2916666639354730, -2.886751345948130876 ) ) ;
#9994=CARTESIAN_POINT ( 'NONE',  ( -4.999999999999999112, 4.083333333333334814, 2.886751345948131764 ) ) ;
#9997=CARTESIAN_POINT ( 'NONE',  ( -4.458734124999999437, -51.39583333196772941, -2.574251347313719407 ) ) ;
#9998=CARTESIAN_POINT ( 'NONE',  ( 5.000000000000000000, -90.37499999726880162, -6.123233995736766282E-16 ) ) ;
#10000=CARTESIAN_POINT ( 'NONE',  ( -3.152548672688508926E-16, -32.56249999863440792, -5.148502694627439702 ) ) ;
#10003=DIRECTION ( 'NONE',  ( 0.5000000000000069944, 0.000000000000000000, 0.8660254037844345998 ) ) ;
#10006=CARTESIAN_POINT ( 'NONE',  ( -2.499999999999996447, -44.83333333333333570, 4.330127018922195425 ) ) ;
#10007=CARTESIAN_POINT ( 'NONE',  ( -6.972266317189433020E-16, -6.124999997268813168, -5.000000000000000000 ) ) ;
#10009=VERTEX_POINT ( 'NONE', #30251 ) ;
#10010=CARTESIAN_POINT ( 'NONE',  ( 4.458734125000001214, -100.8958333319677365, 2.574251347313718519 ) ) ;
#10011=CARTESIAN_POINT ( 'NONE',  ( -2.229367062500000163, 5.270833334698927786, -3.861377020970580443 ) ) ;
#10012=( BOUNDED_CURVE ( )  B_SPLINE_CURVE ( 2, ( #27715, #47343, #22911, #18060, #62141, #8426, #3292, #25894, #42819 ),
 .UNSPECIFIED., .F., .F. ) 
 B_SPLINE_CURVE_WITH_KNOTS ( ( 3, 2, 2, 2, 3 ),
 ( 0.1053571428571428575, 0.1059523809523809507, 0.1071428571428571369, 0.1083333333333333370, 0.1089285714285714302 ),
 .UNSPECIFIED. ) 
 CURVE ( )  GEOMETRIC_REPRESENTATION_ITEM ( )  RATIONAL_B_SPLINE_CURVE ( ( 0.9330127018922194093, 0.9330127018922194093, 1.000000000000000000, 0.8660254037844387076, 1.000000000000000000, 0.8660254037844387076, 1.000000000000000000, 0.9330127018922194093, 0.9330127018922194093 ) ) 
 REPRESENTATION_ITEM ( '' )  );
#10020=ORIENTED_EDGE ( 'NONE', *, *, #22761, .F. ) ;
#10023=CARTESIAN_POINT ( 'NONE',  ( 1.975475456537005874E-15, -50.62499999726881583, 5.000000000000000000 ) ) ;
#10026=CARTESIAN_POINT ( 'NONE',  ( -4.458734124999998549, -27.47916666530106866, 2.574251347313722516 ) ) ;
#10034=ORIENTED_EDGE ( 'NONE', *, *, #4425, .F. ) ;
#10035=FACE_OUTER_BOUND ( 'NONE', #31440, .T. ) ;
#10036=ORIENTED_EDGE ( 'NONE', *, *, #25554, .T. ) ;
#10037=CARTESIAN_POINT ( 'NONE',  ( -4.458734124999999437, -71.56249999863439371, 0.000000000000000000 ) ) ;
#10038=CARTESIAN_POINT ( 'NONE',  ( -1.339745962155613146, 29.20534180126147916, 5.000000000000000000 ) ) ;
#10041=AXIS2_PLACEMENT_3D ( 'NONE', #28727, #18140, #62848 ) ;
#10045=CARTESIAN_POINT ( 'NONE',  ( 4.458734124999999437, -2.062499998634406584, -5.460374474430324690E-16 ) ) ;
#10047=DIRECTION ( 'NONE',  ( -0.000000000000000000, 1.000000000000000000, -0.000000000000000000 ) ) ;
#10048=CARTESIAN_POINT ( 'NONE',  ( -5.000000000000000000, -45.00000000000000000, 0.000000000000000000 ) ) ;
#10053=ORIENTED_EDGE ( 'NONE', *, *, #20126, .F. ) ;
#10054=CARTESIAN_POINT ( 'NONE',  ( -2.229367062499996610, -80.14583333196773651, 3.861377020970582219 ) ) ;
#10056=CARTESIAN_POINT ( 'NONE',  ( 2.229367062500001939, 0.02083333469892964529, 3.861377020970579999 ) ) ;
#10057=CARTESIAN_POINT ( 'NONE',  ( -2.500000000000000444, -83.16666666666667140, -4.330127018922193649 ) ) ;
#10058=CARTESIAN_POINT ( 'NONE',  ( -5.000000000000000000, -42.95833333060214443, -2.886751345948128211 ) ) ;
#10059=CARTESIAN_POINT ( 'NONE',  ( 4.458734124999999437, -66.06249999863440792, -5.460374474430324690E-16 ) ) ;
#10060=CARTESIAN_POINT ( 'NONE',  ( 1.060575238724906964E-15, -24.62499999726881228, 5.773502691896257311 ) ) ;
#10062=CARTESIAN_POINT ( 'NONE',  ( -4.458734124999999437, 27.60416666803226349, -2.574251347313719407 ) ) ;
#10063=CARTESIAN_POINT ( 'NONE',  ( 1.339745962155615144, -49.70534180126148271, 4.999999999999999112 ) ) ;
#10064=CARTESIAN_POINT ( 'NONE',  ( 5.000000000000000888, -43.45833333060214443, 2.886751345948126879 ) ) ;
#10065=CARTESIAN_POINT ( 'NONE',  ( -3.152548672688508926E-16, -44.56249999863440081, -5.148502694627439702 ) ) ;
#10066=CARTESIAN_POINT ( 'NONE',  ( 2.229367062500001939, -32.22916666530106511, 3.861377020970579999 ) ) ;
#10069=CARTESIAN_POINT ( 'NONE',  ( -5.000000000000000000, 19.99999999999999645, 0.000000000000000000 ) ) ;
#10073=CARTESIAN_POINT ( 'NONE',  ( -4.458734124999999437, -37.31249999863440792, 0.000000000000000000 ) ) ;
#10074=CARTESIAN_POINT ( 'NONE',  ( 5.000000000000000000, -75.37499999726880162, -6.123233995736766282E-16 ) ) ;
#10078=CARTESIAN_POINT ( 'NONE',  ( 2.229367062500001939, -80.22916666530106511, 3.861377020970579999 ) ) ;
#10081=DIRECTION ( 'NONE',  ( 0.000000000000000000, 0.000000000000000000, 1.000000000000000000 ) ) ;
#10082=CARTESIAN_POINT ( 'NONE',  ( -6.972266317189433020E-16, -18.25000000000000000, -5.000000000000000000 ) ) ;
#10083=CARTESIAN_POINT ( 'NONE',  ( -4.999999999999999112, -22.91666666666666785, 2.886751345948131764 ) ) ;
#10089=VECTOR ( 'NONE', #11206, 1000.000000000000000 ) ;
#10090=CARTESIAN_POINT ( 'NONE',  ( -4.999999999999999112, 20.20833333606451987, 2.886751345948131764 ) ) ;
#10091=DIRECTION ( 'NONE',  ( -0.000000000000000000, 1.000000000000000000, -0.000000000000000000 ) ) ;
#10094=( BOUNDED_CURVE ( )  B_SPLINE_CURVE ( 2, ( #11173, #50095, #21150, #11494, #25972, #60403, #54607, #40438, #45588 ),
 .UNSPECIFIED., .F., .F. ) 
 B_SPLINE_CURVE_WITH_KNOTS ( ( 3, 2, 2, 2, 3 ),
 ( 0.2553571428571428381, 0.2559523809523809312, 0.2571428571428571175, 0.2583333333333333592, 0.2589285714285714524 ),
 .UNSPECIFIED. ) 
 CURVE ( )  GEOMETRIC_REPRESENTATION_ITEM ( )  RATIONAL_B_SPLINE_CURVE ( ( 0.9330127018922194093, 0.9330127018922194093, 1.000000000000000000, 0.8660254037844387076, 1.000000000000000000, 0.8660254037844387076, 1.000000000000000000, 0.9330127018922194093, 0.9330127018922194093 ) ) 
 REPRESENTATION_ITEM ( '' )  );
#10098=CARTESIAN_POINT ( 'NONE',  ( -2.499999999999996447, -40.70833333060214443, 4.330127018922195425 ) ) ;
#10099=CARTESIAN_POINT ( 'NONE',  ( 5.000000000000000888, -91.45833333060214443, 2.886751345948126879 ) ) ;
#10100=CARTESIAN_POINT ( 'NONE',  ( 5.000000000000000000, -74.50000000000000000, -6.123233995736766282E-16 ) ) ;
#10102=CARTESIAN_POINT ( 'NONE',  ( -2.229367062500000163, -20.47916666530107221, -3.861377020970580443 ) ) ;
#10103=CARTESIAN_POINT ( 'NONE',  ( -2.500000000000000444, -72.04166666393548724, -4.330127018922193649 ) ) ;
#10106=AXIS2_PLACEMENT_3D ( 'NONE', #14962, #9195, #38764 ) ;
#10107=( BOUNDED_CURVE ( )  B_SPLINE_CURVE ( 2, ( #20319, #1996, #50220, #25457, #5847, #30274, #35754, #31233, #35122 ),
 .UNSPECIFIED., .F., .F. ) 
 B_SPLINE_CURVE_WITH_KNOTS ( ( 3, 2, 2, 2, 3 ),
 ( 0.5553571428571428825, 0.5559523809523809756, 0.5571428571428571619, 0.5583333333333333481, 0.5589285714285714413 ),
 .UNSPECIFIED. ) 
 CURVE ( )  GEOMETRIC_REPRESENTATION_ITEM ( )  RATIONAL_B_SPLINE_CURVE ( ( 0.9330127018922194093, 0.9330127018922194093, 1.000000000000000000, 0.8660254037844387076, 1.000000000000000000, 0.8660254037844387076, 1.000000000000000000, 0.9330127018922194093, 0.9330127018922194093 ) ) 
 REPRESENTATION_ITEM ( '' )  );
#10117=DIRECTION ( 'NONE',  ( 0.000000000000000000, 0.000000000000000000, 1.000000000000000000 ) ) ;
#10122=CARTESIAN_POINT ( 'NONE',  ( 5.000000000000000888, -103.4583333306021444, 2.886751345948126879 ) ) ;
#10123=CARTESIAN_POINT ( 'NONE',  ( -4.458734124999999437, 17.68750000136559208, 0.000000000000000000 ) ) ;
#10124=FACE_OUTER_BOUND ( 'NONE', #16131, .T. ) ;
#10125=ORIENTED_EDGE ( 'NONE', *, *, #7139, .T. ) ;
#10128=CARTESIAN_POINT ( 'NONE',  ( 5.000000000000000000, 12.62500000273118417, -6.123233995736766282E-16 ) ) ;
#10131=CARTESIAN_POINT ( 'NONE',  ( -2.500000000000000444, -103.1666666666666572, -4.330127018922193649 ) ) ;
#10132=CARTESIAN_POINT ( 'NONE',  ( -2.229367062499996610, -65.14583333196773651, 3.861377020970582219 ) ) ;
#10133=DIRECTION ( 'NONE',  ( -0.000000000000000000, 1.000000000000000000, -0.000000000000000000 ) ) ;
#10134=CARTESIAN_POINT ( 'NONE',  ( -2.229367062499996610, 17.85416666803225993, 3.861377020970582219 ) ) ;
#10137=CARTESIAN_POINT ( 'NONE',  ( -4.458734124999999437, -47.64583333196775072, -2.574251347313719407 ) ) ;
#10138=CARTESIAN_POINT ( 'NONE',  ( -5.000000000000000000, -11.95833333060214976, -2.886751345948128211 ) ) ;
#10139=CARTESIAN_POINT ( 'NONE',  ( 5.000000000000000000, -25.29166666393547658, -2.886751345948130876 ) ) ;
#10141=CARTESIAN_POINT ( 'NONE',  ( 2.229367062499998831, -107.6458333319677365, -3.861377020970580887 ) ) ;
#10142=CARTESIAN_POINT ( 'NONE',  ( -4.458734124999999437, -16.64583333196773651, -2.574251347313719407 ) ) ;
#10145=CARTESIAN_POINT ( 'NONE',  ( 9.457646018065525792E-16, -100.0624999986344221, 5.148502694627439702 ) ) ;
#10147=CARTESIAN_POINT ( 'NONE',  ( -2.229367062500000163, -95.72916666530107932, -3.861377020970580443 ) ) ;
#10150=CARTESIAN_POINT ( 'NONE',  ( 5.000000000000000888, -58.45833333060214443, 2.886751345948126879 ) ) ;
#10152=AXIS2_PLACEMENT_3D ( 'NONE', #14982, #10160, #45849 ) ;
#10155=CARTESIAN_POINT ( 'NONE',  ( 4.458734124999999437, -18.81249999863440792, -5.460374474430324690E-16 ) ) ;
#10156=CARTESIAN_POINT ( 'NONE',  ( 4.458734124999999437, 6.937500001365594748, -5.460374474430324690E-16 ) ) ;
#10157=CARTESIAN_POINT ( 'NONE',  ( -3.152548672688508926E-16, -56.81249999863440792, -5.148502694627439702 ) ) ;
#10160=DIRECTION ( 'NONE',  ( -0.000000000000000000, 1.000000000000000000, -0.000000000000000000 ) ) ;
#10162=CARTESIAN_POINT ( 'NONE',  ( 1.060575238724906964E-15, -4.749999999999997335, 5.773502691896257311 ) ) ;
#10163=EDGE_LOOP ( 'NONE', ( #45809, #7119, #61825, #20977 ) ) ;
#10165=( BOUNDED_CURVE ( )  B_SPLINE_CURVE ( 2, ( #28658, #44075, #53421, #48274, #9667, #4230, #23845, #24156, #53734 ),
 .UNSPECIFIED., .F., .F. ) 
 B_SPLINE_CURVE_WITH_KNOTS ( ( 3, 2, 2, 2, 3 ),
 ( 0.5374999999999999778, 0.5380952380952380709, 0.5392857142857142572, 0.5404761904761904434, 0.5410714285714285365 ),
 .UNSPECIFIED. ) 
 CURVE ( )  GEOMETRIC_REPRESENTATION_ITEM ( )  RATIONAL_B_SPLINE_CURVE ( ( 0.9330127018922194093, 0.9330127018922194093, 1.000000000000000000, 0.8660254037844387076, 1.000000000000000000, 0.8660254037844387076, 1.000000000000000000, 0.9330127018922194093, 0.9330127018922194093 ) ) 
 REPRESENTATION_ITEM ( '' )  );
#10166=FACE_OUTER_BOUND ( 'NONE', #48771, .T. ) ;
#10167=CARTESIAN_POINT ( 'NONE',  ( -6.972266317189433020E-16, -92.12499999726878741, -5.000000000000000000 ) ) ;
#10169=CARTESIAN_POINT ( 'NONE',  ( -3.152548672688508926E-16, -92.56249999863439371, -5.148502694627439702 ) ) ;
#10170=CARTESIAN_POINT ( 'NONE',  ( 4.458734124999998549, 18.02083333469892779, -2.574251347313721627 ) ) ;
#10173=CARTESIAN_POINT ( 'NONE',  ( 1.339745962155612702, -82.29465819873851729, -5.000000000000000000 ) ) ;
#10174=EDGE_CURVE ( 'NONE', #483, #44925, #29288, .T. ) ;
#10175=CARTESIAN_POINT ( 'NONE',  ( 1.975475456537005874E-15, -29.62499999726881228, 5.000000000000000000 ) ) ;
#10178=CARTESIAN_POINT ( 'NONE',  ( -2.500000000000000444, -76.16666666666665719, -4.330127018922193649 ) ) ;
#10183=CARTESIAN_POINT ( 'NONE',  ( 1.975475456537005874E-15, -54.62499999726880873, 5.000000000000000000 ) ) ;
#10186=VECTOR ( 'NONE', #23588, 1000.000000000000000 ) ;
#10187=EDGE_CURVE ( 'NONE', #42151, #45889, #53748, .T. ) ;
#10189=VERTEX_POINT ( 'NONE', #15152 ) ;
#10193=ORIENTED_EDGE ( 'NONE', *, *, #3416, .T. ) ;
#10196=CARTESIAN_POINT ( 'NONE',  ( -4.458734124999999437, -63.56249999863440792, 0.000000000000000000 ) ) ;
#10198=CYLINDRICAL_SURFACE ( 'NONE', #54968, 5.000000000000000000 ) ;
#10202=CARTESIAN_POINT ( 'NONE',  ( 1.975475456537005874E-15, -52.62499999726880873, 5.000000000000000000 ) ) ;
#10203=ORIENTED_EDGE ( 'NONE', *, *, #39652, .T. ) ;
#10206=CARTESIAN_POINT ( 'NONE',  ( -4.458734124999999437, -103.5624999986344079, 0.000000000000000000 ) ) ;
#10212=CARTESIAN_POINT ( 'NONE',  ( 2.229367062500001939, -45.97916666530106511, 3.861377020970579999 ) ) ;
#10215=CARTESIAN_POINT ( 'NONE',  ( -2.229367062500000163, -15.47916666530107399, -3.861377020970580443 ) ) ;
#10216=CARTESIAN_POINT ( 'NONE',  ( -2.499999999999996447, -100.8333333333333286, 4.330127018922195425 ) ) ;
#10218=CARTESIAN_POINT ( 'NONE',  ( 4.458734124999999437, -34.06249999863440792, -5.460374474430324690E-16 ) ) ;
#10219=CARTESIAN_POINT ( 'NONE',  ( 5.000000000000000888, 5.541666669397854683, 2.886751345948126879 ) ) ;
#10220=FACE_OUTER_BOUND ( 'NONE', #21430, .T. ) ;
#10223=CARTESIAN_POINT ( 'NONE',  ( -6.972266317189433020E-16, -92.24999999999998579, -5.000000000000000000 ) ) ;
#10224=CARTESIAN_POINT ( 'NONE',  ( 0.000000000000000000, -120.0000000000000000, 0.000000000000000000 ) ) ;
#10227=CARTESIAN_POINT ( 'NONE',  ( 4.458734124999998549, 4.020833334698926009, -2.574251347313721627 ) ) ;
#10228=ORIENTED_EDGE ( 'NONE', *, *, #21593, .F. ) ;
#10229=CARTESIAN_POINT ( 'NONE',  ( -6.972266317189433020E-16, -30.25000000000000000, -5.000000000000000000 ) ) ;
#10230=CARTESIAN_POINT ( 'NONE',  ( 6.123233995736766282E-16, -120.0000000000000000, -5.000000000000000000 ) ) ;
#10231=CARTESIAN_POINT ( 'NONE',  ( 5.000000000000000000, -98.41666666666667140, -2.886751345948129988 ) ) ;
#10232=CARTESIAN_POINT ( 'NONE',  ( -3.152548672688508926E-16, -31.56249999863440436, -5.148502694627439702 ) ) ;
#10234=CARTESIAN_POINT ( 'NONE',  ( 9.457646018065525792E-16, -83.31249999863440792, 5.148502694627439702 ) ) ;
#10239=EDGE_CURVE ( 'NONE', #143, #55022, #30835, .T. ) ;
#10240=EDGE_CURVE ( 'NONE', #39571, #57126, #60504, .T. ) ;
#10241=CARTESIAN_POINT ( 'NONE',  ( -3.152548672688508926E-16, -1.562499998634406140, -5.148502694627439702 ) ) ;
#10242=CARTESIAN_POINT ( 'NONE',  ( 4.458734125000001214, 19.85416666803226349, 2.574251347313718519 ) ) ;
#10243=CARTESIAN_POINT ( 'NONE',  ( 4.458734124999998549, -41.97916666530107932, -2.574251347313721627 ) ) ;
#10244=CARTESIAN_POINT ( 'NONE',  ( 2.500000000000002220, -15.66666666666666963, 4.330127018922192761 ) ) ;
#10248=CARTESIAN_POINT ( 'NONE',  ( 4.458734124999998549, -67.72916666530107932, -2.574251347313721627 ) ) ;
#10249=CARTESIAN_POINT ( 'NONE',  ( -2.499999999999996447, -106.7083333306021444, 4.330127018922195425 ) ) ;
#10250=EDGE_CURVE ( 'NONE', #4248, #36690, #1741, .T. ) ;
#10252=CARTESIAN_POINT ( 'NONE',  ( 1.975475456537005874E-15, -101.7499999999999858, 5.000000000000000000 ) ) ;
#10256=CARTESIAN_POINT ( 'NONE',  ( 1.060575238724906964E-15, -57.75000000000000000, 5.773502691896257311 ) ) ;
#10261=CARTESIAN_POINT ( 'NONE',  ( -4.999999999999998224, -98.91666666666667140, 2.886751345948131764 ) ) ;
#10267=VERTEX_POINT ( 'NONE', #61142 ) ;
#10268=CARTESIAN_POINT ( 'NONE',  ( 5.000000000000000000, -35.37499999726881583, -6.123233995736766282E-16 ) ) ;
#10269=CARTESIAN_POINT ( 'NONE',  ( 5.000000000000000000, -98.41666666666668561, -2.886751345948130876 ) ) ;
#10275=CARTESIAN_POINT ( 'NONE',  ( -4.458734124999998549, -41.47916666530107221, 2.574251347313722516 ) ) ;
#10278=AXIS2_PLACEMENT_3D ( 'NONE', #27578, #43622, #47517 ) ;
#10284=CARTESIAN_POINT ( 'NONE',  ( 4.458734124999998549, -89.97916666530105090, -2.574251347313721627 ) ) ;
#10287=CARTESIAN_POINT ( 'NONE',  ( -1.339745962155613812, -32.20534180126148271, -5.000000000000000000 ) ) ;
#10290=CARTESIAN_POINT ( 'NONE',  ( 5.000000000000000000, -82.37499999726881583, -6.123233995736766282E-16 ) ) ;
#10292=CARTESIAN_POINT ( 'NONE',  ( -2.229367062499996610, 3.854166668032260823, 3.861377020970582219 ) ) ;
#10293=( BOUNDED_CURVE ( )  B_SPLINE_CURVE ( 2, ( #2552, #50487, #45653, #61414, #6426, #41132, #55319, #41764, #46290 ),
 .UNSPECIFIED., .F., .F. ) 
 B_SPLINE_CURVE_WITH_KNOTS ( ( 3, 2, 2, 2, 3 ),
 ( 0.2053571428571428492, 0.2059523809523809423, 0.2071428571428571563, 0.2083333333333333426, 0.2089285714285714357 ),
 .UNSPECIFIED. ) 
 CURVE ( )  GEOMETRIC_REPRESENTATION_ITEM ( )  RATIONAL_B_SPLINE_CURVE ( ( 0.9330127018922194093, 0.9330127018922194093, 1.000000000000000000, 0.8660254037844387076, 1.000000000000000000, 0.8660254037844387076, 1.000000000000000000, 0.9330127018922194093, 0.9330127018922194093 ) ) 
 REPRESENTATION_ITEM ( '' )  );
#10295=CARTESIAN_POINT ( 'NONE',  ( 4.458734125000001214, -17.14583333196773651, 2.574251347313718519 ) ) ;
#10297=CARTESIAN_POINT ( 'NONE',  ( 1.975475456537005874E-15, -44.62499999726880162, 5.000000000000000000 ) ) ;
#10299=CARTESIAN_POINT ( 'NONE',  ( -2.229367062499996610, 19.60416666803225993, 3.861377020970582219 ) ) ;
#10301=CARTESIAN_POINT ( 'NONE',  ( 2.229367062500001939, -99.97916666530106511, 3.861377020970579999 ) ) ;
#10302=CARTESIAN_POINT ( 'NONE',  ( 4.458734125000001214, -13.89583333196774007, 2.574251347313718519 ) ) ;
#10303=CARTESIAN_POINT ( 'NONE',  ( 0.000000000000000000, -120.0000000000000000, 0.000000000000000000 ) ) ;
#10304=CYLINDRICAL_SURFACE ( 'NONE', #52037, 5.000000000000000000 ) ;
#10306=ADVANCED_FACE ( 'NONE', ( #46972 ), #6785, .T. ) ;
#10307=CARTESIAN_POINT ( 'NONE',  ( -5.000000000000000000, -39.95833333060213732, -2.886751345948128211 ) ) ;
#10309=CARTESIAN_POINT ( 'NONE',  ( -3.152548672688508926E-16, 14.43750000136559386, -5.148502694627439702 ) ) ;
#10312=CARTESIAN_POINT ( 'NONE',  ( 4.458734124999999437, -60.81249999863440081, -5.460374474430324690E-16 ) ) ;
#10317=CARTESIAN_POINT ( 'NONE',  ( -3.535250795749689387E-16, 5.749999999999998224, -5.773502691896257311 ) ) ;
#10319=CARTESIAN_POINT ( 'NONE',  ( -1.339745962155610925, -98.66965819600734733, 5.000000000000000000 ) ) ;
#10320=CARTESIAN_POINT ( 'NONE',  ( -2.229367062499996610, -53.14583333196773651, 3.861377020970582219 ) ) ;
#10321=CARTESIAN_POINT ( 'NONE',  ( 5.000000000000000000, -89.37499999726880162, -6.123233995736766282E-16 ) ) ;
#10322=CARTESIAN_POINT ( 'NONE',  ( -2.229367062500000163, -32.47916666530106511, -3.861377020970580443 ) ) ;
#10323=EDGE_CURVE ( 'NONE', #45276, #58623, #12239, .T. ) ;
#10326=CARTESIAN_POINT ( 'NONE',  ( -6.972266317189433020E-16, -108.1249999972688158, -5.000000000000000000 ) ) ;
#10328=CARTESIAN_POINT ( 'NONE',  ( 5.000000000000000888, -41.58333333333332860, 2.886751345948126879 ) ) ;
#10332=VERTEX_POINT ( 'NONE', #37313 ) ;
#10333=CARTESIAN_POINT ( 'NONE',  ( 9.457646018065525792E-16, -99.06249999863440792, 5.148502694627439702 ) ) ;
#10334=CARTESIAN_POINT ( 'NONE',  ( -4.458734124999998549, 3.520833334698929118, 2.574251347313722516 ) ) ;
#10338=CARTESIAN_POINT ( 'NONE',  ( -5.000000000000000000, 2.916666666666668739, -2.886751345948128211 ) ) ;
#10339=EDGE_CURVE ( 'NONE', #7464, #23303, #32482, .T. ) ;
#10344=ORIENTED_EDGE ( 'NONE', *, *, #53805, .T. ) ;
#10347=CYLINDRICAL_SURFACE ( 'NONE', #62418, 5.000000000000000000 ) ;
#10349=CARTESIAN_POINT ( 'NONE',  ( 9.457646018065525792E-16, -26.31249999863440792, 5.148502694627439702 ) ) ;
#10359=ORIENTED_EDGE ( 'NONE', *, *, #55866, .T. ) ;
#10360=CARTESIAN_POINT ( 'NONE',  ( -4.458734124999999437, -72.64583333196773651, -2.574251347313719407 ) ) ;
#10365=VECTOR ( 'NONE', #45144, 1000.000000000000000 ) ;
#10367=CARTESIAN_POINT ( 'NONE',  ( -3.152548672688508926E-16, -5.812499998634404363, -5.148502694627439702 ) ) ;
#10369=LINE ( 'NONE', #19699, #21400 ) ;
#10376=VERTEX_POINT ( 'NONE', #2920 ) ;
#10377=CARTESIAN_POINT ( 'NONE',  ( -4.458734124999999437, -82.39583333196773651, -2.574251347313719407 ) ) ;
#10379=CARTESIAN_POINT ( 'NONE',  ( -4.458734124999999437, 3.687500001365594748, 0.000000000000000000 ) ) ;
#10380=CARTESIAN_POINT ( 'NONE',  ( 2.500000000000002220, -83.66666666666667140, 4.330127018922192761 ) ) ;
#10382=CARTESIAN_POINT ( 'NONE',  ( 4.458734124999999437, -65.06249999863440792, -5.460374474430324690E-16 ) ) ;
#10383=CARTESIAN_POINT ( 'NONE',  ( -5.000000000000000000, -22.95833333060214798, -2.886751345948128211 ) ) ;
#10385=CARTESIAN_POINT ( 'NONE',  ( 4.458734124999998549, 27.27083333469892779, -2.574251347313721627 ) ) ;
#10386=CARTESIAN_POINT ( 'NONE',  ( -2.500000000000000444, -38.04166666393548013, -4.330127018922193649 ) ) ;
#10387=CARTESIAN_POINT ( 'NONE',  ( 5.000000000000000888, -3.458333330602147093, 2.886751345948126879 ) ) ;
#10388=CARTESIAN_POINT ( 'NONE',  ( 2.229367062500001939, -44.97916666530106511, 3.861377020970579999 ) ) ;
#10389=CARTESIAN_POINT ( 'NONE',  ( 4.458734124999999437, -30.06249999863440436, -5.460374474430324690E-16 ) ) ;
#10393=CARTESIAN_POINT ( 'NONE',  ( 5.000000000000000000, 18.50000000000000000, -6.123233995736766282E-16 ) ) ;
#10395=CARTESIAN_POINT ( 'NONE',  ( -5.000000000000000000, -50.00000000000000000, 0.000000000000000000 ) ) ;
#10396=CARTESIAN_POINT ( 'NONE',  ( 2.229367062500001939, -37.97916666530107221, 3.861377020970579999 ) ) ;
#10397=CARTESIAN_POINT ( 'NONE',  ( -3.535250795749689387E-16, -72.12499999726881583, -5.773502691896257311 ) ) ;
#10400=CARTESIAN_POINT ( 'NONE',  ( 5.000000000000000000, -15.37499999726881228, -6.123233995736766282E-16 ) ) ;
#10401=CARTESIAN_POINT ( 'NONE',  ( -2.229367062500000163, -79.72916666530106511, -3.861377020970580443 ) ) ;
#10403=CARTESIAN_POINT ( 'NONE',  ( 1.339745962155612702, 18.83034180399265978, -5.000000000000000000 ) ) ;
#10404=CARTESIAN_POINT ( 'NONE',  ( 0.000000000000000000, -120.0000000000000000, 0.000000000000000000 ) ) ;
#10405=CARTESIAN_POINT ( 'NONE',  ( -2.500000000000000444, -26.16666666666666430, -4.330127018922193649 ) ) ;
#10409=ORIENTED_EDGE ( 'NONE', *, *, #18156, .F. ) ;
#10411=CARTESIAN_POINT ( 'NONE',  ( -5.000000000000000000, 23.04166666939785557, -2.886751345948128211 ) ) ;
#10414=VECTOR ( 'NONE', #4729, 1000.000000000000000 ) ;
#10419=CARTESIAN_POINT ( 'NONE',  ( 1.339745962155615144, -91.58034179853028434, 4.999999999999999112 ) ) ;
#10422=CARTESIAN_POINT ( 'NONE',  ( -4.458734124999999437, -21.39583333196774007, -2.574251347313719407 ) ) ;
#10429=ORIENTED_EDGE ( 'NONE', *, *, #29547, .T. ) ;
#10431=CARTESIAN_POINT ( 'NONE',  ( -2.500000000000000444, -29.16666666666666785, -4.330127018922193649 ) ) ;
#10433=VERTEX_POINT ( 'NONE', #27657 ) ;
#10434=CARTESIAN_POINT ( 'NONE',  ( -4.999999999999998224, 11.08333333333333393, 2.886751345948131764 ) ) ;
#10436=CARTESIAN_POINT ( 'NONE',  ( -6.972266317189433020E-16, -86.25000000000001421, -5.000000000000000000 ) ) ;
#10438=ORIENTED_EDGE ( 'NONE', *, *, #53617, .F. ) ;
#10440=CARTESIAN_POINT ( 'NONE',  ( -4.458734124999999437, 14.68750000136559386, 0.000000000000000000 ) ) ;
#10446=CARTESIAN_POINT ( 'NONE',  ( 4.458734124999999437, -65.81249999863440792, -5.460374474430324690E-16 ) ) ;
#10448=CARTESIAN_POINT ( 'NONE',  ( -2.229367062499996610, 18.85416666803225993, 3.861377020970582219 ) ) ;
#10449=CARTESIAN_POINT ( 'NONE',  ( 4.458734124999998549, -50.97916666530107221, -2.574251347313721627 ) ) ;
#10450=CARTESIAN_POINT ( 'NONE',  ( -3.535250795749689387E-16, -10.12499999726881583, -5.773502691896257311 ) ) ;
#10455=CARTESIAN_POINT ( 'NONE',  ( 4.458734124999999437, -18.06249999863440792, -5.460374474430324690E-16 ) ) ;
#10457=CARTESIAN_POINT ( 'NONE',  ( -5.000000000000000000, -46.95833333060214443, -2.886751345948128211 ) ) ;
#10458=CARTESIAN_POINT ( 'NONE',  ( -4.458734124999998549, -105.2291666653010651, 2.574251347313722516 ) ) ;
#10461=CARTESIAN_POINT ( 'NONE',  ( -4.458734124999999437, -95.64583333196772230, -2.574251347313719407 ) ) ;
#10463=CARTESIAN_POINT ( 'NONE',  ( -4.999999999999999112, -57.79166666393548013, 2.886751345948131764 ) ) ;
#10465=( BOUNDED_CURVE ( )  B_SPLINE_CURVE ( 2, ( #52057, #2235, #32105, #21839, #26976, #27911, #23097, #56571, #61084 ),
 .UNSPECIFIED., .F., .F. ) 
 B_SPLINE_CURVE_WITH_KNOTS ( ( 3, 2, 2, 2, 3 ),
 ( 0.4160714285714285920, 0.4166666666666666852, 0.4178571428571428714, 0.4190476190476190577, 0.4196428571428571508 ),
 .UNSPECIFIED. ) 
 CURVE ( )  GEOMETRIC_REPRESENTATION_ITEM ( )  RATIONAL_B_SPLINE_CURVE ( ( 0.9330127018922194093, 0.9330127018922194093, 1.000000000000000000, 0.8660254037844387076, 1.000000000000000000, 0.8660254037844387076, 1.000000000000000000, 0.9330127018922194093, 0.9330127018922194093 ) ) 
 REPRESENTATION_ITEM ( '' )  );
#10468=CARTESIAN_POINT ( 'NONE',  ( 4.458734124999999437, -17.81249999863440792, -5.460374474430324690E-16 ) ) ;
#10469=CARTESIAN_POINT ( 'NONE',  ( 2.229367062500001939, 6.770833334698928674, 3.861377020970579999 ) ) ;
#10470=CARTESIAN_POINT ( 'NONE',  ( 2.229367062500001939, -63.22916666530106511, 3.861377020970579999 ) ) ;
#10475=CARTESIAN_POINT ( 'NONE',  ( -5.000000000000000000, -13.08333333333333570, -2.886751345948128211 ) ) ;
#10480=CARTESIAN_POINT ( 'NONE',  ( -2.500000000000000444, -92.04166666393547303, -4.330127018922193649 ) ) ;
#10482=CARTESIAN_POINT ( 'NONE',  ( 4.458734124999998549, -91.72916666530106511, -2.574251347313721627 ) ) ;
#10483=CARTESIAN_POINT ( 'NONE',  ( -4.458734124999999437, 13.35416666803225993, -2.574251347313719407 ) ) ;
#10486=FACE_OUTER_BOUND ( 'NONE', #6270, .T. ) ;
#10488=CARTESIAN_POINT ( 'NONE',  ( -2.499999999999996447, -73.83333333333332860, 4.330127018922195425 ) ) ;
#10492=ORIENTED_EDGE ( 'NONE', *, *, #43620, .T. ) ;
#10493=CARTESIAN_POINT ( 'NONE',  ( -4.999999999999998224, -50.91666666666666430, 2.886751345948131764 ) ) ;
#10496=ORIENTED_EDGE ( 'NONE', *, *, #38212, .F. ) ;
#10499=ORIENTED_EDGE ( 'NONE', *, *, #13111, .F. ) ;
#10502=CARTESIAN_POINT ( 'NONE',  ( 4.458734125000001214, -65.14583333196773651, 2.574251347313718519 ) ) ;
#10505=ORIENTED_EDGE ( 'NONE', *, *, #9091, .F. ) ;
#10513=CARTESIAN_POINT ( 'NONE',  ( 2.229367062499998831, -108.8958333319677365, -3.861377020970580887 ) ) ;
#10519=CARTESIAN_POINT ( 'NONE',  ( 4.458734124999998549, -45.72916666530106511, -2.574251347313721627 ) ) ;
#10522=CARTESIAN_POINT ( 'NONE',  ( 2.229367062500001939, -49.97916666530107221, 3.861377020970579999 ) ) ;
#10523=CARTESIAN_POINT ( 'NONE',  ( -6.972266317189433020E-16, -71.25000000000000000, -5.000000000000000000 ) ) ;
#10524=CARTESIAN_POINT ( 'NONE',  ( -2.229367062499996610, -11.14583333196773829, 3.861377020970582219 ) ) ;
#10525=CARTESIAN_POINT ( 'NONE',  ( 2.499999999999998668, -99.33333333333332860, -4.330127018922193649 ) ) ;
#10528=CARTESIAN_POINT ( 'NONE',  ( -2.229367062500000163, -34.72916666530107221, -3.861377020970580443 ) ) ;
#10529=EDGE_CURVE ( 'NONE', #33480, #3482, #6235, .T. ) ;
#10530=CARTESIAN_POINT ( 'NONE',  ( -5.000000000000000000, 9.041666669397852019, -2.886751345948128211 ) ) ;
#10537=CARTESIAN_POINT ( 'NONE',  ( 4.458734124999998549, -1.979166665301068662, -2.574251347313721627 ) ) ;
#10538=( BOUNDED_CURVE ( )  B_SPLINE_CURVE ( 2, ( #15854, #20689, #12923, #32224, #51855, #47651, #3605, #18064, #37686 ),
 .UNSPECIFIED., .F., .F. ) 
 B_SPLINE_CURVE_WITH_KNOTS ( ( 3, 2, 2, 2, 3 ),
 ( 0.2410714285714285754, 0.2416666666666666685, 0.2428571428571428548, 0.2440476190476190410, 0.2446428571428571341 ),
 .UNSPECIFIED. ) 
 CURVE ( )  GEOMETRIC_REPRESENTATION_ITEM ( )  RATIONAL_B_SPLINE_CURVE ( ( 0.9330127018922194093, 0.9330127018922194093, 1.000000000000000000, 0.8660254037844387076, 1.000000000000000000, 0.8660254037844387076, 1.000000000000000000, 0.9330127018922194093, 0.9330127018922194093 ) ) 
 REPRESENTATION_ITEM ( '' )  );
#10542=CARTESIAN_POINT ( 'NONE',  ( 4.458734124999999437, -86.81249999863439371, -5.460374474430324690E-16 ) ) ;
#10543=CARTESIAN_POINT ( 'NONE',  ( 2.229367062499998831, -37.64583333196773651, -3.861377020970580887 ) ) ;
#10545=CARTESIAN_POINT ( 'NONE',  ( 2.229367062499998831, -78.89583333196773651, -3.861377020970580887 ) ) ;
#10547=CARTESIAN_POINT ( 'NONE',  ( -1.339745962155613812, -53.20534180126147561, -5.000000000000000000 ) ) ;
#10550=CARTESIAN_POINT ( 'NONE',  ( -2.229367062500000163, -2.479166665301069106, -3.861377020970580443 ) ) ;
#10551=CARTESIAN_POINT ( 'NONE',  ( -2.229367062500000163, 21.27083333469892779, -3.861377020970580443 ) ) ;
#10552=CARTESIAN_POINT ( 'NONE',  ( -3.152548672688508926E-16, -48.81249999863440792, -5.148502694627439702 ) ) ;
#10553=CARTESIAN_POINT ( 'NONE',  ( -1.339745962155613812, -46.08034179853028434, -5.000000000000000000 ) ) ;
#10557=CARTESIAN_POINT ( 'NONE',  ( -2.229367062499996610, -75.14583333196773651, 3.861377020970582219 ) ) ;
#10558=CARTESIAN_POINT ( 'NONE',  ( -3.535250795749689387E-16, -105.1249999972688158, -5.773502691896257311 ) ) ;
#10562=CARTESIAN_POINT ( 'NONE',  ( 6.123233995736766282E-16, -120.0000000000000000, -5.000000000000000000 ) ) ;
#10564=CARTESIAN_POINT ( 'NONE',  ( -2.500000000000000444, -57.16666666666667140, -4.330127018922193649 ) ) ;
#10565=CARTESIAN_POINT ( 'NONE',  ( -6.972266317189433020E-16, -75.25000000000000000, -5.000000000000000000 ) ) ;
#10567=ORIENTED_EDGE ( 'NONE', *, *, #10240, .F. ) ;
#10576=ORIENTED_EDGE ( 'NONE', *, *, #10882, .T. ) ;
#10579=VERTEX_POINT ( 'NONE', #1839 ) ;
#10583=CARTESIAN_POINT ( 'NONE',  ( -4.458734124999999437, -47.56249999863440792, 0.000000000000000000 ) ) ;
#10588=ADVANCED_FACE ( 'NONE', ( #25941 ), #21442, .T. ) ;
#10591=CARTESIAN_POINT ( 'NONE',  ( 1.975475456537005874E-15, -89.74999999999998579, 5.000000000000000000 ) ) ;
#10593=CARTESIAN_POINT ( 'NONE',  ( 2.229367062499998831, -95.89583333196773651, -3.861377020970580887 ) ) ;
#10594=CARTESIAN_POINT ( 'NONE',  ( -1.339745962155610925, -106.7946581987385173, 5.000000000000000000 ) ) ;
#10596=CARTESIAN_POINT ( 'NONE',  ( -2.500000000000000444, -32.16666666666666430, -4.330127018922193649 ) ) ;
#10601=CARTESIAN_POINT ( 'NONE',  ( -4.458734124999999437, 2.604166668032263043, -2.574251347313719407 ) ) ;
#10602=VECTOR ( 'NONE', #15116, 1000.000000000000000 ) ;
#10603=CARTESIAN_POINT ( 'NONE',  ( 2.500000000000002220, -106.6666666666666572, 4.330127018922192761 ) ) ;
#10604=CARTESIAN_POINT ( 'NONE',  ( -4.458734124999998549, -16.47916666530107577, 2.574251347313722516 ) ) ;
#10605=EDGE_CURVE ( 'NONE', #62971, #53159, #25944, .T. ) ;
#10606=CARTESIAN_POINT ( 'NONE',  ( -2.499999999999996447, -100.8333333333333286, 4.330127018922195425 ) ) ;
#10608=EDGE_CURVE ( 'NONE', #3031, #6430, #56773, .T. ) ;
#10611=CARTESIAN_POINT ( 'NONE',  ( 4.458734125000000326, 17.85416666803225993, 2.574251347313718519 ) ) ;
#10613=CARTESIAN_POINT ( 'NONE',  ( -4.458734124999997661, -96.22916666530105090, 2.574251347313722516 ) ) ;
#10614=CARTESIAN_POINT ( 'NONE',  ( -2.500000000000000444, -19.04166666393547658, -4.330127018922193649 ) ) ;
#10615=CARTESIAN_POINT ( 'NONE',  ( 0.000000000000000000, -120.0000000000000000, 0.000000000000000000 ) ) ;
#10616=CARTESIAN_POINT ( 'NONE',  ( 4.458734124999999437, -16.81249999863440436, -5.460374474430324690E-16 ) ) ;
#10618=CARTESIAN_POINT ( 'NONE',  ( 2.500000000000002220, -3.666666666666665186, 4.330127018922192761 ) ) ;
#10620=CARTESIAN_POINT ( 'NONE',  ( -2.500000000000000444, -44.04166666393546592, -4.330127018922193649 ) ) ;
#10622=CARTESIAN_POINT ( 'NONE',  ( -4.458734124999999437, 12.68750000136559564, 0.000000000000000000 ) ) ;
#10626=CARTESIAN_POINT ( 'NONE',  ( -3.152548672688508926E-16, -62.56249999863440792, -5.148502694627439702 ) ) ;
#10627=ORIENTED_EDGE ( 'NONE', *, *, #46144, .T. ) ;
#10629=CARTESIAN_POINT ( 'NONE',  ( -2.499999999999996447, 7.166666666666665186, 4.330127018922195425 ) ) ;
#10631=CARTESIAN_POINT ( 'NONE',  ( -4.999999999999998224, -98.79166666393544460, 2.886751345948131764 ) ) ;
#10632=CARTESIAN_POINT ( 'NONE',  ( -4.458734124999999437, -57.31249999863440081, 0.000000000000000000 ) ) ;
#10633=CARTESIAN_POINT ( 'NONE',  ( 5.000000000000000000, -88.37499999726880162, -6.123233995736766282E-16 ) ) ;
#10635=CARTESIAN_POINT ( 'NONE',  ( -4.458734124999999437, -32.31249999863440792, 0.000000000000000000 ) ) ;
#10636=DIRECTION ( 'NONE',  ( -0.000000000000000000, 1.000000000000000000, -0.000000000000000000 ) ) ;
#10638=CARTESIAN_POINT ( 'NONE',  ( -4.999999999999998224, -107.7916666639354730, 2.886751345948131764 ) ) ;
#10641=CARTESIAN_POINT ( 'NONE',  ( 5.000000000000000000, -43.41666666666666430, -2.886751345948129988 ) ) ;
#10642=CARTESIAN_POINT ( 'NONE',  ( -5.000000000000000000, 18.91666666666666430, -2.886751345948128211 ) ) ;
#10645=CARTESIAN_POINT ( 'NONE',  ( 2.229367062500001939, -101.9791666653010651, 3.861377020970579999 ) ) ;
#10646=CARTESIAN_POINT ( 'NONE',  ( 2.229367062500001939, 4.770833334698926897, 3.861377020970579999 ) ) ;
#10655=CARTESIAN_POINT ( 'NONE',  ( 1.975475456537005874E-15, -76.75000000000000000, 5.000000000000000000 ) ) ;
#10656=CARTESIAN_POINT ( 'NONE',  ( -1.339745962155610925, -16.66965819600733312, 5.000000000000000000 ) ) ;
#10658=LINE ( 'NONE', #60840, #50469 ) ;
#10661=CARTESIAN_POINT ( 'NONE',  ( -2.229367062499996610, -28.39583333196774007, 3.861377020970582219 ) ) ;
#10668=( BOUNDED_CURVE ( )  B_SPLINE_CURVE ( 2, ( #20054, #10403, #49323, #39980, #35178, #39658, #44170, #30331, #49957 ),
 .UNSPECIFIED., .F., .F. ) 
 B_SPLINE_CURVE_WITH_KNOTS ( ( 3, 2, 2, 2, 3 ),
 ( 0.07321428571428571785, 0.07380952380952381098, 0.07499999999999999722, 0.07619047619047619735, 0.07678571428571429047 ),
 .UNSPECIFIED. ) 
 CURVE ( )  GEOMETRIC_REPRESENTATION_ITEM ( )  RATIONAL_B_SPLINE_CURVE ( ( 0.9330127018922194093, 0.9330127018922194093, 1.000000000000000000, 0.8660254037844387076, 1.000000000000000000, 0.8660254037844387076, 1.000000000000000000, 0.9330127018922194093, 0.9330127018922194093 ) ) 
 REPRESENTATION_ITEM ( '' )  );
#10671=EDGE_CURVE ( 'NONE', #14391, #7881, #41910, .T. ) ;
#10674=CARTESIAN_POINT ( 'NONE',  ( 4.458734124999998549, -74.97916666530106511, -2.574251347313721627 ) ) ;
#10677=ORIENTED_EDGE ( 'NONE', *, *, #23458, .F. ) ;
#10680=CARTESIAN_POINT ( 'NONE',  ( -2.500000000000000444, 7.833333333333334814, -4.330127018922193649 ) ) ;
#10683=CARTESIAN_POINT ( 'NONE',  ( 2.229367062499998831, -2.895833331967738289, -3.861377020970580887 ) ) ;
#10686=CARTESIAN_POINT ( 'NONE',  ( -2.499999999999996447, 3.291666669397851575, 4.330127018922195425 ) ) ;
#10687=CARTESIAN_POINT ( 'NONE',  ( -2.500000000000000444, -45.16666666666665719, -4.330127018922193649 ) ) ;
#10688=EDGE_CURVE ( 'NONE', #45629, #43365, #12798, .T. ) ;
#10689=ADVANCED_FACE ( 'NONE', ( #14615 ), #15261, .T. ) ;
#10694=CARTESIAN_POINT ( 'NONE',  ( -6.972266317189433020E-16, -102.1249999972688158, -5.000000000000000000 ) ) ;
#10695=ORIENTED_EDGE ( 'NONE', *, *, #37272, .T. ) ;
#10696=EDGE_CURVE ( 'NONE', #54583, #15515, #27, .T. ) ;
#10697=CARTESIAN_POINT ( 'NONE',  ( 9.457646018065525792E-16, -81.06249999863440792, 5.148502694627439702 ) ) ;
#10698=EDGE_CURVE ( 'NONE', #2721, #18523, #55299, .T. ) ;
#10699=CARTESIAN_POINT ( 'NONE',  ( 2.499999999999998668, -75.33333333333332860, -4.330127018922193649 ) ) ;
#10700=CARTESIAN_POINT ( 'NONE',  ( -3.152548672688508926E-16, -0.5624999986344053626, -5.148502694627439702 ) ) ;
#10704=CARTESIAN_POINT ( 'NONE',  ( -4.458734124999999437, -71.64583333196773651, -2.574251347313719407 ) ) ;
#10705=CARTESIAN_POINT ( 'NONE',  ( 2.499999999999998668, -27.20833333060214798, -4.330127018922193649 ) ) ;
#10708=CARTESIAN_POINT ( 'NONE',  ( 1.975475456537005874E-15, -110.6249999972688158, 5.000000000000000000 ) ) ;
#10709=PLANE ( 'NONE',  #8998 ) ;
#10710=CARTESIAN_POINT ( 'NONE',  ( 2.229367062499998831, -44.64583333196774362, -3.861377020970580887 ) ) ;
#10711=CARTESIAN_POINT ( 'NONE',  ( -2.229367062499996610, -34.39583333196772941, 3.861377020970582219 ) ) ;
#10714=CARTESIAN_POINT ( 'NONE',  ( -5.000000000000000000, 23.00000000000000000, 0.000000000000000000 ) ) ;
#10716=LINE ( 'NONE', #438, #33604 ) ;
#10717=CARTESIAN_POINT ( 'NONE',  ( -4.458734124999998549, -38.22916666530107932, 2.574251347313722516 ) ) ;
#10718=CARTESIAN_POINT ( 'NONE',  ( -4.999999999999999112, -74.79166666393547303, 2.886751345948131764 ) ) ;
#10720=CARTESIAN_POINT ( 'NONE',  ( 2.500000000000002220, -24.54166666393548368, 4.330127018922192761 ) ) ;
#10722=CARTESIAN_POINT ( 'NONE',  ( -3.152548672688508926E-16, -81.81249999863440792, -5.148502694627439702 ) ) ;
#10724=( BOUNDED_CURVE ( )  B_SPLINE_CURVE ( 2, ( #46674, #46036, #8080, #60843, #61795, #51511, #32506, #37649, #52138 ),
 .UNSPECIFIED., .F., .F. ) 
 B_SPLINE_CURVE_WITH_KNOTS ( ( 3, 2, 2, 2, 3 ),
 ( 0.2839285714285714191, 0.2845238095238095122, 0.2857142857142856984, 0.2869047619047618847, 0.2874999999999999778 ),
 .UNSPECIFIED. ) 
 CURVE ( )  GEOMETRIC_REPRESENTATION_ITEM ( )  RATIONAL_B_SPLINE_CURVE ( ( 0.9330127018922194093, 0.9330127018922194093, 1.000000000000000000, 0.8660254037844387076, 1.000000000000000000, 0.8660254037844387076, 1.000000000000000000, 0.9330127018922194093, 0.9330127018922194093 ) ) 
 REPRESENTATION_ITEM ( '' )  );
#10726=CARTESIAN_POINT ( 'NONE',  ( -5.000000000000000000, -26.00000000000000355, 0.000000000000000000 ) ) ;
#10728=ORIENTED_EDGE ( 'NONE', *, *, #61829, .F. ) ;
#10730=ORIENTED_EDGE ( 'NONE', *, *, #58870, .T. ) ;
#10732=( BOUNDED_CURVE ( )  B_SPLINE_CURVE ( 2, ( #31006, #12021, #56101, #41285, #31651, #7219, #34772, #25437, #54397 ),
 .UNSPECIFIED., .F., .F. ) 
 B_SPLINE_CURVE_WITH_KNOTS ( ( 3, 2, 2, 2, 3 ),
 ( 0.2732142857142857428, 0.2738095238095238360, 0.2750000000000000222, 0.2761904761904762085, 0.2767857142857143016 ),
 .UNSPECIFIED. ) 
 CURVE ( )  GEOMETRIC_REPRESENTATION_ITEM ( )  RATIONAL_B_SPLINE_CURVE ( ( 0.9330127018922194093, 0.9330127018922225179, 1.000000000000000000, 0.8660254037844387076, 1.000000000000000000, 0.8660254037844387076, 1.000000000000000000, 0.9330127018922194093, 0.9330127018922194093 ) ) 
 REPRESENTATION_ITEM ( '' )  );
#10733=CARTESIAN_POINT ( 'NONE',  ( -5.000000000000000000, 19.12500000273118772, 0.000000000000000000 ) ) ;
#10739=CARTESIAN_POINT ( 'NONE',  ( 1.339745962155615144, 15.41965820146970678, 4.999999999999999112 ) ) ;
#10740=CARTESIAN_POINT ( 'NONE',  ( -5.000000000000000000, 0.000000000000000000, 0.000000000000000000 ) ) ;
#10741=CARTESIAN_POINT ( 'NONE',  ( 2.500000000000002220, 28.45833333606451987, 4.330127018922192761 ) ) ;
#10742=CARTESIAN_POINT ( 'NONE',  ( 0.000000000000000000, -120.0000000000000000, 5.000000000000000000 ) ) ;
#10744=CARTESIAN_POINT ( 'NONE',  ( 2.229367062500001939, -20.97916666530107221, 3.861377020970579999 ) ) ;
#10745=CARTESIAN_POINT ( 'NONE',  ( 1.975475456537005874E-15, -77.62499999726881583, 5.000000000000000000 ) ) ;
#10751=CARTESIAN_POINT ( 'NONE',  ( 5.000000000000000000, 13.49999999999999822, -6.123233995736766282E-16 ) ) ;
#10753=ORIENTED_EDGE ( 'NONE', *, *, #34641, .T. ) ;
#10756=CARTESIAN_POINT ( 'NONE',  ( -6.972266317189433020E-16, -3.250000000000001332, -5.000000000000000000 ) ) ;
#10762=EDGE_LOOP ( 'NONE', ( #61650, #42630, #333, #803 ) ) ;
#10764=CARTESIAN_POINT ( 'NONE',  ( 2.229367062499998831, 15.35416666803225993, -3.861377020970580887 ) ) ;
#10768=CYLINDRICAL_SURFACE ( 'NONE', #21306, 5.000000000000000000 ) ;
#10772=CARTESIAN_POINT ( 'NONE',  ( 9.457646018065525792E-16, -63.06249999863440792, 5.148502694627439702 ) ) ;
#10774=CARTESIAN_POINT ( 'NONE',  ( 4.458734124999999437, 16.18750000136559564, -5.460374474430324690E-16 ) ) ;
#10778=CARTESIAN_POINT ( 'NONE',  ( 4.458734125000001214, -47.14583333196774362, 2.574251347313718519 ) ) ;
#10779=CARTESIAN_POINT ( 'NONE',  ( 2.499999999999998668, -10.20833333060214621, -4.330127018922193649 ) ) ;
#10783=DIRECTION ( 'NONE',  ( -0.000000000000000000, 1.000000000000000000, -0.000000000000000000 ) ) ;
#10784=CARTESIAN_POINT ( 'NONE',  ( -3.152548672688508926E-16, -16.81249999863440436, -5.148502694627439702 ) ) ;
#10785=ORIENTED_EDGE ( 'NONE', *, *, #43292, .T. ) ;
#10787=CARTESIAN_POINT ( 'NONE',  ( 2.229367062500001939, -102.9791666653010651, 3.861377020970579999 ) ) ;
#10790=CARTESIAN_POINT ( 'NONE',  ( 4.458734125000001214, -99.14583333196773651, 2.574251347313718519 ) ) ;
#10791=CARTESIAN_POINT ( 'NONE',  ( -4.999999999999999112, -58.79166666393546592, 2.886751345948131764 ) ) ;
#10794=CARTESIAN_POINT ( 'NONE',  ( -2.229367062500000163, -22.47916666530107221, -3.861377020970580443 ) ) ;
#10795=CARTESIAN_POINT ( 'NONE',  ( 9.457646018065525792E-16, 6.687500001365594748, 5.148502694627439702 ) ) ;
#10796=CARTESIAN_POINT ( 'NONE',  ( -2.229367062499996610, -66.39583333196773651, 3.861377020970582219 ) ) ;
#10801=CARTESIAN_POINT ( 'NONE',  ( -4.999999999999999112, -10.91666666666666607, 2.886751345948131764 ) ) ;
#10813=CARTESIAN_POINT ( 'NONE',  ( 5.000000000000000000, -77.41666666666665719, -2.886751345948129988 ) ) ;
#10816=CARTESIAN_POINT ( 'NONE',  ( 5.000000000000000888, -80.45833333060213022, 2.886751345948126879 ) ) ;
#10818=CARTESIAN_POINT ( 'NONE',  ( -6.972266317189433020E-16, -85.25000000000000000, -5.000000000000000000 ) ) ;
#10820=EDGE_CURVE ( 'NONE', #31465, #14946, #39076, .T. ) ;
#10822=EDGE_LOOP ( 'NONE', ( #62279, #10677, #1242, #56827 ) ) ;
#10824=VERTEX_POINT ( 'NONE', #63207 ) ;
#10832=FACE_OUTER_BOUND ( 'NONE', #59269, .T. ) ;
#10833=ORIENTED_EDGE ( 'NONE', *, *, #29647, .T. ) ;
#10836=CARTESIAN_POINT ( 'NONE',  ( -4.458734124999999437, 27.68750000136559208, 0.000000000000000000 ) ) ;
#10841=CARTESIAN_POINT ( 'NONE',  ( -2.229367062499996610, -42.14583333196773651, 3.861377020970582219 ) ) ;
#10844=CARTESIAN_POINT ( 'NONE',  ( 4.458734124999999437, -50.81249999863440792, -5.460374474430324690E-16 ) ) ;
#10845=CARTESIAN_POINT ( 'NONE',  ( -5.000000000000000000, -71.08333333333332860, -2.886751345948128211 ) ) ;
#10846=CARTESIAN_POINT ( 'NONE',  ( 2.229367062500001939, -17.97916666530106866, 3.861377020970579999 ) ) ;
#10848=CARTESIAN_POINT ( 'NONE',  ( 1.060575238724906964E-15, -100.7500000000000000, 5.773502691896257311 ) ) ;
#10850=CARTESIAN_POINT ( 'NONE',  ( -2.229367062499996610, -32.39583333196773651, 3.861377020970582219 ) ) ;
#10851=CARTESIAN_POINT ( 'NONE',  ( -4.999999999999999112, 9.208333336064519870, 2.886751345948131764 ) ) ;
#10858=CARTESIAN_POINT ( 'NONE',  ( -4.458734124999999437, 0.4375000013655955255, 0.000000000000000000 ) ) ;
#10860=CARTESIAN_POINT ( 'NONE',  ( -6.972266317189433020E-16, -54.12499999726880162, -5.000000000000000000 ) ) ;
#10862=CARTESIAN_POINT ( 'NONE',  ( -4.458734124999999437, -86.39583333196772230, -2.574251347313719407 ) ) ;
#10863=CARTESIAN_POINT ( 'NONE',  ( 4.458734124999998549, -37.72916666530107221, -2.574251347313721627 ) ) ;
#10864=DIRECTION ( 'NONE',  ( -0.000000000000000000, 1.000000000000000000, -0.000000000000000000 ) ) ;
#10865=CARTESIAN_POINT ( 'NONE',  ( 2.229367062499998831, -82.89583333196773651, -3.861377020970580887 ) ) ;
#10867=CARTESIAN_POINT ( 'NONE',  ( 0.000000000000000000, -120.0000000000000000, 0.000000000000000000 ) ) ;
#10869=( BOUNDED_CURVE ( )  B_SPLINE_CURVE ( 2, ( #43860, #20394, #39358, #33907, #24579, #35191, #53531, #5280, #34214 ),
 .UNSPECIFIED., .F., .F. ) 
 B_SPLINE_CURVE_WITH_KNOTS ( ( 3, 2, 2, 2, 3 ),
 ( 0.1839285714285714413, 0.1845238095238095344, 0.1857142857142857206, 0.1869047619047619069, 0.1875000000000000000 ),
 .UNSPECIFIED. ) 
 CURVE ( )  GEOMETRIC_REPRESENTATION_ITEM ( )  RATIONAL_B_SPLINE_CURVE ( ( 0.9330127018922194093, 0.9330127018922209636, 1.000000000000000000, 0.8660254037844387076, 1.000000000000000000, 0.8660254037844387076, 1.000000000000000000, 0.9330127018922194093, 0.9330127018922194093 ) ) 
 REPRESENTATION_ITEM ( '' )  );
#10870=CARTESIAN_POINT ( 'NONE',  ( -2.229367062499996610, -3.145833331967738733, 3.861377020970582219 ) ) ;
#10871=CARTESIAN_POINT ( 'NONE',  ( -4.458734124999999437, 22.43750000136559564, 0.000000000000000000 ) ) ;
#10872=CARTESIAN_POINT ( 'NONE',  ( -2.229367062500000163, -47.72916666530106511, -3.861377020970580443 ) ) ;
#10876=AXIS2_PLACEMENT_3D ( 'NONE', #40501, #11553, #45969 ) ;
#10880=CARTESIAN_POINT ( 'NONE',  ( 4.458734125000001214, -75.89583333196775072, 2.574251347313718519 ) ) ;
#10881=CARTESIAN_POINT ( 'NONE',  ( -4.458734124999999437, 29.43750000136559208, 0.000000000000000000 ) ) ;
#10882=EDGE_CURVE ( 'NONE', #44517, #50477, #19739, .T. ) ;
#10884=CARTESIAN_POINT ( 'NONE',  ( 6.123233995736766282E-16, -120.0000000000000000, -5.000000000000000000 ) ) ;
#10887=CARTESIAN_POINT ( 'NONE',  ( -3.535250795749689387E-16, -57.25000000000000000, -5.773502691896257311 ) ) ;
#10888=CARTESIAN_POINT ( 'NONE',  ( 1.339745962155615144, -90.58034179853029855, 4.999999999999999112 ) ) ;
#10892=CARTESIAN_POINT ( 'NONE',  ( -6.972266317189433020E-16, -99.24999999999998579, -5.000000000000000000 ) ) ;
#10900=CYLINDRICAL_SURFACE ( 'NONE', #13046, 5.000000000000000000 ) ;
#10901=CARTESIAN_POINT ( 'NONE',  ( 6.158835246850666199E-14, -1.250000000000002442, -4.999999999999999112 ) ) ;
#10903=ORIENTED_EDGE ( 'NONE', *, *, #32893, .F. ) ;
#10907=CARTESIAN_POINT ( 'NONE',  ( -4.458734124999999437, -46.56249999863440792, 0.000000000000000000 ) ) ;
#10910=CARTESIAN_POINT ( 'NONE',  ( -1.339745962155610925, -81.66965819600736154, 5.000000000000000000 ) ) ;
#10916=CARTESIAN_POINT ( 'NONE',  ( 2.229367062500001939, -94.22916666530106511, 3.861377020970579999 ) ) ;
#10917=ORIENTED_EDGE ( 'NONE', *, *, #34941, .F. ) ;
#10918=CARTESIAN_POINT ( 'NONE',  ( -5.000000000000000000, -32.00000000000000000, 0.000000000000000000 ) ) ;
#10921=( BOUNDED_CURVE ( )  B_SPLINE_CURVE ( 2, ( #60564, #25177, #50903, #60252, #49936, #21002, #30315, #2034, #21639 ),
 .UNSPECIFIED., .F., .F. ) 
 B_SPLINE_CURVE_WITH_KNOTS ( ( 3, 2, 2, 2, 3 ),
 ( 0.6125000000000000444, 0.6130952380952381375, 0.6142857142857143238, 0.6154761904761905100, 0.6160714285714286031 ),
 .UNSPECIFIED. ) 
 CURVE ( )  GEOMETRIC_REPRESENTATION_ITEM ( )  RATIONAL_B_SPLINE_CURVE ( ( 0.9330127018922194093, 0.9330127018922194093, 1.000000000000000000, 0.8660254037844387076, 1.000000000000000000, 0.8660254037844387076, 1.000000000000000000, 0.9330127018922194093, 0.9330127018922194093 ) ) 
 REPRESENTATION_ITEM ( '' )  );
#10922=CARTESIAN_POINT ( 'NONE',  ( 1.975475456537005874E-15, -100.6249999972688016, 5.000000000000000000 ) ) ;
#10924=CARTESIAN_POINT ( 'NONE',  ( -2.229367062499996610, -4.145833331967739177, 3.861377020970582219 ) ) ;
#10925=VECTOR ( 'NONE', #56690, 1000.000000000000000 ) ;
#10927=CARTESIAN_POINT ( 'NONE',  ( -2.229367062499996610, -16.39583333196773651, 3.861377020970582219 ) ) ;
#10930=CARTESIAN_POINT ( 'NONE',  ( 1.339745962155612702, -55.16965819600732601, -5.000000000000000000 ) ) ;
#10932=CARTESIAN_POINT ( 'NONE',  ( 2.229367062499998831, 18.10416666803225993, -3.861377020970580887 ) ) ;
#10934=CARTESIAN_POINT ( 'NONE',  ( -4.458734124999999437, -20.31249999863440081, 0.000000000000000000 ) ) ;
#10938=CARTESIAN_POINT ( 'NONE',  ( -2.500000000000000444, -46.04166666393547303, -4.330127018922193649 ) ) ;
#10939=CARTESIAN_POINT ( 'NONE',  ( -4.458734124999997661, 14.77083333469892779, 2.574251347313722516 ) ) ;
#10941=CARTESIAN_POINT ( 'NONE',  ( -2.499999999999996447, -47.70833333060215153, 4.330127018922195425 ) ) ;
#10943=CARTESIAN_POINT ( 'NONE',  ( 2.229367062499998831, -68.64583333196773651, -3.861377020970580887 ) ) ;
#10946=( BOUNDED_CURVE ( )  B_SPLINE_CURVE ( 2, ( #5712, #54919, #578, #15996, #53954, #10845, #39471, #15679, #10523 ),
 .UNSPECIFIED., .F., .F. ) 
 B_SPLINE_CURVE_WITH_KNOTS ( ( 3, 2, 2, 2, 3 ),
 ( 0.7196428571428571397, 0.7202380952380952328, 0.7214285714285714191, 0.7226190476190476053, 0.7232142857142856984 ),
 .UNSPECIFIED. ) 
 CURVE ( )  GEOMETRIC_REPRESENTATION_ITEM ( )  RATIONAL_B_SPLINE_CURVE ( ( 0.9330127018922194093, 0.9330127018922194093, 1.000000000000000000, 0.8660254037844387076, 1.000000000000000000, 0.8660254037844387076, 1.000000000000000000, 0.9330127018922194093, 0.9330127018922194093 ) ) 
 REPRESENTATION_ITEM ( '' )  );
#10947=CARTESIAN_POINT ( 'NONE',  ( 2.499999999999998668, 2.666666666666667851, -4.330127018922193649 ) ) ;
#10949=CARTESIAN_POINT ( 'NONE',  ( -2.500000000000000444, 25.95833333606451632, -4.330127018922193649 ) ) ;
#10950=CARTESIAN_POINT ( 'NONE',  ( 9.457646018065525792E-16, -60.06249999863440792, 5.148502694627439702 ) ) ;
#10951=CARTESIAN_POINT ( 'NONE',  ( -3.535250795749689387E-16, -95.12499999726881583, -5.773502691896257311 ) ) ;
#10952=EDGE_CURVE ( 'NONE', #21555, #55752, #55073, .T. ) ;
#10953=CARTESIAN_POINT ( 'NONE',  ( -3.152548672688508926E-16, -35.56249999863440792, -5.148502694627439702 ) ) ;
#10956=CARTESIAN_POINT ( 'NONE',  ( -5.000000000000000000, -107.8749999972687874, 0.000000000000000000 ) ) ;
#10957=CARTESIAN_POINT ( 'NONE',  ( -5.000000000000000000, -78.95833333060213022, -2.886751345948128211 ) ) ;
#10959=CARTESIAN_POINT ( 'NONE',  ( -4.999999999999999112, -44.91666666666666430, 2.886751345948131764 ) ) ;
#10961=CARTESIAN_POINT ( 'NONE',  ( 5.000000000000000888, -17.45833333060214443, 2.886751345948126879 ) ) ;
#10963=CARTESIAN_POINT ( 'NONE',  ( -4.458734124999999437, -104.3124999986344079, 0.000000000000000000 ) ) ;
#10964=CARTESIAN_POINT ( 'NONE',  ( 2.229367062499998831, 3.104166668032259935, -3.861377020970580887 ) ) ;
#10965=AXIS2_PLACEMENT_3D ( 'NONE', #34120, #53743, #24799 ) ;
#10966=CARTESIAN_POINT ( 'NONE',  ( -5.000000000000000000, -96.87499999726881583, 0.000000000000000000 ) ) ;
#10968=EDGE_CURVE ( 'NONE', #55556, #36504, #52253, .T. ) ;
#10969=AXIS2_PLACEMENT_3D ( 'NONE', #57820, #43941, #24979 ) ;
#10975=CARTESIAN_POINT ( 'NONE',  ( 2.499999999999998668, -22.20833333060215153, -4.330127018922193649 ) ) ;
#10976=EDGE_CURVE ( 'NONE', #24051, #57423, #35522, .T. ) ;
#10978=ORIENTED_EDGE ( 'NONE', *, *, #62040, .F. ) ;
#10981=CARTESIAN_POINT ( 'NONE',  ( 2.229367062500001939, -32.22916666530106511, 3.861377020970579999 ) ) ;
#10988=ORIENTED_EDGE ( 'NONE', *, *, #22101, .T. ) ;
#10989=CARTESIAN_POINT ( 'NONE',  ( -1.339745962155610925, -82.66965819600731891, 5.000000000000000000 ) ) ;
#10991=CARTESIAN_POINT ( 'NONE',  ( -4.458734124999999437, -80.64583333196773651, -2.574251347313719407 ) ) ;
#10992=CARTESIAN_POINT ( 'NONE',  ( -1.339745962155610925, 13.33034180399266688, 5.000000000000000000 ) ) ;
#10994=CARTESIAN_POINT ( 'NONE',  ( 0.000000000000000000, -120.0000000000000000, 0.000000000000000000 ) ) ;
#10997=CARTESIAN_POINT ( 'NONE',  ( -4.458734124999999437, -3.645833331967739621, -2.574251347313719407 ) ) ;
#10999=CARTESIAN_POINT ( 'NONE',  ( 4.769696007084727185, -120.0000000000000000, -1.500000000000000444 ) ) ;
#11001=CARTESIAN_POINT ( 'NONE',  ( 0.000000000000000000, -120.0000000000000000, 0.000000000000000000 ) ) ;
#11006=AXIS2_PLACEMENT_3D ( 'NONE', #29329, #4911, #34476 ) ;
#11008=CARTESIAN_POINT ( 'NONE',  ( -2.229367062500000163, -80.47916666530106511, -3.861377020970580443 ) ) ;
#11009=CARTESIAN_POINT ( 'NONE',  ( 1.975475456537005874E-15, -96.75000000000000000, 5.000000000000000000 ) ) ;
#11010=CARTESIAN_POINT ( 'NONE',  ( 4.458734124999999437, -4.812499998634402587, -5.460374474430324690E-16 ) ) ;
#11011=AXIS2_PLACEMENT_3D ( 'NONE', #2670, #42526, #33202 ) ;
#11014=CARTESIAN_POINT ( 'NONE',  ( 2.229367062500001939, -68.22916666530106511, 3.861377020970579999 ) ) ;
#11015=AXIS2_PLACEMENT_3D ( 'NONE', #63633, #54612, #40124 ) ;
#11016=CARTESIAN_POINT ( 'NONE',  ( -3.535250795749689387E-16, -33.12499999726881583, -5.773502691896257311 ) ) ;
#11017=CARTESIAN_POINT ( 'NONE',  ( -2.499999999999996447, -14.83333333333333037, 4.330127018922195425 ) ) ;
#11018=CARTESIAN_POINT ( 'NONE',  ( -2.229367062499996610, 27.85416666803225993, 3.861377020970582219 ) ) ;
#11019=CARTESIAN_POINT ( 'NONE',  ( 5.000000000000000000, -110.3749999972688016, -6.123233995736766282E-16 ) ) ;
#11021=CARTESIAN_POINT ( 'NONE',  ( -2.229367062500000163, -53.47916666530107221, -3.861377020970580443 ) ) ;
#11022=CARTESIAN_POINT ( 'NONE',  ( 2.229367062499998831, -34.89583333196772941, -3.861377020970580887 ) ) ;
#11025=CARTESIAN_POINT ( 'NONE',  ( -3.535250795749689387E-16, 22.75000000000000000, -5.773502691896257311 ) ) ;
#11027=CARTESIAN_POINT ( 'NONE',  ( -2.229367062500000163, -41.47916666530107932, -3.861377020970580443 ) ) ;
#11028=CARTESIAN_POINT ( 'NONE',  ( -2.499999999999996447, -73.70833333060214443, 4.330127018922195425 ) ) ;
#11031=EDGE_CURVE ( 'NONE', #14930, #25261, #32906, .T. ) ;
#11032=CARTESIAN_POINT ( 'NONE',  ( 6.123233995736766282E-16, -120.0000000000000000, -5.000000000000000000 ) ) ;
#11033=EDGE_CURVE ( 'NONE', #10332, #40250, #11386, .T. ) ;
#11034=CARTESIAN_POINT ( 'NONE',  ( 2.229367062500001939, -78.22916666530106511, 3.861377020970579999 ) ) ;
#11037=FACE_OUTER_BOUND ( 'NONE', #26186, .T. ) ;
#11038=CARTESIAN_POINT ( 'NONE',  ( 2.499999999999998668, -27.33333333333333570, -4.330127018922193649 ) ) ;
#11040=ORIENTED_EDGE ( 'NONE', *, *, #8031, .F. ) ;
#11044=CARTESIAN_POINT ( 'NONE',  ( 2.499999999999998668, 21.79166666939785202, -4.330127018922193649 ) ) ;
#11047=EDGE_CURVE ( 'NONE', #27288, #63081, #61277, .T. ) ;
#11052=CARTESIAN_POINT ( 'NONE',  ( 5.000000000000000000, -99.37499999726881583, -6.123233995736766282E-16 ) ) ;
#11054=EDGE_CURVE ( 'NONE', #12980, #50712, #10732, .T. ) ;
#11055=CARTESIAN_POINT ( 'NONE',  ( 5.000000000000000888, 28.54166666939784847, 2.886751345948126879 ) ) ;
#11058=CARTESIAN_POINT ( 'NONE',  ( 4.458734124999998549, -14.97916666530107221, -2.574251347313721627 ) ) ;
#11059=AXIS2_PLACEMENT_3D ( 'NONE', #5953, #21063, #4985 ) ;
#11066=ORIENTED_EDGE ( 'NONE', *, *, #15869, .F. ) ;
#11067=CARTESIAN_POINT ( 'NONE',  ( 0.000000000000000000, -120.0000000000000000, 0.000000000000000000 ) ) ;
#11069=VERTEX_POINT ( 'NONE', #15480 ) ;
#11076=CARTESIAN_POINT ( 'NONE',  ( 2.499999999999998668, 15.66666666666666607, -4.330127018922193649 ) ) ;
#11079=CARTESIAN_POINT ( 'NONE',  ( -6.972266317189433020E-16, -110.1249999972688158, -5.000000000000000000 ) ) ;
#11080=CARTESIAN_POINT ( 'NONE',  ( 4.458734124999999437, 12.18750000136559564, -5.460374474430324690E-16 ) ) ;
#11083=CARTESIAN_POINT ( 'NONE',  ( -6.972266317189433020E-16, 12.87500000273118417, -5.000000000000000000 ) ) ;
#11084=CARTESIAN_POINT ( 'NONE',  ( 6.123233995736766282E-16, -120.0000000000000000, -5.000000000000000000 ) ) ;
#11085=CARTESIAN_POINT ( 'NONE',  ( 4.458734124999999437, -64.81249999863440792, -5.460374474430324690E-16 ) ) ;
#11087=CARTESIAN_POINT ( 'NONE',  ( -3.152548672688508926E-16, 12.43750000136559564, -5.148502694627439702 ) ) ;
#11090=CARTESIAN_POINT ( 'NONE',  ( 2.229367062500001939, -53.22916666530107221, 3.861377020970579999 ) ) ;
#11091=CARTESIAN_POINT ( 'NONE',  ( -2.499999999999996447, -7.708333330602144429, 4.330127018922195425 ) ) ;
#11092=CARTESIAN_POINT ( 'NONE',  ( 1.339745962155612702, -25.16965819600734022, -5.000000000000000000 ) ) ;
#11096=CARTESIAN_POINT ( 'NONE',  ( 2.229367062499998831, -16.89583333196773651, -3.861377020970580887 ) ) ;
#11099=AXIS2_PLACEMENT_3D ( 'NONE', #47709, #23277, #47400 ) ;
#11100=CARTESIAN_POINT ( 'NONE',  ( -2.229367062499996610, -104.1458333319677365, 3.861377020970582219 ) ) ;
#11103=CARTESIAN_POINT ( 'NONE',  ( -4.458734124999998549, -95.47916666530106511, 2.574251347313722516 ) ) ;
#11104=CARTESIAN_POINT ( 'NONE',  ( -2.229367062499996610, -25.14583333196773651, 3.861377020970582219 ) ) ;
#11105=CARTESIAN_POINT ( 'NONE',  ( 1.060575238724906964E-15, -57.62499999726880873, 5.773502691896257311 ) ) ;
#11109=CARTESIAN_POINT ( 'NONE',  ( 2.229367062499998831, -23.64583333196773651, -3.861377020970580887 ) ) ;
#11110=CARTESIAN_POINT ( 'NONE',  ( 4.458734125000000326, -65.14583333196773651, 2.574251347313718519 ) ) ;
#11111=CARTESIAN_POINT ( 'NONE',  ( 4.330127018922154569, 45.00000000000000000, -7.499999999999971578 ) ) ;
#11114=CARTESIAN_POINT ( 'NONE',  ( -2.500000000000000444, -13.16666666666666607, -4.330127018922193649 ) ) ;
#11118=CARTESIAN_POINT ( 'NONE',  ( -5.000000000000000000, -38.08333333333333570, -2.886751345948128211 ) ) ;
#11124=FACE_OUTER_BOUND ( 'NONE', #12824, .T. ) ;
#11127=CARTESIAN_POINT ( 'NONE',  ( -2.500000000000000444, -79.16666666666665719, -4.330127018922193649 ) ) ;
#11133=CARTESIAN_POINT ( 'NONE',  ( -2.480964764533239819E-13, -108.6249999972688016, 5.000000000000000000 ) ) ;
#11139=VERTEX_POINT ( 'NONE', #20300 ) ;
#11144=AXIS2_PLACEMENT_3D ( 'NONE', #61503, #38835, #62127 ) ;
#11145=( BOUNDED_CURVE ( )  B_SPLINE_CURVE ( 2, ( #23415, #19435, #39047, #9772, #28219, #27284, #44189, #43017, #29379 ),
 .UNSPECIFIED., .F., .F. ) 
 B_SPLINE_CURVE_WITH_KNOTS ( ( 3, 2, 2, 2, 3 ),
 ( 0.08035714285714286309, 0.08095238095238095621, 0.08214285714285714246, 0.08333333333333332871, 0.08392857142857143571 ),
 .UNSPECIFIED. ) 
 CURVE ( )  GEOMETRIC_REPRESENTATION_ITEM ( )  RATIONAL_B_SPLINE_CURVE ( ( 0.9330127018922192983, 0.9330127018922200755, 1.000000000000000000, 0.8660254037844387076, 1.000000000000000000, 0.8660254037844387076, 1.000000000000000000, 0.9330127018922185211, 0.9330127018922192983 ) ) 
 REPRESENTATION_ITEM ( '' )  );
#11153=VERTEX_POINT ( 'NONE', #44091 ) ;
#11155=CARTESIAN_POINT ( 'NONE',  ( 2.229367062499998831, -78.64583333196773651, -3.861377020970580887 ) ) ;
#11156=CARTESIAN_POINT ( 'NONE',  ( -4.458734124999999437, -109.6458333319677365, -2.574251347313719407 ) ) ;
#11158=ORIENTED_EDGE ( 'NONE', *, *, #39188, .T. ) ;
#11163=CARTESIAN_POINT ( 'NONE',  ( 4.458734124999998549, -43.72916666530106511, -2.574251347313721627 ) ) ;
#11165=CARTESIAN_POINT ( 'NONE',  ( -3.152548672688508926E-16, -51.56249999863440792, -5.148502694627439702 ) ) ;
#11168=CARTESIAN_POINT ( 'NONE',  ( 9.457646018065525792E-16, -17.06249999863440792, 5.148502694627439702 ) ) ;
#11169=CARTESIAN_POINT ( 'NONE',  ( 5.000000000000000888, -99.58333333333334281, 2.886751345948126879 ) ) ;
#11171=CARTESIAN_POINT ( 'NONE',  ( 2.229367062499998831, -37.89583333196773651, -3.861377020970580887 ) ) ;
#11172=CARTESIAN_POINT ( 'NONE',  ( 2.499999999999998668, 8.791666669397853795, -4.330127018922193649 ) ) ;
#11173=CARTESIAN_POINT ( 'NONE',  ( 1.975475456537005874E-15, -6.624999997268813168, 5.000000000000000000 ) ) ;
#11177=FACE_OUTER_BOUND ( 'NONE', #24271, .T. ) ;
#11178=CARTESIAN_POINT ( 'NONE',  ( 4.458734124999998549, 0.02083333469892617584, -2.574251347313721627 ) ) ;
#11180=CARTESIAN_POINT ( 'NONE',  ( 1.339745962155612702, -30.29465819873851729, -5.000000000000000000 ) ) ;
#11181=DIRECTION ( 'NONE',  ( -0.000000000000000000, 1.000000000000000000, -0.000000000000000000 ) ) ;
#11182=CARTESIAN_POINT ( 'NONE',  ( 4.458734124999998549, -85.72916666530106511, -2.574251347313721627 ) ) ;
#11183=CARTESIAN_POINT ( 'NONE',  ( 4.458734124999999437, -36.81249999863440792, -5.460374474430324690E-16 ) ) ;
#11184=DIRECTION ( 'NONE',  ( -0.000000000000000000, 1.000000000000000000, -0.000000000000000000 ) ) ;
#11185=CARTESIAN_POINT ( 'NONE',  ( 2.229367062500001939, -80.22916666530106511, 3.861377020970579999 ) ) ;
#11190=CARTESIAN_POINT ( 'NONE',  ( -2.229367062499996610, -6.145833331967740953, 3.861377020970582219 ) ) ;
#11191=CARTESIAN_POINT ( 'NONE',  ( -4.458734124999998549, 20.52083333469892423, 2.574251347313722516 ) ) ;
#11192=CARTESIAN_POINT ( 'NONE',  ( 2.229367062499998831, -45.89583333196774362, -3.861377020970580887 ) ) ;
#11193=CARTESIAN_POINT ( 'NONE',  ( 1.975475456537005874E-15, -105.7500000000000000, 5.000000000000000000 ) ) ;
#11201=CARTESIAN_POINT ( 'NONE',  ( 4.458734124999998549, -76.72916666530106511, -2.574251347313721627 ) ) ;
#11202=CARTESIAN_POINT ( 'NONE',  ( 2.229367062499998831, 28.10416666803225993, -3.861377020970580887 ) ) ;
#11205=LINE ( 'NONE', #54954, #35913 ) ;
#11206=DIRECTION ( 'NONE',  ( -0.000000000000000000, 1.000000000000000000, -0.000000000000000000 ) ) ;
#11208=CARTESIAN_POINT ( 'NONE',  ( 2.500000000000002220, -60.66666666666665719, 4.330127018922192761 ) ) ;
#11211=CARTESIAN_POINT ( 'NONE',  ( 3.044556291839386294E-14, 18.75000000000000355, -5.000000000000000000 ) ) ;
#11221=CARTESIAN_POINT ( 'NONE',  ( 2.500000000000002220, -59.54166666393546592, 4.330127018922192761 ) ) ;
#11223=ORIENTED_EDGE ( 'NONE', *, *, #9608, .T. ) ;
#11226=CARTESIAN_POINT ( 'NONE',  ( 2.229367062499998831, -45.89583333196774362, -3.861377020970580887 ) ) ;
#11227=CARTESIAN_POINT ( 'NONE',  ( 2.499999999999998668, -23.33333333333333215, -4.330127018922193649 ) ) ;
#11236=CARTESIAN_POINT ( 'NONE',  ( 4.458734124999999437, -97.06249999863440792, -5.460374474430324690E-16 ) ) ;
#11237=CARTESIAN_POINT ( 'NONE',  ( -2.499999999999996447, -106.8333333333333428, 4.330127018922195425 ) ) ;
#11239=CARTESIAN_POINT ( 'NONE',  ( -4.999999999999998224, 14.20833333606451987, 2.886751345948131764 ) ) ;
#11245=CARTESIAN_POINT ( 'NONE',  ( -4.458734124999999437, -1.312499998634406140, 0.000000000000000000 ) ) ;
#11247=CARTESIAN_POINT ( 'NONE',  ( -4.458734124999999437, -15.56249999863440436, 0.000000000000000000 ) ) ;
#11252=CARTESIAN_POINT ( 'NONE',  ( 4.458734124999998549, 17.02083333469892779, -2.574251347313721627 ) ) ;
#11253=ORIENTED_EDGE ( 'NONE', *, *, #33502, .T. ) ;
#11255=CARTESIAN_POINT ( 'NONE',  ( -1.339745962155613812, -13.20534180126147916, -5.000000000000000000 ) ) ;
#11256=CARTESIAN_POINT ( 'NONE',  ( -2.229367062500000163, -18.47916666530106866, -3.861377020970580443 ) ) ;
#11260=CARTESIAN_POINT ( 'NONE',  ( 5.000000000000000000, -49.37499999726880873, -6.123233995736766282E-16 ) ) ;
#11262=CARTESIAN_POINT ( 'NONE',  ( -4.458734124999997661, 8.770833334698927786, 2.574251347313722516 ) ) ;
#11263=CARTESIAN_POINT ( 'NONE',  ( 1.243387493232115550E-13, -9.124999997268817609, -5.000000000000000000 ) ) ;
#11264=CARTESIAN_POINT ( 'NONE',  ( 0.000000000000000000, -120.0000000000000000, 5.000000000000000000 ) ) ;
#11266=CARTESIAN_POINT ( 'NONE',  ( 2.229367062499998831, -65.64583333196773651, -3.861377020970580887 ) ) ;
#11268=CARTESIAN_POINT ( 'NONE',  ( -2.499999999999996447, 3.166666666666664742, 4.330127018922195425 ) ) ;
#11271=CARTESIAN_POINT ( 'NONE',  ( -3.152548672688508926E-16, -60.56249999863440792, -5.148502694627439702 ) ) ;
#11272=CARTESIAN_POINT ( 'NONE',  ( 2.499999999999998668, -96.20833333060213022, -4.330127018922193649 ) ) ;
#11273=CARTESIAN_POINT ( 'NONE',  ( -4.330127018922101279, 30.00000000000000000, 7.500000000000002665 ) ) ;
#11274=CARTESIAN_POINT ( 'NONE',  ( -4.999999999999998224, -69.91666666666667140, 2.886751345948131764 ) ) ;
#11275=CARTESIAN_POINT ( 'NONE',  ( 1.975475456537005874E-15, -56.75000000000000000, 5.000000000000000000 ) ) ;
#11278=CARTESIAN_POINT ( 'NONE',  ( -3.535250795749689387E-16, -41.25000000000000000, -5.773502691896257311 ) ) ;
#11280=CARTESIAN_POINT ( 'NONE',  ( -5.000000000000000000, -107.9999999999999858, 0.000000000000000000 ) ) ;
#11281=ORIENTED_EDGE ( 'NONE', *, *, #61532, .F. ) ;
#11282=CARTESIAN_POINT ( 'NONE',  ( 9.457646018065525792E-16, -107.0624999986343937, 5.148502694627439702 ) ) ;
#11283=CARTESIAN_POINT ( 'NONE',  ( -2.229367062500000163, -3.729166665301070438, -3.861377020970580443 ) ) ;
#11290=ORIENTED_EDGE ( 'NONE', *, *, #5800, .T. ) ;
#11291=CARTESIAN_POINT ( 'NONE',  ( 2.499999999999998668, -6.333333333333336590, -4.330127018922193649 ) ) ;
#11294=CARTESIAN_POINT ( 'NONE',  ( 2.499999999999998668, -101.3333333333333286, -4.330127018922193649 ) ) ;
#11296=CARTESIAN_POINT ( 'NONE',  ( -4.458734124999998549, -29.47916666530106866, 2.574251347313722516 ) ) ;
#11297=DIRECTION ( 'NONE',  ( -0.000000000000000000, 1.000000000000000000, -0.000000000000000000 ) ) ;
#11306=ORIENTED_EDGE ( 'NONE', *, *, #48449, .T. ) ;
#11307=CARTESIAN_POINT ( 'NONE',  ( -2.229367062500000163, -78.72916666530106511, -3.861377020970580443 ) ) ;
#11308=CYLINDRICAL_SURFACE ( 'NONE', #30710, 5.000000000000000000 ) ;
#11311=CARTESIAN_POINT ( 'NONE',  ( -1.339745962155613812, 7.794658198738521726, -5.000000000000000000 ) ) ;
#11313=EDGE_CURVE ( 'NONE', #52441, #1445, #47729, .T. ) ;
#11314=CARTESIAN_POINT ( 'NONE',  ( 4.458734124999998549, -4.979166665301072214, -2.574251347313721627 ) ) ;
#11315=VERTEX_POINT ( 'NONE', #1023 ) ;
#11317=CARTESIAN_POINT ( 'NONE',  ( 0.000000000000000000, -120.0000000000000000, 0.000000000000000000 ) ) ;
#11319=CARTESIAN_POINT ( 'NONE',  ( 5.000000000000000888, -91.58333333333334281, 2.886751345948126879 ) ) ;
#11321=AXIS2_PLACEMENT_3D ( 'NONE', #62064, #26696, #17977 ) ;
#11323=( BOUNDED_CURVE ( )  B_SPLINE_CURVE ( 2, ( #12746, #53483, #43817, #58630, #18206 ),
 .UNSPECIFIED., .F., .F. ) 
 B_SPLINE_CURVE_WITH_KNOTS ( ( 3, 2, 3 ),
 ( 0.000000000000000000, 0.001190476190476190584, 0.001785714285714286092 ),
 .UNSPECIFIED. ) 
 CURVE ( )  GEOMETRIC_REPRESENTATION_ITEM ( )  RATIONAL_B_SPLINE_CURVE ( ( 1.000000000000000000, 0.8660254037844387076, 1.000000000000000000, 0.9330127018922192983, 0.9330127018922194093 ) ) 
 REPRESENTATION_ITEM ( '' )  );
#11325=VERTEX_POINT ( 'NONE', #24804 ) ;
#11326=CARTESIAN_POINT ( 'NONE',  ( -4.458734124999999437, -79.39583333196773651, -2.574251347313719407 ) ) ;
#11327=CARTESIAN_POINT ( 'NONE',  ( 5.000000000000000000, -75.50000000000000000, -6.123233995736766282E-16 ) ) ;
#11328=CARTESIAN_POINT ( 'NONE',  ( 2.229367062500001939, -1.979166665301068662, 3.861377020970579999 ) ) ;
#11332=CARTESIAN_POINT ( 'NONE',  ( -4.458734124999999437, -69.64583333196773651, -2.574251347313719407 ) ) ;
#11333=CARTESIAN_POINT ( 'NONE',  ( -3.535250795749689387E-16, -31.12499999726881228, -5.773502691896257311 ) ) ;
#11334=ADVANCED_FACE ( 'NONE', ( #59219 ), #20628, .T. ) ;
#11335=CARTESIAN_POINT ( 'NONE',  ( -5.000000000000000000, -15.00000000000000000, 0.000000000000000000 ) ) ;
#11336=CARTESIAN_POINT ( 'NONE',  ( -2.229367062499996610, 28.85416666803226349, 3.861377020970582219 ) ) ;
#11337=CARTESIAN_POINT ( 'NONE',  ( 5.000000000000000888, -104.5833333333333286, 2.886751345948126879 ) ) ;
#11339=CARTESIAN_POINT ( 'NONE',  ( -4.458734124999999437, -53.39583333196773651, -2.574251347313719407 ) ) ;
#11340=CARTESIAN_POINT ( 'NONE',  ( 9.457646018065525792E-16, -34.31249999863440792, 5.148502694627439702 ) ) ;
#11343=CARTESIAN_POINT ( 'NONE',  ( 2.499999999999998668, 20.66666666666666785, -4.330127018922193649 ) ) ;
#11345=CARTESIAN_POINT ( 'NONE',  ( 5.000000000000000000, -26.29166666393547658, -2.886751345948130876 ) ) ;
#11346=CARTESIAN_POINT ( 'NONE',  ( -3.152548672688508926E-16, -41.56249999863439371, -5.148502694627439702 ) ) ;
#11347=CARTESIAN_POINT ( 'NONE',  ( 5.000000000000000000, -77.29166666393545881, -2.886751345948129988 ) ) ;
#11352=CARTESIAN_POINT ( 'NONE',  ( -3.152548672688508926E-16, -78.81249999863442213, -5.148502694627439702 ) ) ;
#11354=CARTESIAN_POINT ( 'NONE',  ( -2.499999999999996447, -24.83333333333333215, 4.330127018922195425 ) ) ;
#11359=CARTESIAN_POINT ( 'NONE',  ( 5.000000000000000000, 18.62500000273118772, -6.123233995736766282E-16 ) ) ;
#11369=CARTESIAN_POINT ( 'NONE',  ( 5.000000000000000888, -11.45833333060214976, 2.886751345948126879 ) ) ;
#11371=CARTESIAN_POINT ( 'NONE',  ( 2.500000000000002220, -56.54166666393548013, 4.330127018922192761 ) ) ;
#11374=CARTESIAN_POINT ( 'NONE',  ( -3.152548672688508926E-16, -14.81249999863440436, -5.148502694627439702 ) ) ;
#11384=ORIENTED_EDGE ( 'NONE', *, *, #37762, .F. ) ;
#11386=LINE ( 'NONE', #21369, #16261 ) ;
#11391=CARTESIAN_POINT ( 'NONE',  ( -6.972266317189433020E-16, 15.75000000000000000, -5.000000000000000000 ) ) ;
#11393=ADVANCED_FACE ( 'NONE', ( #13420 ), #55361, .T. ) ;
#11396=ADVANCED_FACE ( 'NONE', ( #55678 ), #52351, .T. ) ;
#11398=CARTESIAN_POINT ( 'NONE',  ( -4.458734124999998549, 11.77083333469892601, 2.574251347313722516 ) ) ;
#11401=CARTESIAN_POINT ( 'NONE',  ( 4.330127018922258486, 30.00000000000000000, 7.499999999999910294 ) ) ;
#11403=VERTEX_POINT ( 'NONE', #60186 ) ;
#11404=CARTESIAN_POINT ( 'NONE',  ( 2.229367062500001939, -65.97916666530106511, 3.861377020970579999 ) ) ;
#11405=CARTESIAN_POINT ( 'NONE',  ( 9.457646018065525792E-16, 12.93750000136559386, 5.148502694627439702 ) ) ;
#11409=CARTESIAN_POINT ( 'NONE',  ( 4.458734124999999437, -53.06249999863440792, -5.460374474430324690E-16 ) ) ;
#11410=CARTESIAN_POINT ( 'NONE',  ( -4.999999999999999112, -12.79166666393547835, 2.886751345948131764 ) ) ;
#11414=CARTESIAN_POINT ( 'NONE',  ( 8.660254037844342889, 30.00000000000000000, 0.000000000000000000 ) ) ;
#11415=CARTESIAN_POINT ( 'NONE',  ( 5.000000000000000000, -104.2916666639354730, -2.886751345948130876 ) ) ;
#11416=CARTESIAN_POINT ( 'NONE',  ( 2.229367062499998831, -14.89583333196773474, -3.861377020970580887 ) ) ;
#11419=CARTESIAN_POINT ( 'NONE',  ( 2.229367062499998831, -103.6458333319677365, -3.861377020970580887 ) ) ;
#11421=ORIENTED_EDGE ( 'NONE', *, *, #49870, .T. ) ;
#11422=CARTESIAN_POINT ( 'NONE',  ( -4.458734124999999437, -101.6458333319677365, -2.574251347313719407 ) ) ;
#11424=CARTESIAN_POINT ( 'NONE',  ( 4.458734124999999437, -28.81249999863440436, -5.460374474430324690E-16 ) ) ;
#11425=CARTESIAN_POINT ( 'NONE',  ( 5.000000000000000000, -61.29166666393548013, -2.886751345948129988 ) ) ;
#11427=( BOUNDED_CURVE ( )  B_SPLINE_CURVE ( 2, ( #23380, #9506, #47800, #52950, #8887, #48432, #23691, #43290, #28812 ),
 .UNSPECIFIED., .F., .F. ) 
 B_SPLINE_CURVE_WITH_KNOTS ( ( 3, 2, 2, 2, 3 ),
 ( 0.5875000000000000222, 0.5880952380952381153, 0.5892857142857143016, 0.5904761904761904878, 0.5910714285714285809 ),
 .UNSPECIFIED. ) 
 CURVE ( )  GEOMETRIC_REPRESENTATION_ITEM ( )  RATIONAL_B_SPLINE_CURVE ( ( 0.9330127018922194093, 0.9330127018922194093, 1.000000000000000000, 0.8660254037844387076, 1.000000000000000000, 0.8660254037844387076, 1.000000000000000000, 0.9330127018922194093, 0.9330127018922194093 ) ) 
 REPRESENTATION_ITEM ( '' )  );
#11429=CARTESIAN_POINT ( 'NONE',  ( 4.458734125000000326, -23.89583333196773651, 2.574251347313718519 ) ) ;
#11430=CARTESIAN_POINT ( 'NONE',  ( -2.229367062500000163, -61.72916666530106511, -3.861377020970580443 ) ) ;
#11433=CARTESIAN_POINT ( 'NONE',  ( -6.031010364368858512E-14, 4.249999999999995559, 5.000000000000000000 ) ) ;
#11435=CARTESIAN_POINT ( 'NONE',  ( -5.000000000000000000, -13.99999999999999822, 0.000000000000000000 ) ) ;
#11439=CARTESIAN_POINT ( 'NONE',  ( 1.975475456537005874E-15, -12.62499999726881050, 5.000000000000000000 ) ) ;
#11445=CARTESIAN_POINT ( 'NONE',  ( -1.339745962155614700, 26.20534180126147561, 4.999999999999999112 ) ) ;
#11447=CARTESIAN_POINT ( 'NONE',  ( -4.999999999999999112, -81.91666666666665719, 2.886751345948131764 ) ) ;
#11451=ORIENTED_EDGE ( 'NONE', *, *, #7605, .T. ) ;
#11452=DIRECTION ( 'NONE',  ( -0.000000000000000000, 1.000000000000000000, -0.000000000000000000 ) ) ;
#11456=ORIENTED_EDGE ( 'NONE', *, *, #27532, .T. ) ;
#11463=ORIENTED_EDGE ( 'NONE', *, *, #2093, .F. ) ;
#11467=CARTESIAN_POINT ( 'NONE',  ( -5.000000000000000000, -84.08333333333332860, -2.886751345948128211 ) ) ;
#11469=EDGE_CURVE ( 'NONE', #19054, #24216, #8286, .T. ) ;
#11470=EDGE_CURVE ( 'NONE', #23690, #37137, #39454, .T. ) ;
#11471=CARTESIAN_POINT ( 'NONE',  ( -3.152548672688508926E-16, -79.56249999863440792, -5.148502694627439702 ) ) ;
#11472=CARTESIAN_POINT ( 'NONE',  ( -2.229367062500000163, -109.7291666653010651, -3.861377020970580443 ) ) ;
#11474=EDGE_CURVE ( 'NONE', #23099, #45276, #30440, .T. ) ;
#11475=EDGE_LOOP ( 'NONE', ( #22229, #12396, #41921, #56033 ) ) ;
#11480=CARTESIAN_POINT ( 'NONE',  ( -4.458734124999999437, -42.39583333196773651, -2.574251347313719407 ) ) ;
#11484=CARTESIAN_POINT ( 'NONE',  ( -2.229367062500000163, -50.47916666530107221, -3.861377020970580443 ) ) ;
#11488=CARTESIAN_POINT ( 'NONE',  ( 2.229367062500001939, -15.97916666530107399, 3.861377020970579999 ) ) ;
#11489=EDGE_CURVE ( 'NONE', #2897, #19298, #63258, .T. ) ;
#11490=CARTESIAN_POINT ( 'NONE',  ( 2.499999999999998668, -102.3333333333333286, -4.330127018922193649 ) ) ;
#11492=CARTESIAN_POINT ( 'NONE',  ( -3.152548672688508926E-16, -37.81249999863440792, -5.148502694627439702 ) ) ;
#11493=CARTESIAN_POINT ( 'NONE',  ( -2.499999999999996447, 1.291666669397853351, 4.330127018922195425 ) ) ;
#11494=CARTESIAN_POINT ( 'NONE',  ( -4.999999999999998224, -6.791666663935481019, 2.886751345948131764 ) ) ;
#11497=EDGE_CURVE ( 'NONE', #45023, #23818, #8301, .T. ) ;
#11498=CARTESIAN_POINT ( 'NONE',  ( 1.975475456537005874E-15, -71.75000000000000000, 5.000000000000000000 ) ) ;
#11499=CARTESIAN_POINT ( 'NONE',  ( -6.972266317189433020E-16, 19.87500000273118417, -5.000000000000000000 ) ) ;
#11500=CARTESIAN_POINT ( 'NONE',  ( 2.229367062500001939, -1.229166665301071548, 3.861377020970579999 ) ) ;
#11502=CARTESIAN_POINT ( 'NONE',  ( 5.000000000000000000, 16.70833333606451987, -2.886751345948130876 ) ) ;
#11503=ADVANCED_FACE ( 'NONE', ( #63577 ), #28832, .T. ) ;
#11504=CARTESIAN_POINT ( 'NONE',  ( 4.458734124999998549, -86.72916666530107932, -2.574251347313721627 ) ) ;
#11506=CARTESIAN_POINT ( 'NONE',  ( 4.458734124999998549, -86.97916666530106511, -2.574251347313721627 ) ) ;
#11508=DIRECTION ( 'NONE',  ( -0.000000000000000000, 1.000000000000000000, -0.000000000000000000 ) ) ;
#11510=CARTESIAN_POINT ( 'NONE',  ( -3.152548672688508926E-16, -5.562499998634400811, -5.148502694627439702 ) ) ;
#11511=CARTESIAN_POINT ( 'NONE',  ( -2.229367062499996610, 16.60416666803225638, 3.861377020970582219 ) ) ;
#11512=CARTESIAN_POINT ( 'NONE',  ( 9.457646018065525792E-16, -49.31249999863440792, 5.148502694627439702 ) ) ;
#11513=CARTESIAN_POINT ( 'NONE',  ( -5.000000000000000000, 17.12500000273118417, 0.000000000000000000 ) ) ;
#11520=CARTESIAN_POINT ( 'NONE',  ( 2.229367062499998831, -73.64583333196773651, -3.861377020970580887 ) ) ;
#11521=CARTESIAN_POINT ( 'NONE',  ( 4.458734124999999437, 27.93750000136559208, -5.460374474430324690E-16 ) ) ;
#11523=CARTESIAN_POINT ( 'NONE',  ( 1.975475456537005874E-15, -57.62499999726880873, 5.000000000000000000 ) ) ;
#11526=CARTESIAN_POINT ( 'NONE',  ( -2.499999999999996447, -65.83333333333332860, 4.330127018922195425 ) ) ;
#11527=CARTESIAN_POINT ( 'NONE',  ( -2.499999999999996447, -31.70833333060214798, 4.330127018922195425 ) ) ;
#11529=ORIENTED_EDGE ( 'NONE', *, *, #40068, .T. ) ;
#11530=CARTESIAN_POINT ( 'NONE',  ( -1.339745962155610925, -56.79465819873851729, 5.000000000000000000 ) ) ;
#11545=CARTESIAN_POINT ( 'NONE',  ( -2.229367062500000163, -44.72916666530106511, -3.861377020970580443 ) ) ;
#11549=FACE_OUTER_BOUND ( 'NONE', #12029, .T. ) ;
#11553=DIRECTION ( 'NONE',  ( -0.000000000000000000, 1.000000000000000000, -0.000000000000000000 ) ) ;
#11555=CARTESIAN_POINT ( 'NONE',  ( -4.458734124999998549, -93.47916666530106511, 2.574251347313722516 ) ) ;
#11556=CARTESIAN_POINT ( 'NONE',  ( -4.999999999999998224, -106.9166666666666572, 2.886751345948131764 ) ) ;
#11557=VERTEX_POINT ( 'NONE', #14666 ) ;
#11561=LINE ( 'NONE', #55647, #57918 ) ;
#11562=ORIENTED_EDGE ( 'NONE', *, *, #35751, .F. ) ;
#11563=CARTESIAN_POINT ( 'NONE',  ( -2.229367062499996610, -0.1458333319677394824, 3.861377020970582219 ) ) ;
#11564=CARTESIAN_POINT ( 'NONE',  ( 5.000000000000000888, 6.416666666666667851, 2.886751345948126879 ) ) ;
#11565=CARTESIAN_POINT ( 'NONE',  ( 4.458734125000001214, -21.14583333196774362, 2.574251347313718519 ) ) ;
#11566=CARTESIAN_POINT ( 'NONE',  ( 1.339745962155612702, -72.29465819873850307, -5.000000000000000000 ) ) ;
#11570=CARTESIAN_POINT ( 'NONE',  ( -4.458734124999997661, 17.52083333469892779, 2.574251347313722516 ) ) ;
#11572=CARTESIAN_POINT ( 'NONE',  ( -1.339745962155613812, -14.08034179853029144, -5.000000000000000000 ) ) ;
#11573=CARTESIAN_POINT ( 'NONE',  ( -1.339745962155610925, -12.79465819873851906, 5.000000000000000000 ) ) ;
#11574=CARTESIAN_POINT ( 'NONE',  ( 5.000000000000000000, -86.41666666666667140, -2.886751345948129988 ) ) ;
#11575=CARTESIAN_POINT ( 'NONE',  ( -4.458734124999999437, -18.39583333196774007, -2.574251347313719407 ) ) ;
#11580=CARTESIAN_POINT ( 'NONE',  ( -3.535250795749689387E-16, -44.12499999726880873, -5.773502691896257311 ) ) ;
#11581=CARTESIAN_POINT ( 'NONE',  ( 0.000000000000000000, -120.0000000000000000, 0.000000000000000000 ) ) ;
#11582=CARTESIAN_POINT ( 'NONE',  ( 2.229367062499998831, 7.354166668032259935, -3.861377020970580887 ) ) ;
#11584=FACE_OUTER_BOUND ( 'NONE', #24117, .T. ) ;
#11586=CARTESIAN_POINT ( 'NONE',  ( 4.458734125000001214, -68.89583333196773651, 2.574251347313718519 ) ) ;
#11588=CARTESIAN_POINT ( 'NONE',  ( -3.535250795749689387E-16, -1.250000000000001110, -5.773502691896257311 ) ) ;
#11591=CARTESIAN_POINT ( 'NONE',  ( -4.458734124999999437, -56.39583333196773651, -2.574251347313719407 ) ) ;
#11592=CARTESIAN_POINT ( 'NONE',  ( -2.499999999999996447, -96.70833333060213022, 4.330127018922195425 ) ) ;
#11595=CARTESIAN_POINT ( 'NONE',  ( -5.000000000000000000, -90.95833333060213022, -2.886751345948128211 ) ) ;
#11596=CARTESIAN_POINT ( 'NONE',  ( 1.060575238724906964E-15, -48.75000000000000000, 5.773502691896257311 ) ) ;
#11597=CARTESIAN_POINT ( 'NONE',  ( 5.000000000000000000, -13.41666666666666785, -2.886751345948130876 ) ) ;
#11598=CARTESIAN_POINT ( 'NONE',  ( 1.339745962155615144, -17.58034179853029499, 4.999999999999999112 ) ) ;
#11599=VERTEX_POINT ( 'NONE', #24325 ) ;
#11600=CARTESIAN_POINT ( 'NONE',  ( -2.229367062499996610, -108.1458333319677365, 3.861377020970582219 ) ) ;
#11601=CARTESIAN_POINT ( 'NONE',  ( 4.458734124999999437, -0.06249999863440491854, -5.460374474430324690E-16 ) ) ;
#11602=CARTESIAN_POINT ( 'NONE',  ( -1.339745962155613812, -97.08034179853028434, -5.000000000000000000 ) ) ;
#11605=( BOUNDED_CURVE ( )  B_SPLINE_CURVE ( 2, ( #16719, #27632, #45984, #31827, #36020, #32134, #46946, #40832, #7076 ),
 .UNSPECIFIED., .F., .F. ) 
 B_SPLINE_CURVE_WITH_KNOTS ( ( 3, 2, 2, 2, 3 ),
 ( 0.7160714285714285809, 0.7166666666666666741, 0.7178571428571428603, 0.7190476190476190466, 0.7196428571428571397 ),
 .UNSPECIFIED. ) 
 CURVE ( )  GEOMETRIC_REPRESENTATION_ITEM ( )  RATIONAL_B_SPLINE_CURVE ( ( 0.9330127018922194093, 0.9330127018922194093, 1.000000000000000000, 0.8660254037844387076, 1.000000000000000000, 0.8660254037844387076, 1.000000000000000000, 0.9330127018922194093, 0.9330127018922194093 ) ) 
 REPRESENTATION_ITEM ( '' )  );
#11606=DIRECTION ( 'NONE',  ( 0.000000000000000000, -0.000000000000000000, 1.000000000000000000 ) ) ;
#11609=ORIENTED_EDGE ( 'NONE', *, *, #17395, .F. ) ;
#11613=CARTESIAN_POINT ( 'NONE',  ( -1.339745962155606929, 24.79465819873852439, -5.000000000000004441 ) ) ;
#11615=CARTESIAN_POINT ( 'NONE',  ( 2.229367062499998831, -27.89583333196774007, -3.861377020970580887 ) ) ;
#11622=CARTESIAN_POINT ( 'NONE',  ( -5.000000000000000000, -93.87499999726881583, 0.000000000000000000 ) ) ;
#11624=CARTESIAN_POINT ( 'NONE',  ( 2.229367062499998831, -75.89583333196773651, -3.861377020970580887 ) ) ;
#11628=CARTESIAN_POINT ( 'NONE',  ( 0.000000000000000000, -120.0000000000000000, 5.000000000000000000 ) ) ;
#11630=CARTESIAN_POINT ( 'NONE',  ( 4.458734124999999437, -11.06249999863440792, -5.460374474430324690E-16 ) ) ;
#11633=CARTESIAN_POINT ( 'NONE',  ( -1.339745962155610925, -92.66965819600731891, 5.000000000000000000 ) ) ;
#11634=EDGE_LOOP ( 'NONE', ( #41044, #6126, #29481, #54802 ) ) ;
#11635=CARTESIAN_POINT ( 'NONE',  ( 4.458734125000001214, -7.145833331967734736, 2.574251347313718519 ) ) ;
#11637=CARTESIAN_POINT ( 'NONE',  ( -1.339745962155610925, -11.66965819600733667, 5.000000000000000000 ) ) ;
#11639=CARTESIAN_POINT ( 'NONE',  ( -4.458734124999999437, 29.43750000136559208, 0.000000000000000000 ) ) ;
#11640=ORIENTED_EDGE ( 'NONE', *, *, #11474, .F. ) ;
#11641=CARTESIAN_POINT ( 'NONE',  ( 4.458734124999999437, -85.81249999863439371, -5.460374474430324690E-16 ) ) ;
#11642=CARTESIAN_POINT ( 'NONE',  ( 2.499999999999998668, -29.20833333060214798, -4.330127018922193649 ) ) ;
#11643=CARTESIAN_POINT ( 'NONE',  ( -2.229367062500000163, -1.479166665301071770, -3.861377020970580443 ) ) ;
#11645=CARTESIAN_POINT ( 'NONE',  ( 5.000000000000000000, -31.29166666393548368, -2.886751345948129988 ) ) ;
#11647=CARTESIAN_POINT ( 'NONE',  ( 9.457646018065525792E-16, 25.93750000136559564, 5.148502694627439702 ) ) ;
#11649=( BOUNDED_CURVE ( )  B_SPLINE_CURVE ( 2, ( #50122, #24409, #295, #63658, #19576, #24726, #1266, #20224, #58815 ),
 .UNSPECIFIED., .F., .F. ) 
 B_SPLINE_CURVE_WITH_KNOTS ( ( 3, 2, 2, 2, 3 ),
 ( 0.1410714285714285698, 0.1416666666666666630, 0.1428571428571428492, 0.1440476190476190355, 0.1446428571428571563 ),
 .UNSPECIFIED. ) 
 CURVE ( )  GEOMETRIC_REPRESENTATION_ITEM ( )  RATIONAL_B_SPLINE_CURVE ( ( 0.9330127018922194093, 0.9330127018922194093, 1.000000000000000000, 0.8660254037844387076, 1.000000000000000000, 0.8660254037844387076, 1.000000000000000000, 0.9330127018922178550, 0.9330127018922194093 ) ) 
 REPRESENTATION_ITEM ( '' )  );
#11651=CARTESIAN_POINT ( 'NONE',  ( 4.458734124999999437, -48.81249999863440792, -5.460374474430324690E-16 ) ) ;
#11652=CARTESIAN_POINT ( 'NONE',  ( 4.458734125000000326, -37.14583333196773651, 2.574251347313718519 ) ) ;
#11655=CARTESIAN_POINT ( 'NONE',  ( 5.000000000000000888, 13.41666666666666607, 2.886751345948126879 ) ) ;
#11657=CARTESIAN_POINT ( 'NONE',  ( -1.230605004983934782E-13, -26.62499999726881583, 5.000000000000000000 ) ) ;
#11658=CARTESIAN_POINT ( 'NONE',  ( -2.229367062500000163, -44.47916666530106511, -3.861377020970580443 ) ) ;
#11659=CARTESIAN_POINT ( 'NONE',  ( -5.000000000000000000, -77.87499999726881583, 0.000000000000000000 ) ) ;
#11661=VECTOR ( 'NONE', #52854, 1000.000000000000000 ) ;
#11662=CARTESIAN_POINT ( 'NONE',  ( 5.000000000000000000, -24.29166666393548368, -2.886751345948130876 ) ) ;
#11664=CARTESIAN_POINT ( 'NONE',  ( 2.229367062500001939, -86.22916666530107932, 3.861377020970579999 ) ) ;
#11667=CARTESIAN_POINT ( 'NONE',  ( 1.060575238724906964E-15, -29.74999999999999645, 5.773502691896257311 ) ) ;
#11669=ORIENTED_EDGE ( 'NONE', *, *, #46497, .F. ) ;
#11672=CARTESIAN_POINT ( 'NONE',  ( -2.229367062500000163, -91.47916666530106511, -3.861377020970580443 ) ) ;
#11673=CARTESIAN_POINT ( 'NONE',  ( -2.229367062499996610, 12.60416666803226171, 3.861377020970582219 ) ) ;
#11674=CARTESIAN_POINT ( 'NONE',  ( 1.060575238724906964E-15, 15.37500000273118417, 5.773502691896257311 ) ) ;
#11680=CARTESIAN_POINT ( 'NONE',  ( 1.975475456537005874E-15, 0.2500000000000001665, 5.000000000000000000 ) ) ;
#11681=CARTESIAN_POINT ( 'NONE',  ( -2.499999999999996447, -51.83333333333332860, 4.330127018922195425 ) ) ;
#11682=CARTESIAN_POINT ( 'NONE',  ( -5.000000000000000000, -109.9999999999999858, 0.000000000000000000 ) ) ;
#11683=CARTESIAN_POINT ( 'NONE',  ( 1.975475456537005874E-15, 2.249999999999999556, 5.000000000000000000 ) ) ;
#11684=CARTESIAN_POINT ( 'NONE',  ( -5.000000000000000000, -62.00000000000000000, 0.000000000000000000 ) ) ;
#11686=CARTESIAN_POINT ( 'NONE',  ( 6.123233995736766282E-16, -120.0000000000000000, -5.000000000000000000 ) ) ;
#11687=DIRECTION ( 'NONE',  ( -0.000000000000000000, 1.000000000000000000, -0.000000000000000000 ) ) ;
#11688=CARTESIAN_POINT ( 'NONE',  ( -4.458734124999999437, -16.56249999863440436, 0.000000000000000000 ) ) ;
#11699=CARTESIAN_POINT ( 'NONE',  ( -4.458734124999999437, -63.64583333196773651, -2.574251347313719407 ) ) ;
#11701=CARTESIAN_POINT ( 'NONE',  ( 5.000000000000000000, -58.50000000000000000, -6.123233995736766282E-16 ) ) ;
#11705=CARTESIAN_POINT ( 'NONE',  ( -5.000000000000000000, -7.874999997268813168, 0.000000000000000000 ) ) ;
#11709=ORIENTED_EDGE ( 'NONE', *, *, #12848, .F. ) ;
#11710=VECTOR ( 'NONE', #43361, 1000.000000000000000 ) ;
#11712=CARTESIAN_POINT ( 'NONE',  ( -2.229367062499996610, 7.854166668032260823, 3.861377020970582219 ) ) ;
#11715=CARTESIAN_POINT ( 'NONE',  ( 1.339745962155499015, -108.5803417985302843, 5.000000000000065725 ) ) ;
#11717=EDGE_LOOP ( 'NONE', ( #45483, #49505, #55539, #22066 ) ) ;
#11718=CARTESIAN_POINT ( 'NONE',  ( -4.458734124999999437, -70.31249999863439371, 0.000000000000000000 ) ) ;
#11719=DIRECTION ( 'NONE',  ( -0.000000000000000000, 1.000000000000000000, -0.000000000000000000 ) ) ;
#11720=CARTESIAN_POINT ( 'NONE',  ( -3.152548672688508926E-16, 10.43750000136559386, -5.148502694627439702 ) ) ;
#11721=CARTESIAN_POINT ( 'NONE',  ( 2.499999999999998668, 7.791666669397852019, -4.330127018922193649 ) ) ;
#11723=CARTESIAN_POINT ( 'NONE',  ( -3.152548672688508926E-16, -54.81249999863440081, -5.148502694627439702 ) ) ;
#11724=CARTESIAN_POINT ( 'NONE',  ( 5.000000000000000000, -12.29166666393547835, -2.886751345948129988 ) ) ;
#11727=CARTESIAN_POINT ( 'NONE',  ( -4.458734124999999437, -21.56249999863440436, 0.000000000000000000 ) ) ;
#11728=ORIENTED_EDGE ( 'NONE', *, *, #2774, .F. ) ;
#11730=CARTESIAN_POINT ( 'NONE',  ( -4.458734124999998549, -106.2291666653010793, 2.574251347313722516 ) ) ;
#11733=CARTESIAN_POINT ( 'NONE',  ( 2.229367062500001939, -104.2291666653010651, 3.861377020970579999 ) ) ;
#11734=CARTESIAN_POINT ( 'NONE',  ( 4.458734124999999437, -27.81249999863440081, -5.460374474430324690E-16 ) ) ;
#11735=CARTESIAN_POINT ( 'NONE',  ( -3.535250795749689387E-16, -61.12499999726880873, -5.773502691896257311 ) ) ;
#11738=CARTESIAN_POINT ( 'NONE',  ( -4.458734124999999437, -25.39583333196773651, -2.574251347313719407 ) ) ;
#11739=CARTESIAN_POINT ( 'NONE',  ( -4.458734124999999437, -62.56249999863440792, 0.000000000000000000 ) ) ;
#11742=CARTESIAN_POINT ( 'NONE',  ( 5.000000000000000000, -32.41666666666666430, -2.886751345948130876 ) ) ;
#11744=CARTESIAN_POINT ( 'NONE',  ( 5.000000000000000000, -12.49999999999999645, -6.123233995736766282E-16 ) ) ;
#11752=FACE_OUTER_BOUND ( 'NONE', #24204, .T. ) ;
#11753=AXIS2_PLACEMENT_3D ( 'NONE', #59966, #26492, #21035 ) ;
#11756=CARTESIAN_POINT ( 'NONE',  ( 5.000000000000000000, -95.29166666393547303, -2.886751345948130876 ) ) ;
#11763=CARTESIAN_POINT ( 'NONE',  ( -6.972266317189433020E-16, -51.25000000000000000, -5.000000000000000000 ) ) ;
#11768=EDGE_LOOP ( 'NONE', ( #13261, #22399, #49158, #46990 ) ) ;
#11770=EDGE_CURVE ( 'NONE', #33683, #14691, #46051, .T. ) ;
#11774=CARTESIAN_POINT ( 'NONE',  ( 1.339745962155615144, -55.70534180126148271, 4.999999999999999112 ) ) ;
#11778=CARTESIAN_POINT ( 'NONE',  ( 1.975475456537005874E-15, 21.24999999999999289, 5.000000000000000000 ) ) ;
#11781=CARTESIAN_POINT ( 'NONE',  ( -3.152548672688508926E-16, -75.56249999863439371, -5.148502694627439702 ) ) ;
#11782=CARTESIAN_POINT ( 'NONE',  ( 2.229367062499998831, 28.35416666803225993, -3.861377020970580887 ) ) ;
#11783=CARTESIAN_POINT ( 'NONE',  ( 6.123233995736766282E-16, -120.0000000000000000, -5.000000000000000000 ) ) ;
#11784=ORIENTED_EDGE ( 'NONE', *, *, #21385, .F. ) ;
#11785=LINE ( 'NONE', #40739, #52077 ) ;
#11792=CARTESIAN_POINT ( 'NONE',  ( 4.458734124999998549, -47.72916666530106511, -2.574251347313721627 ) ) ;
#11794=CARTESIAN_POINT ( 'NONE',  ( 9.457646018065525792E-16, 27.93750000136559208, 5.148502694627439702 ) ) ;
#11795=EDGE_CURVE ( 'NONE', #6430, #42800, #29136, .T. ) ;
#11796=CARTESIAN_POINT ( 'NONE',  ( -2.500000000000000444, -105.1666666666666572, -4.330127018922193649 ) ) ;
#11800=CARTESIAN_POINT ( 'NONE',  ( -2.229367062499996610, -37.39583333196773651, 3.861377020970582219 ) ) ;
#11801=CARTESIAN_POINT ( 'NONE',  ( 2.499999999999998668, -0.2083333306021478704, -4.330127018922193649 ) ) ;
#11805=CARTESIAN_POINT ( 'NONE',  ( -4.458734124999997661, -95.22916666530106511, 2.574251347313722516 ) ) ;
#11806=CARTESIAN_POINT ( 'NONE',  ( -3.152548672688508926E-16, 0.1875000013655953035, -5.148502694627439702 ) ) ;
#11808=CARTESIAN_POINT ( 'NONE',  ( 0.000000000000000000, -120.0000000000000000, 5.000000000000000000 ) ) ;
#11810=CARTESIAN_POINT ( 'NONE',  ( -3.152548672688508926E-16, -85.56249999863439371, -5.148502694627439702 ) ) ;
#11811=CARTESIAN_POINT ( 'NONE',  ( 2.229367062499998831, -84.89583333196773651, -3.861377020970580887 ) ) ;
#11815=CARTESIAN_POINT ( 'NONE',  ( 2.229367062499998831, -5.645833331967740953, -3.861377020970580887 ) ) ;
#11816=CARTESIAN_POINT ( 'NONE',  ( -3.152548672688508926E-16, 16.18750000136559564, -5.148502694627439702 ) ) ;
#11817=CARTESIAN_POINT ( 'NONE',  ( 2.229367062500001939, -50.22916666530107221, 3.861377020970579999 ) ) ;
#11821=LINE ( 'NONE', #55277, #60706 ) ;
#11822=ORIENTED_EDGE ( 'NONE', *, *, #48201, .T. ) ;
#11825=CARTESIAN_POINT ( 'NONE',  ( -3.152548672688508926E-16, -75.56249999863439371, -5.148502694627439702 ) ) ;
#11826=CARTESIAN_POINT ( 'NONE',  ( -2.499999999999996447, -110.7083333306021444, 4.330127018922195425 ) ) ;
#11828=EDGE_CURVE ( 'NONE', #17309, #42628, #2120, .T. ) ;
#11829=EDGE_CURVE ( 'NONE', #12275, #10579, #8665, .T. ) ;
#11830=CARTESIAN_POINT ( 'NONE',  ( -2.499999999999996447, -93.83333333333332860, 4.330127018922195425 ) ) ;
#11833=CARTESIAN_POINT ( 'NONE',  ( 5.000000000000000000, -63.41666666666665719, -2.886751345948129988 ) ) ;
#11835=CARTESIAN_POINT ( 'NONE',  ( 5.000000000000000000, -36.37499999726881583, -6.123233995736766282E-16 ) ) ;
#11838=CARTESIAN_POINT ( 'NONE',  ( -1.339745962155613812, -57.20534180126148271, -5.000000000000000000 ) ) ;
#11844=ADVANCED_FACE ( 'NONE', ( #17635 ), #46907, .T. ) ;
#11847=VERTEX_POINT ( 'NONE', #13120 ) ;
#11848=CARTESIAN_POINT ( 'NONE',  ( 5.000000000000000000, -59.29166666393547303, -2.886751345948130876 ) ) ;
#11854=CARTESIAN_POINT ( 'NONE',  ( 2.229367062499998831, -44.89583333196774362, -3.861377020970580887 ) ) ;
#11855=CARTESIAN_POINT ( 'NONE',  ( -6.972266317189433020E-16, -68.24999999999998579, -5.000000000000000000 ) ) ;
#11857=EDGE_CURVE ( 'NONE', #57389, #51032, #43580, .T. ) ;
#11859=CARTESIAN_POINT ( 'NONE',  ( -5.000000000000000000, -81.95833333060213022, -2.886751345948128211 ) ) ;
#11863=CARTESIAN_POINT ( 'NONE',  ( 2.500000000000002220, 22.33333333333333215, 4.330127018922192761 ) ) ;
#11865=CARTESIAN_POINT ( 'NONE',  ( 4.458734124999998549, -95.97916666530107932, -2.574251347313721627 ) ) ;
#11867=VERTEX_POINT ( 'NONE', #3791 ) ;
#11868=DIRECTION ( 'NONE',  ( -0.000000000000000000, 1.000000000000000000, -0.000000000000000000 ) ) ;
#11872=CARTESIAN_POINT ( 'NONE',  ( 2.229367062500001939, 0.02083333469892964529, 3.861377020970579999 ) ) ;
#11873=CARTESIAN_POINT ( 'NONE',  ( -3.152548672688508926E-16, -97.81249999863439371, -5.148502694627439702 ) ) ;
#11875=CARTESIAN_POINT ( 'NONE',  ( -4.458734124999999437, -24.64583333196773651, -2.574251347313719407 ) ) ;
#11879=CARTESIAN_POINT ( 'NONE',  ( -6.972266317189433020E-16, -93.12499999726881583, -5.000000000000000000 ) ) ;
#11881=( BOUNDED_CURVE ( )  B_SPLINE_CURVE ( 2, ( #4320, #49875, #25439, #43853, #30579, #52898, #58034, #35101, #30252 ),
 .UNSPECIFIED., .F., .F. ) 
 B_SPLINE_CURVE_WITH_KNOTS ( ( 3, 2, 2, 2, 3 ),
 ( 0.3232142857142857317, 0.3238095238095238249, 0.3250000000000000111, 0.3261904761904761973, 0.3267857142857142905 ),
 .UNSPECIFIED. ) 
 CURVE ( )  GEOMETRIC_REPRESENTATION_ITEM ( )  RATIONAL_B_SPLINE_CURVE ( ( 0.9330127018922194093, 0.9330127018922194093, 1.000000000000000000, 0.8660254037844387076, 1.000000000000000000, 0.8660254037844387076, 1.000000000000000000, 0.9330127018922194093, 0.9330127018922194093 ) ) 
 REPRESENTATION_ITEM ( '' )  );
#11882=CARTESIAN_POINT ( 'NONE',  ( -4.458734124999997661, 14.52083333469892779, 2.574251347313722516 ) ) ;
#11884=CARTESIAN_POINT ( 'NONE',  ( -4.999999999999998224, -13.79166666393548191, 2.886751345948131764 ) ) ;
#11885=CARTESIAN_POINT ( 'NONE',  ( 1.339745962155612702, -66.16965819600733312, -5.000000000000000000 ) ) ;
#11886=CARTESIAN_POINT ( 'NONE',  ( -4.999999999999999112, -83.91666666666667140, 2.886751345948131764 ) ) ;
#11887=CARTESIAN_POINT ( 'NONE',  ( -4.458734124999999437, -19.39583333196774007, -2.574251347313719407 ) ) ;
#11892=CARTESIAN_POINT ( 'NONE',  ( -3.535250795749689387E-16, -48.12499999726880873, -5.773502691896257311 ) ) ;
#11893=CARTESIAN_POINT ( 'NONE',  ( 2.499999999999998668, -41.20833333060214443, -4.330127018922193649 ) ) ;
#11894=CARTESIAN_POINT ( 'NONE',  ( 4.458734124999998549, 10.27083333469892779, -2.574251347313721627 ) ) ;
#11895=FACE_OUTER_BOUND ( 'NONE', #21259, .T. ) ;
#11897=CYLINDRICAL_SURFACE ( 'NONE', #11985, 5.000000000000000000 ) ;
#11899=CARTESIAN_POINT ( 'NONE',  ( -4.458734124999999437, -65.39583333196773651, -2.574251347313719407 ) ) ;
#11902=CARTESIAN_POINT ( 'NONE',  ( -5.000000000000000000, 1.000000000000000888, 0.000000000000000000 ) ) ;
#11905=CARTESIAN_POINT ( 'NONE',  ( -4.458734124999998549, -60.22916666530106511, 2.574251347313722516 ) ) ;
#11906=CARTESIAN_POINT ( 'NONE',  ( -4.999999999999999112, -92.79166666393547303, 2.886751345948131764 ) ) ;
#11912=CARTESIAN_POINT ( 'NONE',  ( 5.000000000000000000, -50.50000000000000000, -6.123233995736766282E-16 ) ) ;
#11913=CARTESIAN_POINT ( 'NONE',  ( 1.975475456537005874E-15, -13.75000000000000000, 5.000000000000000000 ) ) ;
#11916=CARTESIAN_POINT ( 'NONE',  ( -4.458734124999999437, -108.3124999986343937, 0.000000000000000000 ) ) ;
#11917=CARTESIAN_POINT ( 'NONE',  ( 2.229367062499998831, -0.8958333319677401763, -3.861377020970580887 ) ) ;
#11925=ORIENTED_EDGE ( 'NONE', *, *, #50417, .T. ) ;
#11926=FACE_OUTER_BOUND ( 'NONE', #36238, .T. ) ;
#11930=CARTESIAN_POINT ( 'NONE',  ( 2.229367062500001939, -30.22916666530107221, 3.861377020970579999 ) ) ;
#11931=CARTESIAN_POINT ( 'NONE',  ( -1.339745962155613812, -87.20534180126148271, -5.000000000000000000 ) ) ;
#11938=VECTOR ( 'NONE', #32795, 1000.000000000000000 ) ;
#11942=ORIENTED_EDGE ( 'NONE', *, *, #39284, .T. ) ;
#11943=CARTESIAN_POINT ( 'NONE',  ( 2.229367062499998831, -78.89583333196773651, -3.861377020970580887 ) ) ;
#11944=CARTESIAN_POINT ( 'NONE',  ( 5.000000000000000000, 3.583333333333333925, -2.886751345948130876 ) ) ;
#11946=CARTESIAN_POINT ( 'NONE',  ( 0.000000000000000000, -120.0000000000000000, 5.000000000000000000 ) ) ;
#11947=DIRECTION ( 'NONE',  ( -0.000000000000000000, 1.000000000000000000, -0.000000000000000000 ) ) ;
#11949=CARTESIAN_POINT ( 'NONE',  ( 4.458734124999998549, -7.979166665301073991, -2.574251347313721627 ) ) ;
#11950=VERTEX_POINT ( 'NONE', #10183 ) ;
#11951=CARTESIAN_POINT ( 'NONE',  ( -6.972266317189433020E-16, -85.25000000000000000, -5.000000000000000000 ) ) ;
#11952=CARTESIAN_POINT ( 'NONE',  ( -4.999999999999998224, -92.79166666393545881, 2.886751345948131764 ) ) ;
#11954=CARTESIAN_POINT ( 'NONE',  ( -4.458734124999999437, -6.562499998634403475, 0.000000000000000000 ) ) ;
#11961=CARTESIAN_POINT ( 'NONE',  ( -4.458734124999999437, -85.31249999863439371, 0.000000000000000000 ) ) ;
#11962=CARTESIAN_POINT ( 'NONE',  ( 0.000000000000000000, -120.0000000000000000, 0.000000000000000000 ) ) ;
#11963=CARTESIAN_POINT ( 'NONE',  ( -2.229367062500000163, -2.479166665301069106, -3.861377020970580443 ) ) ;
#11964=FACE_OUTER_BOUND ( 'NONE', #58136, .T. ) ;
#11965=CARTESIAN_POINT ( 'NONE',  ( -3.535250795749689387E-16, -28.12499999726880873, -5.773502691896257311 ) ) ;
#11967=CARTESIAN_POINT ( 'NONE',  ( -2.229367062499996610, 22.85416666803225993, 3.861377020970582219 ) ) ;
#11970=CARTESIAN_POINT ( 'NONE',  ( 2.229367062499998831, -52.64583333196773651, -3.861377020970580887 ) ) ;
#11971=CARTESIAN_POINT ( 'NONE',  ( 4.458734125000000326, -39.14583333196773651, 2.574251347313718519 ) ) ;
#11974=CARTESIAN_POINT ( 'NONE',  ( 1.975475456537005874E-15, -97.62499999726880162, 5.000000000000000000 ) ) ;
#11975=CARTESIAN_POINT ( 'NONE',  ( -4.999999999999999112, 16.08333333333333215, 2.886751345948131764 ) ) ;
#11977=CARTESIAN_POINT ( 'NONE',  ( -2.916731409357579869E-14, 12.37500000273118594, 5.000000000000000888 ) ) ;
#11978=CARTESIAN_POINT ( 'NONE',  ( 4.458734124999999437, -41.81249999863440081, -5.460374474430324690E-16 ) ) ;
#11979=CARTESIAN_POINT ( 'NONE',  ( 1.060575238724906964E-15, -79.62499999726881583, 5.773502691896257311 ) ) ;
#11982=( BOUNDED_CURVE ( )  B_SPLINE_CURVE ( 2, ( #40891, #26749, #6500, #2627, #21923, #16776, #27370, #61802, #56024 ),
 .UNSPECIFIED., .F., .F. ) 
 B_SPLINE_CURVE_WITH_KNOTS ( ( 3, 2, 2, 2, 3 ),
 ( 0.7089285714285714635, 0.7095238095238095566, 0.7107142857142857428, 0.7119047619047619291, 0.7125000000000000222 ),
 .UNSPECIFIED. ) 
 CURVE ( )  GEOMETRIC_REPRESENTATION_ITEM ( )  RATIONAL_B_SPLINE_CURVE ( ( 0.9330127018922194093, 0.9330127018922194093, 1.000000000000000000, 0.8660254037844387076, 1.000000000000000000, 0.8660254037844387076, 1.000000000000000000, 0.9330127018922194093, 0.9330127018922194093 ) ) 
 REPRESENTATION_ITEM ( '' )  );
#11983=CARTESIAN_POINT ( 'NONE',  ( -6.972266317189433020E-16, -65.12499999726880162, -5.000000000000000000 ) ) ;
#11985=AXIS2_PLACEMENT_3D ( 'NONE', #56623, #27022, #42432 ) ;
#11986=CARTESIAN_POINT ( 'NONE',  ( -2.229367062500000163, -87.72916666530107932, -3.861377020970580443 ) ) ;
#11989=CARTESIAN_POINT ( 'NONE',  ( 2.499999999999998668, -33.33333333333332860, -4.330127018922193649 ) ) ;
#11991=ORIENTED_EDGE ( 'NONE', *, *, #36714, .T. ) ;
#11993=ORIENTED_EDGE ( 'NONE', *, *, #42855, .T. ) ;
#11994=CARTESIAN_POINT ( 'NONE',  ( 4.458734124999998549, -88.72916666530106511, -2.574251347313721627 ) ) ;
#11995=CARTESIAN_POINT ( 'NONE',  ( -4.458734124999999437, 14.43750000136559386, 0.000000000000000000 ) ) ;
#11996=CARTESIAN_POINT ( 'NONE',  ( 2.499999999999998668, 14.79166666939785202, -4.330127018922193649 ) ) ;
#11997=CARTESIAN_POINT ( 'NONE',  ( 0.000000000000000000, -120.0000000000000000, 5.000000000000000000 ) ) ;
#12001=CARTESIAN_POINT ( 'NONE',  ( -5.000000000000000000, -52.08333333333332860, -2.886751345948128211 ) ) ;
#12003=CARTESIAN_POINT ( 'NONE',  ( 5.000000000000000888, -1.583333333333332371, 2.886751345948126879 ) ) ;
#12004=CARTESIAN_POINT ( 'NONE',  ( -4.999999999999998224, 18.20833333606451632, 2.886751345948131764 ) ) ;
#12006=CARTESIAN_POINT ( 'NONE',  ( 2.499999999999998668, -96.33333333333332860, -4.330127018922193649 ) ) ;
#12008=CARTESIAN_POINT ( 'NONE',  ( 2.229367062500001939, -15.22916666530107399, 3.861377020970579999 ) ) ;
#12016=VERTEX_POINT ( 'NONE', #43631 ) ;
#12019=CARTESIAN_POINT ( 'NONE',  ( 4.458734124999999437, -60.06249999863440081, -5.460374474430324690E-16 ) ) ;
#12020=CARTESIAN_POINT ( 'NONE',  ( 1.975475456537005874E-15, -27.74999999999999645, 5.000000000000000000 ) ) ;
#12021=CARTESIAN_POINT ( 'NONE',  ( 1.339745962155670655, -8.294658198738522614, -4.999999999999966249 ) ) ;
#12027=LINE ( 'NONE', #55789, #26784 ) ;
#12029=EDGE_LOOP ( 'NONE', ( #36953, #53245, #6345, #5103 ) ) ;
#12032=CLOSED_SHELL ( 'NONE', ( #32837, #57750, #31074, #60679, #4782, #34619, #63659, #2411, #54418, #4459, #8442, #13444, #34621, #46501, #47286, #6254, #47306, #50514, #34269, #26004, #30266, #62534, #21598, #4657, #3897, #41679, #14524, #46195, #51220, #27459, #731, #43895, #53883, #39772, #40186, #41617, #50611, #29923, #1231, #31980, #44886, #21303, #17700, #4819, #50763, #918, #41418, #28610, #28746, #26673, #13821, #52818, #29171, #25208, #37781, #52724, #18099, #2359, #55957, #49118, #12289, #30926, #44660, #30633, #18033, #35809, #44361, #44058, #21218, #60160, #6607, #37504, #14429, #61029, #4787, #44983, #34280, #17391, #40967, #31618, #38981, #29451, #54988, #50796, #10588, #11396, #22083, #44423, #34785, #12144, #8996, #16062, #3185, #10689, #30687, #935, #52310, #9871, #21503, #5620, #24047, #7, #30609, #60877, #16662, #55047, #7582, #84, #51572, #39410, #49487, #39436, #42396, #11393, #27982, #31823, #48007, #110, #45169, #2273, #293, #62559, #21033, #45346, #12309, #35335, #24859, #49800, #1291, #8712, #55962, #32240, #59406, #16864, #48794, #38140, #903, #35381, #31545, #36240, #7422, #60139, #33440, #62385, #20955, #38218, #21963, #41410, #20414, #21298, #18596, #24324, #42569, #55515, #38992, #47739, #59778, #42472, #12535, #43266, #7454, #18441, #61320, #21302, #1622, #5230, #23092, #48365, #4328, #44079, #6976, #57486, #39813, #57021, #53378, #17521, #56595, #59795, #42056, #36913, #47993, #18951, #27604, #34733, #58094, #61831, #3589, #57813, #8397, #10306, #47499, #61695, #11844, #42083, #55929, #51577, #17470, #42132, #37607, #52028, #15512, #186, #33753, #41227, #7465, #60315, #57919, #55360, #32334, #58076, #15047, #55606, #22087, #58098, #32333, #36271, #2447, #62964, #18669, #49147, #1154, #37405, #49151, #55854, #35450, #8746, #32972, #50865, #38302, #38905, #46352, #47148, #462, #46510, #53357, #61662, #26436, #54167, #925, #37497, #29452, #44022, #32701, #33046, #59792, #28760, #8721, #47555, #4449, #49617, #43706, #37426, #52752, #15067, #59418, #21670, #40003, #46365, #28249, #23354, #29416, #61381, #8716, #37369, #14327, #53048, #57535, #7773, #2096, #11334, #17814, #3650, #53170, #29902, #62966, #26278, #38558, #31075, #11503, #34181, #17369, #59713, #60959, #44422, #50702, #1297, #52643, #27625, #8311, #55650, #20105, #45568, #32179, #60501, #3950, #53616, #52395, #26670, #51589, #33320 ) ) ;
#12033=CARTESIAN_POINT ( 'NONE',  ( -4.458734124999999437, 9.687500001365593860, 0.000000000000000000 ) ) ;
#12034=( BOUNDED_CURVE ( )  B_SPLINE_CURVE ( 2, ( #21971, #27970, #63032, #8985, #58507, #18640, #9609, #3853, #2362 ),
 .UNSPECIFIED., .F., .F. ) 
 B_SPLINE_CURVE_WITH_KNOTS ( ( 3, 2, 2, 2, 3 ),
 ( 0.6696428571428570953, 0.6702380952380951884, 0.6714285714285713746, 0.6726190476190476719, 0.6732142857142857650 ),
 .UNSPECIFIED. ) 
 CURVE ( )  GEOMETRIC_REPRESENTATION_ITEM ( )  RATIONAL_B_SPLINE_CURVE ( ( 0.9330127018922194093, 0.9330127018922194093, 1.000000000000000000, 0.8660254037844387076, 1.000000000000000000, 0.8660254037844387076, 1.000000000000000000, 0.9330127018922194093, 0.9330127018922194093 ) ) 
 REPRESENTATION_ITEM ( '' )  );
#12037=CARTESIAN_POINT ( 'NONE',  ( 5.000000000000000888, -108.4583333306021444, 2.886751345948126879 ) ) ;
#12039=ORIENTED_EDGE ( 'NONE', *, *, #49514, .T. ) ;
#12040=CARTESIAN_POINT ( 'NONE',  ( 2.229367062500001939, -70.97916666530107932, 3.861377020970579999 ) ) ;
#12041=CARTESIAN_POINT ( 'NONE',  ( -1.339745962155610925, -49.66965819600732601, 5.000000000000000000 ) ) ;
#12042=CARTESIAN_POINT ( 'NONE',  ( -4.458734124999998549, 14.77083333469892779, 2.574251347313722516 ) ) ;
#12044=CYLINDRICAL_SURFACE ( 'NONE', #61808, 5.000000000000000000 ) ;
#12045=DIRECTION ( 'NONE',  ( 0.000000000000000000, 0.000000000000000000, 1.000000000000000000 ) ) ;
#12046=CARTESIAN_POINT ( 'NONE',  ( -4.458734124999999437, -53.56249999863439371, 0.000000000000000000 ) ) ;
#12047=CARTESIAN_POINT ( 'NONE',  ( -5.000000000000000000, -14.87499999726881228, 0.000000000000000000 ) ) ;
#12048=CARTESIAN_POINT ( 'NONE',  ( 1.975475456537005874E-15, -18.74999999999999645, 5.000000000000000000 ) ) ;
#12050=CARTESIAN_POINT ( 'NONE',  ( -1.339745962155610925, -83.66965819600733312, 5.000000000000000000 ) ) ;
#12051=CARTESIAN_POINT ( 'NONE',  ( 2.229367062500001939, -23.22916666530107221, 3.861377020970579999 ) ) ;
#12052=VERTEX_POINT ( 'NONE', #15003 ) ;
#12053=CARTESIAN_POINT ( 'NONE',  ( -1.339745962155610925, -101.7946581987385315, 5.000000000000000000 ) ) ;
#12054=CARTESIAN_POINT ( 'NONE',  ( 2.229367062500001939, -106.9791666653010651, 3.861377020970579999 ) ) ;
#12056=EDGE_LOOP ( 'NONE', ( #47420, #41394, #29236, #43507 ) ) ;
#12057=CARTESIAN_POINT ( 'NONE',  ( 4.458734124999999437, -103.0624999986344079, -5.460374474430324690E-16 ) ) ;
#12058=CARTESIAN_POINT ( 'NONE',  ( 9.457646018065525792E-16, -27.06249999863440081, 5.148502694627439702 ) ) ;
#12059=CARTESIAN_POINT ( 'NONE',  ( 2.499999999999998668, -64.20833333060213022, -4.330127018922193649 ) ) ;
#12062=CARTESIAN_POINT ( 'NONE',  ( -4.458734124999997661, -25.22916666530106866, 2.574251347313722516 ) ) ;
#12063=CARTESIAN_POINT ( 'NONE',  ( -4.458734124999999437, -67.56249999863440792, 0.000000000000000000 ) ) ;
#12064=CARTESIAN_POINT ( 'NONE',  ( 4.330127018922154569, 45.00000000000000000, -7.499999999999971578 ) ) ;
#12068=CARTESIAN_POINT ( 'NONE',  ( -2.500000000000000444, -16.16666666666666785, -4.330127018922193649 ) ) ;
#12070=VERTEX_POINT ( 'NONE', #58121 ) ;
#12074=CARTESIAN_POINT ( 'NONE',  ( -2.499999999999996447, -2.708333330602146649, 4.330127018922195425 ) ) ;
#12075=CARTESIAN_POINT ( 'NONE',  ( 2.500000000000002220, -38.54166666393548013, 4.330127018922192761 ) ) ;
#12078=VECTOR ( 'NONE', #2449, 1000.000000000000000 ) ;
#12079=DIRECTION ( 'NONE',  ( -0.000000000000000000, 1.000000000000000000, -0.000000000000000000 ) ) ;
#12086=ORIENTED_EDGE ( 'NONE', *, *, #26702, .T. ) ;
#12088=ORIENTED_EDGE ( 'NONE', *, *, #27163, .T. ) ;
#12089=( BOUNDED_CURVE ( )  B_SPLINE_CURVE ( 2, ( #51622, #12688, #36496, #54930, #47415, #47103, #41948, #56126, #22982 ),
 .UNSPECIFIED., .F., .F. ) 
 B_SPLINE_CURVE_WITH_KNOTS ( ( 3, 2, 2, 2, 3 ),
 ( 0.5267857142857143016, 0.5273809523809523947, 0.5285714285714285809, 0.5297619047619047672, 0.5303571428571428603 ),
 .UNSPECIFIED. ) 
 CURVE ( )  GEOMETRIC_REPRESENTATION_ITEM ( )  RATIONAL_B_SPLINE_CURVE ( ( 0.9330127018922194093, 0.9330127018922194093, 1.000000000000000000, 0.8660254037844387076, 1.000000000000000000, 0.8660254037844387076, 1.000000000000000000, 0.9330127018922194093, 0.9330127018922194093 ) ) 
 REPRESENTATION_ITEM ( '' )  );
#12096=ORIENTED_EDGE ( 'NONE', *, *, #7288, .T. ) ;
#12104=CARTESIAN_POINT ( 'NONE',  ( 4.458734124999999437, -76.81249999863440792, -5.460374474430324690E-16 ) ) ;
#12105=CARTESIAN_POINT ( 'NONE',  ( 4.458734124999998549, 24.27083333469892779, -2.574251347313721627 ) ) ;
#12112=CARTESIAN_POINT ( 'NONE',  ( -6.972266317189433020E-16, -84.12499999726880162, -5.000000000000000000 ) ) ;
#12114=VECTOR ( 'NONE', #46785, 1000.000000000000000 ) ;
#12116=CARTESIAN_POINT ( 'NONE',  ( 2.229367062499998831, -53.64583333196773651, -3.861377020970580887 ) ) ;
#12118=CARTESIAN_POINT ( 'NONE',  ( 4.458734124999998549, 26.27083333469893134, -2.574251347313721627 ) ) ;
#12119=EDGE_CURVE ( 'NONE', #25261, #59413, #15235, .T. ) ;
#12120=AXIS2_PLACEMENT_3D ( 'NONE', #47818, #52659, #33043 ) ;
#12121=CARTESIAN_POINT ( 'NONE',  ( -3.535250795749689387E-16, -104.2500000000000142, -5.773502691896257311 ) ) ;
#12123=CARTESIAN_POINT ( 'NONE',  ( 2.229367062500001939, -38.22916666530107221, 3.861377020970579999 ) ) ;
#12124=CARTESIAN_POINT ( 'NONE',  ( 1.060575238724906964E-15, 2.375000002731185500, 5.773502691896257311 ) ) ;
#12128=CARTESIAN_POINT ( 'NONE',  ( -1.339745962155613812, 5.794658198738519950, -5.000000000000000000 ) ) ;
#12129=CARTESIAN_POINT ( 'NONE',  ( 9.457646018065525792E-16, -103.0624999986343937, 5.148502694627439702 ) ) ;
#12130=CARTESIAN_POINT ( 'NONE',  ( 9.457646018065525792E-16, -7.312499998634403475, 5.148502694627439702 ) ) ;
#12134=CARTESIAN_POINT ( 'NONE',  ( -3.152548672688508926E-16, -91.56249999863440792, -5.148502694627439702 ) ) ;
#12136=CARTESIAN_POINT ( 'NONE',  ( -4.458734124999999437, -86.64583333196773651, -2.574251347313719407 ) ) ;
#12139=AXIS2_PLACEMENT_3D ( 'NONE', #10994, #21927, #60855 ) ;
#12142=CARTESIAN_POINT ( 'NONE',  ( 4.458734124999999437, -8.812499998634406140, -5.460374474430324690E-16 ) ) ;
#12143=CARTESIAN_POINT ( 'NONE',  ( -2.229367062500000163, 18.27083333469892779, -3.861377020970580443 ) ) ;
#12144=ADVANCED_FACE ( 'NONE', ( #15329 ), #19190, .T. ) ;
#12145=CARTESIAN_POINT ( 'NONE',  ( 4.458734125000000326, -53.14583333196773651, 2.574251347313718519 ) ) ;
#12146=CARTESIAN_POINT ( 'NONE',  ( 3.044556291839386294E-14, 16.87500000273118417, -5.000000000000000000 ) ) ;
#12149=CARTESIAN_POINT ( 'NONE',  ( 2.500000000000002220, -106.5416666639354730, 4.330127018922192761 ) ) ;
#12153=CARTESIAN_POINT ( 'NONE',  ( 2.229367062499998831, -77.64583333196773651, -3.861377020970580887 ) ) ;
#12154=CARTESIAN_POINT ( 'NONE',  ( -3.535250795749689387E-16, -110.1249999972687874, -5.773502691896257311 ) ) ;
#12161=CARTESIAN_POINT ( 'NONE',  ( 2.500000000000002220, -66.66666666666667140, 4.330127018922192761 ) ) ;
#12165=CARTESIAN_POINT ( 'NONE',  ( -4.999999999999998224, -61.79166666393547303, 2.886751345948131764 ) ) ;
#12167=CARTESIAN_POINT ( 'NONE',  ( -1.339745962155613146, 28.20534180126148271, 5.000000000000000000 ) ) ;
#12168=CARTESIAN_POINT ( 'NONE',  ( -4.999999999999998224, -106.7916666639354730, 2.886751345948131764 ) ) ;
#12171=VECTOR ( 'NONE', #40648, 1000.000000000000000 ) ;
#12173=( BOUNDED_CURVE ( )  B_SPLINE_CURVE ( 2, ( #30370, #5944, #25550, #45170, #1137, #14468, #33463, #53087, #9023 ),
 .UNSPECIFIED., .F., .F. ) 
 B_SPLINE_CURVE_WITH_KNOTS ( ( 3, 2, 2, 2, 3 ),
 ( 0.9232142857142857650, 0.9238095238095238582, 0.9250000000000000444, 0.9261904761904762307, 0.9267857142857143238 ),
 .UNSPECIFIED. ) 
 CURVE ( )  GEOMETRIC_REPRESENTATION_ITEM ( )  RATIONAL_B_SPLINE_CURVE ( ( 0.9330127018922194093, 0.9330127018922194093, 1.000000000000000000, 0.8660254037844387076, 1.000000000000000000, 0.8660254037844387076, 1.000000000000000000, 0.9330127018922194093, 0.9330127018922194093 ) ) 
 REPRESENTATION_ITEM ( '' )  );
#12184=CARTESIAN_POINT ( 'NONE',  ( -2.229367062499996610, -52.39583333196773651, 3.861377020970582219 ) ) ;
#12185=CARTESIAN_POINT ( 'NONE',  ( -2.500000000000000444, -0.04166666393548221214, -4.330127018922193649 ) ) ;
#12191=( BOUNDED_CURVE ( )  B_SPLINE_CURVE ( 2, ( #2410, #13560, #40674, #42500, #21713, #31027, #18056, #60319, #50978 ),
 .UNSPECIFIED., .F., .F. ) 
 B_SPLINE_CURVE_WITH_KNOTS ( ( 3, 2, 2, 2, 3 ),
 ( 0.7053571428571429047, 0.7059523809523809978, 0.7071428571428571841, 0.7083333333333333703, 0.7089285714285714635 ),
 .UNSPECIFIED. ) 
 CURVE ( )  GEOMETRIC_REPRESENTATION_ITEM ( )  RATIONAL_B_SPLINE_CURVE ( ( 0.9330127018922194093, 0.9330127018922194093, 1.000000000000000000, 0.8660254037844387076, 1.000000000000000000, 0.8660254037844387076, 1.000000000000000000, 0.9330127018922194093, 0.9330127018922194093 ) ) 
 REPRESENTATION_ITEM ( '' )  );
#12192=CARTESIAN_POINT ( 'NONE',  ( 5.000000000000000000, 22.58333333333333215, -2.886751345948130876 ) ) ;
#12194=CARTESIAN_POINT ( 'NONE',  ( -4.458734124999998549, -101.4791666653010651, 2.574251347313722516 ) ) ;
#12199=EDGE_CURVE ( 'NONE', #19063, #50378, #34965, .T. ) ;
#12200=CARTESIAN_POINT ( 'NONE',  ( -3.152548672688508926E-16, -3.562499998634408360, -5.148502694627439702 ) ) ;
#12201=CARTESIAN_POINT ( 'NONE',  ( -3.152548672688508926E-16, -95.81249999863442213, -5.148502694627439702 ) ) ;
#12202=EDGE_CURVE ( 'NONE', #34735, #55556, #28008, .T. ) ;
#12203=EDGE_CURVE ( 'NONE', #44569, #58717, #40717, .T. ) ;
#12205=CARTESIAN_POINT ( 'NONE',  ( -2.229367062500000163, -23.72916666530107577, -3.861377020970580443 ) ) ;
#12206=CARTESIAN_POINT ( 'NONE',  ( 5.000000000000000888, -46.58333333333334991, 2.886751345948126879 ) ) ;
#12212=AXIS2_PLACEMENT_3D ( 'NONE', #27509, #47139, #41985 ) ;
#12213=CARTESIAN_POINT ( 'NONE',  ( 2.229367062500001939, 9.770833334698927786, 3.861377020970579999 ) ) ;
#12214=ORIENTED_EDGE ( 'NONE', *, *, #49250, .T. ) ;
#12215=CARTESIAN_POINT ( 'NONE',  ( -2.500000000000000444, -81.16666666666667140, -4.330127018922193649 ) ) ;
#12217=CARTESIAN_POINT ( 'NONE',  ( -5.000000000000000000, -85.08333333333332860, -2.886751345948128211 ) ) ;
#12218=CARTESIAN_POINT ( 'NONE',  ( -2.229367062499996610, -27.14583333196774007, 3.861377020970582219 ) ) ;
#12222=CARTESIAN_POINT ( 'NONE',  ( 1.339745962155615144, -79.58034179853028434, 4.999999999999999112 ) ) ;
#12224=CARTESIAN_POINT ( 'NONE',  ( -2.500000000000000444, -48.04166666393547303, -4.330127018922193649 ) ) ;
#12225=CYLINDRICAL_SURFACE ( 'NONE', #12845, 5.000000000000000000 ) ;
#12226=CARTESIAN_POINT ( 'NONE',  ( -2.229367062500000163, 7.520833334698929562, -3.861377020970580443 ) ) ;
#12228=EDGE_CURVE ( 'NONE', #11847, #10332, #41527, .T. ) ;
#12231=CARTESIAN_POINT ( 'NONE',  ( -4.458734124999999437, -68.39583333196773651, -2.574251347313719407 ) ) ;
#12233=CARTESIAN_POINT ( 'NONE',  ( -2.500000000000000444, -3.166666666666664742, -4.330127018922193649 ) ) ;
#12236=CARTESIAN_POINT ( 'NONE',  ( 4.458734124999998549, -62.72916666530106511, -2.574251347313721627 ) ) ;
#12237=CARTESIAN_POINT ( 'NONE',  ( 1.060575238724906964E-15, -94.62499999726881583, 5.773502691896257311 ) ) ;
#12239=LINE ( 'NONE', #7423, #42877 ) ;
#12243=CARTESIAN_POINT ( 'NONE',  ( 1.060575238724906964E-15, -46.75000000000000000, 5.773502691896257311 ) ) ;
#12245=CARTESIAN_POINT ( 'NONE',  ( -5.000000000000000000, 16.00000000000000000, 0.000000000000000000 ) ) ;
#12247=CARTESIAN_POINT ( 'NONE',  ( 4.458734124999998549, -105.7291666653010651, -2.574251347313721627 ) ) ;
#12248=CARTESIAN_POINT ( 'NONE',  ( 9.457646018065525792E-16, -3.312499998634407472, 5.148502694627439702 ) ) ;
#12249=( BOUNDED_CURVE ( )  B_SPLINE_CURVE ( 2, ( #27513, #47451, #22067, #51660, #46823, #41659, #2767, #61629, #17563 ),
 .UNSPECIFIED., .F., .F. ) 
 B_SPLINE_CURVE_WITH_KNOTS ( ( 3, 2, 2, 2, 3 ),
 ( 0.4196428571428571508, 0.4202380952380952439, 0.4214285714285714302, 0.4226190476190476164, 0.4232142857142857095 ),
 .UNSPECIFIED. ) 
 CURVE ( )  GEOMETRIC_REPRESENTATION_ITEM ( )  RATIONAL_B_SPLINE_CURVE ( ( 0.9330127018922194093, 0.9330127018922194093, 1.000000000000000000, 0.8660254037844387076, 1.000000000000000000, 0.8660254037844387076, 1.000000000000000000, 0.9330127018922194093, 0.9330127018922194093 ) ) 
 REPRESENTATION_ITEM ( '' )  );
#12252=CARTESIAN_POINT ( 'NONE',  ( -1.339745962155613812, -6.205341801261478274, -5.000000000000000000 ) ) ;
#12255=ORIENTED_EDGE ( 'NONE', *, *, #49558, .F. ) ;
#12262=CARTESIAN_POINT ( 'NONE',  ( 2.229367062500001939, -37.22916666530107221, 3.861377020970579999 ) ) ;
#12263=MECHANICAL_DESIGN_GEOMETRIC_PRESENTATION_REPRESENTATION('',(#24551),#49208);
#12268=VECTOR ( 'NONE', #2962, 1000.000000000000000 ) ;
#12273=CARTESIAN_POINT ( 'NONE',  ( 9.457646018065525792E-16, -80.31249999863440792, 5.148502694627439702 ) ) ;
#12275=VERTEX_POINT ( 'NONE', #11133 ) ;
#12276=DIRECTION ( 'NONE',  ( -0.000000000000000000, 1.000000000000000000, -0.000000000000000000 ) ) ;
#12279=CARTESIAN_POINT ( 'NONE',  ( 2.229367062499998831, -10.89583333196773829, -3.861377020970580887 ) ) ;
#12282=EDGE_CURVE ( 'NONE', #18224, #50232, #48103, .T. ) ;
#12283=CARTESIAN_POINT ( 'NONE',  ( 1.975475456537005874E-15, -83.74999999999998579, 5.000000000000000000 ) ) ;
#12284=CARTESIAN_POINT ( 'NONE',  ( -2.229367062500000163, -4.729166665301071326, -3.861377020970580443 ) ) ;
#12289=ADVANCED_FACE ( 'NONE', ( #50058 ), #44919, .T. ) ;
#12290=CARTESIAN_POINT ( 'NONE',  ( 4.458734124999999437, 23.93750000136559564, -5.460374474430324690E-16 ) ) ;
#12291=ORIENTED_EDGE ( 'NONE', *, *, #53534, .F. ) ;
#12292=CARTESIAN_POINT ( 'NONE',  ( -4.458734124999997661, -88.22916666530107932, 2.574251347313722516 ) ) ;
#12293=CARTESIAN_POINT ( 'NONE',  ( 4.458734124999999437, -1.812499998634406584, -5.460374474430324690E-16 ) ) ;
#12294=EDGE_CURVE ( 'NONE', #58440, #6256, #35267, .T. ) ;
#12295=DIRECTION ( 'NONE',  ( -0.000000000000000000, 1.000000000000000000, -0.000000000000000000 ) ) ;
#12296=EDGE_CURVE ( 'NONE', #36130, #47006, #30759, .T. ) ;
#12297=CARTESIAN_POINT ( 'NONE',  ( 5.000000000000000000, -32.37499999726880873, -6.123233995736766282E-16 ) ) ;
#12298=CARTESIAN_POINT ( 'NONE',  ( -2.480964764533239819E-13, -59.75000000000000711, 5.000000000000000000 ) ) ;
#12299=CARTESIAN_POINT ( 'NONE',  ( 4.458734124999999437, 25.18750000136559208, -5.460374474430324690E-16 ) ) ;
#12300=CARTESIAN_POINT ( 'NONE',  ( -6.972266317189433020E-16, -7.249999999999998224, -5.000000000000000000 ) ) ;
#12303=CARTESIAN_POINT ( 'NONE',  ( 2.229367062499998831, -50.64583333196772941, -3.861377020970580887 ) ) ;
#12304=CARTESIAN_POINT ( 'NONE',  ( -4.458734124999999437, -39.64583333196773651, -2.574251347313719407 ) ) ;
#12308=CARTESIAN_POINT ( 'NONE',  ( 5.000000000000000000, 17.50000000000000000, -6.123233995736766282E-16 ) ) ;
#12309=ADVANCED_FACE ( 'NONE', ( #31712 ), #3093, .T. ) ;
#12313=CARTESIAN_POINT ( 'NONE',  ( 9.457646018065525792E-16, -43.06249999863440081, 5.148502694627439702 ) ) ;
#12314=CARTESIAN_POINT ( 'NONE',  ( -5.000000000000000000, -79.87499999726881583, 0.000000000000000000 ) ) ;
#12319=CARTESIAN_POINT ( 'NONE',  ( 4.458734124999999437, -85.06249999863439371, -5.460374474430324690E-16 ) ) ;
#12321=CARTESIAN_POINT ( 'NONE',  ( 2.500000000000002220, -33.66666666666666430, 4.330127018922192761 ) ) ;
#12323=ORIENTED_EDGE ( 'NONE', *, *, #5099, .T. ) ;
#12326=CARTESIAN_POINT ( 'NONE',  ( 4.458734124999999437, -92.81249999863440792, -5.460374474430324690E-16 ) ) ;
#12327=CARTESIAN_POINT ( 'NONE',  ( -2.229367062499996610, 15.60416666803225993, 3.861377020970582219 ) ) ;
#12328=CARTESIAN_POINT ( 'NONE',  ( 2.499999999999998668, 16.79166666939785202, -4.330127018922193649 ) ) ;
#12334=CARTESIAN_POINT ( 'NONE',  ( 0.000000000000000000, -120.0000000000000000, 5.000000000000000000 ) ) ;
#12335=CARTESIAN_POINT ( 'NONE',  ( 2.500000000000002220, -1.666666666666663410, 4.330127018922192761 ) ) ;
#12338=CARTESIAN_POINT ( 'NONE',  ( 1.975475456537005874E-15, -96.75000000000000000, 5.000000000000000000 ) ) ;
#12339=CARTESIAN_POINT ( 'NONE',  ( 1.975475456537005874E-15, 14.25000000000000000, 5.000000000000000000 ) ) ;
#12340=CARTESIAN_POINT ( 'NONE',  ( 4.458734124999999437, -12.06249999863440081, -5.460374474430324690E-16 ) ) ;
#12347=ORIENTED_EDGE ( 'NONE', *, *, #26834, .F. ) ;
#12348=CYLINDRICAL_SURFACE ( 'NONE', #22060, 5.000000000000000000 ) ;
#12350=CARTESIAN_POINT ( 'NONE',  ( -2.229367062499996610, -63.39583333196774362, 3.861377020970582219 ) ) ;
#12353=ORIENTED_EDGE ( 'NONE', *, *, #31046, .T. ) ;
#12354=CARTESIAN_POINT ( 'NONE',  ( 1.975475456537005874E-15, -46.74999999999999289, 5.000000000000000000 ) ) ;
#12360=CARTESIAN_POINT ( 'NONE',  ( 2.229367062500001939, 8.020833334698926009, 3.861377020970579999 ) ) ;
#12363=CARTESIAN_POINT ( 'NONE',  ( 2.493747252781420335E-13, -78.12499999726881583, -5.000000000000000000 ) ) ;
#12366=CARTESIAN_POINT ( 'NONE',  ( 4.458734125000000326, -69.89583333196773651, 2.574251347313718519 ) ) ;
#12368=CARTESIAN_POINT ( 'NONE',  ( -4.458734124999998549, 12.77083333469892601, 2.574251347313722516 ) ) ;
#12369=VECTOR ( 'NONE', #49528, 1000.000000000000000 ) ;
#12372=CARTESIAN_POINT ( 'NONE',  ( 2.229367062500001939, -55.22916666530107221, 3.861377020970579999 ) ) ;
#12373=CARTESIAN_POINT ( 'NONE',  ( 2.500000000000002220, -12.54166666393548013, 4.330127018922192761 ) ) ;
#12374=CARTESIAN_POINT ( 'NONE',  ( 1.243387493232115550E-13, -9.124999997268817609, -5.000000000000000000 ) ) ;
#12377=CARTESIAN_POINT ( 'NONE',  ( 4.458734125000001214, -32.89583333196774362, 2.574251347313718519 ) ) ;
#12378=CARTESIAN_POINT ( 'NONE',  ( 9.457646018065525792E-16, -22.31249999863440792, 5.148502694627439702 ) ) ;
#12379=ORIENTED_EDGE ( 'NONE', *, *, #24306, .T. ) ;
#12381=CARTESIAN_POINT ( 'NONE',  ( -4.458734124999999437, -109.3124999986343937, 0.000000000000000000 ) ) ;
#12383=ORIENTED_EDGE ( 'NONE', *, *, #35116, .F. ) ;
#12384=CARTESIAN_POINT ( 'NONE',  ( -4.458734124999998549, -103.4791666653010509, 2.574251347313722516 ) ) ;
#12385=CARTESIAN_POINT ( 'NONE',  ( 4.458734125000001214, -27.89583333196774007, 2.574251347313718519 ) ) ;
#12386=CARTESIAN_POINT ( 'NONE',  ( -2.499999999999996447, -62.70833333060214443, 4.330127018922195425 ) ) ;
#12389=CARTESIAN_POINT ( 'NONE',  ( 4.458734124999999437, -30.81249999863440436, -5.460374474430324690E-16 ) ) ;
#12390=CARTESIAN_POINT ( 'NONE',  ( 2.229367062499998831, -67.89583333196773651, -3.861377020970580887 ) ) ;
#12391=CARTESIAN_POINT ( 'NONE',  ( 5.000000000000000000, 8.583333333333332149, -2.886751345948130876 ) ) ;
#12393=CARTESIAN_POINT ( 'NONE',  ( 1.339745962155615144, -5.580341798530291442, 4.999999999999999112 ) ) ;
#12394=CARTESIAN_POINT ( 'NONE',  ( -3.535250795749689387E-16, -16.25000000000000000, -5.773502691896257311 ) ) ;
#12396=ORIENTED_EDGE ( 'NONE', *, *, #6693, .T. ) ;
#12397=AXIS2_PLACEMENT_3D ( 'NONE', #34496, #49311, #34191 ) ;
#12401=CARTESIAN_POINT ( 'NONE',  ( -2.499999999999996447, -0.8333333333333317050, 4.330127018922195425 ) ) ;
#12403=AXIS2_PLACEMENT_3D ( 'NONE', #59218, #29935, #5501 ) ;
#12404=CARTESIAN_POINT ( 'NONE',  ( 5.000000000000000888, -76.45833333060215864, 2.886751345948126879 ) ) ;
#12412=ORIENTED_EDGE ( 'NONE', *, *, #31527, .F. ) ;
#12423=( BOUNDED_CURVE ( )  B_SPLINE_CURVE ( 2, ( #31951, #7835, #27436, #37728, #22950, #47070, #17792, #60922, #37416 ),
 .UNSPECIFIED., .F., .F. ) 
 B_SPLINE_CURVE_WITH_KNOTS ( ( 3, 2, 2, 2, 3 ),
 ( 0.9732142857142856984, 0.9738095238095237915, 0.9749999999999999778, 0.9761904761904761640, 0.9767857142857142572 ),
 .UNSPECIFIED. ) 
 CURVE ( )  GEOMETRIC_REPRESENTATION_ITEM ( )  RATIONAL_B_SPLINE_CURVE ( ( 0.9330127018922194093, 0.9330127018922194093, 1.000000000000000000, 0.8660254037844387076, 1.000000000000000000, 0.8660254037844387076, 1.000000000000000000, 0.9330127018922194093, 0.9330127018922194093 ) ) 
 REPRESENTATION_ITEM ( '' )  );
#12424=DIRECTION ( 'NONE',  ( -0.000000000000000000, 1.000000000000000000, -0.000000000000000000 ) ) ;
#12429=CARTESIAN_POINT ( 'NONE',  ( 2.229367062500001939, -76.97916666530106511, 3.861377020970579999 ) ) ;
#12430=CARTESIAN_POINT ( 'NONE',  ( 2.229367062499998831, 22.35416666803225993, -3.861377020970580887 ) ) ;
#12431=CARTESIAN_POINT ( 'NONE',  ( -1.339745962155613812, -54.20534180126147561, -5.000000000000000000 ) ) ;
#12439=CARTESIAN_POINT ( 'NONE',  ( -4.458734124999999437, -54.31249999863440081, 0.000000000000000000 ) ) ;
#12442=CARTESIAN_POINT ( 'NONE',  ( -5.000000000000000000, -105.0000000000000142, 0.000000000000000000 ) ) ;
#12444=CARTESIAN_POINT ( 'NONE',  ( -4.458734124999999437, -38.56249999863440081, 0.000000000000000000 ) ) ;
#12445=CARTESIAN_POINT ( 'NONE',  ( -5.000000000000000000, -0.9583333306021485365, -2.886751345948128211 ) ) ;
#12451=CARTESIAN_POINT ( 'NONE',  ( -4.458734124999999437, -104.3958333319677365, -2.574251347313719407 ) ) ;
#12452=CARTESIAN_POINT ( 'NONE',  ( -2.229367062499996610, -4.395833331967740065, 3.861377020970582219 ) ) ;
#12454=CARTESIAN_POINT ( 'NONE',  ( -6.972266317189433020E-16, -58.24999999999999289, -5.000000000000000000 ) ) ;
#12455=CARTESIAN_POINT ( 'NONE',  ( -2.229367062500000163, -92.47916666530106511, -3.861377020970580443 ) ) ;
#12457=CARTESIAN_POINT ( 'NONE',  ( 2.229367062500001939, -87.22916666530107932, 3.861377020970579999 ) ) ;
#12459=CARTESIAN_POINT ( 'NONE',  ( 5.000000000000000000, -2.374999997268815388, -6.123233995736766282E-16 ) ) ;
#12461=CARTESIAN_POINT ( 'NONE',  ( 4.458734124999998549, -9.729166665301068662, -2.574251347313721627 ) ) ;
#12462=CARTESIAN_POINT ( 'NONE',  ( 4.458734124999999437, 15.93750000136559564, -5.460374474430324690E-16 ) ) ;
#12463=CARTESIAN_POINT ( 'NONE',  ( -4.458734124999997661, -55.47916666530106511, 2.574251347313722516 ) ) ;
#12465=CARTESIAN_POINT ( 'NONE',  ( -4.999999999999998224, -36.91666666666667140, 2.886751345948131764 ) ) ;
#12467=CARTESIAN_POINT ( 'NONE',  ( -4.999999999999998224, -38.91666666666667140, 2.886751345948131764 ) ) ;
#12470=( BOUNDED_CURVE ( )  B_SPLINE_CURVE ( 2, ( #60826, #60509, #60193, #55365, #11280, #1981, #40552, #30256, #50849 ),
 .UNSPECIFIED., .F., .F. ) 
 B_SPLINE_CURVE_WITH_KNOTS ( ( 3, 2, 2, 2, 3 ),
 ( 0.9839285714285714857, 0.9845238095238095788, 0.9857142857142857650, 0.9869047619047619513, 0.9875000000000000444 ),
 .UNSPECIFIED. ) 
 CURVE ( )  GEOMETRIC_REPRESENTATION_ITEM ( )  RATIONAL_B_SPLINE_CURVE ( ( 0.9330127018922194093, 0.9330127018922256266, 1.000000000000000000, 0.8660254037844387076, 1.000000000000000000, 0.8660254037844387076, 1.000000000000000000, 0.9330127018922194093, 0.9330127018922194093 ) ) 
 REPRESENTATION_ITEM ( '' )  );
#12473=CARTESIAN_POINT ( 'NONE',  ( -2.229367062499996610, -82.14583333196773651, 3.861377020970582219 ) ) ;
#12474=CARTESIAN_POINT ( 'NONE',  ( -4.458734124999999437, 26.35416666803226349, -2.574251347313719407 ) ) ;
#12479=CARTESIAN_POINT ( 'NONE',  ( 5.000000000000000000, -65.50000000000000000, -6.123233995736766282E-16 ) ) ;
#12484=CARTESIAN_POINT ( 'NONE',  ( 2.499999999999998668, 7.666666666666665186, -4.330127018922193649 ) ) ;
#12485=CARTESIAN_POINT ( 'NONE',  ( -5.000000000000000000, -72.00000000000000000, 0.000000000000000000 ) ) ;
#12492=ORIENTED_EDGE ( 'NONE', *, *, #28311, .T. ) ;
#12495=ORIENTED_EDGE ( 'NONE', *, *, #51869, .T. ) ;
#12498=CARTESIAN_POINT ( 'NONE',  ( -3.152548672688508926E-16, -49.81249999863440081, -5.148502694627439702 ) ) ;
#12500=CARTESIAN_POINT ( 'NONE',  ( -1.339745962155610925, -21.66965819600733312, 5.000000000000000000 ) ) ;
#12509=CARTESIAN_POINT ( 'NONE',  ( 2.229367062500001939, -97.22916666530105090, 3.861377020970579999 ) ) ;
#12510=DIRECTION ( 'NONE',  ( -0.000000000000000000, 1.000000000000000000, -0.000000000000000000 ) ) ;
#12515=CARTESIAN_POINT ( 'NONE',  ( -2.229367062500000163, -7.479166665301073991, -3.861377020970580443 ) ) ;
#12516=CARTESIAN_POINT ( 'NONE',  ( 4.458734125000000326, -98.14583333196773651, 2.574251347313718519 ) ) ;
#12518=CARTESIAN_POINT ( 'NONE',  ( -4.458734124999999437, -21.64583333196774362, -2.574251347313719407 ) ) ;
#12525=CARTESIAN_POINT ( 'NONE',  ( -3.152548672688508926E-16, 10.18750000136559208, -5.148502694627439702 ) ) ;
#12527=CARTESIAN_POINT ( 'NONE',  ( -1.339745962155613812, -53.08034179853029144, -5.000000000000000000 ) ) ;
#12529=CARTESIAN_POINT ( 'NONE',  ( 2.499999999999998668, -88.33333333333332860, -4.330127018922193649 ) ) ;
#12530=CARTESIAN_POINT ( 'NONE',  ( -2.229367062500000163, -25.47916666530106866, -3.861377020970580443 ) ) ;
#12532=CARTESIAN_POINT ( 'NONE',  ( 4.458734125000001214, -73.14583333196773651, 2.574251347313718519 ) ) ;
#12533=DIRECTION ( 'NONE',  ( 0.000000000000000000, 0.000000000000000000, 1.000000000000000000 ) ) ;
#12535=ADVANCED_FACE ( 'NONE', ( #61632 ), #51971, .T. ) ;
#12536=CARTESIAN_POINT ( 'NONE',  ( 1.975475456537005874E-15, -24.74999999999999645, 5.000000000000000000 ) ) ;
#12537=CARTESIAN_POINT ( 'NONE',  ( -3.152548672688508926E-16, 10.43750000136559386, -5.148502694627439702 ) ) ;
#12539=CARTESIAN_POINT ( 'NONE',  ( -4.458734124999999437, -71.31249999863439371, 0.000000000000000000 ) ) ;
#12541=CARTESIAN_POINT ( 'NONE',  ( 2.500000000000002220, 0.3333333333333348136, 4.330127018922192761 ) ) ;
#12545=CARTESIAN_POINT ( 'NONE',  ( -4.458734124999998549, -66.22916666530107932, 2.574251347313722516 ) ) ;
#12546=CARTESIAN_POINT ( 'NONE',  ( 2.499999999999998668, -100.2083333306021444, -4.330127018922193649 ) ) ;
#12552=CARTESIAN_POINT ( 'NONE',  ( -2.499999999999996447, -49.83333333333332860, 4.330127018922195425 ) ) ;
#12553=CARTESIAN_POINT ( 'NONE',  ( -1.339745962155610259, 26.79465819873851729, -5.000000000000002665 ) ) ;
#12554=CARTESIAN_POINT ( 'NONE',  ( -4.999999999999998224, 16.08333333333333215, 2.886751345948131764 ) ) ;
#12555=VERTEX_POINT ( 'NONE', #42308 ) ;
#12556=CARTESIAN_POINT ( 'NONE',  ( 2.499999999999998668, -94.33333333333332860, -4.330127018922193649 ) ) ;
#12565=ORIENTED_EDGE ( 'NONE', *, *, #13014, .F. ) ;
#12568=ORIENTED_EDGE ( 'NONE', *, *, #62179, .T. ) ;
#12572=CARTESIAN_POINT ( 'NONE',  ( -4.458734124999999437, -35.64583333196772941, -2.574251347313719407 ) ) ;
#12576=EDGE_CURVE ( 'NONE', #43124, #42363, #16931, .T. ) ;
#12582=EDGE_CURVE ( 'NONE', #23583, #28403, #25565, .T. ) ;
#12583=CARTESIAN_POINT ( 'NONE',  ( -4.458734124999999437, -82.64583333196772230, -2.574251347313719407 ) ) ;
#12584=CARTESIAN_POINT ( 'NONE',  ( 2.500000000000002220, 3.333333333333333925, 4.330127018922192761 ) ) ;
#12586=EDGE_CURVE ( 'NONE', #14724, #47799, #62959, .T. ) ;
#12590=CARTESIAN_POINT ( 'NONE',  ( -4.458734124999999437, -40.39583333196773651, -2.574251347313719407 ) ) ;
#12591=CARTESIAN_POINT ( 'NONE',  ( -4.458734124999999437, -7.562499998634404363, 0.000000000000000000 ) ) ;
#12595=CARTESIAN_POINT ( 'NONE',  ( -4.458734124999999437, -7.645833331967735624, -2.574251347313719407 ) ) ;
#12600=CARTESIAN_POINT ( 'NONE',  ( -2.229367062500000163, 28.27083333469892779, -3.861377020970580443 ) ) ;
#12602=CARTESIAN_POINT ( 'NONE',  ( -4.458734124999999437, -88.39583333196773651, -2.574251347313719407 ) ) ;
#12604=CARTESIAN_POINT ( 'NONE',  ( -4.458734124999999437, -8.395833331967736513, -2.574251347313719407 ) ) ;
#12607=CARTESIAN_POINT ( 'NONE',  ( 1.975475456537005874E-15, -48.74999999999999289, 5.000000000000000000 ) ) ;
#12608=CARTESIAN_POINT ( 'NONE',  ( 5.000000000000000000, -37.29166666393548013, -2.886751345948129988 ) ) ;
#12610=CARTESIAN_POINT ( 'NONE',  ( -3.152548672688508926E-16, 26.43750000136559564, -5.148502694627439702 ) ) ;
#12611=CARTESIAN_POINT ( 'NONE',  ( -6.972266317189433020E-16, -98.12499999726880162, -5.000000000000000000 ) ) ;
#12613=CARTESIAN_POINT ( 'NONE',  ( 9.457646018065525792E-16, -55.06249999863439371, 5.148502694627439702 ) ) ;
#12616=LINE ( 'NONE', #1718, #53474 ) ;
#12617=CARTESIAN_POINT ( 'NONE',  ( -5.000000000000000000, 13.99999999999999822, 0.000000000000000000 ) ) ;
#12620=CARTESIAN_POINT ( 'NONE',  ( 4.458734124999998549, -45.72916666530106511, -2.574251347313721627 ) ) ;
#12621=CARTESIAN_POINT ( 'NONE',  ( 2.499999999999998668, -80.20833333060213022, -4.330127018922193649 ) ) ;
#12623=CARTESIAN_POINT ( 'NONE',  ( -6.972266317189433020E-16, -37.12499999726881583, -5.000000000000000000 ) ) ;
#12625=CARTESIAN_POINT ( 'NONE',  ( -4.458734124999999437, -86.64583333196773651, -2.574251347313719407 ) ) ;
#12627=CARTESIAN_POINT ( 'NONE',  ( -2.500000000000000444, -30.16666666666666785, -4.330127018922193649 ) ) ;
#12631=CARTESIAN_POINT ( 'NONE',  ( -2.229367062500000163, -96.47916666530105090, -3.861377020970580443 ) ) ;
#12632=CARTESIAN_POINT ( 'NONE',  ( 4.458734124999998549, 14.02083333469892779, -2.574251347313721627 ) ) ;
#12633=CARTESIAN_POINT ( 'NONE',  ( -3.535250795749689387E-16, 16.87500000273118417, -5.773502691896257311 ) ) ;
#12634=CARTESIAN_POINT ( 'NONE',  ( -2.500000000000000444, -60.16666666666665719, -4.330127018922193649 ) ) ;
#12637=CARTESIAN_POINT ( 'NONE',  ( 5.000000000000000888, -61.45833333060214443, 2.886751345948126879 ) ) ;
#12638=CARTESIAN_POINT ( 'NONE',  ( 2.499999999999998668, -82.33333333333332860, -4.330127018922193649 ) ) ;
#12642=CARTESIAN_POINT ( 'NONE',  ( 2.499999999999998668, -40.20833333060214443, -4.330127018922193649 ) ) ;
#12643=CARTESIAN_POINT ( 'NONE',  ( -1.339745962155610925, -12.66965819600733134, 5.000000000000000000 ) ) ;
#12644=EDGE_CURVE ( 'NONE', #45741, #1619, #58994, .T. ) ;
#12645=CARTESIAN_POINT ( 'NONE',  ( 2.500000000000002220, -109.6666666666666572, 4.330127018922192761 ) ) ;
#12648=( BOUNDED_CURVE ( )  B_SPLINE_CURVE ( 2, ( #48062, #43541, #23940, #45059, #29060, #10957, #35412, #23636, #57733 ),
 .UNSPECIFIED., .F., .F. ) 
 B_SPLINE_CURVE_WITH_KNOTS ( ( 3, 2, 2, 2, 3 ),
 ( 0.7696428571428571841, 0.7702380952380952772, 0.7714285714285714635, 0.7726190476190476497, 0.7732142857142857428 ),
 .UNSPECIFIED. ) 
 CURVE ( )  GEOMETRIC_REPRESENTATION_ITEM ( )  RATIONAL_B_SPLINE_CURVE ( ( 0.9330127018922194093, 0.9330127018922194093, 1.000000000000000000, 0.8660254037844387076, 1.000000000000000000, 0.8660254037844387076, 1.000000000000000000, 0.9330127018922194093, 0.9330127018922194093 ) ) 
 REPRESENTATION_ITEM ( '' )  );
#12649=CARTESIAN_POINT ( 'NONE',  ( -4.458734124999999437, -18.56249999863440792, 0.000000000000000000 ) ) ;
#12655=EDGE_CURVE ( 'NONE', #26835, #19510, #60905, .T. ) ;
#12661=ORIENTED_EDGE ( 'NONE', *, *, #5968, .T. ) ;
#12662=CARTESIAN_POINT ( 'NONE',  ( -2.229367062499996610, -67.39583333196773651, 3.861377020970582219 ) ) ;
#12663=CARTESIAN_POINT ( 'NONE',  ( -6.972266317189433020E-16, -100.2499999999999858, -5.000000000000000000 ) ) ;
#12664=( NAMED_UNIT ( * ) SI_UNIT ( $, .STERADIAN. ) SOLID_ANGLE_UNIT ( ) );
#12667=EDGE_CURVE ( 'NONE', #22959, #26195, #3789, .T. ) ;
#12673=VERTEX_POINT ( 'NONE', #15580 ) ;
#12675=CARTESIAN_POINT ( 'NONE',  ( 4.458734125000001214, 11.10416666803225993, 2.574251347313718519 ) ) ;
#12678=CARTESIAN_POINT ( 'NONE',  ( -6.972266317189433020E-16, -108.1249999972688158, -5.000000000000000000 ) ) ;
#12681=CARTESIAN_POINT ( 'NONE',  ( -4.458734124999999437, -71.31249999863439371, 0.000000000000000000 ) ) ;
#12682=CARTESIAN_POINT ( 'NONE',  ( 2.500000000000002220, -10.54166666393547835, 4.330127018922192761 ) ) ;
#12683=CARTESIAN_POINT ( 'NONE',  ( -2.229367062499996610, 7.854166668032260823, 3.861377020970582219 ) ) ;
#12685=CARTESIAN_POINT ( 'NONE',  ( -2.229367062499996610, -58.39583333196773651, 3.861377020970582219 ) ) ;
#12686=CARTESIAN_POINT ( 'NONE',  ( -5.000000000000000000, -19.87499999726880873, 0.000000000000000000 ) ) ;
#12687=CARTESIAN_POINT ( 'NONE',  ( -5.000000000000000000, -100.0000000000000000, 0.000000000000000000 ) ) ;
#12688=CARTESIAN_POINT ( 'NONE',  ( -1.339745962155610925, -44.66965819600733312, 5.000000000000000000 ) ) ;
#12689=CARTESIAN_POINT ( 'NONE',  ( 1.339745962155615144, -30.58034179853029499, 4.999999999999999112 ) ) ;
#12690=CARTESIAN_POINT ( 'NONE',  ( 0.000000000000000000, -120.0000000000000000, 5.000000000000000000 ) ) ;
#12691=CARTESIAN_POINT ( 'NONE',  ( 4.458734125000001214, -35.89583333196773651, 2.574251347313718519 ) ) ;
#12692=CARTESIAN_POINT ( 'NONE',  ( -4.458734124999999437, -23.56249999863440436, 0.000000000000000000 ) ) ;
#12693=ORIENTED_EDGE ( 'NONE', *, *, #10323, .T. ) ;
#12695=CARTESIAN_POINT ( 'NONE',  ( 4.458734124999999437, -108.8124999986343937, -5.460374474430324690E-16 ) ) ;
#12697=EDGE_LOOP ( 'NONE', ( #7916, #10036, #16589, #20170 ) ) ;
#12698=CARTESIAN_POINT ( 'NONE',  ( -3.152548672688508926E-16, -107.8124999986343937, -5.148502694627439702 ) ) ;
#12699=CARTESIAN_POINT ( 'NONE',  ( 2.229367062500001939, -33.97916666530107221, 3.861377020970579999 ) ) ;
#12700=CARTESIAN_POINT ( 'NONE',  ( 5.000000000000000000, -64.29166666393547303, -2.886751345948129988 ) ) ;
#12703=CARTESIAN_POINT ( 'NONE',  ( 2.229367062500001939, -29.97916666530107221, 3.861377020970579999 ) ) ;
#12704=CARTESIAN_POINT ( 'NONE',  ( 9.457646018065525792E-16, -71.31249999863439371, 5.148502694627439702 ) ) ;
#12708=CARTESIAN_POINT ( 'NONE',  ( 2.499999999999998668, -18.33333333333333215, -4.330127018922193649 ) ) ;
#12710=ORIENTED_EDGE ( 'NONE', *, *, #57324, .T. ) ;
#12711=FACE_OUTER_BOUND ( 'NONE', #41933, .T. ) ;
#12719=LINE ( 'NONE', #8842, #9125 ) ;
#12722=VERTEX_POINT ( 'NONE', #40000 ) ;
#12740=( BOUNDED_CURVE ( )  B_SPLINE_CURVE ( 2, ( #22350, #16880, #2115, #47102, #42583, #47414, #27475, #32300, #51308 ),
 .UNSPECIFIED., .F., .F. ) 
 B_SPLINE_CURVE_WITH_KNOTS ( ( 3, 2, 2, 2, 3 ),
 ( 0.4410714285714285587, 0.4416666666666666519, 0.4428571428571428381, 0.4440476190476190244, 0.4446428571428571175 ),
 .UNSPECIFIED. ) 
 CURVE ( )  GEOMETRIC_REPRESENTATION_ITEM ( )  RATIONAL_B_SPLINE_CURVE ( ( 0.9330127018922194093, 0.9330127018922194093, 1.000000000000000000, 0.8660254037844387076, 1.000000000000000000, 0.8660254037844387076, 1.000000000000000000, 0.9330127018922194093, 0.9330127018922194093 ) ) 
 REPRESENTATION_ITEM ( '' )  );
#12741=EDGE_CURVE ( 'NONE', #57389, #47780, #40962, .T. ) ;
#12742=CARTESIAN_POINT ( 'NONE',  ( 2.229367062500001939, -80.97916666530106511, 3.861377020970579999 ) ) ;
#12743=CARTESIAN_POINT ( 'NONE',  ( -2.229367062500000163, 26.52083333469892779, -3.861377020970580443 ) ) ;
#12745=EDGE_LOOP ( 'NONE', ( #19810, #26250, #59340, #32658 ) ) ;
#12746=CARTESIAN_POINT ( 'NONE',  ( -5.000000000000000000, 29.12500000273118417, 0.000000000000000000 ) ) ;
#12752=CARTESIAN_POINT ( 'NONE',  ( -2.229367062499996610, -53.14583333196773651, 3.861377020970582219 ) ) ;
#12754=CARTESIAN_POINT ( 'NONE',  ( -4.458734124999999437, 29.68750000136559208, 0.000000000000000000 ) ) ;
#12755=CARTESIAN_POINT ( 'NONE',  ( -2.500000000000000444, -106.1666666666666572, -4.330127018922193649 ) ) ;
#12757=CARTESIAN_POINT ( 'NONE',  ( 4.458734125000001214, -43.14583333196773651, 2.574251347313718519 ) ) ;
#12758=CARTESIAN_POINT ( 'NONE',  ( 2.499999999999998668, 2.791666669397851130, -4.330127018922193649 ) ) ;
#12762=CARTESIAN_POINT ( 'NONE',  ( -2.229367062499996610, -103.1458333319677365, 3.861377020970582219 ) ) ;
#12763=CARTESIAN_POINT ( 'NONE',  ( -2.229367062500000163, -5.729166665301072214, -3.861377020970580443 ) ) ;
#12765=DIRECTION ( 'NONE',  ( -0.000000000000000000, 1.000000000000000000, -0.000000000000000000 ) ) ;
#12766=CARTESIAN_POINT ( 'NONE',  ( -4.458734124999999437, -94.39583333196773651, -2.574251347313719407 ) ) ;
#12768=CARTESIAN_POINT ( 'NONE',  ( -2.229367062499996610, -85.39583333196773651, 3.861377020970582219 ) ) ;
#12773=CARTESIAN_POINT ( 'NONE',  ( -4.458734124999999437, -14.39583333196773474, -2.574251347313719407 ) ) ;
#12774=CARTESIAN_POINT ( 'NONE',  ( -4.458734124999999437, 16.35416666803225993, -2.574251347313719407 ) ) ;
#12775=CARTESIAN_POINT ( 'NONE',  ( 2.229367062500001939, -54.22916666530107221, 3.861377020970579999 ) ) ;
#12779=CARTESIAN_POINT ( 'NONE',  ( -2.500000000000000444, -39.16666666666667140, -4.330127018922193649 ) ) ;
#12783=CARTESIAN_POINT ( 'NONE',  ( 5.000000000000000000, -76.41666666666665719, -2.886751345948130876 ) ) ;
#12784=CARTESIAN_POINT ( 'NONE',  ( -4.458734124999998549, -78.22916666530106511, 2.574251347313722516 ) ) ;
#12785=CARTESIAN_POINT ( 'NONE',  ( -2.229367062500000163, 23.27083333469892779, -3.861377020970580443 ) ) ;
#12788=EDGE_CURVE ( 'NONE', #34883, #26190, #36657, .T. ) ;
#12789=CARTESIAN_POINT ( 'NONE',  ( 1.975475456537005874E-15, -47.74999999999999289, 5.000000000000000000 ) ) ;
#12792=CARTESIAN_POINT ( 'NONE',  ( -2.500000000000000444, -62.16666666666666430, -4.330127018922193649 ) ) ;
#12796=ORIENTED_EDGE ( 'NONE', *, *, #20959, .F. ) ;
#12797=CARTESIAN_POINT ( 'NONE',  ( -6.972266317189433020E-16, -62.12499999726880162, -5.000000000000000000 ) ) ;
#12798=( BOUNDED_CURVE ( )  B_SPLINE_CURVE ( 2, ( #39687, #59657, #805, #24593, #4649, #44200, #10431, #20083, #59327 ),
 .UNSPECIFIED., .F., .F. ) 
 B_SPLINE_CURVE_WITH_KNOTS ( ( 3, 2, 2, 2, 3 ),
 ( 0.4196428571428571508, 0.4202380952380952439, 0.4214285714285714302, 0.4226190476190476164, 0.4232142857142857095 ),
 .UNSPECIFIED. ) 
 CURVE ( )  GEOMETRIC_REPRESENTATION_ITEM ( )  RATIONAL_B_SPLINE_CURVE ( ( 0.9330127018922194093, 0.9330127018922194093, 1.000000000000000000, 0.8660254037844387076, 1.000000000000000000, 0.8660254037844387076, 1.000000000000000000, 0.9330127018922194093, 0.9330127018922194093 ) ) 
 REPRESENTATION_ITEM ( '' )  );
#12800=DIRECTION ( 'NONE',  ( 0.000000000000000000, 0.000000000000000000, 1.000000000000000000 ) ) ;
#12806=EDGE_LOOP ( 'NONE', ( #26411, #11306, #26573, #16300 ) ) ;
#12809=ORIENTED_EDGE ( 'NONE', *, *, #29089, .F. ) ;
#12812=CARTESIAN_POINT ( 'NONE',  ( -2.229367062500000163, -51.72916666530107221, -3.861377020970580443 ) ) ;
#12814=CARTESIAN_POINT ( 'NONE',  ( -2.499999999999996447, -54.70833333060213732, 4.330127018922195425 ) ) ;
#12815=ORIENTED_EDGE ( 'NONE', *, *, #24694, .T. ) ;
#12821=CARTESIAN_POINT ( 'NONE',  ( -2.229367062499996610, -98.39583333196773651, 3.861377020970582219 ) ) ;
#12824=EDGE_LOOP ( 'NONE', ( #27159, #17469, #43886, #38216 ) ) ;
#12828=CARTESIAN_POINT ( 'NONE',  ( -4.458734124999999437, -9.395833331967736513, -2.574251347313719407 ) ) ;
#12829=CARTESIAN_POINT ( 'NONE',  ( -2.229367062499996610, -96.39583333196773651, 3.861377020970582219 ) ) ;
#12831=CARTESIAN_POINT ( 'NONE',  ( -3.152548672688508926E-16, -22.81249999863440436, -5.148502694627439702 ) ) ;
#12832=CYLINDRICAL_SURFACE ( 'NONE', #20103, 5.000000000000000000 ) ;
#12835=CARTESIAN_POINT ( 'NONE',  ( 0.000000000000000000, -120.0000000000000000, 5.000000000000000000 ) ) ;
#12836=DIRECTION ( 'NONE',  ( -0.000000000000000000, 1.000000000000000000, -0.000000000000000000 ) ) ;
#12838=( BOUNDED_CURVE ( )  B_SPLINE_CURVE ( 2, ( #4610, #20044, #24233, #5257, #43839, #39972, #15218, #59287, #49635 ),
 .UNSPECIFIED., .F., .F. ) 
 B_SPLINE_CURVE_WITH_KNOTS ( ( 3, 2, 2, 2, 3 ),
 ( 0.5946428571428571397, 0.5952380952380952328, 0.5964285714285714191, 0.5976190476190476053, 0.5982142857142856984 ),
 .UNSPECIFIED. ) 
 CURVE ( )  GEOMETRIC_REPRESENTATION_ITEM ( )  RATIONAL_B_SPLINE_CURVE ( ( 0.9330127018922194093, 0.9330127018922194093, 1.000000000000000000, 0.8660254037844387076, 1.000000000000000000, 0.8660254037844387076, 1.000000000000000000, 0.9330127018922194093, 0.9330127018922194093 ) ) 
 REPRESENTATION_ITEM ( '' )  );
#12839=CARTESIAN_POINT ( 'NONE',  ( 4.458734125000000326, 9.854166668032261711, 2.574251347313718519 ) ) ;
#12841=CARTESIAN_POINT ( 'NONE',  ( -6.972266317189433020E-16, -5.249999999999998224, -5.000000000000000000 ) ) ;
#12843=CARTESIAN_POINT ( 'NONE',  ( 5.000000000000000000, -89.50000000000000000, -6.123233995736766282E-16 ) ) ;
#12844=CARTESIAN_POINT ( 'NONE',  ( -2.229367062500000163, -26.47916666530106866, -3.861377020970580443 ) ) ;
#12845=AXIS2_PLACEMENT_3D ( 'NONE', #11581, #26380, #45998 ) ;
#12847=CARTESIAN_POINT ( 'NONE',  ( -4.458734124999998549, -73.47916666530106511, 2.574251347313722516 ) ) ;
#12848=EDGE_CURVE ( 'NONE', #23690, #14367, #16527, .T. ) ;
#12850=CARTESIAN_POINT ( 'NONE',  ( 5.000000000000000000, -79.37499999726881583, -6.123233995736766282E-16 ) ) ;
#12852=CARTESIAN_POINT ( 'NONE',  ( -4.458734124999999437, 4.604166668032261711, -2.574251347313719407 ) ) ;
#12854=CARTESIAN_POINT ( 'NONE',  ( -6.972266317189433020E-16, 5.875000002731185056, -5.000000000000000000 ) ) ;
#12856=CARTESIAN_POINT ( 'NONE',  ( -3.152548672688508926E-16, -70.56249999863439371, -5.148502694627439702 ) ) ;
#12858=CARTESIAN_POINT ( 'NONE',  ( -5.000000000000000000, -3.083333333333333925, -2.886751345948128211 ) ) ;
#12861=CARTESIAN_POINT ( 'NONE',  ( -4.458734124999998549, -62.22916666530106511, 2.574251347313722516 ) ) ;
#12862=CARTESIAN_POINT ( 'NONE',  ( -2.499999999999996447, -100.7083333306021444, 4.330127018922195425 ) ) ;
#12866=CARTESIAN_POINT ( 'NONE',  ( -2.229367062499996610, -108.3958333319677365, 3.861377020970582219 ) ) ;
#12868=CARTESIAN_POINT ( 'NONE',  ( 5.000000000000000000, -49.50000000000000000, -6.123233995736766282E-16 ) ) ;
#12869=CARTESIAN_POINT ( 'NONE',  ( -5.926426369611017623E-15, 27.24999999999999645, 5.000000000000000000 ) ) ;
#12870=CARTESIAN_POINT ( 'NONE',  ( 1.975475456537005874E-15, 19.25000000000000000, 5.000000000000000000 ) ) ;
#12877=CARTESIAN_POINT ( 'NONE',  ( -2.499999999999996447, -4.708333330602147981, 4.330127018922195425 ) ) ;
#12881=CARTESIAN_POINT ( 'NONE',  ( -6.972266317189433020E-16, -51.12499999726880873, -5.000000000000000000 ) ) ;
#12883=EDGE_LOOP ( 'NONE', ( #55054, #13920, #38222, #31232, #47827, #5477 ) ) ;
#12887=CARTESIAN_POINT ( 'NONE',  ( -3.152548672688508926E-16, -37.81249999863440792, -5.148502694627439702 ) ) ;
#12894=CARTESIAN_POINT ( 'NONE',  ( 4.458734124999998549, -83.97916666530107932, -2.574251347313721627 ) ) ;
#12900=CARTESIAN_POINT ( 'NONE',  ( 9.457646018065525792E-16, -9.312499998634406140, 5.148502694627439702 ) ) ;
#12905=CARTESIAN_POINT ( 'NONE',  ( -2.229367062500000163, -5.729166665301072214, -3.861377020970580443 ) ) ;
#12906=CARTESIAN_POINT ( 'NONE',  ( 0.000000000000000000, -120.0000000000000000, 0.000000000000000000 ) ) ;
#12908=FACE_OUTER_BOUND ( 'NONE', #25947, .T. ) ;
#12910=CARTESIAN_POINT ( 'NONE',  ( 4.458734125000000326, 25.85416666803225993, 2.574251347313718519 ) ) ;
#12911=ORIENTED_EDGE ( 'NONE', *, *, #57098, .F. ) ;
#12912=CARTESIAN_POINT ( 'NONE',  ( 2.229367062500001939, -88.97916666530106511, 3.861377020970579999 ) ) ;
#12914=CARTESIAN_POINT ( 'NONE',  ( -4.458734124999999437, -6.312499998634403475, 0.000000000000000000 ) ) ;
#12916=CARTESIAN_POINT ( 'NONE',  ( 6.123233995736766282E-16, -120.0000000000000000, -5.000000000000000000 ) ) ;
#12918=( BOUNDED_CURVE ( )  B_SPLINE_CURVE ( 2, ( #41580, #55766, #16202, #50617, #21675, #12003, #12335, #30677, #36145 ),
 .UNSPECIFIED., .F., .F. ) 
 B_SPLINE_CURVE_WITH_KNOTS ( ( 3, 2, 2, 2, 3 ),
 ( 0.2232142857142857262, 0.2238095238095238193, 0.2250000000000000056, 0.2261904761904761918, 0.2267857142857142849 ),
 .UNSPECIFIED. ) 
 CURVE ( )  GEOMETRIC_REPRESENTATION_ITEM ( )  RATIONAL_B_SPLINE_CURVE ( ( 0.9330127018922194093, 0.9330127018922209636, 1.000000000000000000, 0.8660254037844387076, 1.000000000000000000, 0.8660254037844387076, 1.000000000000000000, 0.9330127018922194093, 0.9330127018922194093 ) ) 
 REPRESENTATION_ITEM ( '' )  );
#12919=CARTESIAN_POINT ( 'NONE',  ( 1.975475456537005874E-15, -13.75000000000000000, 5.000000000000000000 ) ) ;
#12920=CARTESIAN_POINT ( 'NONE',  ( -4.999999999999999112, -35.79166666393548013, 2.886751345948131764 ) ) ;
#12922=CARTESIAN_POINT ( 'NONE',  ( -2.229367062500000163, 26.52083333469892779, -3.861377020970580443 ) ) ;
#12923=CARTESIAN_POINT ( 'NONE',  ( -2.499999999999996447, -3.833333333333334370, 4.330127018922195425 ) ) ;
#12925=CARTESIAN_POINT ( 'NONE',  ( 2.229367062499998831, -54.64583333196773651, -3.861377020970580887 ) ) ;
#12928=CARTESIAN_POINT ( 'NONE',  ( 2.499999999999998668, 14.66666666666666607, -4.330127018922193649 ) ) ;
#12932=CARTESIAN_POINT ( 'NONE',  ( 4.458734124999999437, -49.81249999863440792, -5.460374474430324690E-16 ) ) ;
#12933=CARTESIAN_POINT ( 'NONE',  ( 5.000000000000000000, -85.29166666393547303, -2.886751345948129988 ) ) ;
#12936=( BOUNDED_CURVE ( )  B_SPLINE_CURVE ( 2, ( #28378, #62807, #3951, #43168, #14525, #33838, #18726, #57977, #28997 ),
 .UNSPECIFIED., .F., .F. ) 
 B_SPLINE_CURVE_WITH_KNOTS ( ( 3, 2, 2, 2, 3 ),
 ( 0.3517857142857143127, 0.3523809523809524058, 0.3535714285714285920, 0.3547619047619047783, 0.3553571428571428714 ),
 .UNSPECIFIED. ) 
 CURVE ( )  GEOMETRIC_REPRESENTATION_ITEM ( )  RATIONAL_B_SPLINE_CURVE ( ( 0.9330127018922194093, 0.9330127018922225179, 1.000000000000000000, 0.8660254037844387076, 1.000000000000000000, 0.8660254037844387076, 1.000000000000000000, 0.9330127018922194093, 0.9330127018922194093 ) ) 
 REPRESENTATION_ITEM ( '' )  );
#12939=CARTESIAN_POINT ( 'NONE',  ( 4.458734124999998549, -84.97916666530107932, -2.574251347313721627 ) ) ;
#12941=CARTESIAN_POINT ( 'NONE',  ( -3.535250795749689387E-16, -32.25000000000000000, -5.773502691896257311 ) ) ;
#12942=ORIENTED_EDGE ( 'NONE', *, *, #60235, .T. ) ;
#12944=ORIENTED_EDGE ( 'NONE', *, *, #53033, .T. ) ;
#12945=CARTESIAN_POINT ( 'NONE',  ( -4.458734124999999437, -98.31249999863440792, 0.000000000000000000 ) ) ;
#12946=CARTESIAN_POINT ( 'NONE',  ( 2.229367062500001939, 7.770833334698926009, 3.861377020970579999 ) ) ;
#12947=CARTESIAN_POINT ( 'NONE',  ( -4.999999999999999112, 13.20833333606451809, 2.886751345948131764 ) ) ;
#12953=CARTESIAN_POINT ( 'NONE',  ( 5.000000000000000888, -79.58333333333331439, 2.886751345948126879 ) ) ;
#12955=CARTESIAN_POINT ( 'NONE',  ( -6.972266317189433020E-16, -55.12499999726880873, -5.000000000000000000 ) ) ;
#12960=CARTESIAN_POINT ( 'NONE',  ( 4.458734125000001214, -22.14583333196773296, 2.574251347313718519 ) ) ;
#12968=ORIENTED_EDGE ( 'NONE', *, *, #26823, .T. ) ;
#12970=DIRECTION ( 'NONE',  ( -0.000000000000000000, 1.000000000000000000, -0.000000000000000000 ) ) ;
#12971=ORIENTED_EDGE ( 'NONE', *, *, #3927, .F. ) ;
#12972=CARTESIAN_POINT ( 'NONE',  ( 2.229367062500001939, -65.22916666530106511, 3.861377020970579999 ) ) ;
#12974=CARTESIAN_POINT ( 'NONE',  ( -2.499999999999996447, -5.708333330602148870, 4.330127018922195425 ) ) ;
#12980=VERTEX_POINT ( 'NONE', #27755 ) ;
#12981=CARTESIAN_POINT ( 'NONE',  ( 1.339745962155615144, -45.70534180126146850, 4.999999999999999112 ) ) ;
#12982=CARTESIAN_POINT ( 'NONE',  ( -4.458734124999998549, 9.770833334698927786, 2.574251347313722516 ) ) ;
#12986=DIRECTION ( 'NONE',  ( -0.000000000000000000, 1.000000000000000000, -0.000000000000000000 ) ) ;
#12990=CARTESIAN_POINT ( 'NONE',  ( 4.458734124999998549, -71.72916666530107932, -2.574251347313721627 ) ) ;
#12991=CARTESIAN_POINT ( 'NONE',  ( -6.972266317189433020E-16, -10.12499999726881406, -5.000000000000000000 ) ) ;
#12992=CARTESIAN_POINT ( 'NONE',  ( -2.229367062499996610, 5.854166668032262599, 3.861377020970582219 ) ) ;
#12994=VECTOR ( 'NONE', #11719, 1000.000000000000000 ) ;
#12998=CARTESIAN_POINT ( 'NONE',  ( 4.458734124999998549, -61.97916666530106511, -2.574251347313721627 ) ) ;
#12999=CARTESIAN_POINT ( 'NONE',  ( 5.000000000000000000, -19.37499999726881583, -6.123233995736766282E-16 ) ) ;
#13004=CARTESIAN_POINT ( 'NONE',  ( -2.229367062499996610, -38.14583333196773651, 3.861377020970582219 ) ) ;
#13005=CARTESIAN_POINT ( 'NONE',  ( -4.458734124999999437, -20.64583333196774007, -2.574251347313719407 ) ) ;
#13006=ORIENTED_EDGE ( 'NONE', *, *, #18045, .F. ) ;
#13007=CARTESIAN_POINT ( 'NONE',  ( 0.000000000000000000, -120.0000000000000000, 5.000000000000000000 ) ) ;
#13008=CARTESIAN_POINT ( 'NONE',  ( -2.229367062500000163, -107.4791666653010651, -3.861377020970580443 ) ) ;
#13011=CARTESIAN_POINT ( 'NONE',  ( -4.458734124999999437, -106.6458333319677365, -2.574251347313719407 ) ) ;
#13012=CARTESIAN_POINT ( 'NONE',  ( 4.458734125000001214, -31.89583333196773651, 2.574251347313718519 ) ) ;
#13013=CARTESIAN_POINT ( 'NONE',  ( -2.499999999999996447, -67.70833333060214443, 4.330127018922195425 ) ) ;
#13014=EDGE_CURVE ( 'NONE', #50926, #17569, #12423, .T. ) ;
#13017=CARTESIAN_POINT ( 'NONE',  ( -4.458734124999999437, -28.39583333196773651, -2.574251347313719407 ) ) ;
#13018=EDGE_CURVE ( 'NONE', #62985, #27288, #18981, .T. ) ;
#13019=CARTESIAN_POINT ( 'NONE',  ( -2.229367062500000163, -70.72916666530107932, -3.861377020970580443 ) ) ;
#13022=CARTESIAN_POINT ( 'NONE',  ( 5.000000000000000888, -32.58333333333333570, 2.886751345948126879 ) ) ;
#13023=CYLINDRICAL_SURFACE ( 'NONE', #54407, 5.000000000000000000 ) ;
#13024=CARTESIAN_POINT ( 'NONE',  ( -3.535250795749689387E-16, -15.25000000000000000, -5.773502691896257311 ) ) ;
#13026=ORIENTED_EDGE ( 'NONE', *, *, #7928, .T. ) ;
#13027=DIRECTION ( 'NONE',  ( -0.000000000000000000, 1.000000000000000000, -0.000000000000000000 ) ) ;
#13029=( BOUNDED_CURVE ( )  B_SPLINE_CURVE ( 2, ( #34819, #23900, #29328, #48958, #102, #29979, #5547, #33862, #49291 ),
 .UNSPECIFIED., .F., .F. ) 
 B_SPLINE_CURVE_WITH_KNOTS ( ( 3, 2, 2, 2, 3 ),
 ( 0.3553571428571428714, 0.3559523809523809645, 0.3571428571428571508, 0.3583333333333333370, 0.3589285714285714302 ),
 .UNSPECIFIED. ) 
 CURVE ( )  GEOMETRIC_REPRESENTATION_ITEM ( )  RATIONAL_B_SPLINE_CURVE ( ( 0.9330127018922194093, 0.9330127018922194093, 1.000000000000000000, 0.8660254037844387076, 1.000000000000000000, 0.8660254037844387076, 1.000000000000000000, 0.9330127018922194093, 0.9330127018922194093 ) ) 
 REPRESENTATION_ITEM ( '' )  );
#13035=CARTESIAN_POINT ( 'NONE',  ( -1.339745962155610925, -51.66965819600733312, 5.000000000000000000 ) ) ;
#13036=DIRECTION ( 'NONE',  ( -0.000000000000000000, 1.000000000000000000, -0.000000000000000000 ) ) ;
#13040=DIRECTION ( 'NONE',  ( -0.000000000000000000, 1.000000000000000000, -0.000000000000000000 ) ) ;
#13046=AXIS2_PLACEMENT_3D ( 'NONE', #50784, #30515, #20568 ) ;
#13047=VECTOR ( 'NONE', #51147, 1000.000000000000000 ) ;
#13052=CARTESIAN_POINT ( 'NONE',  ( -2.500000000000000444, -103.0416666639354730, -4.330127018922193649 ) ) ;
#13054=FACE_OUTER_BOUND ( 'NONE', #31653, .T. ) ;
#13057=CARTESIAN_POINT ( 'NONE',  ( -5.000000000000000000, 23.12500000273118417, 0.000000000000000000 ) ) ;
#13058=ORIENTED_EDGE ( 'NONE', *, *, #32793, .T. ) ;
#13059=CARTESIAN_POINT ( 'NONE',  ( 4.458734124999999437, -80.81249999863440792, -5.460374474430324690E-16 ) ) ;
#13060=CARTESIAN_POINT ( 'NONE',  ( 4.458734125000001214, 26.10416666803225993, 2.574251347313718519 ) ) ;
#13067=CARTESIAN_POINT ( 'NONE',  ( -6.972266317189433020E-16, 0.8750000027311866102, -5.000000000000000000 ) ) ;
#13069=CARTESIAN_POINT ( 'NONE',  ( 5.000000000000000000, -13.37499999726881050, -6.123233995736766282E-16 ) ) ;
#13070=CARTESIAN_POINT ( 'NONE',  ( 2.229367062499998831, -55.64583333196773651, -3.861377020970580887 ) ) ;
#13071=CARTESIAN_POINT ( 'NONE',  ( 5.000000000000000000, 21.50000000000000000, -6.123233995736766282E-16 ) ) ;
#13072=CARTESIAN_POINT ( 'NONE',  ( 9.457646018065525792E-16, 21.93750000136559208, 5.148502694627439702 ) ) ;
#13073=CARTESIAN_POINT ( 'NONE',  ( 5.000000000000000000, -105.5000000000000142, -6.123233995736766282E-16 ) ) ;
#13074=CARTESIAN_POINT ( 'NONE',  ( -2.499999999999996447, -43.83333333333333570, 4.330127018922195425 ) ) ;
#13076=CARTESIAN_POINT ( 'NONE',  ( 4.458734125000001214, -46.14583333196773651, 2.574251347313718519 ) ) ;
#13077=CARTESIAN_POINT ( 'NONE',  ( 1.060575238724906964E-15, -5.624999997268811391, 5.773502691896257311 ) ) ;
#13081=CARTESIAN_POINT ( 'NONE',  ( 4.458734125000000326, -100.8958333319677365, 2.574251347313718519 ) ) ;
#13082=CARTESIAN_POINT ( 'NONE',  ( 9.457646018065525792E-16, -6.312499998634403475, 5.148502694627439702 ) ) ;
#13085=CARTESIAN_POINT ( 'NONE',  ( -5.000000000000000000, -85.87499999726880162, 0.000000000000000000 ) ) ;
#13086=CARTESIAN_POINT ( 'NONE',  ( -2.229367062499996610, -93.14583333196773651, 3.861377020970582219 ) ) ;
#13088=CARTESIAN_POINT ( 'NONE',  ( -2.229367062499996610, -91.39583333196773651, 3.861377020970582219 ) ) ;
#13091=AXIS2_PLACEMENT_3D ( 'NONE', #11962, #51224, #7161 ) ;
#13094=CARTESIAN_POINT ( 'NONE',  ( 9.457646018065525792E-16, -13.06249999863440259, 5.148502694627439702 ) ) ;
#13095=CARTESIAN_POINT ( 'NONE',  ( -4.458734124999999437, 12.35416666803225993, -2.574251347313719407 ) ) ;
#13096=CARTESIAN_POINT ( 'NONE',  ( -2.229367062500000163, -52.72916666530107221, -3.861377020970580443 ) ) ;
#13097=DIRECTION ( 'NONE',  ( 0.000000000000000000, 0.000000000000000000, 1.000000000000000000 ) ) ;
#13098=CARTESIAN_POINT ( 'NONE',  ( 1.975475456537005874E-15, -105.7500000000000000, 5.000000000000000000 ) ) ;
#13101=EDGE_CURVE ( 'NONE', #11403, #47219, #24189, .T. ) ;
#13108=CARTESIAN_POINT ( 'NONE',  ( -3.152548672688508926E-16, -80.56249999863440792, -5.148502694627439702 ) ) ;
#13109=CARTESIAN_POINT ( 'NONE',  ( 2.229367062500001939, 21.77083333469892779, 3.861377020970579999 ) ) ;
#13111=EDGE_CURVE ( 'NONE', #26645, #11325, #18423, .T. ) ;
#13112=CARTESIAN_POINT ( 'NONE',  ( -6.972266317189433020E-16, 6.750000000000000000, -5.000000000000000000 ) ) ;
#13114=CARTESIAN_POINT ( 'NONE',  ( -5.000000000000000000, -71.08333333333332860, -2.886751345948128211 ) ) ;
#13119=CARTESIAN_POINT ( 'NONE',  ( -1.339745962155610925, -89.79465819873851729, 5.000000000000000000 ) ) ;
#13120=CARTESIAN_POINT ( 'NONE',  ( 1.975475456537005874E-15, -50.75000000000000000, 5.000000000000000000 ) ) ;
#13123=( BOUNDED_CURVE ( )  B_SPLINE_CURVE ( 2, ( #58347, #48372, #14582, #4618, #4011, #43226, #29054, #23934, #13958 ),
 .UNSPECIFIED., .F., .F. ) 
 B_SPLINE_CURVE_WITH_KNOTS ( ( 3, 2, 2, 2, 3 ),
 ( 0.4053571428571428603, 0.4059523809523809534, 0.4071428571428571397, 0.4083333333333333259, 0.4089285714285714191 ),
 .UNSPECIFIED. ) 
 CURVE ( )  GEOMETRIC_REPRESENTATION_ITEM ( )  RATIONAL_B_SPLINE_CURVE ( ( 0.9330127018922194093, 0.9330127018922194093, 1.000000000000000000, 0.8660254037844387076, 1.000000000000000000, 0.8660254037844387076, 1.000000000000000000, 0.9330127018922194093, 0.9330127018922194093 ) ) 
 REPRESENTATION_ITEM ( '' )  );
#13132=CARTESIAN_POINT ( 'NONE',  ( 2.229367062499998831, -52.89583333196773651, -3.861377020970580887 ) ) ;
#13135=CARTESIAN_POINT ( 'NONE',  ( 1.975475456537005874E-15, 10.37500000273118417, 5.000000000000000000 ) ) ;
#13143=CARTESIAN_POINT ( 'NONE',  ( -4.458734124999998549, -102.4791666653010509, 2.574251347313722516 ) ) ;
#13148=CARTESIAN_POINT ( 'NONE',  ( 4.458734125000001214, -8.895833331967736513, 2.574251347313718519 ) ) ;
#13149=CARTESIAN_POINT ( 'NONE',  ( 2.229367062499998831, -96.89583333196773651, -3.861377020970580887 ) ) ;
#13151=CARTESIAN_POINT ( 'NONE',  ( -4.458734124999998549, -29.47916666530106866, 2.574251347313722516 ) ) ;
#13152=CARTESIAN_POINT ( 'NONE',  ( 1.975475456537005874E-15, -66.74999999999998579, 5.000000000000000000 ) ) ;
#13155=CARTESIAN_POINT ( 'NONE',  ( 2.500000000000002220, -21.54166666393548013, 4.330127018922192761 ) ) ;
#13156=CARTESIAN_POINT ( 'NONE',  ( -2.500000000000000444, -34.16666666666666430, -4.330127018922193649 ) ) ;
#13158=CARTESIAN_POINT ( 'NONE',  ( 4.458734124999998549, 11.02083333469892956, -2.574251347313721627 ) ) ;
#13162=CARTESIAN_POINT ( 'NONE',  ( -3.535250795749689387E-16, -93.24999999999998579, -5.773502691896257311 ) ) ;
#13163=CARTESIAN_POINT ( 'NONE',  ( 4.458734124999999437, -22.81249999863440436, -5.460374474430324690E-16 ) ) ;
#13164=CARTESIAN_POINT ( 'NONE',  ( -1.339745962155610925, 7.330341803992665994, 5.000000000000000000 ) ) ;
#13165=CARTESIAN_POINT ( 'NONE',  ( 9.457646018065525792E-16, -77.31249999863440792, 5.148502694627439702 ) ) ;
#13169=CARTESIAN_POINT ( 'NONE',  ( -4.458734124999997661, 4.770833334698926009, 2.574251347313722516 ) ) ;
#13170=CARTESIAN_POINT ( 'NONE',  ( -1.339745962155610925, -62.66965819600734022, 5.000000000000000000 ) ) ;
#13171=( BOUNDED_CURVE ( )  B_SPLINE_CURVE ( 2, ( #480, #53232, #59326, #43874, #19117, #38736, #9471, #19444, #43251 ),
 .UNSPECIFIED., .F., .F. ) 
 B_SPLINE_CURVE_WITH_KNOTS ( ( 3, 2, 2, 2, 3 ),
 ( 0.8375000000000000222, 0.8380952380952381153, 0.8392857142857143016, 0.8404761904761904878, 0.8410714285714285809 ),
 .UNSPECIFIED. ) 
 CURVE ( )  GEOMETRIC_REPRESENTATION_ITEM ( )  RATIONAL_B_SPLINE_CURVE ( ( 0.9330127018922194093, 0.9330127018922194093, 1.000000000000000000, 0.8660254037844387076, 1.000000000000000000, 0.8660254037844387076, 1.000000000000000000, 0.9330127018922194093, 0.9330127018922194093 ) ) 
 REPRESENTATION_ITEM ( '' )  );
#13174=CARTESIAN_POINT ( 'NONE',  ( 2.229367062499998831, -72.64583333196773651, -3.861377020970580887 ) ) ;
#13177=AXIS2_PLACEMENT_3D ( 'NONE', #19893, #951, #34363 ) ;
#13178=CARTESIAN_POINT ( 'NONE',  ( 5.000000000000000888, -3.583333333333333925, 2.886751345948126879 ) ) ;
#13181=CARTESIAN_POINT ( 'NONE',  ( -2.229367062500000163, -61.47916666530106511, -3.861377020970580443 ) ) ;
#13182=CARTESIAN_POINT ( 'NONE',  ( -4.999999999999999112, -100.7916666639354730, 2.886751345948131764 ) ) ;
#13184=CYLINDRICAL_SURFACE ( 'NONE', #19450, 5.000000000000000000 ) ;
#13185=CARTESIAN_POINT ( 'NONE',  ( 4.458734125000000326, -106.1458333319677365, 2.574251347313718519 ) ) ;
#13187=CARTESIAN_POINT ( 'NONE',  ( 5.000000000000000000, -55.41666666666667140, -2.886751345948129988 ) ) ;
#13196=CIRCLE ( 'NONE', #52229, 5.000000000000000000 ) ;
#13200=ORIENTED_EDGE ( 'NONE', *, *, #39783, .F. ) ;
#13201=CARTESIAN_POINT ( 'NONE',  ( 1.975475456537005874E-15, -81.74999999999998579, 5.000000000000000000 ) ) ;
#13207=CARTESIAN_POINT ( 'NONE',  ( 4.458734125000001214, -36.14583333196773651, 2.574251347313718519 ) ) ;
#13208=CARTESIAN_POINT ( 'NONE',  ( 1.339745962155615144, -10.70534180126147916, 4.999999999999999112 ) ) ;
#13215=CARTESIAN_POINT ( 'NONE',  ( -6.972266317189433020E-16, -26.25000000000000000, -5.000000000000000000 ) ) ;
#13216=CARTESIAN_POINT ( 'NONE',  ( 2.229367062500001939, -81.22916666530106511, 3.861377020970579999 ) ) ;
#13219=AXIS2_PLACEMENT_3D ( 'NONE', #53763, #3948, #24184 ) ;
#13223=AXIS2_PLACEMENT_3D ( 'NONE', #24592, #18806, #48707 ) ;
#13227=CARTESIAN_POINT ( 'NONE',  ( -2.229367062499996610, -11.39583333196773829, 3.861377020970582219 ) ) ;
#13228=CARTESIAN_POINT ( 'NONE',  ( 0.000000000000000000, -120.0000000000000000, 0.000000000000000000 ) ) ;
#13230=CARTESIAN_POINT ( 'NONE',  ( 1.339745962155612702, -77.16965819600731891, -5.000000000000000000 ) ) ;
#13232=CARTESIAN_POINT ( 'NONE',  ( -4.458734124999997661, 27.52083333469892779, 2.574251347313722516 ) ) ;
#13233=ORIENTED_EDGE ( 'NONE', *, *, #55161, .T. ) ;
#13234=CARTESIAN_POINT ( 'NONE',  ( 2.229367062499998831, -91.64583333196773651, -3.861377020970580887 ) ) ;
#13236=CARTESIAN_POINT ( 'NONE',  ( -2.499999999999996447, -62.83333333333333570, 4.330127018922195425 ) ) ;
#13237=CARTESIAN_POINT ( 'NONE',  ( 4.458734124999998549, -6.729166665301073103, -2.574251347313721627 ) ) ;
#13240=DIRECTION ( 'NONE',  ( 0.5000000000000069944, 0.000000000000000000, 0.8660254037844345998 ) ) ;
#13241=CARTESIAN_POINT ( 'NONE',  ( 5.000000000000000888, -35.45833333060213732, 2.886751345948126879 ) ) ;
#13242=CARTESIAN_POINT ( 'NONE',  ( 1.339745962155615144, -49.58034179853029144, 4.999999999999999112 ) ) ;
#13243=CARTESIAN_POINT ( 'NONE',  ( 9.457646018065525792E-16, 16.93750000136559564, 5.148502694627439702 ) ) ;
#13244=CARTESIAN_POINT ( 'NONE',  ( -1.339745962155610925, -20.66965819600733312, 5.000000000000000000 ) ) ;
#13246=CARTESIAN_POINT ( 'NONE',  ( -3.152548672688508926E-16, -58.56249999863440081, -5.148502694627439702 ) ) ;
#13248=FACE_OUTER_BOUND ( 'NONE', #16693, .T. ) ;
#13249=CARTESIAN_POINT ( 'NONE',  ( -3.535250795749689387E-16, 9.749999999999998224, -5.773502691896257311 ) ) ;
#13251=CARTESIAN_POINT ( 'NONE',  ( -4.999999999999998224, -45.91666666666665719, 2.886751345948131764 ) ) ;
#13252=CARTESIAN_POINT ( 'NONE',  ( 2.229367062499998831, -48.64583333196772941, -3.861377020970580887 ) ) ;
#13253=CARTESIAN_POINT ( 'NONE',  ( -5.000000000000000000, -85.95833333060213022, -2.886751345948128211 ) ) ;
#13257=CARTESIAN_POINT ( 'NONE',  ( 4.458734124999998549, -91.97916666530106511, -2.574251347313721627 ) ) ;
#13259=CARTESIAN_POINT ( 'NONE',  ( 2.500000000000002220, -32.66666666666666430, 4.330127018922192761 ) ) ;
#13261=ORIENTED_EDGE ( 'NONE', *, *, #55500, .F. ) ;
#13263=ORIENTED_EDGE ( 'NONE', *, *, #11469, .T. ) ;
#13264=CARTESIAN_POINT ( 'NONE',  ( 2.229367062499998831, -95.64583333196773651, -3.861377020970580887 ) ) ;
#13265=CARTESIAN_POINT ( 'NONE',  ( 4.458734125000001214, 10.85416666803225993, 2.574251347313718519 ) ) ;
#13267=CARTESIAN_POINT ( 'NONE',  ( 2.499999999999998668, 11.79166666939785202, -4.330127018922193649 ) ) ;
#13268=CARTESIAN_POINT ( 'NONE',  ( -5.000000000000000000, -43.87499999726880873, 0.000000000000000000 ) ) ;
#13270=VECTOR ( 'NONE', #52468, 1000.000000000000000 ) ;
#13273=CARTESIAN_POINT ( 'NONE',  ( -4.999999999999999112, -80.91666666666667140, 2.886751345948131764 ) ) ;
#13275=DIRECTION ( 'NONE',  ( -0.000000000000000000, 1.000000000000000000, -0.000000000000000000 ) ) ;
#13277=DIRECTION ( 'NONE',  ( -0.000000000000000000, 1.000000000000000000, -0.000000000000000000 ) ) ;
#13280=CARTESIAN_POINT ( 'NONE',  ( -6.972266317189433020E-16, -90.12499999726880162, -5.000000000000000000 ) ) ;
#13281=CARTESIAN_POINT ( 'NONE',  ( -4.458734124999998549, -21.47916666530107221, 2.574251347313722516 ) ) ;
#13282=CARTESIAN_POINT ( 'NONE',  ( 1.975475456537005874E-15, -57.74999999999999289, 5.000000000000000000 ) ) ;
#13286=EDGE_CURVE ( 'NONE', #14049, #51281, #53461, .T. ) ;
#13293=CARTESIAN_POINT ( 'NONE',  ( -3.152548672688508926E-16, -67.81249999863440792, -5.148502694627439702 ) ) ;
#13295=CARTESIAN_POINT ( 'NONE',  ( -6.972266317189433020E-16, -91.24999999999998579, -5.000000000000000000 ) ) ;
#13296=ORIENTED_EDGE ( 'NONE', *, *, #45205, .T. ) ;
#13297=CARTESIAN_POINT ( 'NONE',  ( 0.000000000000000000, -120.0000000000000000, 0.000000000000000000 ) ) ;
#13303=CARTESIAN_POINT ( 'NONE',  ( -5.000000000000000000, 2.125000002731185056, 0.000000000000000000 ) ) ;
#13304=EDGE_CURVE ( 'NONE', #28142, #17776, #5846, .T. ) ;
#13305=CARTESIAN_POINT ( 'NONE',  ( -4.458734124999998549, 4.770833334698926009, 2.574251347313722516 ) ) ;
#13310=PRODUCT_DEFINITION_FORMATION_WITH_SPECIFIED_SOURCE ( 'ANY', '', #5039, .NOT_KNOWN. ) ;
#13311=ORIENTED_EDGE ( 'NONE', *, *, #19764, .T. ) ;
#13312=CARTESIAN_POINT ( 'NONE',  ( 4.458734124999998549, -73.72916666530106511, -2.574251347313721627 ) ) ;
#13314=CARTESIAN_POINT ( 'NONE',  ( 9.457646018065525792E-16, 4.937500001365596525, 5.148502694627439702 ) ) ;
#13317=CARTESIAN_POINT ( 'NONE',  ( 4.458734124999998549, -60.97916666530106511, -2.574251347313721627 ) ) ;
#13318=CARTESIAN_POINT ( 'NONE',  ( -5.000000000000000000, -17.87499999726881583, 0.000000000000000000 ) ) ;
#13319=CARTESIAN_POINT ( 'NONE',  ( -6.972266317189433020E-16, -100.2499999999999858, -5.000000000000000000 ) ) ;
#13324=CARTESIAN_POINT ( 'NONE',  ( 2.229367062499998831, -38.64583333196773651, -3.861377020970580887 ) ) ;
#13325=CARTESIAN_POINT ( 'NONE',  ( -2.229367062500000163, -25.72916666530106866, -3.861377020970580443 ) ) ;
#13327=CARTESIAN_POINT ( 'NONE',  ( -2.229367062499996610, -109.1458333319677365, 3.861377020970582219 ) ) ;
#13329=ORIENTED_EDGE ( 'NONE', *, *, #37350, .T. ) ;
#13330=CARTESIAN_POINT ( 'NONE',  ( 2.229367062500001939, -107.2291666653010651, 3.861377020970579999 ) ) ;
#13331=CARTESIAN_POINT ( 'NONE',  ( 4.458734124999998549, -30.72916666530107221, -2.574251347313721627 ) ) ;
#13332=CARTESIAN_POINT ( 'NONE',  ( -2.500000000000000444, -70.04166666393547303, -4.330127018922193649 ) ) ;
#13336=CARTESIAN_POINT ( 'NONE',  ( 9.457646018065525792E-16, -27.06249999863440081, 5.148502694627439702 ) ) ;
#13337=CARTESIAN_POINT ( 'NONE',  ( -4.458734124999999437, -71.56249999863439371, 0.000000000000000000 ) ) ;
#13342=CARTESIAN_POINT ( 'NONE',  ( -5.000000000000000000, -18.00000000000000355, 0.000000000000000000 ) ) ;
#13345=DIRECTION ( 'NONE',  ( -0.000000000000000000, 1.000000000000000000, -0.000000000000000000 ) ) ;
#13347=CARTESIAN_POINT ( 'NONE',  ( 2.499999999999998668, 27.79166666939785202, -4.330127018922193649 ) ) ;
#13350=CARTESIAN_POINT ( 'NONE',  ( -4.999999999999998224, 8.208333336064518093, 2.886751345948131764 ) ) ;
#13353=CARTESIAN_POINT ( 'NONE',  ( 6.123233995736766282E-16, -120.0000000000000000, -5.000000000000000000 ) ) ;
#13355=VERTEX_POINT ( 'NONE', #5209 ) ;
#13357=ORIENTED_EDGE ( 'NONE', *, *, #14246, .F. ) ;
#13362=EDGE_CURVE ( 'NONE', #60689, #28617, #45401, .T. ) ;
#13365=ORIENTED_EDGE ( 'NONE', *, *, #12119, .T. ) ;
#13368=CARTESIAN_POINT ( 'NONE',  ( -6.972266317189433020E-16, -34.25000000000000000, -5.000000000000000000 ) ) ;
#13372=DIRECTION ( 'NONE',  ( -0.000000000000000000, 1.000000000000000000, -0.000000000000000000 ) ) ;
#13375=ORIENTED_EDGE ( 'NONE', *, *, #10174, .T. ) ;
#13376=CARTESIAN_POINT ( 'NONE',  ( -2.229367062499996610, -82.14583333196773651, 3.861377020970582219 ) ) ;
#13378=CARTESIAN_POINT ( 'NONE',  ( -2.229367062499996610, 22.85416666803225993, 3.861377020970582219 ) ) ;
#13379=CARTESIAN_POINT ( 'NONE',  ( 0.000000000000000000, -120.0000000000000000, 0.000000000000000000 ) ) ;
#13384=CYLINDRICAL_SURFACE ( 'NONE', #60349, 5.000000000000000000 ) ;
#13387=CARTESIAN_POINT ( 'NONE',  ( -2.229367062500000163, -56.47916666530107221, -3.861377020970580443 ) ) ;
#13389=CARTESIAN_POINT ( 'NONE',  ( 9.457646018065525792E-16, 23.93750000136559564, 5.148502694627439702 ) ) ;
#13391=CARTESIAN_POINT ( 'NONE',  ( -2.500000000000000444, -44.16666666666665719, -4.330127018922193649 ) ) ;
#13392=CARTESIAN_POINT ( 'NONE',  ( -4.458734124999998549, -43.47916666530106511, 2.574251347313722516 ) ) ;
#13393=CARTESIAN_POINT ( 'NONE',  ( -5.000000000000000000, -1.958333330602145761, -2.886751345948128211 ) ) ;
#13397=CARTESIAN_POINT ( 'NONE',  ( -4.458734124999997661, -104.2291666653010651, 2.574251347313722516 ) ) ;
#13398=AXIS2_PLACEMENT_3D ( 'NONE', #9805, #49046, #59024 ) ;
#13400=CARTESIAN_POINT ( 'NONE',  ( -2.229367062500000163, -8.729166665301073991, -3.861377020970580443 ) ) ;
#13401=ORIENTED_EDGE ( 'NONE', *, *, #51847, .T. ) ;
#13403=CARTESIAN_POINT ( 'NONE',  ( -2.229367062499996610, -94.14583333196772230, 3.861377020970582219 ) ) ;
#13405=CARTESIAN_POINT ( 'NONE',  ( 4.458734125000001214, -91.14583333196773651, 2.574251347313718519 ) ) ;
#13407=CARTESIAN_POINT ( 'NONE',  ( -2.499999999999996447, -52.70833333060213732, 4.330127018922195425 ) ) ;
#13410=CARTESIAN_POINT ( 'NONE',  ( 4.458734124999999437, -14.81249999863440436, -5.460374474430324690E-16 ) ) ;
#13411=CARTESIAN_POINT ( 'NONE',  ( -4.458734124999999437, 13.43750000136559386, 0.000000000000000000 ) ) ;
#13412=CARTESIAN_POINT ( 'NONE',  ( -2.229367062500000163, -53.72916666530107221, -3.861377020970580443 ) ) ;
#13420=FACE_OUTER_BOUND ( 'NONE', #37881, .T. ) ;
#13421=CARTESIAN_POINT ( 'NONE',  ( -4.458734124999999437, -79.31249999863440792, 0.000000000000000000 ) ) ;
#13422=CARTESIAN_POINT ( 'NONE',  ( -4.458734124999999437, 26.43750000136559564, 0.000000000000000000 ) ) ;
#13427=CARTESIAN_POINT ( 'NONE',  ( 1.060575238724906964E-15, -68.74999999999998579, 5.773502691896257311 ) ) ;
#13429=ORIENTED_EDGE ( 'NONE', *, *, #42575, .F. ) ;
#13430=CARTESIAN_POINT ( 'NONE',  ( -5.000000000000000000, -61.87499999726880873, 0.000000000000000000 ) ) ;
#13432=CARTESIAN_POINT ( 'NONE',  ( 6.123233995736766282E-16, -120.0000000000000000, -5.000000000000000000 ) ) ;
#13435=CYLINDRICAL_SURFACE ( 'NONE', #61263, 5.000000000000000000 ) ;
#13444=ADVANCED_FACE ( 'NONE', ( #5852 ), #45082, .T. ) ;
#13448=CARTESIAN_POINT ( 'NONE',  ( 9.457646018065525792E-16, -54.31249999863440081, 5.148502694627439702 ) ) ;
#13449=EDGE_CURVE ( 'NONE', #37904, #62889, #6173, .T. ) ;
#13451=CARTESIAN_POINT ( 'NONE',  ( -1.339745962155613812, -55.08034179853029144, -5.000000000000000000 ) ) ;
#13459=ORIENTED_EDGE ( 'NONE', *, *, #9786, .F. ) ;
#13462=CARTESIAN_POINT ( 'NONE',  ( 4.458734124999998549, -101.9791666653010651, -2.574251347313721627 ) ) ;
#13464=VERTEX_POINT ( 'NONE', #31236 ) ;
#13469=EDGE_CURVE ( 'NONE', #60305, #56096, #2944, .T. ) ;
#13470=CARTESIAN_POINT ( 'NONE',  ( 5.000000000000000000, -83.49999999999998579, -6.123233995736766282E-16 ) ) ;
#13471=CARTESIAN_POINT ( 'NONE',  ( 2.229367062500001939, -4.979166665301071326, 3.861377020970579999 ) ) ;
#13472=CARTESIAN_POINT ( 'NONE',  ( -3.152548672688508926E-16, -98.81249999863440792, -5.148502694627439702 ) ) ;
#13474=CARTESIAN_POINT ( 'NONE',  ( -4.458734124999999437, -27.64583333196774007, -2.574251347313719407 ) ) ;
#13478=CYLINDRICAL_SURFACE ( 'NONE', #54877, 5.000000000000000000 ) ;
#13479=LINE ( 'NONE', #27318, #22376 ) ;
#13481=CARTESIAN_POINT ( 'NONE',  ( 4.458734124999999437, 7.937500001365595637, -5.460374474430324690E-16 ) ) ;
#13482=ORIENTED_EDGE ( 'NONE', *, *, #9879, .T. ) ;
#13483=CARTESIAN_POINT ( 'NONE',  ( -1.339745962155610925, 2.205341801261479606, 5.000000000000000000 ) ) ;
#13485=CARTESIAN_POINT ( 'NONE',  ( -2.500000000000000444, -88.16666666666665719, -4.330127018922193649 ) ) ;
#13486=CARTESIAN_POINT ( 'NONE',  ( 9.457646018065525792E-16, -25.06249999863440792, 5.148502694627439702 ) ) ;
#13487=LINE ( 'NONE', #33104, #44906 ) ;
#13488=CARTESIAN_POINT ( 'NONE',  ( -4.458734124999998549, -74.47916666530106511, 2.574251347313722516 ) ) ;
#13493=CARTESIAN_POINT ( 'NONE',  ( -4.458734124999997661, 0.7708333346989268975, 2.574251347313722516 ) ) ;
#13494=CARTESIAN_POINT ( 'NONE',  ( -4.458734124999998549, 26.52083333469892779, 2.574251347313722516 ) ) ;
#13495=CARTESIAN_POINT ( 'NONE',  ( 9.457646018065525792E-16, -37.31249999863440792, 5.148502694627439702 ) ) ;
#13498=CARTESIAN_POINT ( 'NONE',  ( 4.458734124999999437, -71.81249999863439371, -5.460374474430324690E-16 ) ) ;
#13500=CARTESIAN_POINT ( 'NONE',  ( 2.499999999999998668, -5.333333333333335702, -4.330127018922193649 ) ) ;
#13503=AXIS2_PLACEMENT_3D ( 'NONE', #27677, #46355, #32502 ) ;
#13504=CARTESIAN_POINT ( 'NONE',  ( 4.458734124999999437, -65.81249999863440792, -5.460374474430324690E-16 ) ) ;
#13505=CARTESIAN_POINT ( 'NONE',  ( 1.060575238724906964E-15, -97.62499999726881583, 5.773502691896257311 ) ) ;
#13506=( BOUNDED_CURVE ( )  B_SPLINE_CURVE ( 2, ( #57497, #27260, #46886, #42362, #36592, #56228, #12149, #48134, #58102 ),
 .UNSPECIFIED., .F., .F. ) 
 B_SPLINE_CURVE_WITH_KNOTS ( ( 3, 2, 2, 2, 3 ),
 ( 0.9660714285714285809, 0.9666666666666666741, 0.9678571428571428603, 0.9690476190476190466, 0.9696428571428571397 ),
 .UNSPECIFIED. ) 
 CURVE ( )  GEOMETRIC_REPRESENTATION_ITEM ( )  RATIONAL_B_SPLINE_CURVE ( ( 0.9330127018922194093, 0.9330127018922194093, 1.000000000000000000, 0.8660254037844387076, 1.000000000000000000, 0.8660254037844387076, 1.000000000000000000, 0.9330127018922194093, 0.9330127018922194093 ) ) 
 REPRESENTATION_ITEM ( '' )  );
#13507=CARTESIAN_POINT ( 'NONE',  ( 2.500000000000002220, -41.66666666666667140, 4.330127018922192761 ) ) ;
#13509=CARTESIAN_POINT ( 'NONE',  ( -6.972266317189433020E-16, 9.875000002731185944, -5.000000000000000000 ) ) ;
#13510=CARTESIAN_POINT ( 'NONE',  ( 9.457646018065525792E-16, -104.3124999986344221, 5.148502694627439702 ) ) ;
#13512=CARTESIAN_POINT ( 'NONE',  ( 5.000000000000000000, -52.50000000000000711, -6.123233995736766282E-16 ) ) ;
#13513=CARTESIAN_POINT ( 'NONE',  ( 7.204675194429079505E-15, 26.74999999999999645, -5.000000000000000000 ) ) ;
#13514=CARTESIAN_POINT ( 'NONE',  ( 0.000000000000000000, -120.0000000000000000, 0.000000000000000000 ) ) ;
#13516=CARTESIAN_POINT ( 'NONE',  ( 5.000000000000000000, -94.41666666666664298, -2.886751345948130876 ) ) ;
#13517=AXIS2_PLACEMENT_3D ( 'NONE', #39302, #29655, #49285 ) ;
#13522=CYLINDRICAL_SURFACE ( 'NONE', #58581, 5.000000000000000000 ) ;
#13531=CARTESIAN_POINT ( 'NONE',  ( 9.457646018065525792E-16, -36.31249999863440792, 5.148502694627439702 ) ) ;
#13538=CARTESIAN_POINT ( 'NONE',  ( 5.000000000000000888, -54.58333333333332860, 2.886751345948126879 ) ) ;
#13540=CARTESIAN_POINT ( 'NONE',  ( -2.229367062500000163, -81.72916666530106511, -3.861377020970580443 ) ) ;
#13541=CARTESIAN_POINT ( 'NONE',  ( 0.000000000000000000, -120.0000000000000000, 5.000000000000000000 ) ) ;
#13542=EDGE_LOOP ( 'NONE', ( #5462, #22549, #24988, #10193 ) ) ;
#13548=EDGE_CURVE ( 'NONE', #50783, #14315, #8297, .T. ) ;
#13549=CARTESIAN_POINT ( 'NONE',  ( -5.000000000000000000, -13.99999999999999822, 0.000000000000000000 ) ) ;
#13550=CARTESIAN_POINT ( 'NONE',  ( -2.229367062500000163, -10.72916666530106866, -3.861377020970580443 ) ) ;
#13551=CARTESIAN_POINT ( 'NONE',  ( -2.499999999999996447, -34.83333333333332860, 4.330127018922195425 ) ) ;
#13556=CARTESIAN_POINT ( 'NONE',  ( -4.458734124999999437, 24.35416666803225993, -2.574251347313719407 ) ) ;
#13557=ORIENTED_EDGE ( 'NONE', *, *, #53664, .T. ) ;
#13558=CARTESIAN_POINT ( 'NONE',  ( 4.458734125000000326, -93.89583333196772230, 2.574251347313718519 ) ) ;
#13559=CARTESIAN_POINT ( 'NONE',  ( 1.975475456537005874E-15, -77.75000000000000000, 5.000000000000000000 ) ) ;
#13560=CARTESIAN_POINT ( 'NONE',  ( -1.339745962155610925, -69.66965819600731891, 5.000000000000000000 ) ) ;
#13561=CARTESIAN_POINT ( 'NONE',  ( 2.229367062499998831, -9.645833331967738289, -3.861377020970580887 ) ) ;
#13563=DIRECTION ( 'NONE',  ( 0.000000000000000000, 0.000000000000000000, 1.000000000000000000 ) ) ;
#13565=CARTESIAN_POINT ( 'NONE',  ( 2.499999999999998668, -38.20833333060213732, -4.330127018922193649 ) ) ;
#13566=CARTESIAN_POINT ( 'NONE',  ( -6.972266317189433020E-16, -29.25000000000000000, -5.000000000000000000 ) ) ;
#13567=CARTESIAN_POINT ( 'NONE',  ( 2.229367062499998831, 21.35416666803226349, -3.861377020970580887 ) ) ;
#13568=CARTESIAN_POINT ( 'NONE',  ( 1.339745962155612702, -51.16965819600732601, -5.000000000000000000 ) ) ;
#13570=CARTESIAN_POINT ( 'NONE',  ( 2.229367062500001939, -54.97916666530107221, 3.861377020970579999 ) ) ;
#13573=CARTESIAN_POINT ( 'NONE',  ( -4.999999999999999112, 8.083333333333330373, 2.886751345948131764 ) ) ;
#13576=CARTESIAN_POINT ( 'NONE',  ( -2.229367062500000163, -50.47916666530107221, -3.861377020970580443 ) ) ;
#13577=CARTESIAN_POINT ( 'NONE',  ( 1.060575238724906964E-15, -86.62499999726881583, 5.773502691896257311 ) ) ;
#13579=DIRECTION ( 'NONE',  ( 0.000000000000000000, 0.000000000000000000, 1.000000000000000000 ) ) ;
#13580=CARTESIAN_POINT ( 'NONE',  ( -2.229367062500000163, -88.72916666530106511, -3.861377020970580443 ) ) ;
#13582=CARTESIAN_POINT ( 'NONE',  ( 2.499999999999998668, -39.33333333333332860, -4.330127018922193649 ) ) ;
#13583=CARTESIAN_POINT ( 'NONE',  ( 1.975475456537005874E-15, 8.375000002731187720, 5.000000000000000000 ) ) ;
#13586=ORIENTED_EDGE ( 'NONE', *, *, #23995, .T. ) ;
#13587=CARTESIAN_POINT ( 'NONE',  ( -2.229367062499996610, -96.14583333196773651, 3.861377020970582219 ) ) ;
#13588=CARTESIAN_POINT ( 'NONE',  ( 9.457646018065525792E-16, 6.687500001365594748, 5.148502694627439702 ) ) ;
#13589=CARTESIAN_POINT ( 'NONE',  ( -5.000000000000000000, 12.04166666939785379, -2.886751345948128211 ) ) ;
#13593=CARTESIAN_POINT ( 'NONE',  ( 1.975475456537005874E-15, 15.37500000273118417, 5.000000000000000000 ) ) ;
#13596=CARTESIAN_POINT ( 'NONE',  ( -6.972266317189433020E-16, 3.875000002731185500, -5.000000000000000000 ) ) ;
#13597=CARTESIAN_POINT ( 'NONE',  ( 1.975475456537005874E-15, -44.74999999999999289, 5.000000000000000000 ) ) ;
#13600=CARTESIAN_POINT ( 'NONE',  ( -1.339745962155613812, -90.08034179853029855, -5.000000000000000000 ) ) ;
#13601=CARTESIAN_POINT ( 'NONE',  ( 4.458734124999999437, -18.06249999863440792, -5.460374474430324690E-16 ) ) ;
#13611=CARTESIAN_POINT ( 'NONE',  ( 5.000000000000000888, -93.45833333060215864, 2.886751345948126879 ) ) ;
#13613=CARTESIAN_POINT ( 'NONE',  ( -2.229367062499996610, -69.39583333196773651, 3.861377020970582219 ) ) ;
#13615=( LENGTH_UNIT ( ) NAMED_UNIT ( * ) SI_UNIT ( .MILLI., .METRE. ) );
#13619=CARTESIAN_POINT ( 'NONE',  ( -4.458734124999998549, 2.520833334698928674, 2.574251347313722516 ) ) ;
#13621=CARTESIAN_POINT ( 'NONE',  ( -1.339745962155613812, 1.919658201469706116, -5.000000000000000000 ) ) ;
#13622=CARTESIAN_POINT ( 'NONE',  ( -4.458734124999999437, 2.687500001365593860, 0.000000000000000000 ) ) ;
#13628=CARTESIAN_POINT ( 'NONE',  ( 4.458734124999999437, -77.81249999863440792, -5.460374474430324690E-16 ) ) ;
#13629=CARTESIAN_POINT ( 'NONE',  ( -6.972266317189433020E-16, 14.87500000273118594, -5.000000000000000000 ) ) ;
#13630=CARTESIAN_POINT ( 'NONE',  ( -4.458734124999998549, 4.770833334698926009, 2.574251347313722516 ) ) ;
#13632=CARTESIAN_POINT ( 'NONE',  ( 2.229367062499998831, -58.89583333196773651, -3.861377020970580887 ) ) ;
#13633=CARTESIAN_POINT ( 'NONE',  ( -5.000000000000000000, -21.95833333060214798, -2.886751345948128211 ) ) ;
#13634=CARTESIAN_POINT ( 'NONE',  ( 1.339745962155615144, -96.58034179853028434, 4.999999999999999112 ) ) ;
#13637=LINE ( 'NONE', #11808, #746 ) ;
#13638=CARTESIAN_POINT ( 'NONE',  ( -4.458734124999998549, -40.22916666530107932, 2.574251347313722516 ) ) ;
#13639=CARTESIAN_POINT ( 'NONE',  ( -3.152548672688508926E-16, -27.81249999863440436, -5.148502694627439702 ) ) ;
#13641=CARTESIAN_POINT ( 'NONE',  ( -3.535250795749689387E-16, 25.74999999999999645, -5.773502691896257311 ) ) ;
#13643=VERTEX_POINT ( 'NONE', #31562 ) ;
#13644=CARTESIAN_POINT ( 'NONE',  ( 2.229367062500001939, -106.2291666653010651, 3.861377020970579999 ) ) ;
#13646=CARTESIAN_POINT ( 'NONE',  ( 4.458734124999999437, -29.81249999863440436, -5.460374474430324690E-16 ) ) ;
#13647=CARTESIAN_POINT ( 'NONE',  ( 5.000000000000000000, -69.37499999726880162, -6.123233995736766282E-16 ) ) ;
#13650=CARTESIAN_POINT ( 'NONE',  ( 2.229367062499998831, -28.64583333196774007, -3.861377020970580887 ) ) ;
#13651=CARTESIAN_POINT ( 'NONE',  ( 4.458734124999998549, -75.97916666530106511, -2.574251347313721627 ) ) ;
#13655=CARTESIAN_POINT ( 'NONE',  ( 5.000000000000000000, 22.62500000273118772, -6.123233995736766282E-16 ) ) ;
#13656=CARTESIAN_POINT ( 'NONE',  ( -3.535250795749689387E-16, -20.24999999999999645, -5.773502691896257311 ) ) ;
#13658=VERTEX_POINT ( 'NONE', #22559 ) ;
#13659=CARTESIAN_POINT ( 'NONE',  ( -6.972266317189433020E-16, -49.24999999999999289, -5.000000000000000000 ) ) ;
#13661=CARTESIAN_POINT ( 'NONE',  ( -5.000000000000000000, 28.04166666939785202, -2.886751345948128211 ) ) ;
#13662=DIRECTION ( 'NONE',  ( -0.000000000000000000, 1.000000000000000000, -0.000000000000000000 ) ) ;
#13666=CARTESIAN_POINT ( 'NONE',  ( 2.499999999999998668, 28.66666666666666785, -4.330127018922193649 ) ) ;
#13679=CARTESIAN_POINT ( 'NONE',  ( 1.975475456537005874E-15, -95.75000000000000000, 5.000000000000000000 ) ) ;
#13682=ORIENTED_EDGE ( 'NONE', *, *, #20404, .T. ) ;
#13686=ORIENTED_EDGE ( 'NONE', *, *, #22790, .F. ) ;
#13687=CARTESIAN_POINT ( 'NONE',  ( 2.229367062500001939, -79.97916666530106511, 3.861377020970579999 ) ) ;
#13688=CARTESIAN_POINT ( 'NONE',  ( -4.458734124999999437, 20.68750000136559208, 0.000000000000000000 ) ) ;
#13690=ORIENTED_EDGE ( 'NONE', *, *, #43570, .T. ) ;
#13694=CARTESIAN_POINT ( 'NONE',  ( 1.975475456537005874E-15, -74.62499999726880162, 5.000000000000000000 ) ) ;
#13695=CARTESIAN_POINT ( 'NONE',  ( 2.499999999999998668, 4.666666666666666075, -4.330127018922193649 ) ) ;
#13696=CARTESIAN_POINT ( 'NONE',  ( 9.457646018065525792E-16, -60.06249999863440081, 5.148502694627439702 ) ) ;
#13698=CARTESIAN_POINT ( 'NONE',  ( 4.458734125000001214, 25.10416666803225638, 2.574251347313718519 ) ) ;
#13699=CARTESIAN_POINT ( 'NONE',  ( 2.499999999999998668, -97.33333333333332860, -4.330127018922193649 ) ) ;
#13701=CARTESIAN_POINT ( 'NONE',  ( -2.229367062499996610, -45.39583333196774362, 3.861377020970582219 ) ) ;
#13702=CARTESIAN_POINT ( 'NONE',  ( 2.499999999999998668, -5.208333330602148870, -4.330127018922193649 ) ) ;
#13703=CARTESIAN_POINT ( 'NONE',  ( -1.339745962155610925, -92.79465819873851729, 5.000000000000000000 ) ) ;
#13706=CARTESIAN_POINT ( 'NONE',  ( -2.229367062499996610, -108.1458333319677365, 3.861377020970582219 ) ) ;
#13707=CARTESIAN_POINT ( 'NONE',  ( 2.229367062500001939, -10.22916666530106866, 3.861377020970579999 ) ) ;
#13708=ORIENTED_EDGE ( 'NONE', *, *, #49085, .T. ) ;
#13709=CARTESIAN_POINT ( 'NONE',  ( -4.458734124999999437, -98.31249999863440792, 0.000000000000000000 ) ) ;
#13711=CARTESIAN_POINT ( 'NONE',  ( 2.229367062500001939, -91.22916666530106511, 3.861377020970579999 ) ) ;
#13712=EDGE_CURVE ( 'NONE', #25378, #31719, #10724, .T. ) ;
#13713=CARTESIAN_POINT ( 'NONE',  ( -2.500000000000000444, -54.04166666393548013, -4.330127018922193649 ) ) ;
#13717=CARTESIAN_POINT ( 'NONE',  ( 4.458734124999998549, -14.72916666530107221, -2.574251347313721627 ) ) ;
#13718=CARTESIAN_POINT ( 'NONE',  ( 4.458734125000001214, 10.85416666803225993, 2.574251347313718519 ) ) ;
#13719=CARTESIAN_POINT ( 'NONE',  ( -4.458734124999997661, -59.47916666530106511, 2.574251347313722516 ) ) ;
#13720=( BOUNDED_CURVE ( )  B_SPLINE_CURVE ( 2, ( #5425, #15716, #29854, #14745, #59467, #34362, #45299, #53992, #35660 ),
 .UNSPECIFIED., .F., .F. ) 
 B_SPLINE_CURVE_WITH_KNOTS ( ( 3, 2, 2, 2, 3 ),
 ( 0.6767857142857143238, 0.6773809523809524169, 0.6785714285714286031, 0.6797619047619047894, 0.6803571428571428825 ),
 .UNSPECIFIED. ) 
 CURVE ( )  GEOMETRIC_REPRESENTATION_ITEM ( )  RATIONAL_B_SPLINE_CURVE ( ( 0.9330127018922194093, 0.9330127018922194093, 1.000000000000000000, 0.8660254037844387076, 1.000000000000000000, 0.8660254037844387076, 1.000000000000000000, 0.9330127018922194093, 0.9330127018922194093 ) ) 
 REPRESENTATION_ITEM ( '' )  );
#13722=CARTESIAN_POINT ( 'NONE',  ( -2.499999999999996447, -105.8333333333333286, 4.330127018922195425 ) ) ;
#13725=EDGE_LOOP ( 'NONE', ( #8179, #9878, #1165, #60126 ) ) ;
#13727=LINE ( 'NONE', #28830, #5832 ) ;
#13728=CARTESIAN_POINT ( 'NONE',  ( 2.499999999999998668, -68.33333333333332860, -4.330127018922193649 ) ) ;
#13729=EDGE_CURVE ( 'NONE', #53022, #41, #37040, .T. ) ;
#13731=CARTESIAN_POINT ( 'NONE',  ( -2.229367062499996610, -83.14583333196773651, 3.861377020970582219 ) ) ;
#13732=CARTESIAN_POINT ( 'NONE',  ( 2.229367062499998831, 26.10416666803225993, -3.861377020970580887 ) ) ;
#13739=CARTESIAN_POINT ( 'NONE',  ( 2.500000000000002220, -68.66666666666667140, 4.330127018922192761 ) ) ;
#13743=CARTESIAN_POINT ( 'NONE',  ( -2.500000000000000444, -80.04166666393547303, -4.330127018922193649 ) ) ;
#13755=CARTESIAN_POINT ( 'NONE',  ( -3.152548672688508926E-16, -54.81249999863440081, -5.148502694627439702 ) ) ;
#13758=ORIENTED_EDGE ( 'NONE', *, *, #35905, .T. ) ;
#13765=CARTESIAN_POINT ( 'NONE',  ( -4.458734124999999437, -106.5624999986343937, 0.000000000000000000 ) ) ;
#13766=CARTESIAN_POINT ( 'NONE',  ( -6.972266317189433020E-16, -69.12499999726880162, -5.000000000000000000 ) ) ;
#13767=ORIENTED_EDGE ( 'NONE', *, *, #60053, .F. ) ;
#13770=CARTESIAN_POINT ( 'NONE',  ( -2.229367062500000163, -36.47916666530107221, -3.861377020970580443 ) ) ;
#13771=( BOUNDED_CURVE ( )  B_SPLINE_CURVE ( 2, ( #24286, #9486, #62911, #8556, #57772, #43889, #33313, #62288, #8870 ),
 .UNSPECIFIED., .F., .F. ) 
 B_SPLINE_CURVE_WITH_KNOTS ( ( 3, 2, 2, 2, 3 ),
 ( 0.8446428571428571397, 0.8452380952380952328, 0.8464285714285714191, 0.8476190476190476053, 0.8482142857142856984 ),
 .UNSPECIFIED. ) 
 CURVE ( )  GEOMETRIC_REPRESENTATION_ITEM ( )  RATIONAL_B_SPLINE_CURVE ( ( 0.9330127018922194093, 0.9330127018922194093, 1.000000000000000000, 0.8660254037844387076, 1.000000000000000000, 0.8660254037844387076, 1.000000000000000000, 0.9330127018922194093, 0.9330127018922194093 ) ) 
 REPRESENTATION_ITEM ( '' )  );
#13773=CARTESIAN_POINT ( 'NONE',  ( -4.458734124999998549, -6.229166665301072214, 2.574251347313722516 ) ) ;
#13774=CARTESIAN_POINT ( 'NONE',  ( 9.457646018065525792E-16, -98.31249999863440792, 5.148502694627439702 ) ) ;
#13777=CARTESIAN_POINT ( 'NONE',  ( -3.152548672688508926E-16, -27.81249999863440436, -5.148502694627439702 ) ) ;
#13782=CARTESIAN_POINT ( 'NONE',  ( 1.339745962155612702, -88.16965819600733312, -5.000000000000000000 ) ) ;
#13784=CARTESIAN_POINT ( 'NONE',  ( -2.229367062500000163, 7.270833334698929562, -3.861377020970580443 ) ) ;
#13787=CARTESIAN_POINT ( 'NONE',  ( -5.000000000000000000, -93.00000000000000000, 0.000000000000000000 ) ) ;
#13788=CARTESIAN_POINT ( 'NONE',  ( -4.458734124999999437, -28.39583333196774007, -2.574251347313719407 ) ) ;
#13790=CARTESIAN_POINT ( 'NONE',  ( -2.229367062500000163, -76.72916666530106511, -3.861377020970580443 ) ) ;
#13796=EDGE_CURVE ( 'NONE', #38436, #18131, #28932, .T. ) ;
#13797=CARTESIAN_POINT ( 'NONE',  ( 2.229367062499998831, 1.354166668032261933, -3.861377020970580887 ) ) ;
#13798=CARTESIAN_POINT ( 'NONE',  ( 4.458734124999999437, 26.93750000136559564, -5.460374474430324690E-16 ) ) ;
#13799=CARTESIAN_POINT ( 'NONE',  ( -4.458734124999999437, -38.64583333196773651, -2.574251347313719407 ) ) ;
#13805=CARTESIAN_POINT ( 'NONE',  ( -4.458734124999999437, -67.31249999863440792, 0.000000000000000000 ) ) ;
#13806=CARTESIAN_POINT ( 'NONE',  ( -2.499999999999996447, -101.7083333306021444, 4.330127018922195425 ) ) ;
#13809=CARTESIAN_POINT ( 'NONE',  ( 0.000000000000000000, -120.0000000000000000, 5.000000000000000000 ) ) ;
#13811=CARTESIAN_POINT ( 'NONE',  ( -2.229367062499996610, -107.3958333319677365, 3.861377020970582219 ) ) ;
#13813=CARTESIAN_POINT ( 'NONE',  ( 1.060575238724906964E-15, -55.74999999999999289, 5.773502691896257311 ) ) ;
#13821=ADVANCED_FACE ( 'NONE', ( #3879 ), #23498, .T. ) ;
#13826=ORIENTED_EDGE ( 'NONE', *, *, #30346, .F. ) ;
#13829=VERTEX_POINT ( 'NONE', #62741 ) ;
#13833=CARTESIAN_POINT ( 'NONE',  ( -3.152548672688508926E-16, -39.81249999863440081, -5.148502694627439702 ) ) ;
#13839=CARTESIAN_POINT ( 'NONE',  ( 1.339745962155615144, -26.70534180126147561, 4.999999999999999112 ) ) ;
#13841=CARTESIAN_POINT ( 'NONE',  ( 2.229367062499998831, -85.89583333196773651, -3.861377020970580887 ) ) ;
#13843=ORIENTED_EDGE ( 'NONE', *, *, #15606, .T. ) ;
#13847=ORIENTED_EDGE ( 'NONE', *, *, #58177, .T. ) ;
#13850=CARTESIAN_POINT ( 'NONE',  ( -4.458734124999999437, -10.56249999863440792, 0.000000000000000000 ) ) ;
#13855=CARTESIAN_POINT ( 'NONE',  ( -3.152548672688508926E-16, 19.18750000136559208, -5.148502694627439702 ) ) ;
#13857=CARTESIAN_POINT ( 'NONE',  ( -4.458734124999997661, -92.22916666530106511, 2.574251347313722516 ) ) ;
#13858=CARTESIAN_POINT ( 'NONE',  ( 5.000000000000000888, -47.58333333333333570, 2.886751345948126879 ) ) ;
#13859=CARTESIAN_POINT ( 'NONE',  ( -4.999999999999998224, -103.7916666639354730, 2.886751345948131764 ) ) ;
#13860=CARTESIAN_POINT ( 'NONE',  ( -3.152548672688508926E-16, -6.562499998634404363, -5.148502694627439702 ) ) ;
#13862=CYLINDRICAL_SURFACE ( 'NONE', #55106, 5.000000000000000000 ) ;
#13867=CARTESIAN_POINT ( 'NONE',  ( -5.000000000000000000, -34.95833333060213732, -2.886751345948128211 ) ) ;
#13869=CARTESIAN_POINT ( 'NONE',  ( -3.152548672688508926E-16, 21.43750000136559208, -5.148502694627439702 ) ) ;
#13872=CARTESIAN_POINT ( 'NONE',  ( -4.458734124999999437, -56.31249999863440081, 0.000000000000000000 ) ) ;
#13875=CARTESIAN_POINT ( 'NONE',  ( -2.500000000000000444, 7.833333333333334814, -4.330127018922193649 ) ) ;
#13877=CARTESIAN_POINT ( 'NONE',  ( 1.975475456537005874E-15, -69.74999999999998579, 5.000000000000000000 ) ) ;
#13878=CARTESIAN_POINT ( 'NONE',  ( -2.229367062500000163, -55.47916666530107221, -3.861377020970580443 ) ) ;
#13879=CARTESIAN_POINT ( 'NONE',  ( 1.060575238724906964E-15, -83.62499999726881583, 5.773502691896257311 ) ) ;
#13881=CARTESIAN_POINT ( 'NONE',  ( 1.339745962155557191, -37.58034179853029855, 5.000000000000032863 ) ) ;
#13883=CARTESIAN_POINT ( 'NONE',  ( -4.458734124999999437, -92.56249999863440792, 0.000000000000000000 ) ) ;
#13885=CARTESIAN_POINT ( 'NONE',  ( 1.060575238724906964E-15, -38.74999999999998579, 5.773502691896257311 ) ) ;
#13886=CARTESIAN_POINT ( 'NONE',  ( -2.500000000000000444, -20.04166666393548013, -4.330127018922193649 ) ) ;
#13887=EDGE_CURVE ( 'NONE', #31992, #2252, #39070, .T. ) ;
#13888=DIRECTION ( 'NONE',  ( -0.000000000000000000, 1.000000000000000000, -0.000000000000000000 ) ) ;
#13890=CARTESIAN_POINT ( 'NONE',  ( -3.152548672688508926E-16, -97.56249999863440792, -5.148502694627439702 ) ) ;
#13891=CARTESIAN_POINT ( 'NONE',  ( -4.458734124999999437, 10.35416666803225816, -2.574251347313719407 ) ) ;
#13892=CARTESIAN_POINT ( 'NONE',  ( -3.535250795749689387E-16, 10.87500000273118417, -5.773502691896257311 ) ) ;
#13893=CARTESIAN_POINT ( 'NONE',  ( -6.972266317189433020E-16, -80.24999999999998579, -5.000000000000000000 ) ) ;
#13894=EDGE_CURVE ( 'NONE', #30039, #49750, #15741, .T. ) ;
#13901=CARTESIAN_POINT ( 'NONE',  ( -5.000000000000000000, -11.00000000000000355, 0.000000000000000000 ) ) ;
#13902=CARTESIAN_POINT ( 'NONE',  ( 5.000000000000000000, 19.58333333333333215, -2.886751345948130876 ) ) ;
#13904=CARTESIAN_POINT ( 'NONE',  ( -1.339745962155606929, 23.91965820146970145, -5.000000000000004441 ) ) ;
#13905=CARTESIAN_POINT ( 'NONE',  ( 4.458734124999998549, -17.97916666530106866, -2.574251347313721627 ) ) ;
#13915=LINE ( 'NONE', #9095, #31265 ) ;
#13917=CARTESIAN_POINT ( 'NONE',  ( -4.458734124999998549, -65.47916666530107932, 2.574251347313722516 ) ) ;
#13919=DIRECTION ( 'NONE',  ( 1.000000000000000000, 0.000000000000000000, 0.000000000000000000 ) ) ;
#13920=ORIENTED_EDGE ( 'NONE', *, *, #33494, .T. ) ;
#13924=CARTESIAN_POINT ( 'NONE',  ( -2.229367062499996610, 3.604166668032260379, 3.861377020970582219 ) ) ;
#13925=VERTEX_POINT ( 'NONE', #14769 ) ;
#13926=DIRECTION ( 'NONE',  ( -0.000000000000000000, 1.000000000000000000, -0.000000000000000000 ) ) ;
#13931=ORIENTED_EDGE ( 'NONE', *, *, #28064, .T. ) ;
#13932=CARTESIAN_POINT ( 'NONE',  ( 2.229367062500001939, -77.97916666530106511, 3.861377020970579999 ) ) ;
#13934=CARTESIAN_POINT ( 'NONE',  ( -3.152548672688508926E-16, 7.437500001365594748, -5.148502694627439702 ) ) ;
#13935=EDGE_CURVE ( 'NONE', #6651, #25665, #17306, .T. ) ;
#13937=CARTESIAN_POINT ( 'NONE',  ( 9.457646018065525792E-16, -60.31249999863440792, 5.148502694627439702 ) ) ;
#13938=CARTESIAN_POINT ( 'NONE',  ( 2.499999999999998668, -22.20833333060215153, -4.330127018922193649 ) ) ;
#13939=CARTESIAN_POINT ( 'NONE',  ( 2.499999999999998668, -96.20833333060213022, -4.330127018922193649 ) ) ;
#13940=CARTESIAN_POINT ( 'NONE',  ( -6.972266317189433020E-16, -44.12499999726880162, -5.000000000000000000 ) ) ;
#13941=CARTESIAN_POINT ( 'NONE',  ( 5.000000000000000888, -49.58333333333332149, 2.886751345948126879 ) ) ;
#13942=DIRECTION ( 'NONE',  ( -0.000000000000000000, 1.000000000000000000, -0.000000000000000000 ) ) ;
#13944=CARTESIAN_POINT ( 'NONE',  ( -3.152548672688508926E-16, -41.56249999863439371, -5.148502694627439702 ) ) ;
#13945=CARTESIAN_POINT ( 'NONE',  ( 4.458734124999999437, -27.06249999863440081, -5.460374474430324690E-16 ) ) ;
#13947=CARTESIAN_POINT ( 'NONE',  ( 5.000000000000000000, 25.58333333333333215, -2.886751345948129988 ) ) ;
#13949=CARTESIAN_POINT ( 'NONE',  ( 4.458734125000001214, -107.1458333319677507, 2.574251347313718519 ) ) ;
#13950=CARTESIAN_POINT ( 'NONE',  ( -3.152548672688508926E-16, -33.56249999863440792, -5.148502694627439702 ) ) ;
#13951=CARTESIAN_POINT ( 'NONE',  ( -3.535250795749689387E-16, -68.12499999726881583, -5.773502691896257311 ) ) ;
#13952=AXIS2_PLACEMENT_3D ( 'NONE', #50688, #59388, #15644 ) ;
#13955=CARTESIAN_POINT ( 'NONE',  ( -4.458734124999997661, -77.47916666530106511, 2.574251347313722516 ) ) ;
#13958=CARTESIAN_POINT ( 'NONE',  ( -6.972266317189433020E-16, -28.12499999726880873, -5.000000000000000000 ) ) ;
#13960=CARTESIAN_POINT ( 'NONE',  ( 5.000000000000000888, -19.58333333333333215, 2.886751345948126879 ) ) ;
#13968=CARTESIAN_POINT ( 'NONE',  ( 2.500000000000002220, 4.458333336064518093, 4.330127018922192761 ) ) ;
#13976=ORIENTED_EDGE ( 'NONE', *, *, #24062, .F. ) ;
#13977=CARTESIAN_POINT ( 'NONE',  ( 5.000000000000000888, -97.45833333060213022, 2.886751345948126879 ) ) ;
#13984=CARTESIAN_POINT ( 'NONE',  ( 5.000000000000000000, -4.416666666666666075, -2.886751345948130876 ) ) ;
#13988=VECTOR ( 'NONE', #12079, 1000.000000000000000 ) ;
#13992=CARTESIAN_POINT ( 'NONE',  ( 1.339745962155615144, -53.58034179853029144, 4.999999999999999112 ) ) ;
#13996=CARTESIAN_POINT ( 'NONE',  ( 2.229367062499998831, -84.64583333196773651, -3.861377020970580887 ) ) ;
#13997=CARTESIAN_POINT ( 'NONE',  ( -4.458734124999998549, 21.77083333469892779, 2.574251347313722516 ) ) ;
#14004=CARTESIAN_POINT ( 'NONE',  ( 1.339745962155612702, 4.705341801261479162, -5.000000000000000000 ) ) ;
#14005=CARTESIAN_POINT ( 'NONE',  ( -3.152548672688508926E-16, -62.56249999863440792, -5.148502694627439702 ) ) ;
#14007=CARTESIAN_POINT ( 'NONE',  ( -2.229367062499996610, 22.85416666803225993, 3.861377020970582219 ) ) ;
#14008=CARTESIAN_POINT ( 'NONE',  ( 1.339745962155612702, -97.29465819873851729, -5.000000000000000000 ) ) ;
#14010=CARTESIAN_POINT ( 'NONE',  ( -2.229367062500000163, -45.72916666530106511, -3.861377020970580443 ) ) ;
#14011=CARTESIAN_POINT ( 'NONE',  ( 5.000000000000000000, -4.291666663935479242, -2.886751345948129988 ) ) ;
#14012=CARTESIAN_POINT ( 'NONE',  ( 2.499999999999998668, -31.33333333333333215, -4.330127018922193649 ) ) ;
#14013=CARTESIAN_POINT ( 'NONE',  ( 1.975475456537005874E-15, -56.62499999726880162, 5.000000000000000000 ) ) ;
#14015=CARTESIAN_POINT ( 'NONE',  ( 4.458734125000000326, -106.8958333319677649, 2.574251347313718519 ) ) ;
#14016=CARTESIAN_POINT ( 'NONE',  ( -4.458734124999997661, -9.479166665301068662, 2.574251347313722516 ) ) ;
#14017=ORIENTED_EDGE ( 'NONE', *, *, #14087, .F. ) ;
#14019=CARTESIAN_POINT ( 'NONE',  ( 2.229367062500001939, -100.9791666653010651, 3.861377020970579999 ) ) ;
#14021=CARTESIAN_POINT ( 'NONE',  ( 4.458734125000001214, -92.14583333196775072, 2.574251347313718519 ) ) ;
#14022=CARTESIAN_POINT ( 'NONE',  ( -4.999999999999999112, -53.79166666393548013, 2.886751345948131764 ) ) ;
#14026=CARTESIAN_POINT ( 'NONE',  ( -4.458734124999999437, -15.39583333196773651, -2.574251347313719407 ) ) ;
#14027=CARTESIAN_POINT ( 'NONE',  ( -4.458734124999998549, 11.52083333469892779, 2.574251347313722516 ) ) ;
#14028=CARTESIAN_POINT ( 'NONE',  ( -4.458734124999997661, -60.47916666530106511, 2.574251347313722516 ) ) ;
#14029=CYLINDRICAL_SURFACE ( 'NONE', #51075, 5.000000000000000000 ) ;
#14031=CARTESIAN_POINT ( 'NONE',  ( 2.500000000000002220, -8.541666663935483683, 4.330127018922192761 ) ) ;
#14035=CARTESIAN_POINT ( 'NONE',  ( -1.339745962155610925, -91.66965819600733312, 5.000000000000000000 ) ) ;
#14037=CARTESIAN_POINT ( 'NONE',  ( 2.229367062500001939, -83.97916666530106511, 3.861377020970579999 ) ) ;
#14038=CARTESIAN_POINT ( 'NONE',  ( 2.229367062499998831, 17.10416666803225993, -3.861377020970580887 ) ) ;
#14040=VECTOR ( 'NONE', #61993, 1000.000000000000000 ) ;
#14043=CARTESIAN_POINT ( 'NONE',  ( 0.000000000000000000, -120.0000000000000000, 0.000000000000000000 ) ) ;
#14044=AXIS2_PLACEMENT_3D ( 'NONE', #50519, #15781, #6459 ) ;
#14047=CARTESIAN_POINT ( 'NONE',  ( -5.000000000000000000, -70.08333333333332860, -2.886751345948128211 ) ) ;
#14049=VERTEX_POINT ( 'NONE', #58840 ) ;
#14050=CARTESIAN_POINT ( 'NONE',  ( 1.339745962155612702, -102.2946581987385173, -5.000000000000000000 ) ) ;
#14064=CARTESIAN_POINT ( 'NONE',  ( 2.229367062499998831, -58.89583333196773651, -3.861377020970580887 ) ) ;
#14066=ORIENTED_EDGE ( 'NONE', *, *, #50786, .F. ) ;
#14068=EDGE_CURVE ( 'NONE', #50477, #8862, #19354, .T. ) ;
#14073=CARTESIAN_POINT ( 'NONE',  ( -4.458734124999999437, -104.6458333319677365, -2.574251347313719407 ) ) ;
#14077=CARTESIAN_POINT ( 'NONE',  ( -2.229367062500000163, -40.47916666530107221, -3.861377020970580443 ) ) ;
#14080=CARTESIAN_POINT ( 'NONE',  ( -4.458734124999998549, -12.22916666530106866, 2.574251347313722516 ) ) ;
#14082=CARTESIAN_POINT ( 'NONE',  ( 9.457646018065525792E-16, -101.3124999986344079, 5.148502694627439702 ) ) ;
#14085=CARTESIAN_POINT ( 'NONE',  ( -2.229367062499996610, -27.39583333196774007, 3.861377020970582219 ) ) ;
#14086=AXIS2_PLACEMENT_3D ( 'NONE', #29437, #44243, #5017 ) ;
#14087=EDGE_CURVE ( 'NONE', #6727, #20337, #5769, .T. ) ;
#14090=( BOUNDED_CURVE ( )  B_SPLINE_CURVE ( 2, ( #40905, #30941, #60861, #50886, #49363, #24925, #55719, #46057, #19775 ),
 .UNSPECIFIED., .F., .F. ) 
 B_SPLINE_CURVE_WITH_KNOTS ( ( 3, 2, 2, 2, 3 ),
 ( 0.2767857142857143016, 0.2773809523809523947, 0.2785714285714285809, 0.2797619047619047672, 0.2803571428571428603 ),
 .UNSPECIFIED. ) 
 CURVE ( )  GEOMETRIC_REPRESENTATION_ITEM ( )  RATIONAL_B_SPLINE_CURVE ( ( 0.9330127018922194093, 0.9330127018922194093, 1.000000000000000000, 0.8660254037844387076, 1.000000000000000000, 0.8660254037844387076, 1.000000000000000000, 0.9330127018922194093, 0.9330127018922194093 ) ) 
 REPRESENTATION_ITEM ( '' )  );
#14093=CARTESIAN_POINT ( 'NONE',  ( -4.458734124999999437, 7.437500001365594748, 0.000000000000000000 ) ) ;
#14094=VERTEX_POINT ( 'NONE', #11855 ) ;
#14095=CARTESIAN_POINT ( 'NONE',  ( 1.975475456537005874E-15, -63.62499999726880873, 5.000000000000000000 ) ) ;
#14096=LINE ( 'NONE', #4450, #22649 ) ;
#14097=CARTESIAN_POINT ( 'NONE',  ( 2.500000000000002220, -97.66666666666665719, 4.330127018922192761 ) ) ;
#14098=CARTESIAN_POINT ( 'NONE',  ( -4.458734124999998549, -32.22916666530106511, 2.574251347313722516 ) ) ;
#14099=CARTESIAN_POINT ( 'NONE',  ( -6.972266317189433020E-16, -73.25000000000000000, -5.000000000000000000 ) ) ;
#14100=CARTESIAN_POINT ( 'NONE',  ( -4.458734124999999437, -77.56249999863440792, 0.000000000000000000 ) ) ;
#14103=EDGE_CURVE ( 'NONE', #35597, #52286, #36316, .T. ) ;
#14105=CARTESIAN_POINT ( 'NONE',  ( -4.458734124999999437, 1.687500001365593194, 0.000000000000000000 ) ) ;
#14106=CARTESIAN_POINT ( 'NONE',  ( 6.123233995736766282E-16, -120.0000000000000000, -5.000000000000000000 ) ) ;
#14107=CARTESIAN_POINT ( 'NONE',  ( 2.229367062499998831, -44.89583333196774362, -3.861377020970580887 ) ) ;
#14112=CARTESIAN_POINT ( 'NONE',  ( -4.458734124999998549, -71.22916666530106511, 2.574251347313722516 ) ) ;
#14113=CARTESIAN_POINT ( 'NONE',  ( 5.000000000000000000, -107.2916666639354588, -2.886751345948129988 ) ) ;
#14116=EDGE_CURVE ( 'NONE', #17975, #35597, #21441, .T. ) ;
#14117=CARTESIAN_POINT ( 'NONE',  ( -2.229367062499996610, -105.3958333319677365, 3.861377020970582219 ) ) ;
#14119=CARTESIAN_POINT ( 'NONE',  ( 5.000000000000000000, -51.50000000000000711, -6.123233995736766282E-16 ) ) ;
#14120=CARTESIAN_POINT ( 'NONE',  ( -1.339745962155613812, -66.20534180126148271, -5.000000000000000000 ) ) ;
#14124=CARTESIAN_POINT ( 'NONE',  ( 2.500000000000002220, -27.54166666393548013, 4.330127018922192761 ) ) ;
#14131=ORIENTED_EDGE ( 'NONE', *, *, #31176, .T. ) ;
#14132=CARTESIAN_POINT ( 'NONE',  ( 1.339745962155612702, -98.29465819873850307, -5.000000000000000000 ) ) ;
#14134=VERTEX_POINT ( 'NONE', #36628 ) ;
#14138=CARTESIAN_POINT ( 'NONE',  ( -3.152548672688508926E-16, -42.81249999863440081, -5.148502694627439702 ) ) ;
#14139=DIRECTION ( 'NONE',  ( -0.000000000000000000, 1.000000000000000000, -0.000000000000000000 ) ) ;
#14149=CARTESIAN_POINT ( 'NONE',  ( 2.500000000000002220, -83.54166666393547303, 4.330127018922192761 ) ) ;
#14151=CARTESIAN_POINT ( 'NONE',  ( -4.458734124999998549, -91.47916666530106511, 2.574251347313722516 ) ) ;
#14156=CARTESIAN_POINT ( 'NONE',  ( 1.975475456537005874E-15, -43.75000000000000000, 5.000000000000000000 ) ) ;
#14158=CARTESIAN_POINT ( 'NONE',  ( -1.339745962155613812, -14.20534180126148094, -5.000000000000000000 ) ) ;
#14159=CARTESIAN_POINT ( 'NONE',  ( -4.458734124999999437, -9.645833331967738289, -2.574251347313719407 ) ) ;
#14160=EDGE_CURVE ( 'NONE', #23800, #27142, #41524, .T. ) ;
#14161=CARTESIAN_POINT ( 'NONE',  ( 2.499999999999998668, -105.2083333306021444, -4.330127018922193649 ) ) ;
#14165=VECTOR ( 'NONE', #44853, 1000.000000000000114 ) ;
#14166=CARTESIAN_POINT ( 'NONE',  ( -2.229367062499996610, 18.60416666803225993, 3.861377020970582219 ) ) ;
#14167=VERTEX_POINT ( 'NONE', #16381 ) ;
#14168=CARTESIAN_POINT ( 'NONE',  ( 2.229367062500001939, -93.97916666530106511, 3.861377020970579999 ) ) ;
#14170=CARTESIAN_POINT ( 'NONE',  ( -6.972266317189433020E-16, 1.875000002731185722, -5.000000000000000000 ) ) ;
#14171=CARTESIAN_POINT ( 'NONE',  ( 4.458734124999998549, -15.72916666530107399, -2.574251347313721627 ) ) ;
#14172=CARTESIAN_POINT ( 'NONE',  ( -5.000000000000000000, -84.95833333060213022, -2.886751345948128211 ) ) ;
#14173=CARTESIAN_POINT ( 'NONE',  ( 0.000000000000000000, -120.0000000000000000, 0.000000000000000000 ) ) ;
#14175=CARTESIAN_POINT ( 'NONE',  ( -3.535250795749689387E-16, -40.12499999726880162, -5.773502691896257311 ) ) ;
#14176=CARTESIAN_POINT ( 'NONE',  ( 1.339745962155612702, -49.16965819600731891, -5.000000000000000000 ) ) ;
#14177=CARTESIAN_POINT ( 'NONE',  ( 4.458734124999999437, 20.18750000136559208, -5.460374474430324690E-16 ) ) ;
#14178=CARTESIAN_POINT ( 'NONE',  ( -1.339745962155625802, 12.33034180399266511, 4.999999999999991118 ) ) ;
#14181=CARTESIAN_POINT ( 'NONE',  ( 4.458734125000001214, -60.89583333196774362, 2.574251347313718519 ) ) ;
#14183=CARTESIAN_POINT ( 'NONE',  ( 0.000000000000000000, -120.0000000000000000, 5.000000000000000000 ) ) ;
#14184=CARTESIAN_POINT ( 'NONE',  ( 5.000000000000000888, 11.41666666666666607, 2.886751345948126879 ) ) ;
#14186=CARTESIAN_POINT ( 'NONE',  ( -2.499999999999996447, -59.70833333060214443, 4.330127018922195425 ) ) ;
#14187=CARTESIAN_POINT ( 'NONE',  ( -2.229367062499996610, -54.14583333196773651, 3.861377020970582219 ) ) ;
#14188=CARTESIAN_POINT ( 'NONE',  ( 5.000000000000000000, -82.29166666393548724, -2.886751345948129988 ) ) ;
#14193=CARTESIAN_POINT ( 'NONE',  ( -2.229367062500000163, -89.72916666530106511, -3.861377020970580443 ) ) ;
#14195=CARTESIAN_POINT ( 'NONE',  ( 5.000000000000000000, -36.41666666666666430, -2.886751345948129988 ) ) ;
#14196=CARTESIAN_POINT ( 'NONE',  ( -6.972266317189433020E-16, -98.12499999726880162, -5.000000000000000000 ) ) ;
#14199=CARTESIAN_POINT ( 'NONE',  ( -4.458734124999999437, -102.3958333319677365, -2.574251347313719407 ) ) ;
#14200=CARTESIAN_POINT ( 'NONE',  ( 9.457646018065525792E-16, 8.687500001365595637, 5.148502694627439702 ) ) ;
#14201=CARTESIAN_POINT ( 'NONE',  ( 2.499999999999998668, 12.79166666939785379, -4.330127018922193649 ) ) ;
#14210=CARTESIAN_POINT ( 'NONE',  ( 5.000000000000000000, -20.41666666666666785, -2.886751345948130876 ) ) ;
#14212=CARTESIAN_POINT ( 'NONE',  ( 1.975475456537005874E-15, -89.62499999726880162, 5.000000000000000000 ) ) ;
#14213=CARTESIAN_POINT ( 'NONE',  ( 4.458734124999998549, -25.97916666530106866, -2.574251347313721627 ) ) ;
#14215=CARTESIAN_POINT ( 'NONE',  ( 6.123233995736766282E-16, -120.0000000000000000, -5.000000000000000000 ) ) ;
#14220=( BOUNDED_CURVE ( )  B_SPLINE_CURVE ( 2, ( #28474, #52303, #47462, #32671, #18810, #58059, #18513, #2782, #33302 ),
 .UNSPECIFIED., .F., .F. ) 
 B_SPLINE_CURVE_WITH_KNOTS ( ( 3, 2, 2, 2, 3 ),
 ( 0.4839285714285714302, 0.4845238095238095233, 0.4857142857142857095, 0.4869047619047618958, 0.4874999999999999889 ),
 .UNSPECIFIED. ) 
 CURVE ( )  GEOMETRIC_REPRESENTATION_ITEM ( )  RATIONAL_B_SPLINE_CURVE ( ( 0.9330127018922194093, 0.9330127018922194093, 1.000000000000000000, 0.8660254037844387076, 1.000000000000000000, 0.8660254037844387076, 1.000000000000000000, 0.9330127018922194093, 0.9330127018922194093 ) ) 
 REPRESENTATION_ITEM ( '' )  );
#14223=EDGE_CURVE ( 'NONE', #42943, #50850, #19731, .T. ) ;
#14225=CARTESIAN_POINT ( 'NONE',  ( 2.500000000000002220, -93.54166666393547303, 4.330127018922192761 ) ) ;
#14226=VERTEX_POINT ( 'NONE', #51432 ) ;
#14227=CARTESIAN_POINT ( 'NONE',  ( 4.458734125000001214, -71.14583333196773651, 2.574251347313718519 ) ) ;
#14229=VERTEX_POINT ( 'NONE', #28154 ) ;
#14230=CARTESIAN_POINT ( 'NONE',  ( -6.972266317189433020E-16, -79.24999999999998579, -5.000000000000000000 ) ) ;
#14235=CARTESIAN_POINT ( 'NONE',  ( 4.458734125000001214, -1.145833331967740509, 2.574251347313718519 ) ) ;
#14246=EDGE_CURVE ( 'NONE', #14537, #12052, #28005, .T. ) ;
#14247=CARTESIAN_POINT ( 'NONE',  ( -4.458734124999999437, -74.39583333196775072, -2.574251347313719407 ) ) ;
#14248=DIRECTION ( 'NONE',  ( -0.000000000000000000, 1.000000000000000000, -0.000000000000000000 ) ) ;
#14249=CARTESIAN_POINT ( 'NONE',  ( 4.458734125000001214, 2.104166668032262599, 2.574251347313718519 ) ) ;
#14250=EDGE_CURVE ( 'NONE', #14315, #100, #13171, .T. ) ;
#14251=CARTESIAN_POINT ( 'NONE',  ( 4.458734125000001214, -68.14583333196773651, 2.574251347313718519 ) ) ;
#14252=CARTESIAN_POINT ( 'NONE',  ( -4.999999999999999112, -25.79166666393547658, 2.886751345948131764 ) ) ;
#14254=DIRECTION ( 'NONE',  ( 0.000000000000000000, 0.000000000000000000, 1.000000000000000000 ) ) ;
#14255=CARTESIAN_POINT ( 'NONE',  ( -2.500000000000000444, -59.16666666666665719, -4.330127018922193649 ) ) ;
#14256=CARTESIAN_POINT ( 'NONE',  ( -2.500000000000000444, -106.0416666639354730, -4.330127018922193649 ) ) ;
#14257=( NAMED_UNIT ( * ) PLANE_ANGLE_UNIT ( ) SI_UNIT ( $, .RADIAN. ) );
#14258=CARTESIAN_POINT ( 'NONE',  ( 2.229367062499998831, -42.64583333196773651, -3.861377020970580887 ) ) ;
#14259=CARTESIAN_POINT ( 'NONE',  ( -4.458734124999999437, -24.64583333196773651, -2.574251347313719407 ) ) ;
#14264=CARTESIAN_POINT ( 'NONE',  ( 2.499999999999998668, 23.66666666666666430, -4.330127018922193649 ) ) ;
#14267=AXIS2_PLACEMENT_3D ( 'NONE', #13379, #57146, #3422 ) ;
#14268=CARTESIAN_POINT ( 'NONE',  ( 2.229367062499998831, -37.64583333196773651, -3.861377020970580887 ) ) ;
#14269=CARTESIAN_POINT ( 'NONE',  ( 5.000000000000000000, -66.29166666393547303, -2.886751345948129988 ) ) ;
#14272=CARTESIAN_POINT ( 'NONE',  ( -4.458734124999999437, -75.64583333196773651, -2.574251347313719407 ) ) ;
#14276=FACE_OUTER_BOUND ( 'NONE', #22902, .T. ) ;
#14277=CARTESIAN_POINT ( 'NONE',  ( 2.500000000000002220, -23.66666666666666785, 4.330127018922192761 ) ) ;
#14279=ORIENTED_EDGE ( 'NONE', *, *, #27532, .F. ) ;
#14281=CARTESIAN_POINT ( 'NONE',  ( -2.500000000000000444, -49.16666666666666430, -4.330127018922193649 ) ) ;
#14283=CARTESIAN_POINT ( 'NONE',  ( -3.535250795749689387E-16, 28.87500000273118417, -5.773502691896257311 ) ) ;
#14291=CARTESIAN_POINT ( 'NONE',  ( 2.499999999999998668, -56.20833333060214443, -4.330127018922193649 ) ) ;
#14292=( BOUNDED_CURVE ( )  B_SPLINE_CURVE ( 2, ( #28532, #58439, #54240, #48150, #33674, #58118, #4103, #23725, #43321 ),
 .UNSPECIFIED., .F., .F. ) 
 B_SPLINE_CURVE_WITH_KNOTS ( ( 3, 2, 2, 2, 3 ),
 ( 0.7803571428571428603, 0.7809523809523809534, 0.7821428571428571397, 0.7833333333333333259, 0.7839285714285714191 ),
 .UNSPECIFIED. ) 
 CURVE ( )  GEOMETRIC_REPRESENTATION_ITEM ( )  RATIONAL_B_SPLINE_CURVE ( ( 0.9330127018922194093, 0.9330127018922194093, 1.000000000000000000, 0.8660254037844387076, 1.000000000000000000, 0.8660254037844387076, 1.000000000000000000, 0.9330127018922194093, 0.9330127018922194093 ) ) 
 REPRESENTATION_ITEM ( '' )  );
#14293=CARTESIAN_POINT ( 'NONE',  ( -2.229367062499996610, -21.14583333196774007, 3.861377020970582219 ) ) ;
#14294=CARTESIAN_POINT ( 'NONE',  ( 2.499999999999998668, 0.6666666666666660745, -4.330127018922193649 ) ) ;
#14301=FACE_OUTER_BOUND ( 'NONE', #527, .T. ) ;
#14302=CARTESIAN_POINT ( 'NONE',  ( 1.975475456537005874E-15, -67.62499999726881583, 5.000000000000000000 ) ) ;
#14311=ORIENTED_EDGE ( 'NONE', *, *, #54183, .F. ) ;
#14312=DIRECTION ( 'NONE',  ( -0.000000000000000000, 1.000000000000000000, -0.000000000000000000 ) ) ;
#14313=CARTESIAN_POINT ( 'NONE',  ( 4.458734124999998549, 20.27083333469892779, -2.574251347313721627 ) ) ;
#14315=VERTEX_POINT ( 'NONE', #4970 ) ;
#14321=CARTESIAN_POINT ( 'NONE',  ( -2.499999999999996447, -102.8333333333333286, 4.330127018922195425 ) ) ;
#14322=CARTESIAN_POINT ( 'NONE',  ( -4.458734124999999437, -60.39583333196774362, -2.574251347313719407 ) ) ;
#14324=CARTESIAN_POINT ( 'NONE',  ( -3.152548672688508926E-16, 20.43750000136559208, -5.148502694627439702 ) ) ;
#14326=CARTESIAN_POINT ( 'NONE',  ( 1.975475456537005874E-15, -43.75000000000000000, 5.000000000000000000 ) ) ;
#14327=ADVANCED_FACE ( 'NONE', ( #58374 ), #4339, .T. ) ;
#14328=CARTESIAN_POINT ( 'NONE',  ( -4.458734124999999437, -49.56249999863440792, 0.000000000000000000 ) ) ;
#14329=CARTESIAN_POINT ( 'NONE',  ( 2.499999999999998668, -4.208333330602147981, -4.330127018922193649 ) ) ;
#14331=CARTESIAN_POINT ( 'NONE',  ( 6.123233995736766282E-16, -120.0000000000000000, -5.000000000000000000 ) ) ;
#14333=CARTESIAN_POINT ( 'NONE',  ( -4.458734124999997661, -106.2291666653010793, 2.574251347313722516 ) ) ;
#14334=CARTESIAN_POINT ( 'NONE',  ( -4.458734124999999437, -11.56249999863440792, 0.000000000000000000 ) ) ;
#14337=CARTESIAN_POINT ( 'NONE',  ( 2.229367062499998831, -97.64583333196773651, -3.861377020970580887 ) ) ;
#14339=CARTESIAN_POINT ( 'NONE',  ( 9.457646018065525792E-16, -90.31249999863439371, 5.148502694627439702 ) ) ;
#14341=CARTESIAN_POINT ( 'NONE',  ( 5.000000000000000000, -51.37499999726881583, -6.123233995736766282E-16 ) ) ;
#14342=FACE_OUTER_BOUND ( 'NONE', #21274, .T. ) ;
#14345=CARTESIAN_POINT ( 'NONE',  ( -4.458734124999999437, -20.39583333196774362, -2.574251347313719407 ) ) ;
#14346=CARTESIAN_POINT ( 'NONE',  ( 2.229367062499998831, 11.10416666803225993, -3.861377020970580887 ) ) ;
#14347=CARTESIAN_POINT ( 'NONE',  ( 2.229367062500001939, -58.22916666530107932, 3.861377020970579999 ) ) ;
#14350=DIRECTION ( 'NONE',  ( -0.000000000000000000, 1.000000000000000000, -0.000000000000000000 ) ) ;
#14357=CARTESIAN_POINT ( 'NONE',  ( 2.229367062499998831, -86.64583333196773651, -3.861377020970580887 ) ) ;
#14358=CARTESIAN_POINT ( 'NONE',  ( 4.458734124999998549, 20.02083333469892779, -2.574251347313721627 ) ) ;
#14359=VECTOR ( 'NONE', #26490, 1000.000000000000000 ) ;
#14363=CARTESIAN_POINT ( 'NONE',  ( 5.000000000000000000, -72.41666666666667140, -2.886751345948129988 ) ) ;
#14365=VERTEX_POINT ( 'NONE', #62892 ) ;
#14366=CARTESIAN_POINT ( 'NONE',  ( 1.339745962155615144, -102.7053418012614827, 4.999999999999999112 ) ) ;
#14367=VERTEX_POINT ( 'NONE', #23657 ) ;
#14380=CARTESIAN_POINT ( 'NONE',  ( 4.458734124999998549, -54.97916666530107221, -2.574251347313721627 ) ) ;
#14382=DIRECTION ( 'NONE',  ( 0.000000000000000000, 0.000000000000000000, 1.000000000000000000 ) ) ;
#14383=EDGE_LOOP ( 'NONE', ( #38130, #12693, #58046, #22781 ) ) ;
#14386=ORIENTED_EDGE ( 'NONE', *, *, #52826, .T. ) ;
#14389=CARTESIAN_POINT ( 'NONE',  ( 4.458734125000001214, -107.1458333319677507, 2.574251347313718519 ) ) ;
#14391=VERTEX_POINT ( 'NONE', #29080 ) ;
#14393=VECTOR ( 'NONE', #11181, 1000.000000000000000 ) ;
#14395=CARTESIAN_POINT ( 'NONE',  ( -3.152548672688508926E-16, -37.56249999863440792, -5.148502694627439702 ) ) ;
#14397=VECTOR ( 'NONE', #50915, 1000.000000000000000 ) ;
#14398=CYLINDRICAL_SURFACE ( 'NONE', #33736, 5.000000000000000000 ) ;
#14399=CARTESIAN_POINT ( 'NONE',  ( -3.152548672688508926E-16, -10.56249999863440792, -5.148502694627439702 ) ) ;
#14400=CARTESIAN_POINT ( 'NONE',  ( -4.458734124999997661, -102.4791666653010509, 2.574251347313722516 ) ) ;
#14401=ORIENTED_EDGE ( 'NONE', *, *, #5916, .T. ) ;
#14403=CARTESIAN_POINT ( 'NONE',  ( -4.458734124999999437, -29.56249999863440436, 0.000000000000000000 ) ) ;
#14404=CARTESIAN_POINT ( 'NONE',  ( -1.339745962155613812, 11.79465819873851906, -5.000000000000000000 ) ) ;
#14410=CARTESIAN_POINT ( 'NONE',  ( -2.229367062499996610, 2.604166668032259491, 3.861377020970582219 ) ) ;
#14411=ORIENTED_EDGE ( 'NONE', *, *, #1944, .T. ) ;
#14413=CARTESIAN_POINT ( 'NONE',  ( -3.535250795749689387E-16, -95.25000000000000000, -5.773502691896257311 ) ) ;
#14414=CARTESIAN_POINT ( 'NONE',  ( -4.458734124999999437, -30.31249999863440436, 0.000000000000000000 ) ) ;
#14415=CARTESIAN_POINT ( 'NONE',  ( -1.339745962155613812, -23.08034179853029144, -5.000000000000000000 ) ) ;
#14416=CARTESIAN_POINT ( 'NONE',  ( 4.458734124999999437, -77.06249999863440792, -5.460374474430324690E-16 ) ) ;
#14421=CARTESIAN_POINT ( 'NONE',  ( 4.458734125000000326, 0.1041666680322607674, 2.574251347313718519 ) ) ;
#14422=CARTESIAN_POINT ( 'NONE',  ( -2.229367062499996610, 27.60416666803225993, 3.861377020970582219 ) ) ;
#14423=CARTESIAN_POINT ( 'NONE',  ( -2.229367062499996610, -45.39583333196774362, 3.861377020970582219 ) ) ;
#14424=CARTESIAN_POINT ( 'NONE',  ( -5.000000000000000000, -3.958333330602147537, -2.886751345948128211 ) ) ;
#14427=CARTESIAN_POINT ( 'NONE',  ( 4.458734124999998549, -68.72916666530106511, -2.574251347313721627 ) ) ;
#14428=CARTESIAN_POINT ( 'NONE',  ( -4.999999999999999112, -107.7916666639354730, 2.886751345948131764 ) ) ;
#14429=ADVANCED_FACE ( 'NONE', ( #14301 ), #23957, .T. ) ;
#14431=DIRECTION ( 'NONE',  ( -0.000000000000000000, 1.000000000000000000, -0.000000000000000000 ) ) ;
#14432=CARTESIAN_POINT ( 'NONE',  ( 2.229367062499998831, -108.8958333319677365, -3.861377020970580887 ) ) ;
#14434=CARTESIAN_POINT ( 'NONE',  ( 1.060575238724906964E-15, -54.75000000000000000, 5.773502691896257311 ) ) ;
#14436=ORIENTED_EDGE ( 'NONE', *, *, #56313, .T. ) ;
#14437=CARTESIAN_POINT ( 'NONE',  ( 1.975475456537005874E-15, -47.74999999999999289, 5.000000000000000000 ) ) ;
#14439=CARTESIAN_POINT ( 'NONE',  ( 5.000000000000000000, -27.37499999726880873, -6.123233995736766282E-16 ) ) ;
#14449=CARTESIAN_POINT ( 'NONE',  ( 2.499999999999998668, -98.33333333333332860, -4.330127018922193649 ) ) ;
#14455=CARTESIAN_POINT ( 'NONE',  ( 9.457646018065525792E-16, -43.31249999863440792, 5.148502694627439702 ) ) ;
#14458=CARTESIAN_POINT ( 'NONE',  ( 0.000000000000000000, -120.0000000000000000, 0.000000000000000000 ) ) ;
#14462=CARTESIAN_POINT ( 'NONE',  ( 1.975475456537005874E-15, -4.624999997268815832, 5.000000000000000000 ) ) ;
#14464=CARTESIAN_POINT ( 'NONE',  ( -2.229367062500000163, -88.72916666530106511, -3.861377020970580443 ) ) ;
#14467=EDGE_LOOP ( 'NONE', ( #56921, #43491, #41508, #62164 ) ) ;
#14468=CARTESIAN_POINT ( 'NONE',  ( 5.000000000000000888, -99.58333333333332860, 2.886751345948126879 ) ) ;
#14471=CARTESIAN_POINT ( 'NONE',  ( -6.972266317189433020E-16, -82.12499999726881583, -5.000000000000000000 ) ) ;
#14473=CARTESIAN_POINT ( 'NONE',  ( -4.458734124999999437, -13.64583333196774007, -2.574251347313719407 ) ) ;
#14474=CARTESIAN_POINT ( 'NONE',  ( 1.339745962155615144, -105.5803417985302843, 4.999999999999999112 ) ) ;
#14476=CARTESIAN_POINT ( 'NONE',  ( -6.972266317189433020E-16, -55.12499999726880873, -5.000000000000000000 ) ) ;
#14478=CARTESIAN_POINT ( 'NONE',  ( -4.458734124999997661, 18.52083333469892779, 2.574251347313722516 ) ) ;
#14480=CARTESIAN_POINT ( 'NONE',  ( -3.152548672688508926E-16, -93.56249999863440792, -5.148502694627439702 ) ) ;
#14481=CARTESIAN_POINT ( 'NONE',  ( -4.999999999999998224, -33.79166666393547303, 2.886751345948131764 ) ) ;
#14483=CARTESIAN_POINT ( 'NONE',  ( 4.458734124999999437, -13.81249999863440259, -5.460374474430324690E-16 ) ) ;
#14484=VECTOR ( 'NONE', #13277, 1000.000000000000000 ) ;
#14486=FACE_OUTER_BOUND ( 'NONE', #37739, .T. ) ;
#14488=CARTESIAN_POINT ( 'NONE',  ( -5.000000000000000000, -41.87499999726880873, 0.000000000000000000 ) ) ;
#14490=CARTESIAN_POINT ( 'NONE',  ( -4.458734124999999437, 21.60416666803226349, -2.574251347313719407 ) ) ;
#14491=CARTESIAN_POINT ( 'NONE',  ( -1.339745962155599601, 11.91965820146970145, -5.000000000000007994 ) ) ;
#14494=CARTESIAN_POINT ( 'NONE',  ( 4.458734124999999437, -61.81249999863440081, -5.460374474430324690E-16 ) ) ;
#14496=CARTESIAN_POINT ( 'NONE',  ( 1.975475456537005874E-15, -8.624999997268812280, 5.000000000000000000 ) ) ;
#14497=CARTESIAN_POINT ( 'NONE',  ( 1.060575238724906964E-15, 8.250000000000000000, 5.773502691896257311 ) ) ;
#14500=CARTESIAN_POINT ( 'NONE',  ( -4.458734124999998549, -55.22916666530107932, 2.574251347313722516 ) ) ;
#14501=CARTESIAN_POINT ( 'NONE',  ( 5.000000000000000888, -88.45833333060214443, 2.886751345948126879 ) ) ;
#14503=CARTESIAN_POINT ( 'NONE',  ( 2.499999999999998668, -14.20833333060214976, -4.330127018922193649 ) ) ;
#14507=CARTESIAN_POINT ( 'NONE',  ( -4.999999999999999112, -39.91666666666667140, 2.886751345948131764 ) ) ;
#14511=CARTESIAN_POINT ( 'NONE',  ( -2.229367062499996610, -99.14583333196773651, 3.861377020970582219 ) ) ;
#14512=CARTESIAN_POINT ( 'NONE',  ( 2.229367062500001939, 3.770833334698926009, 3.861377020970579999 ) ) ;
#14513=( BOUNDED_SURFACE ( )  B_SPLINE_SURFACE ( 1, 2, ( 
 ( #52900, #57426, #43543, #14283, #58667, #58356, #42612, #43855, #28133, #38412, #53525, #9453, #29062, #13661, #23942, #63188, #13347, #19098, #14589, #32968, #53834, #23011, #63502, #34209, #43232, #62250, #58036, #47751, #38716, #48686, #9763, #47443, #62874, #4626, #3707, #33593, #33281, #8836, #28757, #3394, #42924, #57735, #28449, #52591, #18169, #37798, #8524, #23322, #62570, #18489, #38112, #53213, #4018, #23638, #18785, #9146, #48380, #45143, #39353, #1106, #49965, #5918, #20388, #30023, #19740, #34863, #30669, #21026, #55444, #49652, #40634, #49003, #44496, #10411, #44178, #35501, #34519, #145, #60275, #35821, #39666, #39988, #20062, #58983, #15566, #14911, #5588, #29370, #11044, #25525, #30339, #20715, #40320, #59958, #50288, #15881, #4950, #1427, #55119, #6236, #25845, #45462, #16193, #59303, #24573, #54150, #25205, #10090, #29700, #44819, #49331, #5274, #24895, #54484, #458, #15236, #781, #59633, #35186, #54804, #10733, #51880, #47054, #31293, #61862, #61543, #11359, #31623, #7820, #26163, #27423, #50929, #31939, #2060, #3004, #22621, #41572, #17475, #50607, #42217, #17779, #6870, #36136, #37398, #51567, #27118, #2676, #12633, #12328, #30983, #6548, #7506, #32250, #46731, #45782, #1742, #21667, #21344, #40944, #56076, #22298, #41897, #51259, #60594, #37096, #11674, #16828, #56715, #16514, #55757, #26485, #46099, #11996, #41258, #60906, #36447, #7193, #26801, #46421, #2370, #21979, #61224, #17148, #36772, #56403, #3941, #52518, #43469, #4251, #52823, #33519, #12947, #63115, #23866, #57349, #42532, #14201, #43158, #62798, #19026, #47370, #58282, #32571, #38640, #57033, #13589, #8139, #8760, #13267, #57969, #28679, #52193, #27741, #47987, #9069, #28057, #18717, #38031, #57663, #13892, #22938, #3628, #18411, #33208, #32890, #53137, #3318, #62169, #18089, #8453, #37712, #28366, #47676, #23235, #42849, #62492, #23561, #38342, #48298, #10851, #50094, #10530, #30142, #44954, #11172, #30466, #53960, #25332, #39478, #34662, #49771, #20519, #54281, #20192, #59439, #14716, #5717, #49133, #24698, #59114, #58786, #266, #50423, #5398, #59759, #39793, #30795, #34336, #60079, #15368, #6367, #25971, #6048, #15043, #15685, #29825, #45587, #16001, #914, #45269, #9892, #1545, #35625, #10219, #19864, #39161, #35305, #54925, #29502, #5076, #44302, #49458, #55253, #25014, #34991, #44624, #40118, #583, #25656, #1235, #54606, #20836, #40437, #36895, #21471, #51379, #51055, #26608, #2491, #40753, #16639, #31416, #46225, #31109, #17271, #51693, #12758, #32057, #16328, #61666, #1867, #12124, #7634, #27240, #46862, #6999, #41700, #7321, #22428, #35947, #21149, #61348, #31748, #21792, #11493, #2188, #42025, #32381, #47181, #41387, #52006, #60402, #36261, #61035, #55576, #2807, #26282, #50731, #7946, #27549, #16958, #26931, #11801, #6675, #46548, #45905, #36570, #41070, #17599, #56525, #22106, #12445, #37215, #56841, #60716, #55887, #56201, #38762, #62920, #23984, #18834, #4366, #33950, #13393, #29106, #32697, #47793, #4064, #38452, #42972, #19145, #33638, #3437, #8566, #58081, #53258, #53571, #9497, #9193, #3750, #28806, #43589, #58401, #23052, #3123, #48424, #22744, #23372, #63231, #17899, #14329, #14011, #42341, #38157, #57782, #8879, #61980, #37521, #57162, #52944, #42657, #62296, #13702, #48112, #18218, #62614, #18537, #13077, #33324, #52327, #8262, #37844, #27864, #47484, #57476, #33016, #23683, #28493, #52632, #28177, #43282, #49375, #60000, #40360, #59677, #59351, #34907, #54529, #1155, #39712, #29417, #30389, #11091, #39395, #29744, #49048, #19467, #4997, #5320, #5964, #59028, #48730, #15609, #5638, #39082, #15924, #25251, #44868, #35547, #15285, #830, #24616, #43899, #58711, #25574, #34253, #44222, #14637, #35227, #4673, #53881, #10450, #10779, #20437, #30065, #63547, #49694, #20108, #54847, #40035, #9807, #50011, #45188, #20754, #55172, #24939, #188, #19787, #24295, #14959, #34568, #54199, #44545, #10138, #501, #56451, #21716, #11724, #35869, #55496, #12373, #40998, #25891, #11410, #31341, #36186, #26857, #45830, #46153, #41310, #60642, #16564, #16879, #6286, #50981, #1792, #30716, #6921, #46469, #51620, #56765, #50338, #56124, #55808, #36495, #41620, #2415, #31030, #12047, #45507, #1470, #31671, #26532, #51307, #61271, #22027, #50656, #7245, #17193, #36820, #2114, #60958, #31987, #2730, #7554, #21072, #27167, #6594, #26210, #46781, #22349, #21394, #41946, #61590, #40677, #17524, #60322, #16248, #37143, #32299, #37450, #23912, #42582, #33252, #13318, #48351, #51928, #33564, #32939, #43513, #4295, #23610, #23292, #62540, #18459, #28725, #3678, #57081, #58012, #38689, #3364, #57396, #12999, #47101, #32618, #52562, #53185, #22980, #12686, #43203, #52872, #3051, #63159, #8805, #28421, #19069, #42892, #48036, #52245, #7869, #22668, #9117, #61907, #8186, #42267, #62846, #27474, #17827, #38081, #38385, #3987, #57707, #27788, #13633, #47720, #18760, #13938, #47413, #62220, #18138, #37766, #8495, #28105, #58642, #14561, #10383, #29992, #5562, #49625, #34488, #48975, #53804, #20361, #49304, #39321, #63475, #19393, #39959, #4924, #53494, #39013, #58953, #118, #54457, #9737, #10060, #5243, #24543, #44146, #44469, #33875, #14880, #29341, #58326, #54122, #25174, #15539, #35158, #19712, #14252, #44789, #15207, #29033, #25495, #34832, #752, #5888, #24867, #59607, #34183, #9425, #48658, #54773, #43829, #29672, #4599, #10705, #24222, #427, #20032, #30312, #49933, #39637, #59276, #45115, #1080, #20686, #11965, #50259, #36421, #6842, #26455, #41545, #16486, #40604, #60249, #56049, #31595, #51228, #7164, #36106, #30957, #35793, #2341, #31266, #21317, #45435, #1398, #21948, #50582, #35474, #20999, #40918, #45756, #26774, #55416, #55730, #50900, #6524, #26136, #46073, #15852, #60562, #11333, #40292, #11645, #46393, #61196, #2651, #59930, #2031, #1709, #21636, #17118, #36744, #16168, #41229, #56374, #12297, #60876, #16801, #31913, #51540, #7476, #55091, #27089, #46705, #11016, #30637, #6207, #25821, #3293, #42505, #61518, #52494, #32221, #7794, #42192, #41871, #47028, #33490, #52168, #42820, #22912, #57946, #17448, #43132, #62142, #53109, #13867, #33183, #32864, #8427, #28030, #38318, #13241, #2978, #3914, #48271, #12920, #18061, #22595, #56692, #61834, #37683, #52799, #47649, #3602, #23209, #9046, #62465, #17756, #23532, #22270, #32541, #57326, #37372, #12608, #57005, #18385, #62772, #8112, #37068, #8734, #38004, #51852, #28655, #57637, #13565, #27397, #28342, #47959, #27716, #47344, #18692, #44710, #53419, #48587, #58249, #54381, #23842, #38614, #34418, #29919, #44392, #29596, #19000, #9984, #39247, #10307, #39564, #14175, #351, #54047, #49228, #5486, #44072, #4528, #24153, #19953, #59205, #15133, #34755, #37, #58569, #63401, #49545, #58874, #48902, #9352, #28964, #25100, #14488, #63090, #43756, #4847, #9664, #673, #19317, #19637, #14804, #34109, #53731, #5168, #43445, #24467, #38933, #4228, #24786, #20282, #39884, #30233, #33802, #59529, #29272, #15462, #35080, #54699, #10620, #11580, #21563, #60805, #21238, #40845, #55666, #21880, #41160, #1007, #36034, #50181, #45361, #60488, #31199, #1326, #30884, #6455, #25421, #16416, #59852, #35393, #6133, #5804, #10938, #61127, #16093, #6768, #50515, #41476, #45040, #7089, #26064, #17051, #36667, #50828, #15776, #45681, #56296, #31512, #26379, #45997, #1963, #16732, #36349, #51155, #55979, #20611, #12224, #11892, #26703, #46319, #2276, #49856, #60171, #40216, #55015, #1638, #30556, #25747, #20925, #40529, #35716, #55346, #11260, #28817, #63243, #19480, #39094, #19156, #33335, #38775, #9511, #4685, #52644, #58723, #58413, #31839, #52954, #29120, #46636, #48742, #8577, #53269, #23385, #24308, #43913, #62931, #14341, #7409, #63561, #51471, #28188, #56619, #27018, #9204, #48436, #2582, #41799, #22200, #61443, #17371, #36992, #28504, #13407, #23696, #33027, #4378, #33962, #47804, #3761, #48123, #23996, #42983, #18845, #62626, #38171, #14022, #18549, #57793, #13713, #8891, #4075, #43599, #53583, #43295, #38464, #58091, #33651, #59042, #5651, #45201, #25588, #1168, #44557, #35240, #44883, #15937, #9819, #14649, #54859, #25264, #15297, #5009, #20123, #35560, #6299, #40690, #34920, #25904, #34266, #29756, #59364, #29429, #20768, #19798, #49063, #45522, #21085, #24951, #846, #5334, #24629, #11105, #53893, #10463, #30402, #14972, #20449, #513, #39725, #59692, #44236, #10150, #54542, #30076, #200, #10791, #40373, #1482, #60014, #39406, #55184, #34581, #40048, #30729, #50352, #54213, #49707, #50025, #15623, #49390, #5980, #60335, #36834, #51319, #60971, #50668, #2127, #61603, #51942, #22682, #16891, #7884, #16263, #11735, #41323, #11425, #2742, #1804, #31043, #27487, #3065, #6933, #7257, #50994, #6609, #46482, #26222, #36507, #35881, #41962, #17207, #61285, #12386, #7567, #51633, #17538, #56464, #55510, #32313, #32000, #37157, #27179, #56781, #47116, #26545, #45842, #21408, #56138, #46796, #22362, #12059, #12700, #41011, #60653, #21728, #16577, #36198, #55819, #31352, #46165, #31684, #26870, #2428, #22040, #41631, #29047, #28738, #42282, #62554, #38703, #57094, #19083, #62234, #62860, #32953, #14269, #58340, #8820, #48364, #17841, #33888, #53508, #37780, #3379, #4612, #18773, #58023, #9438, #52262, #48672, #37464, #61921, #13013, #38095, #32633, #33267, #42597, #13951, #4308, #38400, #63173, #8200, #27803, #4002, #3692, #28436, #53198, #33577, #47428, #23623, #9132, #23927, #13647, #52886, #48049, #22996, #43528, #18152, #43220, #57412, #13332, #52577, #8509, #28119, #23306, #18475, #47736, #42906, #57721, #9749, #44162, #43841, #48989, #35487, #54135, #44803, #24880, #59943, #63487, #45128, #44481, #55104, #15866, #35172, #34849, #10397, #30007, #40305, #15220, #4936, #5902, #50274, #14894, #5259, #24558, #58653, #131, #440, #1092, #34501, #24236, #54788, #766, #14573, #11028, #20374, #39975, #30652, #54470, #59620, #19725, #19411, #34196, #20701, #29354, #39334, #53819, #10718, #39025, #58967, #49637, #49947, #15551, #5574, #10074, #25188, #59289, #30325, #25508, #29686, #49316, #20046, #39651, #7489, #46085, #6535, #26149, #21962, #41558, #17133, #61209, #2045, #60577, #1724, #31926, #60889, #50913, #11347, #30970, #51554, #16499, #1412, #50595, #6855, #11659, #2355, #21330, #21650, #16813, #36120, #55743, #56063, #45448, #26470, #40930, #6220, #41243, #60262, #31279, #27103, #61529, #32233, #36433, #17461, #25832, #11979, #31608, #21012, #12314, #45768, #40619, #37083, #12621, #51243, #7179, #26787, #16181, #46405, #35806, #36757, #55431, #46718, #56387, #2663, #22283, #41883, #56703, #53122, #52810, #7808, #23854, #47971, #9056, #3926, #28666, #19014, #62155, #14188, #17767, #32877, #8748, #23545, #28043, #4239, #18704, #52180, #57337, #43145, #38329, #38627, #58267, #57958, #52505, #13879, #48284, #43457, #8125, #51865, #33507, #27409, #8439, #63102, #2990, #47041, #27728, #28353, #42518, #22608, #42204, #18397, #61848, #37384, #57017, #12933, #47355, #32555, #3304, #62785, #22926, #18074, #37695, #13253, #47663, #3615, #23222, #42833, #62477, #38018, #57649, #13577, #33195, #30246, #33814, #29611, #49557, #34122, #365, #52, #39261, #15147, #53433, #29285, #44087, #58887, #43769, #29933, #686, #25435, #44724, #28978, #10633, #14501, #24801, #20295, #39896, #59542, #19650, #54394, #19968, #35093, #48600, #9365, #10321, #44406, #34432, #4540, #5499, #39578, #54060, #24166, #14818, #54714, #45053, #59866, #9998, #1020, #63415, #48915, #49241, #19333, #15477, #38946, #58583, #20625, #40231, #5185, #59216, #24481, #53745, #34768, #9677, #25112, #4860, #49869, #5817, #16744, #31526, #26716, #7101, #17062, #36361, #35406, #51484, #11906, #36679, #51168, #56310, #46648, #26076, #41810, #45374, #60500, #55991, #46331, #55677, #31851, #2289, #16105, #21250, #21892, #41488, #2593, #22213, #61140, #16428, #12237, #7421, #27030, #35729, #15790, #55028, #10951, #36048, #30570, #50194, #6146, #55358, #25762, #6468, #1339, #20938, #46010, #40542, #60183, #11272, #30898, #50526, #45694, #1651, #40857, #11592, #31212, #50841, #6781, #26392, #1975, #21574, #41173, #60819, #52433, #61771, #13505, #47894, #57881, #61456, #57263, #33121, #17698, #27966, #27656, #3232, #42757, #17386, #56941, #8052, #22850, #7736, #57579, #28280, #53045, #8668, #56632, #38260, #42128, #8366, #3850, #23471, #43075, #47283, #18321, #47589, #62712, #12546, #32158, #2919, #42440, #62083, #52737, #12862, #13182, #3540, #17996, #37622, #23149, #37005, #32804, #32481, #51794, #62400, #18638, #13806, #23783, #27340, #37946, #33426, #8982, #28593, #48213, #22532, #4168, #46971, #37312, #52110, #14743, #49162, #15396, #34687, #58185, #29527, #43691, #38869, #34359, #24724, #58505, #24406, #63655, #18937, #9917, #53356, #28909, #63338, #63030, #4469, #54634, #9606, #292, #44009, #35021, #38553, #612, #19574, #10558, #30169, #54309, #53989, #5106, #44328, #59464, #19890, #24096, #25039, #5743, #34052, #39187, #39505, #49799, #9291, #58813, #59140, #15074, #10249, #43385, #29852, #19254, #48839, #49485, #5423, #14113, #33739, #44650, #20221, #39822, #48529, #14428, #53673, #29214, #4779, #25362, #45619, #21818, #40146, #2215, #45297, #45933, #16029, #61066, #41416, #55604, #31445, #947, #16986, #36598, #20865, #50119, #51405, #1896, #41098, #56233, #35332, #31773, #20549, #12154, #44981, #21175, #59791, #16355, #25688, #60745, #11826, #15714, #54952 ),
 ( #10881, #40468, #35656, #30825, #30498, #21502, #55914, #6075, #36291, #1262, #60108, #55283, #35976, #51088, #7026, #26635, #11202, #16669, #11521, #46255, #50455, #6395, #26001, #31136, #1575, #40783, #60429, #50761, #6705, #26311, #7977, #18565, #26958, #22454, #52035, #22133, #13422, #12474, #41728, #38188, #13732, #17625, #62007, #61694, #61377, #57188, #36924, #47209, #33354, #52661, #27893, #8288, #23078, #18247, #62323, #8595, #47514, #46576, #43001, #3465, #28206, #42682, #37873, #2836, #32726, #57809, #56553, #27575, #57506, #33045, #3153, #23401, #47820, #7662, #12785, #3777, #62646, #7347, #2518, #17298, #22772, #32084, #51721, #27268, #42052, #46893, #37242, #56867, #32407, #42368, #17926, #37548, #13109, #52353, #44576, #48761, #28524, #43931, #53285, #5028, #39424, #49408, #52970, #4703, #24647, #9221, #19498, #19177, #58430, #34288, #8908, #48457, #63260, #14358, #62948, #49081, #19816, #533, #218, #48141, #29774, #33666, #63579, #59066, #14991, #34601, #38792, #9837, #39113, #54231, #4093, #23716, #29447, #58741, #53601, #43313, #33980, #10170, #20146, #15317, #9533, #39742, #18862, #4395, #29138, #38482, #5352, #58110, #14038, #59383, #28834, #24327, #14668, #43617, #24014, #53911, #44254, #24970, #42216, #17474, #56401, #36771, #51566, #46730, #27117, #37095, #12327, #54560, #7819, #31938, #56714, #7505, #2675, #31292, #61223, #22620, #1740, #16827, #22297, #41896, #11995, #51879, #61541, #36134, #41257, #12632, #32249, #61861, #34939, #27422, #36446, #47053, #3003, #10483, #55756, #30982, #50606, #6547, #56075, #26162, #45781, #21343, #11673, #40943, #26484, #60593, #16513, #2369, #50928, #6869, #46098, #2058, #21666, #60904, #31622, #51257, #7192, #26800, #46420, #21978, #41571, #17147, #57968, #13265, #43157, #4551, #47369, #62491, #18716, #13891, #57662, #33826, #48297, #18088, #23234, #33518, #4250, #24176, #43780, #23865, #18409, #43468, #58281, #53445, #37711, #17778, #63114, #37397, #38030, #14200, #32570, #9377, #57348, #38341, #8452, #28988, #48612, #47986, #19025, #57032, #12946, #52192, #32889, #42531, #8137, #53136, #9068, #27740, #3317, #22937, #62168, #52517, #28056, #13588, #47675, #8759, #3627, #28678, #38639, #42848, #33207, #52822, #28365, #3940, #23559, #62797, #5195, #44736, #19344, #58900, #10011, #24813, #9688, #59554, #30259, #55039, #10646, #58594, #40243, #44099, #54404, #49882, #5831, #25446, #29623, #20309, #29944, #1032, #14512, #63427, #39909, #10334, #377, #53755, #44416, #20637, #10964, #25774, #19981, #30586, #38956, #14829, #39590, #34134, #45066, #4874, #29296, #50208, #6158, #49254, #49569, #54072, #48925, #5508, #24494, #59227, #63, #59881, #34443, #15159, #25123, #34780, #696, #15489, #19660, #35109, #54726, #39272, #15802, #35419, #17073, #2603, #45385, #36371, #11601, #16754, #2299, #7111, #30909, #56002, #26726, #21901, #1984, #21586, #11917, #51494, #46342, #60196, #31540, #26087, #1662, #41184, #51179, #21261, #31221, #6794, #40555, #60829, #35742, #50536, #45708, #20953, #6479, #7431, #36059, #41498, #50852, #27041, #16114, #56325, #26402, #46657, #1351, #12248, #61151, #36692, #31861, #55368, #11283, #46022, #40868, #60512, #16438, #55687, #42178, #61817, #2021, #17107, #37050, #32209, #12284, #52156, #2965, #36408, #41533, #51837, #22581, #22895, #42490, #17742, #36730, #37360, #12905, #8099, #56038, #62128, #56990, #36094, #56363, #32528, #50890, #27703, #11954, #56678, #26762, #47330, #3280, #2639, #55722, #11635, #31255, #6832, #31581, #60864, #26439, #12595, #7780, #46060, #21625, #41218, #16790, #51215, #7151, #31899, #46382, #27075, #2328, #27383, #21935, #61185, #51529, #7466, #47015, #46692, #22258, #41857, #61504, #17434, #28015, #14159, #48256, #4214, #19303, #57931, #18369, #37990, #33788, #53404, #28950, #9336, #13850, #8715, #13550, #43742, #9029, #62758, #23194, #42807, #63386, #28329, #13227, #62447, #18678, #23518, #48573, #33170, #33472, #28641, #47944, #3898, #23826, #57311, #38304, #52784, #18046, #53094, #4513, #38918, #44057, #37668, #43430, #43118, #63074, #24139, #58553, #57622, #18986, #14473, #34094, #38599, #58232, #53719, #9650, #29259, #32850, #48887, #4832, #24451, #52478, #8413, #47633, #3588, #20268, #39234, #30219, #9970, #49214, #19937, #19623, #24772, #11247, #29901, #20598, #659, #35703, #58859, #20910, #39867, #30871, #55330, #10927, #10604, #49843, #5790, #16079, #54681, #44376, #45348, #26051, #10295, #50499, #54032, #14791, #337, #59515, #40515, #49529, #21, #30542, #40202, #34403, #6442, #59838, #15763, #29581, #25408, #35377, #39549, #5152, #59189, #60156, #15120, #34739, #54367, #50165, #5471, #25086, #45027, #25734, #55000, #994, #44695, #6121, #1315, #15449, #35067, #46940, #46619, #1624, #17669, #41780, #2889, #61426, #51455, #32129, #51765, #7709, #11565, #26687, #2564, #17349, #21864, #61742, #12518, #45981, #51139, #36973, #27313, #32451, #52083, #22501, #46304, #42097, #37284, #56913, #1947, #8021, #12831, #45664, #2261, #21224, #60476, #40831, #21548, #22178, #36334, #16401, #36019, #12205, #55651, #31185, #50813, #6750, #41143, #26362, #60791, #56600, #16717, #55964, #11875, #31493, #7072, #41460, #61109, #17034, #36648, #56279, #31822, #7392, #26999, #24068, #27627, #23445, #43356, #27936, #57856, #57546, #33090, #8954, #47256, #23121, #37916, #52705, #37591, #23760, #58154, #19227, #38526, #22821, #4438, #8337, #18608, #14085, #33712, #53331, #13474, #48186, #13777, #28880, #42410, #3201, #4139, #38236, #28251, #17967, #8639, #48501, #38842, #53646, #47865, #58477, #62053, #42725, #3824, #57234, #9265, #32771, #13151, #14403, #34025, #43047, #33399, #18293, #52406, #53013, #47560, #62687, #3509, #43664, #63003, #28565, #62369, #63305, #18912, #53959, #63626, #59758, #29186, #43980, #39792, #35303, #49770, #34990, #24379, #15367, #44623, #15684, #44953, #19547, #5716, #59438, #54605, #10850, #49456, #9891, #29500, #25331, #913, #20518, #40117, #5397, #265, #5075, #54924, #582, #54280, #14715, #34335, #30465, #19863, #4751, #49132, #10218, #15042, #50093, #24696, #25013, #20191, #39477, #59113, #10528, #48813, #29824, #44301, #9580, #30141, #6047, #25655, #35624, #39160, #45268, #34660, #1234, #20835, #40436, #60077, #16000, #58785, #2490, #26607, #46224, #61034, #27239, #46547, #6366, #41386, #55575, #50730, #2187, #36569, #6674, #36260, #11800, #30794, #21791, #1544, #40752, #11492, #11171, #16327, #2806, #21470, #12123, #55886, #46861, #50422, #12444, #31415, #22426, #42024, #22105, #16957, #56200, #31747, #7633, #51378, #35946, #36894, #17598, #1866, #61665, #45586, #25970, #31108, #51054, #32056, #41069, #55252, #41699, #7320, #21148, #60401, #26930, #61346, #26281, #17270, #56524, #45904, #60715, #51692, #6998, #16638, #32696, #62919, #28176, #18217, #42340, #61979, #18832, #47483, #32380, #17898, #37843, #42656, #33323, #52326, #52631, #47792, #3436, #23051, #23371, #12757, #57475, #8260, #37214, #13392, #52943, #58080, #63230, #56840, #62613, #62295, #42971, #48111, #8878, #37520, #18536, #28492, #4063, #8565, #3749, #38156, #9192, #23682, #52005, #57780, #57161, #27863, #13701, #43281, #33014, #38451, #14010, #7945, #33637, #47179, #22743, #13076, #27548, #53257, #48423, #28805, #4365, #23983, #43587, #3122, #40033, #19786, #30388, #10778, #30064, #29743, #5319, #24938, #35226, #10137, #63546, #829, #45187, #29415, #5963, #9496, #38761, #19466, #39394, #59676, #49047, #19144, #49693, #39711, #53570, #50010, #59350, #15283, #25573, #49374, #34906, #39081, #14328, #29105, #15608, #4671, #58710, #48729, #5637, #58400, #24294, #44544, #44867, #54528, #500, #33949, #20107, #54197, #25250, #10449, #43898, #20436, #54846, #14636, #34252, #59027, #53880, #9806, #4996, #24615, #44221, #187, #14958, #34567, #1153, #60641, #16878, #1469, #31340, #31029, #6593, #46152, #20753, #60321, #11409, #26209, #11090, #60957, #31670, #56450, #12046, #59999, #41619, #45506, #55807, #51306, #7244, #26856, #50655, #21715, #50980, #2414, #15923, #40359, #41309, #11723, #1791, #55171, #45829, #22026, #12372, #27166, #21393, #31986, #35546, #16247, #40997, #30715, #46468, #6285, #50337, #51619, #7553, #16563, #6920, #55495, #25890, #26531, #21071, #36185, #40676, #61270, #36494, #2113, #56123, #17192, #36819, #35868, #47719, #2729, #18759, #42891, #3986, #62539, #52561, #33251, #52871, #8804, #12685, #27787, #3677, #18458, #22979, #62845, #13632, #47100, #52244, #38080, #28419, #33563, #53184, #48035, #47412, #23609, #43202, #38384, #3050, #9116, #58011, #46780, #3363, #13937, #61589, #22348, #22667, #23291, #37449, #41945, #17523, #13317, #37142, #56764, #32298, #51927, #42266, #7868, #27473, #57706, #61906, #17826, #57080, #12998, #32617, #8185, #42581, #62219, #18137, #37765, #57395, #32938, #8494, #28104, #54121, #43512, #34487, #117, #34831, #426, #38687, #24866, #58952, #14879, #29991, #4923, #29032, #48657, #44468, #20031, #39636, #59275, #24542, #19392, #24221, #54456, #19711, #9736, #33874, #53493, #10382, #39012, #23911, #9424, #29340, #34182, #15206, #43828, #44145, #39320, #58641, #14560, #10059, #4294, #48973, #63474, #28724, #29671, #49624, #5561, #54772, #48350, #49303, #53803, #5242, #25173, #44788, #4598, #750, #20360, #39958, #59606, #15538, #35157, #63158, #19068, #58325, #14251, #11014, #6206, #46632, #56615, #25820, #55415, #30956, #49932, #41795, #20685, #59929, #30636, #30311, #35473, #22835, #40603, #32144, #11332, #47269, #5887, #32465, #50581, #42425, #3215, #22516, #22194, #61439, #17365, #27641, #2578, #55090, #56927, #37606, #20998, #62068, #1079, #25494, #50258, #7405, #52097, #60248, #10704, #42111, #51778, #45114, #17981, #7722, #27326, #40291, #36987, #46956, #45434, #15851, #1397, #8036, #16166, #35792, #27012, #61756, #12532, #2903, #17683, #37298, #12847, #63018, #28580, #63320, #28894, #3524, #53344, #23771, #43372, #58492, #33413, #57563, #13488, #9278, #48515, #4454, #24083, #53029, #47879, #52719, #19241, #48200, #38248, #62384, #18306, #38856, #3839, #52419, #37930, #57869, #62700, #43678, #8653, #8969, #4154, #23457, #43062, #18925, #32788, #13790, #28266, #57249, #38539, #14416, #34039, #19562, #13165, #58169, #18625, #14100, #53660, #9594, #33105, #33726, #29202, #48827, #4765, #24392, #43995, #63641, #8351, #27950, #47573, #23134, #42740, #10545, #20534, #34676, #20205, #59451, #14730, #5731, #49146, #24711, #59128, #58799, #280, #50438, #5410, #59773, #39809, #11185, #34348, #60092, #15381, #6379, #30807, #50105, #49785, #25345, #44967, #55267, #30156, #19878, #20848, #1559, #49472, #25985, #29515, #53977, #39492, #35005, #16014, #25027, #39174, #6061, #15700, #9905, #45600, #35319, #54939, #5092, #930, #10865, #15061, #44316, #54295, #35639, #10234, #29840, #44638, #25672, #597, #54621, #40132, #1248, #30481, #45282, #40452, #7645, #21161, #41399, #17609, #35961, #61676, #41083, #41711, #11811, #56851, #37225, #51391, #27249, #60414, #12768, #32391, #16651, #45918, #47192, #61360, #36906, #52016, #31122, #27559, #16339, #7959, #40767, #16971, #55586, #12136, #21485, #56536, #46876, #11506, #50744, #36582, #12457, #60729, #7333, #51067, #26619, #2501, #6688, #36276, #31429, #46237, #26294, #17282, #51705, #1880, #32068, #55899, #7011, #2200, #31758, #2818, #22439, #42034, #21804, #61050, #26944, #56214, #46560, #22119, #43294, #57792, #3760, #57172, #8576, #4377, #58411, #29118, #23383, #14339, #22754, #18228, #47803, #17910, #9203, #8271, #37531, #33960, #9509, #13405, #13711, #57488, #13088, #52953, #32709, #42982, #3134, #48435, #23694, #4074, #18844, #14021, #58090, #23994, #62929, #42352, #38773, #38462, #43598, #33649, #8890, #53268, #28815, #63241, #52337, #62625, #19155, #53581, #18548, #61990, #27874, #3447, #28187, #47494, #23062, #42667, #62306, #37855, #38169, #33026, #52642, #33334, #28503, #48122, #24305, #49387, #19796, #48739, #29754, #44881, #5977, #11103, #4683, #10461, #10147, #34917, #59688, #844, #53892, #30075, #20447, #15621, #20121, #39723, #54540, #20765, #40046, #63559, #49705, #49059, #44233, #59360, #5649, #198, #5332, #24949, #43910, #15295, #58721, #34264, #5007, #19478, #9816, #60012, #14970, #25262, #44555, #40371, #39091, #25586, #511, #15935, #35558, #35238, #54857, #10790, #30400, #1166, #50023, #29427, #45199, #14647, #59040, #55182, #24627, #39404, #34578, #54210, #51631, #41009, #30727, #41629, #51317, #1480, #61601, #7255, #26867, #41958, #21726, #46480, #50666, #25902, #21083, #7565, #16260, #11422, #40688, #17204, #50350, #60333, #60969, #56462, #2426, #56135, #45519, #36505, #2125, #36832, #22038, #35879, #61283, #16889, #12057, #31997, #6931, #31041, #6606, #12384, #27177, #46794, #2740, #26542, #21405, #26220, #22360, #41321, #11733, #55508, #45840, #17536, #60651, #1802, #16574, #31349, #36196, #37154, #55817, #46163, #31681, #6297, #56779, #50992, #33575, #8818, #18473, #62858, #18771, #38397, #42279, #57410, #13644, #28434, #52574, #28736, #43218, #13011, #18150, #48047, #58021, #63170, #19081, #13949, #13330, #53196, #9129, #48362, #32631, #38701, #4306, #12698, #32951, #23925, #27485, #43526, #52259, #33265, #3377, #32311, #51940, #42904, #7882, #47114, #3062, #22680, #8198, #37462, #61919, #52883, #3999, #17839, #57092, #27800, #47425, #22994, #42595, #8507, #62232, #3690, #37778, #23621, #28117, #47734, #23304 ) ),
 .UNSPECIFIED., .F., .F., .F. ) 
 B_SPLINE_SURFACE_WITH_KNOTS ( ( 2, 2 ),
 ( 3, 2, 2, 2, 2, 2, 2, 2, 2, 2, 2, 2, 2, 2, 2, 2, 2, 2, 2, 2, 2, 2, 2, 2, 2, 2, 2, 2, 2, 2, 2, 2, 2, 2, 2, 2, 2, 2, 2, 2, 2, 2, 2, 2, 2, 2, 2, 2, 2, 2, 2, 2, 2, 2, 2, 2, 2, 2, 2, 2, 2, 2, 2, 2, 2, 2, 2, 2, 2, 2, 2, 2, 2, 2, 2, 2, 2, 2, 2, 2, 2, 2, 2, 2, 2, 2, 2, 2, 2, 2, 2, 2, 2, 2, 2, 2, 2, 2, 2, 2, 2, 2, 2, 2, 2, 2, 2, 2, 2, 2, 2, 2, 2, 2, 2, 2, 2, 2, 2, 2, 2, 2, 2, 2, 2, 2, 2, 2, 2, 2, 2, 2, 2, 2, 2, 2, 2, 2, 2, 2, 2, 2, 2, 2, 2, 2, 2, 2, 2, 2, 2, 2, 2, 2, 2, 2, 2, 2, 2, 2, 2, 2, 2, 2, 2, 2, 2, 2, 2, 2, 2, 2, 2, 2, 2, 2, 2, 2, 2, 2, 2, 2, 2, 2, 2, 2, 2, 2, 2, 2, 2, 2, 2, 2, 2, 2, 2, 2, 2, 2, 2, 2, 2, 2, 2, 2, 2, 2, 2, 2, 2, 2, 2, 2, 2, 2, 2, 2, 2, 2, 2, 2, 2, 2, 2, 2, 2, 2, 2, 2, 2, 2, 2, 2, 2, 2, 2, 2, 2, 2, 2, 2, 2, 2, 2, 2, 2, 2, 2, 2, 2, 2, 2, 2, 2, 2, 2, 2, 2, 2, 2, 2, 2, 2, 2, 2, 2, 2, 2, 2, 2, 2, 2, 2, 2, 2, 2, 2, 2, 2, 2, 2, 2, 2, 2, 2, 2, 2, 2, 2, 2, 2, 2, 2, 2, 2, 2, 2, 2, 2, 2, 2, 2, 2, 2, 2, 2, 2, 2, 2, 2, 2, 2, 2, 2, 2, 2, 2, 2, 2, 2, 2, 2, 2, 2, 2, 2, 2, 2, 2, 2, 2, 2, 2, 2, 2, 2, 2, 2, 2, 2, 2, 2, 2, 2, 2, 2, 2, 2, 2, 2, 2, 2, 2, 2, 2, 2, 2, 2, 2, 2, 2, 2, 2, 2, 2, 2, 2, 2, 2, 2, 2, 2, 2, 2, 2, 2, 2, 2, 2, 2, 2, 2, 2, 2, 2, 2, 2, 2, 2, 2, 2, 2, 2, 2, 2, 2, 2, 2, 2, 2, 2, 2, 2, 2, 2, 2, 2, 2, 2, 2, 2, 2, 2, 2, 2, 2, 2, 2, 2, 2, 2, 2, 2, 2, 2, 2, 2, 2, 2, 2, 2, 2, 2, 2, 2, 2, 2, 2, 2, 2, 2, 2, 2, 2, 2, 2, 2, 2, 2, 2, 2, 2, 2, 2, 2, 2, 2, 2, 2, 2, 2, 2, 2, 2, 2, 2, 2, 2, 2, 2, 2, 2, 2, 2, 2, 2, 2, 2, 2, 2, 2, 2, 2, 2, 2, 2, 2, 2, 2, 2, 2, 2, 2, 2, 2, 2, 2, 2, 2, 2, 2, 2, 2, 2, 2, 2, 2, 2, 2, 2, 2, 2, 2, 2, 2, 2, 2, 2, 2, 2, 2, 2, 2, 2, 2, 2, 2, 2, 2, 2, 2, 2, 2, 2, 2, 2, 2, 2, 2, 2, 2, 2, 2, 2, 2, 2, 2, 2, 2, 2, 2, 2, 2, 2, 2, 2, 2, 2, 2, 2, 2, 2, 2, 2, 2, 2, 2, 2, 2, 2, 2, 2, 2, 2, 2, 2, 2, 2, 2, 2, 2, 2, 2, 2, 2, 2, 2, 2, 2, 2, 2, 2, 2, 2, 2, 2, 2, 2, 2, 2, 2, 2, 2, 2, 2, 2, 2, 2, 2, 2, 2, 2, 2, 2, 2, 2, 2, 2, 2, 2, 2, 2, 2, 2, 2, 2, 2, 2, 2, 2, 2, 2, 2, 2, 2, 2, 2, 2, 2, 2, 2, 2, 2, 2, 2, 2, 2, 2, 2, 2, 2, 2, 2, 2, 2, 2, 2, 2, 2, 2, 2, 2, 2, 2, 2, 2, 2, 2, 2, 2, 2, 2, 2, 2, 2, 2, 2, 2, 2, 2, 2, 2, 2, 2, 2, 2, 2, 2, 2, 2, 2, 2, 2, 2, 2, 2, 2, 2, 2, 2, 2, 2, 2, 2, 2, 2, 2, 2, 2, 2, 2, 2, 2, 2, 2, 2, 2, 2, 2, 2, 2, 2, 2, 2, 2, 2, 2, 2, 2, 2, 2, 2, 2, 2, 2, 2, 2, 2, 2, 2, 2, 2, 2, 2, 2, 2, 2, 2, 2, 2, 2, 2, 2, 2, 2, 2, 2, 2, 2, 2, 2, 2, 2, 2, 2, 2, 2, 2, 2, 2, 2, 2, 2, 2, 2, 2, 2, 2, 2, 2, 2, 2, 2, 2, 2, 2, 2, 2, 2, 2, 2, 2, 2, 2, 2, 2, 2, 2, 2, 2, 2, 2, 2, 2, 2, 2, 2, 2, 2, 2, 2, 2, 2, 2, 2, 2, 2, 2, 2, 2, 2, 2, 2, 2, 2, 2, 2, 2, 2, 2, 2, 2, 2, 2, 2, 2, 2, 2, 2, 3 ),
 ( 0.000000000000000000, 1.000000000000000000 ),
 ( 0.000000000000000000, 0.001190476190476190584, 0.002380952380952381167, 0.003571428571428571317, 0.004761904761904762334, 0.005952380952380952051, 0.007142857142857142634, 0.008333333333333333218, 0.009523809523809524669, 0.01071428571428571438, 0.01190476190476190410, 0.01309523809523809555, 0.01428571428571428527, 0.01547619047619047672, 0.01666666666666666644, 0.01785714285714285615, 0.01904761904761904934, 0.02023809523809523905, 0.02142857142857142877, 0.02261904761904761849, 0.02380952380952380820, 0.02500000000000000139, 0.02619047619047619110, 0.02738095238095238082, 0.02857142857142857054, 0.02976190476190476025, 0.03095238095238095344, 0.03214285714285713969, 0.03333333333333333287, 0.03452380952380952606, 0.03571428571428571230, 0.03690476190476190549, 0.03809523809523809867, 0.03928571428571428492, 0.04047619047619047811, 0.04166666666666666435, 0.04285714285714285754, 0.04404761904761905073, 0.04523809523809523697, 0.04642857142857143016, 0.04761904761904761640, 0.04880952380952380959, 0.05000000000000000278, 0.05119047619047618902, 0.05238095238095238221, 0.05357142857142856845, 0.05476190476190476164, 0.05595238095238095483, 0.05714285714285714107, 0.05833333333333333426, 0.05952380952380952051, 0.06071428571428571369, 0.06190476190476190688, 0.06309523809523809312, 0.06428571428571427937, 0.06547619047619047949, 0.06666666666666666574, 0.06785714285714285199, 0.06904761904761905211, 0.07023809523809523836, 0.07142857142857142461, 0.07261904761904762473, 0.07380952380952381098, 0.07499999999999999722, 0.07619047619047619735, 0.07738095238095238360, 0.07857142857142856984, 0.07976190476190475609, 0.08095238095238095621, 0.08214285714285714246, 0.08333333333333332871, 0.08452380952380952883, 0.08571428571428571508, 0.08690476190476190133, 0.08809523809523810145, 0.08928571428571428770, 0.09047619047619047394, 0.09166666666666666019, 0.09285714285714286031, 0.09404761904761904656, 0.09523809523809523281, 0.09642857142857143293, 0.09761904761904761918, 0.09880952380952380543, 0.1000000000000000056, 0.1011904761904761918, 0.1023809523809523780, 0.1035714285714285782, 0.1047619047619047644, 0.1059523809523809507, 0.1071428571428571369, 0.1083333333333333370, 0.1095238095238095233, 0.1107142857142857095, 0.1119047619047619097, 0.1130952380952380959, 0.1142857142857142821, 0.1154761904761904823, 0.1166666666666666685, 0.1178571428571428548, 0.1190476190476190410, 0.1202380952380952411, 0.1214285714285714274, 0.1226190476190476136, 0.1238095238095238138, 0.1250000000000000000, 0.1261904761904761862, 0.1273809523809523725, 0.1285714285714285587, 0.1297619047619047727, 0.1309523809523809590, 0.1321428571428571452, 0.1333333333333333315, 0.1345238095238095177, 0.1357142857142857040, 0.1369047619047619180, 0.1380952380952381042, 0.1392857142857142905, 0.1404761904761904767, 0.1416666666666666630, 0.1428571428571428492, 0.1440476190476190355, 0.1452380952380952495, 0.1464285714285714357, 0.1476190476190476220, 0.1488095238095238082, 0.1499999999999999944, 0.1511904761904761807, 0.1523809523809523947, 0.1535714285714285809, 0.1547619047619047672, 0.1559523809523809534, 0.1571428571428571397, 0.1583333333333333259, 0.1595238095238095122, 0.1607142857142857262, 0.1619047619047619124, 0.1630952380952380987, 0.1642857142857142849, 0.1654761904761904712, 0.1666666666666666574, 0.1678571428571428437, 0.1690476190476190577, 0.1702380952380952439, 0.1714285714285714302, 0.1726190476190476164, 0.1738095238095238027, 0.1749999999999999889, 0.1761904761904762029, 0.1773809523809523891, 0.1785714285714285754, 0.1797619047619047616, 0.1809523809523809479, 0.1821428571428571341, 0.1833333333333333204, 0.1845238095238095344, 0.1857142857142857206, 0.1869047619047619069, 0.1880952380952380931, 0.1892857142857142794, 0.1904761904761904656, 0.1916666666666666796, 0.1928571428571428659, 0.1940476190476190521, 0.1952380952380952384, 0.1964285714285714246, 0.1976190476190476109, 0.1988095238095237971, 0.2000000000000000111, 0.2011904761904761973, 0.2023809523809523836, 0.2035714285714285698, 0.2047619047619047561, 0.2059523809523809423, 0.2071428571428571563, 0.2083333333333333426, 0.2095238095238095288, 0.2107142857142857151, 0.2119047619047619013, 0.2130952380952380876, 0.2142857142857142738, 0.2154761904761904878, 0.2166666666666666741, 0.2178571428571428603, 0.2190476190476190466, 0.2202380952380952328, 0.2214285714285714191, 0.2226190476190476053, 0.2238095238095238193, 0.2250000000000000056, 0.2261904761904761918, 0.2273809523809523780, 0.2285714285714285643, 0.2297619047619047505, 0.2309523809523809645, 0.2321428571428571508, 0.2333333333333333370, 0.2345238095238095233, 0.2357142857142857095, 0.2369047619047618958, 0.2380952380952380820, 0.2392857142857142960, 0.2404761904761904823, 0.2416666666666666685, 0.2428571428571428548, 0.2440476190476190410, 0.2452380952380952273, 0.2464285714285714413, 0.2476190476190476275, 0.2488095238095238138, 0.2500000000000000000, 0.2511904761904761862, 0.2523809523809523725, 0.2535714285714285587, 0.2547619047619047450, 0.2559523809523809312, 0.2571428571428571175, 0.2583333333333333592, 0.2595238095238095455, 0.2607142857142857317, 0.2619047619047619180, 0.2630952380952381042, 0.2642857142857142905, 0.2654761904761904767, 0.2666666666666666630, 0.2678571428571428492, 0.2690476190476190355, 0.2702380952380952217, 0.2714285714285714080, 0.2726190476190475942, 0.2738095238095238360, 0.2750000000000000222, 0.2761904761904762085, 0.2773809523809523947, 0.2785714285714285809, 0.2797619047619047672, 0.2809523809523809534, 0.2821428571428571397, 0.2833333333333333259, 0.2845238095238095122, 0.2857142857142856984, 0.2869047619047618847, 0.2880952380952380709, 0.2892857142857143127, 0.2904761904761904989, 0.2916666666666666852, 0.2928571428571428714, 0.2940476190476190577, 0.2952380952380952439, 0.2964285714285714302, 0.2976190476190476164, 0.2988095238095238027, 0.2999999999999999889, 0.3011904761904761751, 0.3023809523809523614, 0.3035714285714285476, 0.3047619047619047894, 0.3059523809523809756, 0.3071428571428571619, 0.3083333333333333481, 0.3095238095238095344, 0.3107142857142857206, 0.3119047619047619069, 0.3130952380952380931, 0.3142857142857142794, 0.3154761904761904656, 0.3166666666666666519, 0.3178571428571428381, 0.3190476190476190244, 0.3202380952380952106, 0.3214285714285714524, 0.3226190476190476386, 0.3238095238095238249, 0.3250000000000000111, 0.3261904761904761973, 0.3273809523809523836, 0.3285714285714285698, 0.3297619047619047561, 0.3309523809523809423, 0.3321428571428571286, 0.3333333333333333148, 0.3345238095238095011, 0.3357142857142856873, 0.3369047619047619291, 0.3380952380952381153, 0.3392857142857143016, 0.3404761904761904878, 0.3416666666666666741, 0.3428571428571428603, 0.3440476190476190466, 0.3452380952380952328, 0.3464285714285714191, 0.3476190476190476053, 0.3488095238095237915, 0.3499999999999999778, 0.3511904761904761640, 0.3523809523809524058, 0.3535714285714285920, 0.3547619047619047783, 0.3559523809523809645, 0.3571428571428571508, 0.3583333333333333370, 0.3595238095238095233, 0.3607142857142857095, 0.3619047619047618958, 0.3630952380952380820, 0.3642857142857142683, 0.3654761904761904545, 0.3666666666666666408, 0.3678571428571428825, 0.3690476190476190688, 0.3702380952380952550, 0.3714285714285714413, 0.3726190476190476275, 0.3738095238095238138, 0.3750000000000000000, 0.3761904761904761862, 0.3773809523809523725, 0.3785714285714285587, 0.3797619047619047450, 0.3809523809523809312, 0.3821428571428571175, 0.3833333333333333592, 0.3845238095238095455, 0.3857142857142857317, 0.3869047619047619180, 0.3880952380952381042, 0.3892857142857142905, 0.3904761904761904767, 0.3916666666666666630, 0.3928571428571428492, 0.3940476190476190355, 0.3952380952380952217, 0.3964285714285714080, 0.3976190476190475942, 0.3988095238095238360, 0.4000000000000000222, 0.4011904761904762085, 0.4023809523809523947, 0.4035714285714285809, 0.4047619047619047672, 0.4059523809523809534, 0.4071428571428571397, 0.4083333333333333259, 0.4095238095238095122, 0.4107142857142856984, 0.4119047619047618847, 0.4130952380952380709, 0.4142857142857143127, 0.4154761904761904989, 0.4166666666666666852, 0.4178571428571428714, 0.4190476190476190577, 0.4202380952380952439, 0.4214285714285714302, 0.4226190476190476164, 0.4238095238095238027, 0.4249999999999999889, 0.4261904761904761751, 0.4273809523809523614, 0.4285714285714285476, 0.4297619047619047894, 0.4309523809523809756, 0.4321428571428571619, 0.4333333333333333481, 0.4345238095238095344, 0.4357142857142857206, 0.4369047619047619069, 0.4380952380952380931, 0.4392857142857142794, 0.4404761904761904656, 0.4416666666666666519, 0.4428571428571428381, 0.4440476190476190244, 0.4452380952380952106, 0.4464285714285714524, 0.4476190476190476386, 0.4488095238095238249, 0.4500000000000000111, 0.4511904761904761973, 0.4523809523809523836, 0.4535714285714285698, 0.4547619047619047561, 0.4559523809523809423, 0.4571428571428571286, 0.4583333333333333148, 0.4595238095238095011, 0.4607142857142856873, 0.4619047619047619291, 0.4630952380952381153, 0.4642857142857143016, 0.4654761904761904878, 0.4666666666666666741, 0.4678571428571428603, 0.4690476190476190466, 0.4702380952380952328, 0.4714285714285714191, 0.4726190476190476053, 0.4738095238095237915, 0.4749999999999999778, 0.4761904761904761640, 0.4773809523809524058, 0.4785714285714285920, 0.4797619047619047783, 0.4809523809523809645, 0.4821428571428571508, 0.4833333333333333370, 0.4845238095238095233, 0.4857142857142857095, 0.4869047619047618958, 0.4880952380952380820, 0.4892857142857142683, 0.4904761904761904545, 0.4916666666666666408, 0.4928571428571428825, 0.4940476190476190688, 0.4952380952380952550, 0.4964285714285714413, 0.4976190476190476275, 0.4988095238095238138, 0.5000000000000000000, 0.5011904761904761862, 0.5023809523809523725, 0.5035714285714285587, 0.5047619047619047450, 0.5059523809523809312, 0.5071428571428571175, 0.5083333333333333037, 0.5095238095238094900, 0.5107142857142856762, 0.5119047619047618625, 0.5130952380952380487, 0.5142857142857142350, 0.5154761904761904212, 0.5166666666666667185, 0.5178571428571429047, 0.5190476190476190910, 0.5202380952380952772, 0.5214285714285714635, 0.5226190476190476497, 0.5238095238095238360, 0.5250000000000000222, 0.5261904761904762085, 0.5273809523809523947, 0.5285714285714285809, 0.5297619047619047672, 0.5309523809523809534, 0.5321428571428571397, 0.5333333333333333259, 0.5345238095238095122, 0.5357142857142856984, 0.5369047619047618847, 0.5380952380952380709, 0.5392857142857142572, 0.5404761904761904434, 0.5416666666666666297, 0.5428571428571428159, 0.5440476190476190022, 0.5452380952380951884, 0.5464285714285713746, 0.5476190476190476719, 0.5488095238095238582, 0.5500000000000000444, 0.5511904761904762307, 0.5523809523809524169, 0.5535714285714286031, 0.5547619047619047894, 0.5559523809523809756, 0.5571428571428571619, 0.5583333333333333481, 0.5595238095238095344, 0.5607142857142857206, 0.5619047619047619069, 0.5630952380952380931, 0.5642857142857142794, 0.5654761904761904656, 0.5666666666666666519, 0.5678571428571428381, 0.5690476190476190244, 0.5702380952380952106, 0.5714285714285713969, 0.5726190476190475831, 0.5738095238095237693, 0.5749999999999999556, 0.5761904761904761418, 0.5773809523809523281, 0.5785714285714286254, 0.5797619047619048116, 0.5809523809523809978, 0.5821428571428571841, 0.5833333333333333703, 0.5845238095238095566, 0.5857142857142857428, 0.5869047619047619291, 0.5880952380952381153, 0.5892857142857143016, 0.5904761904761904878, 0.5916666666666666741, 0.5928571428571428603, 0.5940476190476190466, 0.5952380952380952328, 0.5964285714285714191, 0.5976190476190476053, 0.5988095238095237915, 0.5999999999999999778, 0.6011904761904761640, 0.6023809523809523503, 0.6035714285714285365, 0.6047619047619047228, 0.6059523809523809090, 0.6071428571428570953, 0.6083333333333332815, 0.6095238095238095788, 0.6107142857142857650, 0.6119047619047619513, 0.6130952380952381375, 0.6142857142857143238, 0.6154761904761905100, 0.6166666666666666963, 0.6178571428571428825, 0.6190476190476190688, 0.6202380952380952550, 0.6214285714285714413, 0.6226190476190476275, 0.6238095238095238138, 0.6250000000000000000, 0.6261904761904761862, 0.6273809523809523725, 0.6285714285714285587, 0.6297619047619047450, 0.6309523809523809312, 0.6321428571428571175, 0.6333333333333333037, 0.6345238095238094900, 0.6357142857142856762, 0.6369047619047618625, 0.6380952380952380487, 0.6392857142857142350, 0.6404761904761904212, 0.6416666666666667185, 0.6428571428571429047, 0.6440476190476190910, 0.6452380952380952772, 0.6464285714285714635, 0.6476190476190476497, 0.6488095238095238360, 0.6500000000000000222, 0.6511904761904762085, 0.6523809523809523947, 0.6535714285714285809, 0.6547619047619047672, 0.6559523809523809534, 0.6571428571428571397, 0.6583333333333333259, 0.6595238095238095122, 0.6607142857142856984, 0.6619047619047618847, 0.6630952380952380709, 0.6642857142857142572, 0.6654761904761904434, 0.6666666666666666297, 0.6678571428571428159, 0.6690476190476190022, 0.6702380952380951884, 0.6714285714285713746, 0.6726190476190476719, 0.6738095238095238582, 0.6750000000000000444, 0.6761904761904762307, 0.6773809523809524169, 0.6785714285714286031, 0.6797619047619047894, 0.6809523809523809756, 0.6821428571428571619, 0.6833333333333333481, 0.6845238095238095344, 0.6857142857142857206, 0.6869047619047619069, 0.6880952380952380931, 0.6892857142857142794, 0.6904761904761904656, 0.6916666666666666519, 0.6928571428571428381, 0.6940476190476190244, 0.6952380952380952106, 0.6964285714285713969, 0.6976190476190475831, 0.6988095238095237693, 0.6999999999999999556, 0.7011904761904761418, 0.7023809523809523281, 0.7035714285714286254, 0.7047619047619048116, 0.7059523809523809978, 0.7071428571428571841, 0.7083333333333333703, 0.7095238095238095566, 0.7107142857142857428, 0.7119047619047619291, 0.7130952380952381153, 0.7142857142857143016, 0.7154761904761904878, 0.7166666666666666741, 0.7178571428571428603, 0.7190476190476190466, 0.7202380952380952328, 0.7214285714285714191, 0.7226190476190476053, 0.7238095238095237915, 0.7249999999999999778, 0.7261904761904761640, 0.7273809523809523503, 0.7285714285714285365, 0.7297619047619047228, 0.7309523809523809090, 0.7321428571428570953, 0.7333333333333332815, 0.7345238095238095788, 0.7357142857142857650, 0.7369047619047619513, 0.7380952380952381375, 0.7392857142857143238, 0.7404761904761905100, 0.7416666666666666963, 0.7428571428571428825, 0.7440476190476190688, 0.7452380952380952550, 0.7464285714285714413, 0.7476190476190476275, 0.7488095238095238138, 0.7500000000000000000, 0.7511904761904761862, 0.7523809523809523725, 0.7535714285714285587, 0.7547619047619047450, 0.7559523809523809312, 0.7571428571428571175, 0.7583333333333333037, 0.7595238095238094900, 0.7607142857142856762, 0.7619047619047618625, 0.7630952380952380487, 0.7642857142857142350, 0.7654761904761904212, 0.7666666666666667185, 0.7678571428571429047, 0.7690476190476190910, 0.7702380952380952772, 0.7714285714285714635, 0.7726190476190476497, 0.7738095238095238360, 0.7750000000000000222, 0.7761904761904762085, 0.7773809523809523947, 0.7785714285714285809, 0.7797619047619047672, 0.7809523809523809534, 0.7821428571428571397, 0.7833333333333333259, 0.7845238095238095122, 0.7857142857142856984, 0.7869047619047618847, 0.7880952380952380709, 0.7892857142857142572, 0.7904761904761904434, 0.7916666666666666297, 0.7928571428571428159, 0.7940476190476190022, 0.7952380952380951884, 0.7964285714285713746, 0.7976190476190476719, 0.7988095238095238582, 0.8000000000000000444, 0.8011904761904762307, 0.8023809523809524169, 0.8035714285714286031, 0.8047619047619047894, 0.8059523809523809756, 0.8071428571428571619, 0.8083333333333333481, 0.8095238095238095344, 0.8107142857142857206, 0.8119047619047619069, 0.8130952380952380931, 0.8142857142857142794, 0.8154761904761904656, 0.8166666666666666519, 0.8178571428571428381, 0.8190476190476190244, 0.8202380952380952106, 0.8214285714285713969, 0.8226190476190475831, 0.8238095238095237693, 0.8249999999999999556, 0.8261904761904761418, 0.8273809523809523281, 0.8285714285714286254, 0.8297619047619048116, 0.8309523809523809978, 0.8321428571428571841, 0.8333333333333333703, 0.8345238095238095566, 0.8357142857142857428, 0.8369047619047619291, 0.8380952380952381153, 0.8392857142857143016, 0.8404761904761904878, 0.8416666666666666741, 0.8428571428571428603, 0.8440476190476190466, 0.8452380952380952328, 0.8464285714285714191, 0.8476190476190476053, 0.8488095238095237915, 0.8499999999999999778, 0.8511904761904761640, 0.8523809523809523503, 0.8535714285714285365, 0.8547619047619047228, 0.8559523809523809090, 0.8571428571428570953, 0.8583333333333332815, 0.8595238095238095788, 0.8607142857142857650, 0.8619047619047619513, 0.8630952380952381375, 0.8642857142857143238, 0.8654761904761905100, 0.8666666666666666963, 0.8678571428571428825, 0.8690476190476190688, 0.8702380952380952550, 0.8714285714285714413, 0.8726190476190476275, 0.8738095238095238138, 0.8750000000000000000, 0.8761904761904761862, 0.8773809523809523725, 0.8785714285714285587, 0.8797619047619047450, 0.8809523809523809312, 0.8821428571428571175, 0.8833333333333333037, 0.8845238095238094900, 0.8857142857142856762, 0.8869047619047618625, 0.8880952380952380487, 0.8892857142857142350, 0.8904761904761904212, 0.8916666666666667185, 0.8928571428571429047, 0.8940476190476190910, 0.8952380952380952772, 0.8964285714285714635, 0.8976190476190476497, 0.8988095238095238360, 0.9000000000000000222, 0.9011904761904762085, 0.9023809523809523947, 0.9035714285714285809, 0.9047619047619047672, 0.9059523809523809534, 0.9071428571428571397, 0.9083333333333333259, 0.9095238095238095122, 0.9107142857142856984, 0.9119047619047618847, 0.9130952380952380709, 0.9142857142857142572, 0.9154761904761904434, 0.9166666666666666297, 0.9178571428571428159, 0.9190476190476190022, 0.9202380952380951884, 0.9214285714285713746, 0.9226190476190476719, 0.9238095238095238582, 0.9250000000000000444, 0.9261904761904762307, 0.9273809523809524169, 0.9285714285714286031, 0.9297619047619047894, 0.9309523809523809756, 0.9321428571428571619, 0.9333333333333333481, 0.9345238095238095344, 0.9357142857142857206, 0.9369047619047619069, 0.9380952380952380931, 0.9392857142857142794, 0.9404761904761904656, 0.9416666666666666519, 0.9428571428571428381, 0.9440476190476190244, 0.9452380952380952106, 0.9464285714285713969, 0.9476190476190475831, 0.9488095238095237693, 0.9499999999999999556, 0.9511904761904761418, 0.9523809523809523281, 0.9535714285714286254, 0.9547619047619048116, 0.9559523809523809978, 0.9571428571428571841, 0.9583333333333333703, 0.9595238095238095566, 0.9607142857142857428, 0.9619047619047619291, 0.9630952380952381153, 0.9642857142857143016, 0.9654761904761904878, 0.9666666666666666741, 0.9678571428571428603, 0.9690476190476190466, 0.9702380952380952328, 0.9714285714285714191, 0.9726190476190476053, 0.9738095238095237915, 0.9749999999999999778, 0.9761904761904761640, 0.9773809523809523503, 0.9785714285714285365, 0.9797619047619047228, 0.9809523809523809090, 0.9821428571428570953, 0.9833333333333332815, 0.9845238095238095788, 0.9857142857142857650, 0.9869047619047619513, 0.9880952380952381375, 0.9892857142857143238, 0.9904761904761905100, 0.9916666666666666963, 0.9928571428571428825, 0.9940476190476190688, 0.9952380952380952550, 0.9964285714285714413, 0.9976190476190476275, 0.9988095238095238138, 1.000000000000000000 ),
 .UNSPECIFIED. ) 
 GEOMETRIC_REPRESENTATION_ITEM ( )  RATIONAL_B_SPLINE_SURFACE ( (
 ( 1.000000000000000000, 0.8660254037844387076, 1.000000000000000000, 0.8660254037844387076, 1.000000000000000000, 0.8660254037844387076, 1.000000000000000000, 0.8660254037844387076, 1.000000000000000000, 0.8660254037844387076, 1.000000000000000000, 0.8660254037844387076, 1.000000000000000000, 0.8660254037844387076, 1.000000000000000000, 0.8660254037844387076, 1.000000000000000000, 0.8660254037844387076, 1.000000000000000000, 0.8660254037844387076, 1.000000000000000000, 0.8660254037844387076, 1.000000000000000000, 0.8660254037844387076, 1.000000000000000000, 0.8660254037844387076, 1.000000000000000000, 0.8660254037844387076, 1.000000000000000000, 0.8660254037844387076, 1.000000000000000000, 0.8660254037844387076, 1.000000000000000000, 0.8660254037844387076, 1.000000000000000000, 0.8660254037844387076, 1.000000000000000000, 0.8660254037844387076, 1.000000000000000000, 0.8660254037844387076, 1.000000000000000000, 0.8660254037844387076, 1.000000000000000000, 0.8660254037844387076, 1.000000000000000000, 0.8660254037844387076, 1.000000000000000000, 0.8660254037844387076, 1.000000000000000000, 0.8660254037844387076, 1.000000000000000000, 0.8660254037844387076, 1.000000000000000000, 0.8660254037844387076, 1.000000000000000000, 0.8660254037844387076, 1.000000000000000000, 0.8660254037844387076, 1.000000000000000000, 0.8660254037844387076, 1.000000000000000000, 0.8660254037844387076, 1.000000000000000000, 0.8660254037844387076, 1.000000000000000000, 0.8660254037844387076, 1.000000000000000000, 0.8660254037844387076, 1.000000000000000000, 0.8660254037844387076, 1.000000000000000000, 0.8660254037844387076, 1.000000000000000000, 0.8660254037844387076, 1.000000000000000000, 0.8660254037844387076, 1.000000000000000000, 0.8660254037844387076, 1.000000000000000000, 0.8660254037844387076, 1.000000000000000000, 0.8660254037844387076, 1.000000000000000000, 0.8660254037844387076, 1.000000000000000000, 0.8660254037844387076, 1.000000000000000000, 0.8660254037844387076, 1.000000000000000000, 0.8660254037844387076, 1.000000000000000000, 0.8660254037844387076, 1.000000000000000000, 0.8660254037844387076, 1.000000000000000000, 0.8660254037844387076, 1.000000000000000000, 0.8660254037844387076, 1.000000000000000000, 0.8660254037844387076, 1.000000000000000000, 0.8660254037844387076, 1.000000000000000000, 0.8660254037844387076, 1.000000000000000000, 0.8660254037844387076, 1.000000000000000000, 0.8660254037844387076, 1.000000000000000000, 0.8660254037844387076, 1.000000000000000000, 0.8660254037844387076, 1.000000000000000000, 0.8660254037844387076, 1.000000000000000000, 0.8660254037844387076, 1.000000000000000000, 0.8660254037844387076, 1.000000000000000000, 0.8660254037844387076, 1.000000000000000000, 0.8660254037844387076, 1.000000000000000000, 0.8660254037844387076, 1.000000000000000000, 0.8660254037844387076, 1.000000000000000000, 0.8660254037844387076, 1.000000000000000000, 0.8660254037844387076, 1.000000000000000000, 0.8660254037844387076, 1.000000000000000000, 0.8660254037844387076, 1.000000000000000000, 0.8660254037844387076, 1.000000000000000000, 0.8660254037844387076, 1.000000000000000000, 0.8660254037844387076, 1.000000000000000000, 0.8660254037844387076, 1.000000000000000000, 0.8660254037844387076, 1.000000000000000000, 0.8660254037844387076, 1.000000000000000000, 0.8660254037844387076, 1.000000000000000000, 0.8660254037844387076, 1.000000000000000000, 0.8660254037844387076, 1.000000000000000000, 0.8660254037844387076, 1.000000000000000000, 0.8660254037844387076, 1.000000000000000000, 0.8660254037844387076, 1.000000000000000000, 0.8660254037844387076, 1.000000000000000000, 0.8660254037844387076, 1.000000000000000000, 0.8660254037844387076, 1.000000000000000000, 0.8660254037844387076, 1.000000000000000000, 0.8660254037844387076, 1.000000000000000000, 0.8660254037844387076, 1.000000000000000000, 0.8660254037844387076, 1.000000000000000000, 0.8660254037844387076, 1.000000000000000000, 0.8660254037844387076, 1.000000000000000000, 0.8660254037844387076, 1.000000000000000000, 0.8660254037844387076, 1.000000000000000000, 0.8660254037844387076, 1.000000000000000000, 0.8660254037844387076, 1.000000000000000000, 0.8660254037844387076, 1.000000000000000000, 0.8660254037844387076, 1.000000000000000000, 0.8660254037844387076, 1.000000000000000000, 0.8660254037844387076, 1.000000000000000000, 0.8660254037844387076, 1.000000000000000000, 0.8660254037844387076, 1.000000000000000000, 0.8660254037844387076, 1.000000000000000000, 0.8660254037844387076, 1.000000000000000000, 0.8660254037844387076, 1.000000000000000000, 0.8660254037844387076, 1.000000000000000000, 0.8660254037844387076, 1.000000000000000000, 0.8660254037844387076, 1.000000000000000000, 0.8660254037844387076, 1.000000000000000000, 0.8660254037844387076, 1.000000000000000000, 0.8660254037844387076, 1.000000000000000000, 0.8660254037844387076, 1.000000000000000000, 0.8660254037844387076, 1.000000000000000000, 0.8660254037844387076, 1.000000000000000000, 0.8660254037844387076, 1.000000000000000000, 0.8660254037844387076, 1.000000000000000000, 0.8660254037844387076, 1.000000000000000000, 0.8660254037844387076, 1.000000000000000000, 0.8660254037844387076, 1.000000000000000000, 0.8660254037844387076, 1.000000000000000000, 0.8660254037844387076, 1.000000000000000000, 0.8660254037844387076, 1.000000000000000000, 0.8660254037844387076, 1.000000000000000000, 0.8660254037844387076, 1.000000000000000000, 0.8660254037844387076, 1.000000000000000000, 0.8660254037844387076, 1.000000000000000000, 0.8660254037844387076, 1.000000000000000000, 0.8660254037844387076, 1.000000000000000000, 0.8660254037844387076, 1.000000000000000000, 0.8660254037844387076, 1.000000000000000000, 0.8660254037844387076, 1.000000000000000000, 0.8660254037844387076, 1.000000000000000000, 0.8660254037844387076, 1.000000000000000000, 0.8660254037844387076, 1.000000000000000000, 0.8660254037844387076, 1.000000000000000000, 0.8660254037844387076, 1.000000000000000000, 0.8660254037844387076, 1.000000000000000000, 0.8660254037844387076, 1.000000000000000000, 0.8660254037844387076, 1.000000000000000000, 0.8660254037844387076, 1.000000000000000000, 0.8660254037844387076, 1.000000000000000000, 0.8660254037844387076, 1.000000000000000000, 0.8660254037844387076, 1.000000000000000000, 0.8660254037844387076, 1.000000000000000000, 0.8660254037844387076, 1.000000000000000000, 0.8660254037844387076, 1.000000000000000000, 0.8660254037844387076, 1.000000000000000000, 0.8660254037844387076, 1.000000000000000000, 0.8660254037844387076, 1.000000000000000000, 0.8660254037844387076, 1.000000000000000000, 0.8660254037844387076, 1.000000000000000000, 0.8660254037844387076, 1.000000000000000000, 0.8660254037844387076, 1.000000000000000000, 0.8660254037844387076, 1.000000000000000000, 0.8660254037844387076, 1.000000000000000000, 0.8660254037844387076, 1.000000000000000000, 0.8660254037844387076, 1.000000000000000000, 0.8660254037844387076, 1.000000000000000000, 0.8660254037844387076, 1.000000000000000000, 0.8660254037844387076, 1.000000000000000000, 0.8660254037844387076, 1.000000000000000000, 0.8660254037844387076, 1.000000000000000000, 0.8660254037844387076, 1.000000000000000000, 0.8660254037844387076, 1.000000000000000000, 0.8660254037844387076, 1.000000000000000000, 0.8660254037844387076, 1.000000000000000000, 0.8660254037844387076, 1.000000000000000000, 0.8660254037844387076, 1.000000000000000000, 0.8660254037844387076, 1.000000000000000000, 0.8660254037844387076, 1.000000000000000000, 0.8660254037844387076, 1.000000000000000000, 0.8660254037844387076, 1.000000000000000000, 0.8660254037844387076, 1.000000000000000000, 0.8660254037844387076, 1.000000000000000000, 0.8660254037844387076, 1.000000000000000000, 0.8660254037844387076, 1.000000000000000000, 0.8660254037844387076, 1.000000000000000000, 0.8660254037844387076, 1.000000000000000000, 0.8660254037844387076, 1.000000000000000000, 0.8660254037844387076, 1.000000000000000000, 0.8660254037844387076, 1.000000000000000000, 0.8660254037844387076, 1.000000000000000000, 0.8660254037844387076, 1.000000000000000000, 0.8660254037844387076, 1.000000000000000000, 0.8660254037844387076, 1.000000000000000000, 0.8660254037844387076, 1.000000000000000000, 0.8660254037844387076, 1.000000000000000000, 0.8660254037844387076, 1.000000000000000000, 0.8660254037844387076, 1.000000000000000000, 0.8660254037844387076, 1.000000000000000000, 0.8660254037844387076, 1.000000000000000000, 0.8660254037844387076, 1.000000000000000000, 0.8660254037844387076, 1.000000000000000000, 0.8660254037844387076, 1.000000000000000000, 0.8660254037844387076, 1.000000000000000000, 0.8660254037844387076, 1.000000000000000000, 0.8660254037844387076, 1.000000000000000000, 0.8660254037844387076, 1.000000000000000000, 0.8660254037844387076, 1.000000000000000000, 0.8660254037844387076, 1.000000000000000000, 0.8660254037844387076, 1.000000000000000000, 0.8660254037844387076, 1.000000000000000000, 0.8660254037844387076, 1.000000000000000000, 0.8660254037844387076, 1.000000000000000000, 0.8660254037844387076, 1.000000000000000000, 0.8660254037844387076, 1.000000000000000000, 0.8660254037844387076, 1.000000000000000000, 0.8660254037844387076, 1.000000000000000000, 0.8660254037844387076, 1.000000000000000000, 0.8660254037844387076, 1.000000000000000000, 0.8660254037844387076, 1.000000000000000000, 0.8660254037844387076, 1.000000000000000000, 0.8660254037844387076, 1.000000000000000000, 0.8660254037844387076, 1.000000000000000000, 0.8660254037844387076, 1.000000000000000000, 0.8660254037844387076, 1.000000000000000000, 0.8660254037844387076, 1.000000000000000000, 0.8660254037844387076, 1.000000000000000000, 0.8660254037844387076, 1.000000000000000000, 0.8660254037844387076, 1.000000000000000000, 0.8660254037844387076, 1.000000000000000000, 0.8660254037844387076, 1.000000000000000000, 0.8660254037844387076, 1.000000000000000000, 0.8660254037844387076, 1.000000000000000000, 0.8660254037844387076, 1.000000000000000000, 0.8660254037844387076, 1.000000000000000000, 0.8660254037844387076, 1.000000000000000000, 0.8660254037844387076, 1.000000000000000000, 0.8660254037844387076, 1.000000000000000000, 0.8660254037844387076, 1.000000000000000000, 0.8660254037844387076, 1.000000000000000000, 0.8660254037844387076, 1.000000000000000000, 0.8660254037844387076, 1.000000000000000000, 0.8660254037844387076, 1.000000000000000000, 0.8660254037844387076, 1.000000000000000000, 0.8660254037844387076, 1.000000000000000000, 0.8660254037844387076, 1.000000000000000000, 0.8660254037844387076, 1.000000000000000000, 0.8660254037844387076, 1.000000000000000000, 0.8660254037844387076, 1.000000000000000000, 0.8660254037844387076, 1.000000000000000000, 0.8660254037844387076, 1.000000000000000000, 0.8660254037844387076, 1.000000000000000000, 0.8660254037844387076, 1.000000000000000000, 0.8660254037844387076, 1.000000000000000000, 0.8660254037844387076, 1.000000000000000000, 0.8660254037844387076, 1.000000000000000000, 0.8660254037844387076, 1.000000000000000000, 0.8660254037844387076, 1.000000000000000000, 0.8660254037844387076, 1.000000000000000000, 0.8660254037844387076, 1.000000000000000000, 0.8660254037844387076, 1.000000000000000000, 0.8660254037844387076, 1.000000000000000000, 0.8660254037844387076, 1.000000000000000000, 0.8660254037844387076, 1.000000000000000000, 0.8660254037844387076, 1.000000000000000000, 0.8660254037844387076, 1.000000000000000000, 0.8660254037844387076, 1.000000000000000000, 0.8660254037844387076, 1.000000000000000000, 0.8660254037844387076, 1.000000000000000000, 0.8660254037844387076, 1.000000000000000000, 0.8660254037844387076, 1.000000000000000000, 0.8660254037844387076, 1.000000000000000000, 0.8660254037844387076, 1.000000000000000000, 0.8660254037844387076, 1.000000000000000000, 0.8660254037844387076, 1.000000000000000000, 0.8660254037844387076, 1.000000000000000000, 0.8660254037844387076, 1.000000000000000000, 0.8660254037844387076, 1.000000000000000000, 0.8660254037844387076, 1.000000000000000000, 0.8660254037844387076, 1.000000000000000000, 0.8660254037844387076, 1.000000000000000000, 0.8660254037844387076, 1.000000000000000000, 0.8660254037844387076, 1.000000000000000000, 0.8660254037844387076, 1.000000000000000000, 0.8660254037844387076, 1.000000000000000000, 0.8660254037844387076, 1.000000000000000000, 0.8660254037844387076, 1.000000000000000000, 0.8660254037844387076, 1.000000000000000000, 0.8660254037844387076, 1.000000000000000000, 0.8660254037844387076, 1.000000000000000000, 0.8660254037844387076, 1.000000000000000000, 0.8660254037844387076, 1.000000000000000000, 0.8660254037844387076, 1.000000000000000000, 0.8660254037844387076, 1.000000000000000000, 0.8660254037844387076, 1.000000000000000000, 0.8660254037844387076, 1.000000000000000000, 0.8660254037844387076, 1.000000000000000000, 0.8660254037844387076, 1.000000000000000000, 0.8660254037844387076, 1.000000000000000000, 0.8660254037844387076, 1.000000000000000000, 0.8660254037844387076, 1.000000000000000000, 0.8660254037844387076, 1.000000000000000000, 0.8660254037844387076, 1.000000000000000000, 0.8660254037844387076, 1.000000000000000000, 0.8660254037844387076, 1.000000000000000000, 0.8660254037844387076, 1.000000000000000000, 0.8660254037844387076, 1.000000000000000000, 0.8660254037844387076, 1.000000000000000000, 0.8660254037844387076, 1.000000000000000000, 0.8660254037844387076, 1.000000000000000000, 0.8660254037844387076, 1.000000000000000000, 0.8660254037844387076, 1.000000000000000000, 0.8660254037844387076, 1.000000000000000000, 0.8660254037844387076, 1.000000000000000000, 0.8660254037844387076, 1.000000000000000000, 0.8660254037844387076, 1.000000000000000000, 0.8660254037844387076, 1.000000000000000000, 0.8660254037844387076, 1.000000000000000000, 0.8660254037844387076, 1.000000000000000000, 0.8660254037844387076, 1.000000000000000000, 0.8660254037844387076, 1.000000000000000000, 0.8660254037844387076, 1.000000000000000000, 0.8660254037844387076, 1.000000000000000000, 0.8660254037844387076, 1.000000000000000000, 0.8660254037844387076, 1.000000000000000000, 0.8660254037844387076, 1.000000000000000000, 0.8660254037844387076, 1.000000000000000000, 0.8660254037844387076, 1.000000000000000000, 0.8660254037844387076, 1.000000000000000000, 0.8660254037844387076, 1.000000000000000000, 0.8660254037844387076, 1.000000000000000000, 0.8660254037844387076, 1.000000000000000000, 0.8660254037844387076, 1.000000000000000000, 0.8660254037844387076, 1.000000000000000000, 0.8660254037844387076, 1.000000000000000000, 0.8660254037844387076, 1.000000000000000000, 0.8660254037844387076, 1.000000000000000000, 0.8660254037844387076, 1.000000000000000000, 0.8660254037844387076, 1.000000000000000000, 0.8660254037844387076, 1.000000000000000000, 0.8660254037844387076, 1.000000000000000000, 0.8660254037844387076, 1.000000000000000000, 0.8660254037844387076, 1.000000000000000000, 0.8660254037844387076, 1.000000000000000000, 0.8660254037844387076, 1.000000000000000000, 0.8660254037844387076, 1.000000000000000000, 0.8660254037844387076, 1.000000000000000000, 0.8660254037844387076, 1.000000000000000000, 0.8660254037844387076, 1.000000000000000000, 0.8660254037844387076, 1.000000000000000000, 0.8660254037844387076, 1.000000000000000000, 0.8660254037844387076, 1.000000000000000000, 0.8660254037844387076, 1.000000000000000000, 0.8660254037844387076, 1.000000000000000000, 0.8660254037844387076, 1.000000000000000000, 0.8660254037844387076, 1.000000000000000000, 0.8660254037844387076, 1.000000000000000000, 0.8660254037844387076, 1.000000000000000000, 0.8660254037844387076, 1.000000000000000000, 0.8660254037844387076, 1.000000000000000000, 0.8660254037844387076, 1.000000000000000000, 0.8660254037844387076, 1.000000000000000000, 0.8660254037844387076, 1.000000000000000000, 0.8660254037844387076, 1.000000000000000000, 0.8660254037844387076, 1.000000000000000000, 0.8660254037844387076, 1.000000000000000000, 0.8660254037844387076, 1.000000000000000000, 0.8660254037844387076, 1.000000000000000000, 0.8660254037844387076, 1.000000000000000000, 0.8660254037844387076, 1.000000000000000000, 0.8660254037844387076, 1.000000000000000000, 0.8660254037844387076, 1.000000000000000000, 0.8660254037844387076, 1.000000000000000000, 0.8660254037844387076, 1.000000000000000000, 0.8660254037844387076, 1.000000000000000000, 0.8660254037844387076, 1.000000000000000000, 0.8660254037844387076, 1.000000000000000000, 0.8660254037844387076, 1.000000000000000000, 0.8660254037844387076, 1.000000000000000000, 0.8660254037844387076, 1.000000000000000000, 0.8660254037844387076, 1.000000000000000000, 0.8660254037844387076, 1.000000000000000000, 0.8660254037844387076, 1.000000000000000000, 0.8660254037844387076, 1.000000000000000000, 0.8660254037844387076, 1.000000000000000000, 0.8660254037844387076, 1.000000000000000000, 0.8660254037844387076, 1.000000000000000000, 0.8660254037844387076, 1.000000000000000000, 0.8660254037844387076, 1.000000000000000000, 0.8660254037844387076, 1.000000000000000000, 0.8660254037844387076, 1.000000000000000000, 0.8660254037844387076, 1.000000000000000000, 0.8660254037844387076, 1.000000000000000000, 0.8660254037844387076, 1.000000000000000000, 0.8660254037844387076, 1.000000000000000000, 0.8660254037844387076, 1.000000000000000000, 0.8660254037844387076, 1.000000000000000000, 0.8660254037844387076, 1.000000000000000000, 0.8660254037844387076, 1.000000000000000000, 0.8660254037844387076, 1.000000000000000000, 0.8660254037844387076, 1.000000000000000000, 0.8660254037844387076, 1.000000000000000000, 0.8660254037844387076, 1.000000000000000000, 0.8660254037844387076, 1.000000000000000000, 0.8660254037844387076, 1.000000000000000000, 0.8660254037844387076, 1.000000000000000000, 0.8660254037844387076, 1.000000000000000000, 0.8660254037844387076, 1.000000000000000000, 0.8660254037844387076, 1.000000000000000000, 0.8660254037844387076, 1.000000000000000000, 0.8660254037844387076, 1.000000000000000000, 0.8660254037844387076, 1.000000000000000000, 0.8660254037844387076, 1.000000000000000000, 0.8660254037844387076, 1.000000000000000000, 0.8660254037844387076, 1.000000000000000000, 0.8660254037844387076, 1.000000000000000000, 0.8660254037844387076, 1.000000000000000000, 0.8660254037844387076, 1.000000000000000000, 0.8660254037844387076, 1.000000000000000000, 0.8660254037844387076, 1.000000000000000000, 0.8660254037844387076, 1.000000000000000000, 0.8660254037844387076, 1.000000000000000000, 0.8660254037844387076, 1.000000000000000000, 0.8660254037844387076, 1.000000000000000000, 0.8660254037844387076, 1.000000000000000000, 0.8660254037844387076, 1.000000000000000000, 0.8660254037844387076, 1.000000000000000000, 0.8660254037844387076, 1.000000000000000000, 0.8660254037844387076, 1.000000000000000000, 0.8660254037844387076, 1.000000000000000000, 0.8660254037844387076, 1.000000000000000000, 0.8660254037844387076, 1.000000000000000000, 0.8660254037844387076, 1.000000000000000000, 0.8660254037844387076, 1.000000000000000000, 0.8660254037844387076, 1.000000000000000000, 0.8660254037844387076, 1.000000000000000000, 0.8660254037844387076, 1.000000000000000000, 0.8660254037844387076, 1.000000000000000000, 0.8660254037844387076, 1.000000000000000000, 0.8660254037844387076, 1.000000000000000000, 0.8660254037844387076, 1.000000000000000000, 0.8660254037844387076, 1.000000000000000000, 0.8660254037844387076, 1.000000000000000000, 0.8660254037844387076, 1.000000000000000000, 0.8660254037844387076, 1.000000000000000000, 0.8660254037844387076, 1.000000000000000000, 0.8660254037844387076, 1.000000000000000000, 0.8660254037844387076, 1.000000000000000000, 0.8660254037844387076, 1.000000000000000000, 0.8660254037844387076, 1.000000000000000000, 0.8660254037844387076, 1.000000000000000000, 0.8660254037844387076, 1.000000000000000000, 0.8660254037844387076, 1.000000000000000000, 0.8660254037844387076, 1.000000000000000000, 0.8660254037844387076, 1.000000000000000000, 0.8660254037844387076, 1.000000000000000000, 0.8660254037844387076, 1.000000000000000000, 0.8660254037844387076, 1.000000000000000000, 0.8660254037844387076, 1.000000000000000000, 0.8660254037844387076, 1.000000000000000000, 0.8660254037844387076, 1.000000000000000000, 0.8660254037844387076, 1.000000000000000000, 0.8660254037844387076, 1.000000000000000000, 0.8660254037844387076, 1.000000000000000000, 0.8660254037844387076, 1.000000000000000000, 0.8660254037844387076, 1.000000000000000000, 0.8660254037844387076, 1.000000000000000000, 0.8660254037844387076, 1.000000000000000000, 0.8660254037844387076, 1.000000000000000000, 0.8660254037844387076, 1.000000000000000000, 0.8660254037844387076, 1.000000000000000000, 0.8660254037844387076, 1.000000000000000000, 0.8660254037844387076, 1.000000000000000000, 0.8660254037844387076, 1.000000000000000000, 0.8660254037844387076, 1.000000000000000000, 0.8660254037844387076, 1.000000000000000000, 0.8660254037844387076, 1.000000000000000000, 0.8660254037844387076, 1.000000000000000000, 0.8660254037844387076, 1.000000000000000000, 0.8660254037844387076, 1.000000000000000000, 0.8660254037844387076, 1.000000000000000000, 0.8660254037844387076, 1.000000000000000000, 0.8660254037844387076, 1.000000000000000000, 0.8660254037844387076, 1.000000000000000000, 0.8660254037844387076, 1.000000000000000000, 0.8660254037844387076, 1.000000000000000000, 0.8660254037844387076, 1.000000000000000000, 0.8660254037844387076, 1.000000000000000000, 0.8660254037844387076, 1.000000000000000000, 0.8660254037844387076, 1.000000000000000000, 0.8660254037844387076, 1.000000000000000000, 0.8660254037844387076, 1.000000000000000000, 0.8660254037844387076, 1.000000000000000000, 0.8660254037844387076, 1.000000000000000000, 0.8660254037844387076, 1.000000000000000000, 0.8660254037844387076, 1.000000000000000000, 0.8660254037844387076, 1.000000000000000000, 0.8660254037844387076, 1.000000000000000000, 0.8660254037844387076, 1.000000000000000000, 0.8660254037844387076, 1.000000000000000000, 0.8660254037844387076, 1.000000000000000000, 0.8660254037844387076, 1.000000000000000000, 0.8660254037844387076, 1.000000000000000000, 0.8660254037844387076, 1.000000000000000000, 0.8660254037844387076, 1.000000000000000000, 0.8660254037844387076, 1.000000000000000000, 0.8660254037844387076, 1.000000000000000000, 0.8660254037844387076, 1.000000000000000000, 0.8660254037844387076, 1.000000000000000000, 0.8660254037844387076, 1.000000000000000000, 0.8660254037844387076, 1.000000000000000000, 0.8660254037844387076, 1.000000000000000000, 0.8660254037844387076, 1.000000000000000000, 0.8660254037844387076, 1.000000000000000000, 0.8660254037844387076, 1.000000000000000000, 0.8660254037844387076, 1.000000000000000000, 0.8660254037844387076, 1.000000000000000000, 0.8660254037844387076, 1.000000000000000000, 0.8660254037844387076, 1.000000000000000000, 0.8660254037844387076, 1.000000000000000000, 0.8660254037844387076, 1.000000000000000000, 0.8660254037844387076, 1.000000000000000000, 0.8660254037844387076, 1.000000000000000000, 0.8660254037844387076, 1.000000000000000000, 0.8660254037844387076, 1.000000000000000000, 0.8660254037844387076, 1.000000000000000000, 0.8660254037844387076, 1.000000000000000000, 0.8660254037844387076, 1.000000000000000000, 0.8660254037844387076, 1.000000000000000000, 0.8660254037844387076, 1.000000000000000000, 0.8660254037844387076, 1.000000000000000000, 0.8660254037844387076, 1.000000000000000000, 0.8660254037844387076, 1.000000000000000000, 0.8660254037844387076, 1.000000000000000000, 0.8660254037844387076, 1.000000000000000000, 0.8660254037844387076, 1.000000000000000000, 0.8660254037844387076, 1.000000000000000000, 0.8660254037844387076, 1.000000000000000000, 0.8660254037844387076, 1.000000000000000000, 0.8660254037844387076, 1.000000000000000000, 0.8660254037844387076, 1.000000000000000000, 0.8660254037844387076, 1.000000000000000000, 0.8660254037844387076, 1.000000000000000000, 0.8660254037844387076, 1.000000000000000000, 0.8660254037844387076, 1.000000000000000000, 0.8660254037844387076, 1.000000000000000000, 0.8660254037844387076, 1.000000000000000000, 0.8660254037844387076, 1.000000000000000000, 0.8660254037844387076, 1.000000000000000000, 0.8660254037844387076, 1.000000000000000000, 0.8660254037844387076, 1.000000000000000000, 0.8660254037844387076, 1.000000000000000000, 0.8660254037844387076, 1.000000000000000000, 0.8660254037844387076, 1.000000000000000000, 0.8660254037844387076, 1.000000000000000000, 0.8660254037844387076, 1.000000000000000000, 0.8660254037844387076, 1.000000000000000000, 0.8660254037844387076, 1.000000000000000000, 0.8660254037844387076, 1.000000000000000000, 0.8660254037844387076, 1.000000000000000000, 0.8660254037844387076, 1.000000000000000000, 0.8660254037844387076, 1.000000000000000000, 0.8660254037844387076, 1.000000000000000000, 0.8660254037844387076, 1.000000000000000000, 0.8660254037844387076, 1.000000000000000000, 0.8660254037844387076, 1.000000000000000000, 0.8660254037844387076, 1.000000000000000000, 0.8660254037844387076, 1.000000000000000000, 0.8660254037844387076, 1.000000000000000000, 0.8660254037844387076, 1.000000000000000000, 0.8660254037844387076, 1.000000000000000000, 0.8660254037844387076, 1.000000000000000000, 0.8660254037844387076, 1.000000000000000000, 0.8660254037844387076, 1.000000000000000000, 0.8660254037844387076, 1.000000000000000000, 0.8660254037844387076, 1.000000000000000000, 0.8660254037844387076, 1.000000000000000000, 0.8660254037844387076, 1.000000000000000000, 0.8660254037844387076, 1.000000000000000000, 0.8660254037844387076, 1.000000000000000000, 0.8660254037844387076, 1.000000000000000000, 0.8660254037844387076, 1.000000000000000000, 0.8660254037844387076, 1.000000000000000000, 0.8660254037844387076, 1.000000000000000000, 0.8660254037844387076, 1.000000000000000000, 0.8660254037844387076, 1.000000000000000000, 0.8660254037844387076, 1.000000000000000000, 0.8660254037844387076, 1.000000000000000000, 0.8660254037844387076, 1.000000000000000000, 0.8660254037844387076, 1.000000000000000000, 0.8660254037844387076, 1.000000000000000000, 0.8660254037844387076, 1.000000000000000000, 0.8660254037844387076, 1.000000000000000000, 0.8660254037844387076, 1.000000000000000000, 0.8660254037844387076, 1.000000000000000000, 0.8660254037844387076, 1.000000000000000000, 0.8660254037844387076, 1.000000000000000000, 0.8660254037844387076, 1.000000000000000000, 0.8660254037844387076, 1.000000000000000000, 0.8660254037844387076, 1.000000000000000000, 0.8660254037844387076, 1.000000000000000000, 0.8660254037844387076, 1.000000000000000000, 0.8660254037844387076, 1.000000000000000000, 0.8660254037844387076, 1.000000000000000000, 0.8660254037844387076, 1.000000000000000000, 0.8660254037844387076, 1.000000000000000000, 0.8660254037844387076, 1.000000000000000000, 0.8660254037844387076, 1.000000000000000000, 0.8660254037844387076, 1.000000000000000000, 0.8660254037844387076, 1.000000000000000000, 0.8660254037844387076, 1.000000000000000000, 0.8660254037844387076, 1.000000000000000000, 0.8660254037844387076, 1.000000000000000000, 0.8660254037844387076, 1.000000000000000000, 0.8660254037844387076, 1.000000000000000000, 0.8660254037844387076, 1.000000000000000000, 0.8660254037844387076, 1.000000000000000000, 0.8660254037844387076, 1.000000000000000000, 0.8660254037844387076, 1.000000000000000000, 0.8660254037844387076, 1.000000000000000000, 0.8660254037844387076, 1.000000000000000000, 0.8660254037844387076, 1.000000000000000000, 0.8660254037844387076, 1.000000000000000000, 0.8660254037844387076, 1.000000000000000000, 0.8660254037844387076, 1.000000000000000000, 0.8660254037844387076, 1.000000000000000000, 0.8660254037844387076, 1.000000000000000000, 0.8660254037844387076, 1.000000000000000000, 0.8660254037844387076, 1.000000000000000000, 0.8660254037844387076, 1.000000000000000000, 0.8660254037844387076, 1.000000000000000000, 0.8660254037844387076, 1.000000000000000000, 0.8660254037844387076, 1.000000000000000000, 0.8660254037844387076, 1.000000000000000000, 0.8660254037844387076, 1.000000000000000000, 0.8660254037844387076, 1.000000000000000000, 0.8660254037844387076, 1.000000000000000000, 0.8660254037844387076, 1.000000000000000000, 0.8660254037844387076, 1.000000000000000000, 0.8660254037844387076, 1.000000000000000000, 0.8660254037844387076, 1.000000000000000000, 0.8660254037844387076, 1.000000000000000000, 0.8660254037844387076, 1.000000000000000000, 0.8660254037844387076, 1.000000000000000000, 0.8660254037844387076, 1.000000000000000000, 0.8660254037844387076, 1.000000000000000000, 0.8660254037844387076, 1.000000000000000000, 0.8660254037844387076, 1.000000000000000000, 0.8660254037844387076, 1.000000000000000000, 0.8660254037844387076, 1.000000000000000000, 0.8660254037844387076, 1.000000000000000000, 0.8660254037844387076, 1.000000000000000000, 0.8660254037844387076, 1.000000000000000000, 0.8660254037844387076, 1.000000000000000000, 0.8660254037844387076, 1.000000000000000000, 0.8660254037844387076, 1.000000000000000000, 0.8660254037844387076, 1.000000000000000000, 0.8660254037844387076, 1.000000000000000000, 0.8660254037844387076, 1.000000000000000000, 0.8660254037844387076, 1.000000000000000000, 0.8660254037844387076, 1.000000000000000000, 0.8660254037844387076, 1.000000000000000000, 0.8660254037844387076, 1.000000000000000000, 0.8660254037844387076, 1.000000000000000000, 0.8660254037844387076, 1.000000000000000000, 0.8660254037844387076, 1.000000000000000000, 0.8660254037844387076, 1.000000000000000000, 0.8660254037844387076, 1.000000000000000000, 0.8660254037844387076, 1.000000000000000000, 0.8660254037844387076, 1.000000000000000000, 0.8660254037844387076, 1.000000000000000000, 0.8660254037844387076, 1.000000000000000000, 0.8660254037844387076, 1.000000000000000000, 0.8660254037844387076, 1.000000000000000000, 0.8660254037844387076, 1.000000000000000000, 0.8660254037844387076, 1.000000000000000000, 0.8660254037844387076, 1.000000000000000000, 0.8660254037844387076, 1.000000000000000000, 0.8660254037844387076, 1.000000000000000000, 0.8660254037844387076, 1.000000000000000000, 0.8660254037844387076, 1.000000000000000000, 0.8660254037844387076, 1.000000000000000000, 0.8660254037844387076, 1.000000000000000000, 0.8660254037844387076, 1.000000000000000000, 0.8660254037844387076, 1.000000000000000000, 0.8660254037844387076, 1.000000000000000000, 0.8660254037844387076, 1.000000000000000000, 0.8660254037844387076, 1.000000000000000000, 0.8660254037844387076, 1.000000000000000000, 0.8660254037844387076, 1.000000000000000000, 0.8660254037844387076, 1.000000000000000000, 0.8660254037844387076, 1.000000000000000000, 0.8660254037844387076, 1.000000000000000000, 0.8660254037844387076, 1.000000000000000000, 0.8660254037844387076, 1.000000000000000000, 0.8660254037844387076, 1.000000000000000000, 0.8660254037844387076, 1.000000000000000000, 0.8660254037844387076, 1.000000000000000000, 0.8660254037844387076, 1.000000000000000000, 0.8660254037844387076, 1.000000000000000000, 0.8660254037844387076, 1.000000000000000000, 0.8660254037844387076, 1.000000000000000000, 0.8660254037844387076, 1.000000000000000000, 0.8660254037844387076, 1.000000000000000000, 0.8660254037844387076, 1.000000000000000000, 0.8660254037844387076, 1.000000000000000000, 0.8660254037844387076, 1.000000000000000000, 0.8660254037844387076, 1.000000000000000000, 0.8660254037844387076, 1.000000000000000000, 0.8660254037844387076, 1.000000000000000000, 0.8660254037844387076, 1.000000000000000000, 0.8660254037844387076, 1.000000000000000000, 0.8660254037844387076, 1.000000000000000000, 0.8660254037844387076, 1.000000000000000000, 0.8660254037844387076, 1.000000000000000000, 0.8660254037844387076, 1.000000000000000000, 0.8660254037844387076, 1.000000000000000000, 0.8660254037844387076, 1.000000000000000000, 0.8660254037844387076, 1.000000000000000000, 0.8660254037844387076, 1.000000000000000000, 0.8660254037844387076, 1.000000000000000000, 0.8660254037844387076, 1.000000000000000000, 0.8660254037844387076, 1.000000000000000000, 0.8660254037844387076, 1.000000000000000000, 0.8660254037844387076, 1.000000000000000000, 0.8660254037844387076, 1.000000000000000000, 0.8660254037844387076, 1.000000000000000000, 0.8660254037844387076, 1.000000000000000000, 0.8660254037844387076, 1.000000000000000000, 0.8660254037844387076, 1.000000000000000000, 0.8660254037844387076, 1.000000000000000000, 0.8660254037844387076, 1.000000000000000000, 0.8660254037844387076, 1.000000000000000000, 0.8660254037844387076, 1.000000000000000000, 0.8660254037844387076, 1.000000000000000000, 0.8660254037844387076, 1.000000000000000000, 0.8660254037844387076, 1.000000000000000000, 0.8660254037844387076, 1.000000000000000000, 0.8660254037844387076, 1.000000000000000000, 0.8660254037844387076, 1.000000000000000000, 0.8660254037844387076, 1.000000000000000000, 0.8660254037844387076, 1.000000000000000000, 0.8660254037844387076, 1.000000000000000000, 0.8660254037844387076, 1.000000000000000000, 0.8660254037844387076, 1.000000000000000000, 0.8660254037844387076, 1.000000000000000000, 0.8660254037844387076, 1.000000000000000000, 0.8660254037844387076, 1.000000000000000000, 0.8660254037844387076, 1.000000000000000000, 0.8660254037844387076, 1.000000000000000000, 0.8660254037844387076, 1.000000000000000000, 0.8660254037844387076, 1.000000000000000000, 0.8660254037844387076, 1.000000000000000000, 0.8660254037844387076, 1.000000000000000000, 0.8660254037844387076, 1.000000000000000000, 0.8660254037844387076, 1.000000000000000000, 0.8660254037844387076, 1.000000000000000000, 0.8660254037844387076, 1.000000000000000000, 0.8660254037844387076, 1.000000000000000000, 0.8660254037844387076, 1.000000000000000000, 0.8660254037844387076, 1.000000000000000000, 0.8660254037844387076, 1.000000000000000000, 0.8660254037844387076, 1.000000000000000000, 0.8660254037844387076, 1.000000000000000000, 0.8660254037844387076, 1.000000000000000000, 0.8660254037844387076, 1.000000000000000000, 0.8660254037844387076, 1.000000000000000000, 0.8660254037844387076, 1.000000000000000000, 0.8660254037844387076, 1.000000000000000000, 0.8660254037844387076, 1.000000000000000000, 0.8660254037844387076, 1.000000000000000000, 0.8660254037844387076, 1.000000000000000000, 0.8660254037844387076, 1.000000000000000000, 0.8660254037844387076, 1.000000000000000000, 0.8660254037844387076, 1.000000000000000000, 0.8660254037844387076, 1.000000000000000000, 0.8660254037844387076, 1.000000000000000000, 0.8660254037844387076, 1.000000000000000000, 0.8660254037844387076, 1.000000000000000000, 0.8660254037844387076, 1.000000000000000000, 0.8660254037844387076, 1.000000000000000000, 0.8660254037844387076, 1.000000000000000000, 0.8660254037844387076, 1.000000000000000000, 0.8660254037844387076, 1.000000000000000000, 0.8660254037844387076, 1.000000000000000000, 0.8660254037844387076, 1.000000000000000000, 0.8660254037844387076, 1.000000000000000000, 0.8660254037844387076, 1.000000000000000000, 0.8660254037844387076, 1.000000000000000000, 0.8660254037844387076, 1.000000000000000000, 0.8660254037844387076, 1.000000000000000000, 0.8660254037844387076, 1.000000000000000000, 0.8660254037844387076, 1.000000000000000000, 0.8660254037844387076, 1.000000000000000000, 0.8660254037844387076, 1.000000000000000000, 0.8660254037844387076, 1.000000000000000000, 0.8660254037844387076, 1.000000000000000000, 0.8660254037844387076, 1.000000000000000000, 0.8660254037844387076, 1.000000000000000000, 0.8660254037844387076, 1.000000000000000000, 0.8660254037844387076, 1.000000000000000000, 0.8660254037844387076, 1.000000000000000000, 0.8660254037844387076, 1.000000000000000000, 0.8660254037844387076, 1.000000000000000000, 0.8660254037844387076, 1.000000000000000000, 0.8660254037844387076, 1.000000000000000000, 0.8660254037844387076, 1.000000000000000000, 0.8660254037844387076, 1.000000000000000000, 0.8660254037844387076, 1.000000000000000000, 0.8660254037844387076, 1.000000000000000000, 0.8660254037844387076, 1.000000000000000000, 0.8660254037844387076, 1.000000000000000000, 0.8660254037844387076, 1.000000000000000000, 0.8660254037844387076, 1.000000000000000000, 0.8660254037844387076, 1.000000000000000000, 0.8660254037844387076, 1.000000000000000000, 0.8660254037844387076, 1.000000000000000000, 0.8660254037844387076, 1.000000000000000000, 0.8660254037844387076, 1.000000000000000000, 0.8660254037844387076, 1.000000000000000000, 0.8660254037844387076, 1.000000000000000000, 0.8660254037844387076, 1.000000000000000000, 0.8660254037844387076, 1.000000000000000000, 0.8660254037844387076, 1.000000000000000000, 0.8660254037844387076, 1.000000000000000000, 0.8660254037844387076, 1.000000000000000000, 0.8660254037844387076, 1.000000000000000000, 0.8660254037844387076, 1.000000000000000000, 0.8660254037844387076, 1.000000000000000000, 0.8660254037844387076, 1.000000000000000000, 0.8660254037844387076, 1.000000000000000000, 0.8660254037844387076, 1.000000000000000000, 0.8660254037844387076, 1.000000000000000000, 0.8660254037844387076, 1.000000000000000000, 0.8660254037844387076, 1.000000000000000000, 0.8660254037844387076, 1.000000000000000000, 0.8660254037844387076, 1.000000000000000000, 0.8660254037844387076, 1.000000000000000000, 0.8660254037844387076, 1.000000000000000000, 0.8660254037844387076, 1.000000000000000000, 0.8660254037844387076, 1.000000000000000000, 0.8660254037844387076, 1.000000000000000000, 0.8660254037844387076, 1.000000000000000000, 0.8660254037844387076, 1.000000000000000000, 0.8660254037844387076, 1.000000000000000000, 0.8660254037844387076, 1.000000000000000000, 0.8660254037844387076, 1.000000000000000000, 0.8660254037844387076, 1.000000000000000000, 0.8660254037844387076, 1.000000000000000000, 0.8660254037844387076, 1.000000000000000000, 0.8660254037844387076, 1.000000000000000000, 0.8660254037844387076, 1.000000000000000000, 0.8660254037844387076, 1.000000000000000000),
 ( 1.000000000000000000, 0.8660254037844387076, 1.000000000000000000, 0.8660254037844387076, 1.000000000000000000, 0.8660254037844387076, 1.000000000000000000, 0.8660254037844387076, 1.000000000000000000, 0.8660254037844387076, 1.000000000000000000, 0.8660254037844387076, 1.000000000000000000, 0.8660254037844387076, 1.000000000000000000, 0.8660254037844387076, 1.000000000000000000, 0.8660254037844387076, 1.000000000000000000, 0.8660254037844387076, 1.000000000000000000, 0.8660254037844387076, 1.000000000000000000, 0.8660254037844387076, 1.000000000000000000, 0.8660254037844387076, 1.000000000000000000, 0.8660254037844387076, 1.000000000000000000, 0.8660254037844387076, 1.000000000000000000, 0.8660254037844387076, 1.000000000000000000, 0.8660254037844387076, 1.000000000000000000, 0.8660254037844387076, 1.000000000000000000, 0.8660254037844387076, 1.000000000000000000, 0.8660254037844387076, 1.000000000000000000, 0.8660254037844387076, 1.000000000000000000, 0.8660254037844387076, 1.000000000000000000, 0.8660254037844387076, 1.000000000000000000, 0.8660254037844387076, 1.000000000000000000, 0.8660254037844387076, 1.000000000000000000, 0.8660254037844387076, 1.000000000000000000, 0.8660254037844387076, 1.000000000000000000, 0.8660254037844387076, 1.000000000000000000, 0.8660254037844387076, 1.000000000000000000, 0.8660254037844387076, 1.000000000000000000, 0.8660254037844387076, 1.000000000000000000, 0.8660254037844387076, 1.000000000000000000, 0.8660254037844387076, 1.000000000000000000, 0.8660254037844387076, 1.000000000000000000, 0.8660254037844387076, 1.000000000000000000, 0.8660254037844387076, 1.000000000000000000, 0.8660254037844387076, 1.000000000000000000, 0.8660254037844387076, 1.000000000000000000, 0.8660254037844387076, 1.000000000000000000, 0.8660254037844387076, 1.000000000000000000, 0.8660254037844387076, 1.000000000000000000, 0.8660254037844387076, 1.000000000000000000, 0.8660254037844387076, 1.000000000000000000, 0.8660254037844387076, 1.000000000000000000, 0.8660254037844387076, 1.000000000000000000, 0.8660254037844387076, 1.000000000000000000, 0.8660254037844387076, 1.000000000000000000, 0.8660254037844387076, 1.000000000000000000, 0.8660254037844387076, 1.000000000000000000, 0.8660254037844387076, 1.000000000000000000, 0.8660254037844387076, 1.000000000000000000, 0.8660254037844387076, 1.000000000000000000, 0.8660254037844387076, 1.000000000000000000, 0.8660254037844387076, 1.000000000000000000, 0.8660254037844387076, 1.000000000000000000, 0.8660254037844387076, 1.000000000000000000, 0.8660254037844387076, 1.000000000000000000, 0.8660254037844387076, 1.000000000000000000, 0.8660254037844387076, 1.000000000000000000, 0.8660254037844387076, 1.000000000000000000, 0.8660254037844387076, 1.000000000000000000, 0.8660254037844387076, 1.000000000000000000, 0.8660254037844387076, 1.000000000000000000, 0.8660254037844387076, 1.000000000000000000, 0.8660254037844387076, 1.000000000000000000, 0.8660254037844387076, 1.000000000000000000, 0.8660254037844387076, 1.000000000000000000, 0.8660254037844387076, 1.000000000000000000, 0.8660254037844387076, 1.000000000000000000, 0.8660254037844387076, 1.000000000000000000, 0.8660254037844387076, 1.000000000000000000, 0.8660254037844387076, 1.000000000000000000, 0.8660254037844387076, 1.000000000000000000, 0.8660254037844387076, 1.000000000000000000, 0.8660254037844387076, 1.000000000000000000, 0.8660254037844387076, 1.000000000000000000, 0.8660254037844387076, 1.000000000000000000, 0.8660254037844387076, 1.000000000000000000, 0.8660254037844387076, 1.000000000000000000, 0.8660254037844387076, 1.000000000000000000, 0.8660254037844387076, 1.000000000000000000, 0.8660254037844387076, 1.000000000000000000, 0.8660254037844387076, 1.000000000000000000, 0.8660254037844387076, 1.000000000000000000, 0.8660254037844387076, 1.000000000000000000, 0.8660254037844387076, 1.000000000000000000, 0.8660254037844387076, 1.000000000000000000, 0.8660254037844387076, 1.000000000000000000, 0.8660254037844387076, 1.000000000000000000, 0.8660254037844387076, 1.000000000000000000, 0.8660254037844387076, 1.000000000000000000, 0.8660254037844387076, 1.000000000000000000, 0.8660254037844387076, 1.000000000000000000, 0.8660254037844387076, 1.000000000000000000, 0.8660254037844387076, 1.000000000000000000, 0.8660254037844387076, 1.000000000000000000, 0.8660254037844387076, 1.000000000000000000, 0.8660254037844387076, 1.000000000000000000, 0.8660254037844387076, 1.000000000000000000, 0.8660254037844387076, 1.000000000000000000, 0.8660254037844387076, 1.000000000000000000, 0.8660254037844387076, 1.000000000000000000, 0.8660254037844387076, 1.000000000000000000, 0.8660254037844387076, 1.000000000000000000, 0.8660254037844387076, 1.000000000000000000, 0.8660254037844387076, 1.000000000000000000, 0.8660254037844387076, 1.000000000000000000, 0.8660254037844387076, 1.000000000000000000, 0.8660254037844387076, 1.000000000000000000, 0.8660254037844387076, 1.000000000000000000, 0.8660254037844387076, 1.000000000000000000, 0.8660254037844387076, 1.000000000000000000, 0.8660254037844387076, 1.000000000000000000, 0.8660254037844387076, 1.000000000000000000, 0.8660254037844387076, 1.000000000000000000, 0.8660254037844387076, 1.000000000000000000, 0.8660254037844387076, 1.000000000000000000, 0.8660254037844387076, 1.000000000000000000, 0.8660254037844387076, 1.000000000000000000, 0.8660254037844387076, 1.000000000000000000, 0.8660254037844387076, 1.000000000000000000, 0.8660254037844387076, 1.000000000000000000, 0.8660254037844387076, 1.000000000000000000, 0.8660254037844387076, 1.000000000000000000, 0.8660254037844387076, 1.000000000000000000, 0.8660254037844387076, 1.000000000000000000, 0.8660254037844387076, 1.000000000000000000, 0.8660254037844387076, 1.000000000000000000, 0.8660254037844387076, 1.000000000000000000, 0.8660254037844387076, 1.000000000000000000, 0.8660254037844387076, 1.000000000000000000, 0.8660254037844387076, 1.000000000000000000, 0.8660254037844387076, 1.000000000000000000, 0.8660254037844387076, 1.000000000000000000, 0.8660254037844387076, 1.000000000000000000, 0.8660254037844387076, 1.000000000000000000, 0.8660254037844387076, 1.000000000000000000, 0.8660254037844387076, 1.000000000000000000, 0.8660254037844387076, 1.000000000000000000, 0.8660254037844387076, 1.000000000000000000, 0.8660254037844387076, 1.000000000000000000, 0.8660254037844387076, 1.000000000000000000, 0.8660254037844387076, 1.000000000000000000, 0.8660254037844387076, 1.000000000000000000, 0.8660254037844387076, 1.000000000000000000, 0.8660254037844387076, 1.000000000000000000, 0.8660254037844387076, 1.000000000000000000, 0.8660254037844387076, 1.000000000000000000, 0.8660254037844387076, 1.000000000000000000, 0.8660254037844387076, 1.000000000000000000, 0.8660254037844387076, 1.000000000000000000, 0.8660254037844387076, 1.000000000000000000, 0.8660254037844387076, 1.000000000000000000, 0.8660254037844387076, 1.000000000000000000, 0.8660254037844387076, 1.000000000000000000, 0.8660254037844387076, 1.000000000000000000, 0.8660254037844387076, 1.000000000000000000, 0.8660254037844387076, 1.000000000000000000, 0.8660254037844387076, 1.000000000000000000, 0.8660254037844387076, 1.000000000000000000, 0.8660254037844387076, 1.000000000000000000, 0.8660254037844387076, 1.000000000000000000, 0.8660254037844387076, 1.000000000000000000, 0.8660254037844387076, 1.000000000000000000, 0.8660254037844387076, 1.000000000000000000, 0.8660254037844387076, 1.000000000000000000, 0.8660254037844387076, 1.000000000000000000, 0.8660254037844387076, 1.000000000000000000, 0.8660254037844387076, 1.000000000000000000, 0.8660254037844387076, 1.000000000000000000, 0.8660254037844387076, 1.000000000000000000, 0.8660254037844387076, 1.000000000000000000, 0.8660254037844387076, 1.000000000000000000, 0.8660254037844387076, 1.000000000000000000, 0.8660254037844387076, 1.000000000000000000, 0.8660254037844387076, 1.000000000000000000, 0.8660254037844387076, 1.000000000000000000, 0.8660254037844387076, 1.000000000000000000, 0.8660254037844387076, 1.000000000000000000, 0.8660254037844387076, 1.000000000000000000, 0.8660254037844387076, 1.000000000000000000, 0.8660254037844387076, 1.000000000000000000, 0.8660254037844387076, 1.000000000000000000, 0.8660254037844387076, 1.000000000000000000, 0.8660254037844387076, 1.000000000000000000, 0.8660254037844387076, 1.000000000000000000, 0.8660254037844387076, 1.000000000000000000, 0.8660254037844387076, 1.000000000000000000, 0.8660254037844387076, 1.000000000000000000, 0.8660254037844387076, 1.000000000000000000, 0.8660254037844387076, 1.000000000000000000, 0.8660254037844387076, 1.000000000000000000, 0.8660254037844387076, 1.000000000000000000, 0.8660254037844387076, 1.000000000000000000, 0.8660254037844387076, 1.000000000000000000, 0.8660254037844387076, 1.000000000000000000, 0.8660254037844387076, 1.000000000000000000, 0.8660254037844387076, 1.000000000000000000, 0.8660254037844387076, 1.000000000000000000, 0.8660254037844387076, 1.000000000000000000, 0.8660254037844387076, 1.000000000000000000, 0.8660254037844387076, 1.000000000000000000, 0.8660254037844387076, 1.000000000000000000, 0.8660254037844387076, 1.000000000000000000, 0.8660254037844387076, 1.000000000000000000, 0.8660254037844387076, 1.000000000000000000, 0.8660254037844387076, 1.000000000000000000, 0.8660254037844387076, 1.000000000000000000, 0.8660254037844387076, 1.000000000000000000, 0.8660254037844387076, 1.000000000000000000, 0.8660254037844387076, 1.000000000000000000, 0.8660254037844387076, 1.000000000000000000, 0.8660254037844387076, 1.000000000000000000, 0.8660254037844387076, 1.000000000000000000, 0.8660254037844387076, 1.000000000000000000, 0.8660254037844387076, 1.000000000000000000, 0.8660254037844387076, 1.000000000000000000, 0.8660254037844387076, 1.000000000000000000, 0.8660254037844387076, 1.000000000000000000, 0.8660254037844387076, 1.000000000000000000, 0.8660254037844387076, 1.000000000000000000, 0.8660254037844387076, 1.000000000000000000, 0.8660254037844387076, 1.000000000000000000, 0.8660254037844387076, 1.000000000000000000, 0.8660254037844387076, 1.000000000000000000, 0.8660254037844387076, 1.000000000000000000, 0.8660254037844387076, 1.000000000000000000, 0.8660254037844387076, 1.000000000000000000, 0.8660254037844387076, 1.000000000000000000, 0.8660254037844387076, 1.000000000000000000, 0.8660254037844387076, 1.000000000000000000, 0.8660254037844387076, 1.000000000000000000, 0.8660254037844387076, 1.000000000000000000, 0.8660254037844387076, 1.000000000000000000, 0.8660254037844387076, 1.000000000000000000, 0.8660254037844387076, 1.000000000000000000, 0.8660254037844387076, 1.000000000000000000, 0.8660254037844387076, 1.000000000000000000, 0.8660254037844387076, 1.000000000000000000, 0.8660254037844387076, 1.000000000000000000, 0.8660254037844387076, 1.000000000000000000, 0.8660254037844387076, 1.000000000000000000, 0.8660254037844387076, 1.000000000000000000, 0.8660254037844387076, 1.000000000000000000, 0.8660254037844387076, 1.000000000000000000, 0.8660254037844387076, 1.000000000000000000, 0.8660254037844387076, 1.000000000000000000, 0.8660254037844387076, 1.000000000000000000, 0.8660254037844387076, 1.000000000000000000, 0.8660254037844387076, 1.000000000000000000, 0.8660254037844387076, 1.000000000000000000, 0.8660254037844387076, 1.000000000000000000, 0.8660254037844387076, 1.000000000000000000, 0.8660254037844387076, 1.000000000000000000, 0.8660254037844387076, 1.000000000000000000, 0.8660254037844387076, 1.000000000000000000, 0.8660254037844387076, 1.000000000000000000, 0.8660254037844387076, 1.000000000000000000, 0.8660254037844387076, 1.000000000000000000, 0.8660254037844387076, 1.000000000000000000, 0.8660254037844387076, 1.000000000000000000, 0.8660254037844387076, 1.000000000000000000, 0.8660254037844387076, 1.000000000000000000, 0.8660254037844387076, 1.000000000000000000, 0.8660254037844387076, 1.000000000000000000, 0.8660254037844387076, 1.000000000000000000, 0.8660254037844387076, 1.000000000000000000, 0.8660254037844387076, 1.000000000000000000, 0.8660254037844387076, 1.000000000000000000, 0.8660254037844387076, 1.000000000000000000, 0.8660254037844387076, 1.000000000000000000, 0.8660254037844387076, 1.000000000000000000, 0.8660254037844387076, 1.000000000000000000, 0.8660254037844387076, 1.000000000000000000, 0.8660254037844387076, 1.000000000000000000, 0.8660254037844387076, 1.000000000000000000, 0.8660254037844387076, 1.000000000000000000, 0.8660254037844387076, 1.000000000000000000, 0.8660254037844387076, 1.000000000000000000, 0.8660254037844387076, 1.000000000000000000, 0.8660254037844387076, 1.000000000000000000, 0.8660254037844387076, 1.000000000000000000, 0.8660254037844387076, 1.000000000000000000, 0.8660254037844387076, 1.000000000000000000, 0.8660254037844387076, 1.000000000000000000, 0.8660254037844387076, 1.000000000000000000, 0.8660254037844387076, 1.000000000000000000, 0.8660254037844387076, 1.000000000000000000, 0.8660254037844387076, 1.000000000000000000, 0.8660254037844387076, 1.000000000000000000, 0.8660254037844387076, 1.000000000000000000, 0.8660254037844387076, 1.000000000000000000, 0.8660254037844387076, 1.000000000000000000, 0.8660254037844387076, 1.000000000000000000, 0.8660254037844387076, 1.000000000000000000, 0.8660254037844387076, 1.000000000000000000, 0.8660254037844387076, 1.000000000000000000, 0.8660254037844387076, 1.000000000000000000, 0.8660254037844387076, 1.000000000000000000, 0.8660254037844387076, 1.000000000000000000, 0.8660254037844387076, 1.000000000000000000, 0.8660254037844387076, 1.000000000000000000, 0.8660254037844387076, 1.000000000000000000, 0.8660254037844387076, 1.000000000000000000, 0.8660254037844387076, 1.000000000000000000, 0.8660254037844387076, 1.000000000000000000, 0.8660254037844387076, 1.000000000000000000, 0.8660254037844387076, 1.000000000000000000, 0.8660254037844387076, 1.000000000000000000, 0.8660254037844387076, 1.000000000000000000, 0.8660254037844387076, 1.000000000000000000, 0.8660254037844387076, 1.000000000000000000, 0.8660254037844387076, 1.000000000000000000, 0.8660254037844387076, 1.000000000000000000, 0.8660254037844387076, 1.000000000000000000, 0.8660254037844387076, 1.000000000000000000, 0.8660254037844387076, 1.000000000000000000, 0.8660254037844387076, 1.000000000000000000, 0.8660254037844387076, 1.000000000000000000, 0.8660254037844387076, 1.000000000000000000, 0.8660254037844387076, 1.000000000000000000, 0.8660254037844387076, 1.000000000000000000, 0.8660254037844387076, 1.000000000000000000, 0.8660254037844387076, 1.000000000000000000, 0.8660254037844387076, 1.000000000000000000, 0.8660254037844387076, 1.000000000000000000, 0.8660254037844387076, 1.000000000000000000, 0.8660254037844387076, 1.000000000000000000, 0.8660254037844387076, 1.000000000000000000, 0.8660254037844387076, 1.000000000000000000, 0.8660254037844387076, 1.000000000000000000, 0.8660254037844387076, 1.000000000000000000, 0.8660254037844387076, 1.000000000000000000, 0.8660254037844387076, 1.000000000000000000, 0.8660254037844387076, 1.000000000000000000, 0.8660254037844387076, 1.000000000000000000, 0.8660254037844387076, 1.000000000000000000, 0.8660254037844387076, 1.000000000000000000, 0.8660254037844387076, 1.000000000000000000, 0.8660254037844387076, 1.000000000000000000, 0.8660254037844387076, 1.000000000000000000, 0.8660254037844387076, 1.000000000000000000, 0.8660254037844387076, 1.000000000000000000, 0.8660254037844387076, 1.000000000000000000, 0.8660254037844387076, 1.000000000000000000, 0.8660254037844387076, 1.000000000000000000, 0.8660254037844387076, 1.000000000000000000, 0.8660254037844387076, 1.000000000000000000, 0.8660254037844387076, 1.000000000000000000, 0.8660254037844387076, 1.000000000000000000, 0.8660254037844387076, 1.000000000000000000, 0.8660254037844387076, 1.000000000000000000, 0.8660254037844387076, 1.000000000000000000, 0.8660254037844387076, 1.000000000000000000, 0.8660254037844387076, 1.000000000000000000, 0.8660254037844387076, 1.000000000000000000, 0.8660254037844387076, 1.000000000000000000, 0.8660254037844387076, 1.000000000000000000, 0.8660254037844387076, 1.000000000000000000, 0.8660254037844387076, 1.000000000000000000, 0.8660254037844387076, 1.000000000000000000, 0.8660254037844387076, 1.000000000000000000, 0.8660254037844387076, 1.000000000000000000, 0.8660254037844387076, 1.000000000000000000, 0.8660254037844387076, 1.000000000000000000, 0.8660254037844387076, 1.000000000000000000, 0.8660254037844387076, 1.000000000000000000, 0.8660254037844387076, 1.000000000000000000, 0.8660254037844387076, 1.000000000000000000, 0.8660254037844387076, 1.000000000000000000, 0.8660254037844387076, 1.000000000000000000, 0.8660254037844387076, 1.000000000000000000, 0.8660254037844387076, 1.000000000000000000, 0.8660254037844387076, 1.000000000000000000, 0.8660254037844387076, 1.000000000000000000, 0.8660254037844387076, 1.000000000000000000, 0.8660254037844387076, 1.000000000000000000, 0.8660254037844387076, 1.000000000000000000, 0.8660254037844387076, 1.000000000000000000, 0.8660254037844387076, 1.000000000000000000, 0.8660254037844387076, 1.000000000000000000, 0.8660254037844387076, 1.000000000000000000, 0.8660254037844387076, 1.000000000000000000, 0.8660254037844387076, 1.000000000000000000, 0.8660254037844387076, 1.000000000000000000, 0.8660254037844387076, 1.000000000000000000, 0.8660254037844387076, 1.000000000000000000, 0.8660254037844387076, 1.000000000000000000, 0.8660254037844387076, 1.000000000000000000, 0.8660254037844387076, 1.000000000000000000, 0.8660254037844387076, 1.000000000000000000, 0.8660254037844387076, 1.000000000000000000, 0.8660254037844387076, 1.000000000000000000, 0.8660254037844387076, 1.000000000000000000, 0.8660254037844387076, 1.000000000000000000, 0.8660254037844387076, 1.000000000000000000, 0.8660254037844387076, 1.000000000000000000, 0.8660254037844387076, 1.000000000000000000, 0.8660254037844387076, 1.000000000000000000, 0.8660254037844387076, 1.000000000000000000, 0.8660254037844387076, 1.000000000000000000, 0.8660254037844387076, 1.000000000000000000, 0.8660254037844387076, 1.000000000000000000, 0.8660254037844387076, 1.000000000000000000, 0.8660254037844387076, 1.000000000000000000, 0.8660254037844387076, 1.000000000000000000, 0.8660254037844387076, 1.000000000000000000, 0.8660254037844387076, 1.000000000000000000, 0.8660254037844387076, 1.000000000000000000, 0.8660254037844387076, 1.000000000000000000, 0.8660254037844387076, 1.000000000000000000, 0.8660254037844387076, 1.000000000000000000, 0.8660254037844387076, 1.000000000000000000, 0.8660254037844387076, 1.000000000000000000, 0.8660254037844387076, 1.000000000000000000, 0.8660254037844387076, 1.000000000000000000, 0.8660254037844387076, 1.000000000000000000, 0.8660254037844387076, 1.000000000000000000, 0.8660254037844387076, 1.000000000000000000, 0.8660254037844387076, 1.000000000000000000, 0.8660254037844387076, 1.000000000000000000, 0.8660254037844387076, 1.000000000000000000, 0.8660254037844387076, 1.000000000000000000, 0.8660254037844387076, 1.000000000000000000, 0.8660254037844387076, 1.000000000000000000, 0.8660254037844387076, 1.000000000000000000, 0.8660254037844387076, 1.000000000000000000, 0.8660254037844387076, 1.000000000000000000, 0.8660254037844387076, 1.000000000000000000, 0.8660254037844387076, 1.000000000000000000, 0.8660254037844387076, 1.000000000000000000, 0.8660254037844387076, 1.000000000000000000, 0.8660254037844387076, 1.000000000000000000, 0.8660254037844387076, 1.000000000000000000, 0.8660254037844387076, 1.000000000000000000, 0.8660254037844387076, 1.000000000000000000, 0.8660254037844387076, 1.000000000000000000, 0.8660254037844387076, 1.000000000000000000, 0.8660254037844387076, 1.000000000000000000, 0.8660254037844387076, 1.000000000000000000, 0.8660254037844387076, 1.000000000000000000, 0.8660254037844387076, 1.000000000000000000, 0.8660254037844387076, 1.000000000000000000, 0.8660254037844387076, 1.000000000000000000, 0.8660254037844387076, 1.000000000000000000, 0.8660254037844387076, 1.000000000000000000, 0.8660254037844387076, 1.000000000000000000, 0.8660254037844387076, 1.000000000000000000, 0.8660254037844387076, 1.000000000000000000, 0.8660254037844387076, 1.000000000000000000, 0.8660254037844387076, 1.000000000000000000, 0.8660254037844387076, 1.000000000000000000, 0.8660254037844387076, 1.000000000000000000, 0.8660254037844387076, 1.000000000000000000, 0.8660254037844387076, 1.000000000000000000, 0.8660254037844387076, 1.000000000000000000, 0.8660254037844387076, 1.000000000000000000, 0.8660254037844387076, 1.000000000000000000, 0.8660254037844387076, 1.000000000000000000, 0.8660254037844387076, 1.000000000000000000, 0.8660254037844387076, 1.000000000000000000, 0.8660254037844387076, 1.000000000000000000, 0.8660254037844387076, 1.000000000000000000, 0.8660254037844387076, 1.000000000000000000, 0.8660254037844387076, 1.000000000000000000, 0.8660254037844387076, 1.000000000000000000, 0.8660254037844387076, 1.000000000000000000, 0.8660254037844387076, 1.000000000000000000, 0.8660254037844387076, 1.000000000000000000, 0.8660254037844387076, 1.000000000000000000, 0.8660254037844387076, 1.000000000000000000, 0.8660254037844387076, 1.000000000000000000, 0.8660254037844387076, 1.000000000000000000, 0.8660254037844387076, 1.000000000000000000, 0.8660254037844387076, 1.000000000000000000, 0.8660254037844387076, 1.000000000000000000, 0.8660254037844387076, 1.000000000000000000, 0.8660254037844387076, 1.000000000000000000, 0.8660254037844387076, 1.000000000000000000, 0.8660254037844387076, 1.000000000000000000, 0.8660254037844387076, 1.000000000000000000, 0.8660254037844387076, 1.000000000000000000, 0.8660254037844387076, 1.000000000000000000, 0.8660254037844387076, 1.000000000000000000, 0.8660254037844387076, 1.000000000000000000, 0.8660254037844387076, 1.000000000000000000, 0.8660254037844387076, 1.000000000000000000, 0.8660254037844387076, 1.000000000000000000, 0.8660254037844387076, 1.000000000000000000, 0.8660254037844387076, 1.000000000000000000, 0.8660254037844387076, 1.000000000000000000, 0.8660254037844387076, 1.000000000000000000, 0.8660254037844387076, 1.000000000000000000, 0.8660254037844387076, 1.000000000000000000, 0.8660254037844387076, 1.000000000000000000, 0.8660254037844387076, 1.000000000000000000, 0.8660254037844387076, 1.000000000000000000, 0.8660254037844387076, 1.000000000000000000, 0.8660254037844387076, 1.000000000000000000, 0.8660254037844387076, 1.000000000000000000, 0.8660254037844387076, 1.000000000000000000, 0.8660254037844387076, 1.000000000000000000, 0.8660254037844387076, 1.000000000000000000, 0.8660254037844387076, 1.000000000000000000, 0.8660254037844387076, 1.000000000000000000, 0.8660254037844387076, 1.000000000000000000, 0.8660254037844387076, 1.000000000000000000, 0.8660254037844387076, 1.000000000000000000, 0.8660254037844387076, 1.000000000000000000, 0.8660254037844387076, 1.000000000000000000, 0.8660254037844387076, 1.000000000000000000, 0.8660254037844387076, 1.000000000000000000, 0.8660254037844387076, 1.000000000000000000, 0.8660254037844387076, 1.000000000000000000, 0.8660254037844387076, 1.000000000000000000, 0.8660254037844387076, 1.000000000000000000, 0.8660254037844387076, 1.000000000000000000, 0.8660254037844387076, 1.000000000000000000, 0.8660254037844387076, 1.000000000000000000, 0.8660254037844387076, 1.000000000000000000, 0.8660254037844387076, 1.000000000000000000, 0.8660254037844387076, 1.000000000000000000, 0.8660254037844387076, 1.000000000000000000, 0.8660254037844387076, 1.000000000000000000, 0.8660254037844387076, 1.000000000000000000, 0.8660254037844387076, 1.000000000000000000, 0.8660254037844387076, 1.000000000000000000, 0.8660254037844387076, 1.000000000000000000, 0.8660254037844387076, 1.000000000000000000, 0.8660254037844387076, 1.000000000000000000, 0.8660254037844387076, 1.000000000000000000, 0.8660254037844387076, 1.000000000000000000, 0.8660254037844387076, 1.000000000000000000, 0.8660254037844387076, 1.000000000000000000, 0.8660254037844387076, 1.000000000000000000, 0.8660254037844387076, 1.000000000000000000, 0.8660254037844387076, 1.000000000000000000, 0.8660254037844387076, 1.000000000000000000, 0.8660254037844387076, 1.000000000000000000, 0.8660254037844387076, 1.000000000000000000, 0.8660254037844387076, 1.000000000000000000, 0.8660254037844387076, 1.000000000000000000, 0.8660254037844387076, 1.000000000000000000, 0.8660254037844387076, 1.000000000000000000, 0.8660254037844387076, 1.000000000000000000, 0.8660254037844387076, 1.000000000000000000, 0.8660254037844387076, 1.000000000000000000, 0.8660254037844387076, 1.000000000000000000, 0.8660254037844387076, 1.000000000000000000, 0.8660254037844387076, 1.000000000000000000, 0.8660254037844387076, 1.000000000000000000, 0.8660254037844387076, 1.000000000000000000, 0.8660254037844387076, 1.000000000000000000, 0.8660254037844387076, 1.000000000000000000, 0.8660254037844387076, 1.000000000000000000, 0.8660254037844387076, 1.000000000000000000, 0.8660254037844387076, 1.000000000000000000, 0.8660254037844387076, 1.000000000000000000, 0.8660254037844387076, 1.000000000000000000, 0.8660254037844387076, 1.000000000000000000, 0.8660254037844387076, 1.000000000000000000, 0.8660254037844387076, 1.000000000000000000, 0.8660254037844387076, 1.000000000000000000, 0.8660254037844387076, 1.000000000000000000, 0.8660254037844387076, 1.000000000000000000, 0.8660254037844387076, 1.000000000000000000, 0.8660254037844387076, 1.000000000000000000, 0.8660254037844387076, 1.000000000000000000, 0.8660254037844387076, 1.000000000000000000, 0.8660254037844387076, 1.000000000000000000, 0.8660254037844387076, 1.000000000000000000, 0.8660254037844387076, 1.000000000000000000, 0.8660254037844387076, 1.000000000000000000, 0.8660254037844387076, 1.000000000000000000, 0.8660254037844387076, 1.000000000000000000, 0.8660254037844387076, 1.000000000000000000, 0.8660254037844387076, 1.000000000000000000, 0.8660254037844387076, 1.000000000000000000, 0.8660254037844387076, 1.000000000000000000, 0.8660254037844387076, 1.000000000000000000, 0.8660254037844387076, 1.000000000000000000, 0.8660254037844387076, 1.000000000000000000, 0.8660254037844387076, 1.000000000000000000, 0.8660254037844387076, 1.000000000000000000, 0.8660254037844387076, 1.000000000000000000, 0.8660254037844387076, 1.000000000000000000, 0.8660254037844387076, 1.000000000000000000, 0.8660254037844387076, 1.000000000000000000, 0.8660254037844387076, 1.000000000000000000, 0.8660254037844387076, 1.000000000000000000, 0.8660254037844387076, 1.000000000000000000, 0.8660254037844387076, 1.000000000000000000, 0.8660254037844387076, 1.000000000000000000, 0.8660254037844387076, 1.000000000000000000, 0.8660254037844387076, 1.000000000000000000, 0.8660254037844387076, 1.000000000000000000, 0.8660254037844387076, 1.000000000000000000, 0.8660254037844387076, 1.000000000000000000, 0.8660254037844387076, 1.000000000000000000, 0.8660254037844387076, 1.000000000000000000, 0.8660254037844387076, 1.000000000000000000, 0.8660254037844387076, 1.000000000000000000, 0.8660254037844387076, 1.000000000000000000, 0.8660254037844387076, 1.000000000000000000, 0.8660254037844387076, 1.000000000000000000, 0.8660254037844387076, 1.000000000000000000, 0.8660254037844387076, 1.000000000000000000, 0.8660254037844387076, 1.000000000000000000, 0.8660254037844387076, 1.000000000000000000, 0.8660254037844387076, 1.000000000000000000, 0.8660254037844387076, 1.000000000000000000, 0.8660254037844387076, 1.000000000000000000, 0.8660254037844387076, 1.000000000000000000, 0.8660254037844387076, 1.000000000000000000, 0.8660254037844387076, 1.000000000000000000, 0.8660254037844387076, 1.000000000000000000, 0.8660254037844387076, 1.000000000000000000, 0.8660254037844387076, 1.000000000000000000, 0.8660254037844387076, 1.000000000000000000, 0.8660254037844387076, 1.000000000000000000, 0.8660254037844387076, 1.000000000000000000, 0.8660254037844387076, 1.000000000000000000, 0.8660254037844387076, 1.000000000000000000, 0.8660254037844387076, 1.000000000000000000, 0.8660254037844387076, 1.000000000000000000, 0.8660254037844387076, 1.000000000000000000, 0.8660254037844387076, 1.000000000000000000, 0.8660254037844387076, 1.000000000000000000, 0.8660254037844387076, 1.000000000000000000, 0.8660254037844387076, 1.000000000000000000, 0.8660254037844387076, 1.000000000000000000, 0.8660254037844387076, 1.000000000000000000, 0.8660254037844387076, 1.000000000000000000, 0.8660254037844387076, 1.000000000000000000, 0.8660254037844387076, 1.000000000000000000, 0.8660254037844387076, 1.000000000000000000, 0.8660254037844387076, 1.000000000000000000, 0.8660254037844387076, 1.000000000000000000, 0.8660254037844387076, 1.000000000000000000, 0.8660254037844387076, 1.000000000000000000, 0.8660254037844387076, 1.000000000000000000, 0.8660254037844387076, 1.000000000000000000, 0.8660254037844387076, 1.000000000000000000, 0.8660254037844387076, 1.000000000000000000, 0.8660254037844387076, 1.000000000000000000, 0.8660254037844387076, 1.000000000000000000, 0.8660254037844387076, 1.000000000000000000, 0.8660254037844387076, 1.000000000000000000, 0.8660254037844387076, 1.000000000000000000, 0.8660254037844387076, 1.000000000000000000, 0.8660254037844387076, 1.000000000000000000, 0.8660254037844387076, 1.000000000000000000, 0.8660254037844387076, 1.000000000000000000, 0.8660254037844387076, 1.000000000000000000, 0.8660254037844387076, 1.000000000000000000, 0.8660254037844387076, 1.000000000000000000, 0.8660254037844387076, 1.000000000000000000, 0.8660254037844387076, 1.000000000000000000, 0.8660254037844387076, 1.000000000000000000, 0.8660254037844387076, 1.000000000000000000, 0.8660254037844387076, 1.000000000000000000, 0.8660254037844387076, 1.000000000000000000, 0.8660254037844387076, 1.000000000000000000, 0.8660254037844387076, 1.000000000000000000, 0.8660254037844387076, 1.000000000000000000, 0.8660254037844387076, 1.000000000000000000, 0.8660254037844387076, 1.000000000000000000, 0.8660254037844387076, 1.000000000000000000, 0.8660254037844387076, 1.000000000000000000, 0.8660254037844387076, 1.000000000000000000, 0.8660254037844387076, 1.000000000000000000, 0.8660254037844387076, 1.000000000000000000, 0.8660254037844387076, 1.000000000000000000, 0.8660254037844387076, 1.000000000000000000, 0.8660254037844387076, 1.000000000000000000, 0.8660254037844387076, 1.000000000000000000, 0.8660254037844387076, 1.000000000000000000, 0.8660254037844387076, 1.000000000000000000, 0.8660254037844387076, 1.000000000000000000, 0.8660254037844387076, 1.000000000000000000, 0.8660254037844387076, 1.000000000000000000, 0.8660254037844387076, 1.000000000000000000, 0.8660254037844387076, 1.000000000000000000, 0.8660254037844387076, 1.000000000000000000, 0.8660254037844387076, 1.000000000000000000, 0.8660254037844387076, 1.000000000000000000, 0.8660254037844387076, 1.000000000000000000, 0.8660254037844387076, 1.000000000000000000, 0.8660254037844387076, 1.000000000000000000, 0.8660254037844387076, 1.000000000000000000, 0.8660254037844387076, 1.000000000000000000, 0.8660254037844387076, 1.000000000000000000, 0.8660254037844387076, 1.000000000000000000, 0.8660254037844387076, 1.000000000000000000, 0.8660254037844387076, 1.000000000000000000, 0.8660254037844387076, 1.000000000000000000, 0.8660254037844387076, 1.000000000000000000, 0.8660254037844387076, 1.000000000000000000, 0.8660254037844387076, 1.000000000000000000, 0.8660254037844387076, 1.000000000000000000, 0.8660254037844387076, 1.000000000000000000, 0.8660254037844387076, 1.000000000000000000, 0.8660254037844387076, 1.000000000000000000, 0.8660254037844387076, 1.000000000000000000, 0.8660254037844387076, 1.000000000000000000, 0.8660254037844387076, 1.000000000000000000, 0.8660254037844387076, 1.000000000000000000, 0.8660254037844387076, 1.000000000000000000, 0.8660254037844387076, 1.000000000000000000, 0.8660254037844387076, 1.000000000000000000, 0.8660254037844387076, 1.000000000000000000, 0.8660254037844387076, 1.000000000000000000, 0.8660254037844387076, 1.000000000000000000, 0.8660254037844387076, 1.000000000000000000, 0.8660254037844387076, 1.000000000000000000, 0.8660254037844387076, 1.000000000000000000, 0.8660254037844387076, 1.000000000000000000, 0.8660254037844387076, 1.000000000000000000, 0.8660254037844387076, 1.000000000000000000, 0.8660254037844387076, 1.000000000000000000, 0.8660254037844387076, 1.000000000000000000, 0.8660254037844387076, 1.000000000000000000, 0.8660254037844387076, 1.000000000000000000, 0.8660254037844387076, 1.000000000000000000, 0.8660254037844387076, 1.000000000000000000, 0.8660254037844387076, 1.000000000000000000, 0.8660254037844387076, 1.000000000000000000, 0.8660254037844387076, 1.000000000000000000, 0.8660254037844387076, 1.000000000000000000, 0.8660254037844387076, 1.000000000000000000, 0.8660254037844387076, 1.000000000000000000, 0.8660254037844387076, 1.000000000000000000, 0.8660254037844387076, 1.000000000000000000, 0.8660254037844387076, 1.000000000000000000, 0.8660254037844387076, 1.000000000000000000, 0.8660254037844387076, 1.000000000000000000, 0.8660254037844387076, 1.000000000000000000, 0.8660254037844387076, 1.000000000000000000, 0.8660254037844387076, 1.000000000000000000, 0.8660254037844387076, 1.000000000000000000, 0.8660254037844387076, 1.000000000000000000, 0.8660254037844387076, 1.000000000000000000, 0.8660254037844387076, 1.000000000000000000, 0.8660254037844387076, 1.000000000000000000, 0.8660254037844387076, 1.000000000000000000, 0.8660254037844387076, 1.000000000000000000, 0.8660254037844387076, 1.000000000000000000, 0.8660254037844387076, 1.000000000000000000, 0.8660254037844387076, 1.000000000000000000, 0.8660254037844387076, 1.000000000000000000, 0.8660254037844387076, 1.000000000000000000, 0.8660254037844387076, 1.000000000000000000, 0.8660254037844387076, 1.000000000000000000, 0.8660254037844387076, 1.000000000000000000, 0.8660254037844387076, 1.000000000000000000, 0.8660254037844387076, 1.000000000000000000, 0.8660254037844387076, 1.000000000000000000, 0.8660254037844387076, 1.000000000000000000, 0.8660254037844387076, 1.000000000000000000, 0.8660254037844387076, 1.000000000000000000, 0.8660254037844387076, 1.000000000000000000, 0.8660254037844387076, 1.000000000000000000, 0.8660254037844387076, 1.000000000000000000, 0.8660254037844387076, 1.000000000000000000, 0.8660254037844387076, 1.000000000000000000, 0.8660254037844387076, 1.000000000000000000, 0.8660254037844387076, 1.000000000000000000, 0.8660254037844387076, 1.000000000000000000, 0.8660254037844387076, 1.000000000000000000, 0.8660254037844387076, 1.000000000000000000, 0.8660254037844387076, 1.000000000000000000, 0.8660254037844387076, 1.000000000000000000, 0.8660254037844387076, 1.000000000000000000, 0.8660254037844387076, 1.000000000000000000, 0.8660254037844387076, 1.000000000000000000, 0.8660254037844387076, 1.000000000000000000, 0.8660254037844387076, 1.000000000000000000, 0.8660254037844387076, 1.000000000000000000, 0.8660254037844387076, 1.000000000000000000, 0.8660254037844387076, 1.000000000000000000, 0.8660254037844387076, 1.000000000000000000, 0.8660254037844387076, 1.000000000000000000, 0.8660254037844387076, 1.000000000000000000, 0.8660254037844387076, 1.000000000000000000, 0.8660254037844387076, 1.000000000000000000, 0.8660254037844387076, 1.000000000000000000, 0.8660254037844387076, 1.000000000000000000, 0.8660254037844387076, 1.000000000000000000, 0.8660254037844387076, 1.000000000000000000, 0.8660254037844387076, 1.000000000000000000, 0.8660254037844387076, 1.000000000000000000, 0.8660254037844387076, 1.000000000000000000, 0.8660254037844387076, 1.000000000000000000, 0.8660254037844387076, 1.000000000000000000, 0.8660254037844387076, 1.000000000000000000, 0.8660254037844387076, 1.000000000000000000, 0.8660254037844387076, 1.000000000000000000, 0.8660254037844387076, 1.000000000000000000, 0.8660254037844387076, 1.000000000000000000, 0.8660254037844387076, 1.000000000000000000, 0.8660254037844387076, 1.000000000000000000, 0.8660254037844387076, 1.000000000000000000, 0.8660254037844387076, 1.000000000000000000, 0.8660254037844387076, 1.000000000000000000, 0.8660254037844387076, 1.000000000000000000, 0.8660254037844387076, 1.000000000000000000, 0.8660254037844387076, 1.000000000000000000, 0.8660254037844387076, 1.000000000000000000, 0.8660254037844387076, 1.000000000000000000, 0.8660254037844387076, 1.000000000000000000, 0.8660254037844387076, 1.000000000000000000, 0.8660254037844387076, 1.000000000000000000, 0.8660254037844387076, 1.000000000000000000, 0.8660254037844387076, 1.000000000000000000, 0.8660254037844387076, 1.000000000000000000, 0.8660254037844387076, 1.000000000000000000, 0.8660254037844387076, 1.000000000000000000, 0.8660254037844387076, 1.000000000000000000, 0.8660254037844387076, 1.000000000000000000, 0.8660254037844387076, 1.000000000000000000, 0.8660254037844387076, 1.000000000000000000, 0.8660254037844387076, 1.000000000000000000, 0.8660254037844387076, 1.000000000000000000, 0.8660254037844387076, 1.000000000000000000, 0.8660254037844387076, 1.000000000000000000, 0.8660254037844387076, 1.000000000000000000, 0.8660254037844387076, 1.000000000000000000, 0.8660254037844387076, 1.000000000000000000, 0.8660254037844387076, 1.000000000000000000, 0.8660254037844387076, 1.000000000000000000, 0.8660254037844387076, 1.000000000000000000, 0.8660254037844387076, 1.000000000000000000, 0.8660254037844387076, 1.000000000000000000, 0.8660254037844387076, 1.000000000000000000, 0.8660254037844387076, 1.000000000000000000, 0.8660254037844387076, 1.000000000000000000, 0.8660254037844387076, 1.000000000000000000, 0.8660254037844387076, 1.000000000000000000, 0.8660254037844387076, 1.000000000000000000, 0.8660254037844387076, 1.000000000000000000) ) ) 
 REPRESENTATION_ITEM ( '' )  SURFACE ( )  );
#14521=EDGE_LOOP ( 'NONE', ( #15469, #44445, #4035, #45108 ) ) ;
#14524=ADVANCED_FACE ( 'NONE', ( #48397 ), #29718, .T. ) ;
#14525=CARTESIAN_POINT ( 'NONE',  ( 5.000000000000000000, -19.49999999999999645, -6.123233995736766282E-16 ) ) ;
#14528=CARTESIAN_POINT ( 'NONE',  ( -4.458734124999999437, -24.56249999863440436, 0.000000000000000000 ) ) ;
#14537=VERTEX_POINT ( 'NONE', #60619 ) ;
#14538=CARTESIAN_POINT ( 'NONE',  ( 1.975475456537005874E-15, -79.62499999726881583, 5.000000000000000000 ) ) ;
#14539=ORIENTED_EDGE ( 'NONE', *, *, #33062, .F. ) ;
#14540=CARTESIAN_POINT ( 'NONE',  ( 9.457646018065525792E-16, -75.31249999863440792, 5.148502694627439702 ) ) ;
#14542=EDGE_LOOP ( 'NONE', ( #19737, #22051, #20406, #41451 ) ) ;
#14547=CARTESIAN_POINT ( 'NONE',  ( -4.458734124999999437, 2.354166668032262599, -2.574251347313719407 ) ) ;
#14555=ORIENTED_EDGE ( 'NONE', *, *, #39634, .T. ) ;
#14556=CARTESIAN_POINT ( 'NONE',  ( -4.458734124999999437, -76.31249999863440792, 0.000000000000000000 ) ) ;
#14557=CARTESIAN_POINT ( 'NONE',  ( 2.499999999999998668, -0.2083333306021478704, -4.330127018922193649 ) ) ;
#14558=CARTESIAN_POINT ( 'NONE',  ( 4.458734124999998549, 4.270833334698926897, -2.574251347313721627 ) ) ;
#14559=CARTESIAN_POINT ( 'NONE',  ( -6.972266317189433020E-16, 19.75000000000000000, -5.000000000000000000 ) ) ;
#14560=CARTESIAN_POINT ( 'NONE',  ( 4.458734124999998549, -65.97916666530106511, -2.574251347313721627 ) ) ;
#14561=CARTESIAN_POINT ( 'NONE',  ( -5.000000000000000000, -22.87499999726881228, 0.000000000000000000 ) ) ;
#14562=CARTESIAN_POINT ( 'NONE',  ( -6.972266317189433020E-16, -11.12499999726881406, -5.000000000000000000 ) ) ;
#14563=CARTESIAN_POINT ( 'NONE',  ( 2.499999999999998668, -28.20833333060214798, -4.330127018922193649 ) ) ;
#14565=CARTESIAN_POINT ( 'NONE',  ( 1.975475456537005874E-15, -43.62499999726880873, 5.000000000000000000 ) ) ;
#14566=CARTESIAN_POINT ( 'NONE',  ( 2.229367062500001939, -46.97916666530106511, 3.861377020970579999 ) ) ;
#14567=CARTESIAN_POINT ( 'NONE',  ( 2.229367062500001939, -28.22916666530107221, 3.861377020970579999 ) ) ;
#14569=DIRECTION ( 'NONE',  ( -0.000000000000000000, 1.000000000000000000, -0.000000000000000000 ) ) ;
#14570=CARTESIAN_POINT ( 'NONE',  ( 5.000000000000000888, 27.41666666666666785, 2.886751345948126879 ) ) ;
#14572=CARTESIAN_POINT ( 'NONE',  ( -2.229367062500000163, -39.47916666530107221, -3.861377020970580443 ) ) ;
#14573=CARTESIAN_POINT ( 'NONE',  ( 1.060575238724906964E-15, -73.62499999726881583, 5.773502691896257311 ) ) ;
#14576=EDGE_CURVE ( 'NONE', #9561, #62900, #61274, .T. ) ;
#14578=CARTESIAN_POINT ( 'NONE',  ( 4.458734124999999437, -73.06249999863439371, -5.460374474430324690E-16 ) ) ;
#14582=CARTESIAN_POINT ( 'NONE',  ( -2.499999999999996447, -27.70833333060214798, 4.330127018922195425 ) ) ;
#14583=DIRECTION ( 'NONE',  ( -0.000000000000000000, 1.000000000000000000, -0.000000000000000000 ) ) ;
#14584=CARTESIAN_POINT ( 'NONE',  ( 5.000000000000000888, -20.58333333333333570, 2.886751345948126879 ) ) ;
#14586=VERTEX_POINT ( 'NONE', #40337 ) ;
#14589=CARTESIAN_POINT ( 'NONE',  ( 5.000000000000000000, 27.62500000273118417, -6.123233995736766282E-16 ) ) ;
#14593=EDGE_CURVE ( 'NONE', #6014, #29366, #58806, .T. ) ;
#14604=CARTESIAN_POINT ( 'NONE',  ( -4.458734124999998549, -23.22916666530107221, 2.574251347313722516 ) ) ;
#14605=DIRECTION ( 'NONE',  ( -0.000000000000000000, 1.000000000000000000, -0.000000000000000000 ) ) ;
#14609=( BOUNDED_CURVE ( )  B_SPLINE_CURVE ( 2, ( #55767, #36457, #56084, #12004, #31632, #51268, #7201, #7830, #47064 ),
 .UNSPECIFIED., .F., .F. ) 
 B_SPLINE_CURVE_WITH_KNOTS ( ( 3, 2, 2, 2, 3 ),
 ( 0.07678571428571429047, 0.07738095238095238360, 0.07857142857142856984, 0.07976190476190475609, 0.08035714285714286309 ),
 .UNSPECIFIED. ) 
 CURVE ( )  GEOMETRIC_REPRESENTATION_ITEM ( )  RATIONAL_B_SPLINE_CURVE ( ( 0.9330127018922194093, 0.9330127018922194093, 1.000000000000000000, 0.8660254037844387076, 1.000000000000000000, 0.8660254037844387076, 1.000000000000000000, 0.9330127018922185211, 0.9330127018922192983 ) ) 
 REPRESENTATION_ITEM ( '' )  );
#14613=EDGE_LOOP ( 'NONE', ( #16777, #40892, #48704, #42292 ) ) ;
#14615=FACE_OUTER_BOUND ( 'NONE', #15784, .T. ) ;
#14619=CARTESIAN_POINT ( 'NONE',  ( -6.972266317189433020E-16, -7.249999999999998224, -5.000000000000000000 ) ) ;
#14623=ORIENTED_EDGE ( 'NONE', *, *, #8402, .T. ) ;
#14624=DIRECTION ( 'NONE',  ( -0.000000000000000000, 1.000000000000000000, -0.000000000000000000 ) ) ;
#14625=CARTESIAN_POINT ( 'NONE',  ( -2.229367062500000163, 19.52083333469893134, -3.861377020970580443 ) ) ;
#14627=ORIENTED_EDGE ( 'NONE', *, *, #11828, .T. ) ;
#14632=CARTESIAN_POINT ( 'NONE',  ( 4.458734125000000326, -59.89583333196774362, 2.574251347313718519 ) ) ;
#14634=CARTESIAN_POINT ( 'NONE',  ( -4.458734124999998549, 15.77083333469892601, 2.574251347313722516 ) ) ;
#14636=CARTESIAN_POINT ( 'NONE',  ( 9.457646018065525792E-16, -51.31249999863440792, 5.148502694627439702 ) ) ;
#14637=CARTESIAN_POINT ( 'NONE',  ( -4.999999999999999112, -9.791666663935476578, 2.886751345948131764 ) ) ;
#14641=CARTESIAN_POINT ( 'NONE',  ( 4.458734124999998549, -107.7291666653010509, -2.574251347313721627 ) ) ;
#14642=CARTESIAN_POINT ( 'NONE',  ( -3.152548672688508926E-16, -9.812499998634406140, -5.148502694627439702 ) ) ;
#14645=CARTESIAN_POINT ( 'NONE',  ( -4.458734124999999437, -98.39583333196773651, -2.574251347313719407 ) ) ;
#14647=CARTESIAN_POINT ( 'NONE',  ( -4.458734124999999437, -99.64583333196773651, -2.574251347313719407 ) ) ;
#14649=CARTESIAN_POINT ( 'NONE',  ( 1.060575238724906964E-15, -55.62499999726880873, 5.773502691896257311 ) ) ;
#14650=CARTESIAN_POINT ( 'NONE',  ( -6.972266317189433020E-16, -5.249999999999998224, -5.000000000000000000 ) ) ;
#14653=CARTESIAN_POINT ( 'NONE',  ( -2.229367062500000163, -18.47916666530106866, -3.861377020970580443 ) ) ;
#14654=CARTESIAN_POINT ( 'NONE',  ( 9.457646018065525792E-16, 4.687500001365596525, 5.148502694627439702 ) ) ;
#14655=CARTESIAN_POINT ( 'NONE',  ( 4.458734124999999437, -61.06249999863440081, -5.460374474430324690E-16 ) ) ;
#14658=CARTESIAN_POINT ( 'NONE',  ( 0.000000000000000000, -120.0000000000000000, 5.000000000000000000 ) ) ;
#14660=CARTESIAN_POINT ( 'NONE',  ( -2.499999999999996447, -4.833333333333335702, 4.330127018922195425 ) ) ;
#14664=DIRECTION ( 'NONE',  ( -0.000000000000000000, 1.000000000000000000, -0.000000000000000000 ) ) ;
#14666=CARTESIAN_POINT ( 'NONE',  ( 1.975475456537005874E-15, -81.74999999999998579, 5.000000000000000000 ) ) ;
#14667=CARTESIAN_POINT ( 'NONE',  ( -4.458734124999998549, -85.22916666530107932, 2.574251347313722516 ) ) ;
#14668=CARTESIAN_POINT ( 'NONE',  ( 2.229367062500001939, 16.77083333469892779, 3.861377020970579999 ) ) ;
#14670=CARTESIAN_POINT ( 'NONE',  ( 5.000000000000000000, -0.5000000000000004441, -6.123233995736766282E-16 ) ) ;
#14674=CARTESIAN_POINT ( 'NONE',  ( -5.000000000000000000, -74.08333333333332860, -2.886751345948128211 ) ) ;
#14677=ORIENTED_EDGE ( 'NONE', *, *, #16143, .F. ) ;
#14679=ORIENTED_EDGE ( 'NONE', *, *, #13935, .F. ) ;
#14691=VERTEX_POINT ( 'NONE', #46759 ) ;
#14693=CARTESIAN_POINT ( 'NONE',  ( -3.152548672688508926E-16, -58.81249999863440081, -5.148502694627439702 ) ) ;
#14697=ORIENTED_EDGE ( 'NONE', *, *, #6177, .F. ) ;
#14702=CARTESIAN_POINT ( 'NONE',  ( -3.152548672688508926E-16, -107.8124999986343937, -5.148502694627439702 ) ) ;
#14707=CARTESIAN_POINT ( 'NONE',  ( 4.458734124999999437, -40.81249999863440081, -5.460374474430324690E-16 ) ) ;
#14711=CARTESIAN_POINT ( 'NONE',  ( 4.458734124999998549, -10.72916666530106866, -2.574251347313721627 ) ) ;
#14712=CARTESIAN_POINT ( 'NONE',  ( -4.458734124999999437, -100.5624999986344079, 0.000000000000000000 ) ) ;
#14715=CARTESIAN_POINT ( 'NONE',  ( -4.458734124999999437, -33.56249999863440792, 0.000000000000000000 ) ) ;
#14716=CARTESIAN_POINT ( 'NONE',  ( -3.535250795749689387E-16, 7.875000002731186832, -5.773502691896257311 ) ) ;
#14717=DIRECTION ( 'NONE',  ( -0.000000000000000000, 1.000000000000000000, -0.000000000000000000 ) ) ;
#14720=CARTESIAN_POINT ( 'NONE',  ( 6.123233995736766282E-16, -120.0000000000000000, -5.000000000000000000 ) ) ;
#14722=CARTESIAN_POINT ( 'NONE',  ( 0.000000000000000000, -120.0000000000000000, 0.000000000000000000 ) ) ;
#14723=CARTESIAN_POINT ( 'NONE',  ( -2.229367062500000163, 5.270833334698927786, -3.861377020970580443 ) ) ;
#14724=VERTEX_POINT ( 'NONE', #22961 ) ;
#14726=CARTESIAN_POINT ( 'NONE',  ( 2.499999999999998668, 9.666666666666667851, -4.330127018922193649 ) ) ;
#14727=CARTESIAN_POINT ( 'NONE',  ( 5.000000000000000888, -95.58333333333332860, 2.886751345948126879 ) ) ;
#14728=CARTESIAN_POINT ( 'NONE',  ( 9.457646018065525792E-16, -31.06249999863440436, 5.148502694627439702 ) ) ;
#14729=CARTESIAN_POINT ( 'NONE',  ( -2.500000000000000444, -23.04166666393548013, -4.330127018922193649 ) ) ;
#14730=CARTESIAN_POINT ( 'NONE',  ( 9.457646018065525792E-16, -79.31249999863439371, 5.148502694627439702 ) ) ;
#14735=CARTESIAN_POINT ( 'NONE',  ( 9.457646018065525792E-16, -2.062499998634406584, 5.148502694627439702 ) ) ;
#14736=FACE_OUTER_BOUND ( 'NONE', #55932, .T. ) ;
#14737=CARTESIAN_POINT ( 'NONE',  ( 2.229367062500001939, -43.22916666530107932, 3.861377020970579999 ) ) ;
#14742=CARTESIAN_POINT ( 'NONE',  ( -3.152548672688508926E-16, -69.56249999863439371, -5.148502694627439702 ) ) ;
#14743=CARTESIAN_POINT ( 'NONE',  ( -4.999999999999999112, -102.7916666639354588, 2.886751345948131764 ) ) ;
#14745=CARTESIAN_POINT ( 'NONE',  ( -4.999999999999998224, -64.91666666666665719, 2.886751345948131764 ) ) ;
#14746=LINE ( 'NONE', #53993, #34744 ) ;
#14748=CARTESIAN_POINT ( 'NONE',  ( 5.000000000000000000, -61.50000000000000000, -6.123233995736766282E-16 ) ) ;
#14752=CARTESIAN_POINT ( 'NONE',  ( 6.123233995736766282E-16, -120.0000000000000000, -5.000000000000000000 ) ) ;
#14760=VERTEX_POINT ( 'NONE', #12663 ) ;
#14761=LINE ( 'NONE', #9937, #40768 ) ;
#14768=CARTESIAN_POINT ( 'NONE',  ( -4.458734124999999437, -40.64583333196773651, -2.574251347313719407 ) ) ;
#14769=CARTESIAN_POINT ( 'NONE',  ( 4.769696007084728073, -114.9999999999999858, -1.500000000000000444 ) ) ;
#14771=CARTESIAN_POINT ( 'NONE',  ( 1.975475456537005874E-15, -56.62499999726880162, 5.000000000000000000 ) ) ;
#14778=CARTESIAN_POINT ( 'NONE',  ( -4.458734124999998549, -88.47916666530107932, 2.574251347313722516 ) ) ;
#14781=CARTESIAN_POINT ( 'NONE',  ( -1.339745962155610925, -31.79465819873851373, 5.000000000000000000 ) ) ;
#14788=CARTESIAN_POINT ( 'NONE',  ( -2.229367062500000163, 0.5208333346989266754, -3.861377020970580443 ) ) ;
#14791=CARTESIAN_POINT ( 'NONE',  ( -2.229367062499996610, -17.39583333196773651, 3.861377020970582219 ) ) ;
#14794=CARTESIAN_POINT ( 'NONE',  ( -2.500000000000000444, 3.958333336064518093, -4.330127018922193649 ) ) ;
#14796=CARTESIAN_POINT ( 'NONE',  ( 4.458734124999999437, 22.93750000136559564, -5.460374474430324690E-16 ) ) ;
#14798=CARTESIAN_POINT ( 'NONE',  ( -4.458734124999999437, -99.31249999863440792, 0.000000000000000000 ) ) ;
#14800=CARTESIAN_POINT ( 'NONE',  ( 2.229367062499998831, -12.64583333196774007, -3.861377020970580887 ) ) ;
#14804=CARTESIAN_POINT ( 'NONE',  ( 2.500000000000002220, -42.54166666393548013, 4.330127018922192761 ) ) ;
#14806=CARTESIAN_POINT ( 'NONE',  ( 4.458734124999998549, 12.27083333469892423, -2.574251347313721627 ) ) ;
#14810=CARTESIAN_POINT ( 'NONE',  ( 4.458734124999998549, -63.72916666530107221, -2.574251347313721627 ) ) ;
#14813=CYLINDRICAL_SURFACE ( 'NONE', #37053, 5.000000000000000000 ) ;
#14814=CARTESIAN_POINT ( 'NONE',  ( -2.500000000000000444, 2.833333333333333481, -4.330127018922193649 ) ) ;
#14817=CARTESIAN_POINT ( 'NONE',  ( 4.458734124999999437, -53.81249999863439371, -5.460374474430324690E-16 ) ) ;
#14818=CARTESIAN_POINT ( 'NONE',  ( -2.500000000000000444, -90.04166666393547303, -4.330127018922193649 ) ) ;
#14819=CARTESIAN_POINT ( 'NONE',  ( 2.229367062499998831, -34.64583333196772941, -3.861377020970580887 ) ) ;
#14824=CARTESIAN_POINT ( 'NONE',  ( 5.000000000000000000, -40.49999999999999289, -6.123233995736766282E-16 ) ) ;
#14825=CARTESIAN_POINT ( 'NONE',  ( -5.000000000000000000, -19.87499999726880873, 0.000000000000000000 ) ) ;
#14828=CARTESIAN_POINT ( 'NONE',  ( -2.229367062499996610, -103.1458333319677365, 3.861377020970582219 ) ) ;
#14829=CARTESIAN_POINT ( 'NONE',  ( 9.457646018065525792E-16, 2.687500001365594304, 5.148502694627439702 ) ) ;
#14830=CARTESIAN_POINT ( 'NONE',  ( 1.975475456537005874E-15, -80.74999999999998579, 5.000000000000000000 ) ) ;
#14840=CARTESIAN_POINT ( 'NONE',  ( -6.972266317189433020E-16, -11.25000000000000178, -5.000000000000000000 ) ) ;
#14844=CARTESIAN_POINT ( 'NONE',  ( -2.229367062499996610, -25.39583333196773651, 3.861377020970582219 ) ) ;
#14855=CARTESIAN_POINT ( 'NONE',  ( 4.458734124999998549, -71.97916666530107932, -2.574251347313721627 ) ) ;
#14857=VERTEX_POINT ( 'NONE', #3345 ) ;
#14862=CARTESIAN_POINT ( 'NONE',  ( -4.458734124999999437, -2.562499998634407028, 0.000000000000000000 ) ) ;
#14873=CARTESIAN_POINT ( 'NONE',  ( 4.458734124999999437, -78.81249999863440792, -5.460374474430324690E-16 ) ) ;
#14875=CARTESIAN_POINT ( 'NONE',  ( -2.229367062499996610, 1.854166668032262377, 3.861377020970582219 ) ) ;
#14876=CARTESIAN_POINT ( 'NONE',  ( -5.000000000000000000, -87.00000000000000000, 0.000000000000000000 ) ) ;
#14878=CARTESIAN_POINT ( 'NONE',  ( -4.999999999999998224, -42.79166666393548013, 2.886751345948131764 ) ) ;
#14879=CARTESIAN_POINT ( 'NONE',  ( -4.458734124999999437, -63.64583333196773651, -2.574251347313719407 ) ) ;
#14880=CARTESIAN_POINT ( 'NONE',  ( -3.535250795749689387E-16, -25.12499999726881228, -5.773502691896257311 ) ) ;
#14881=EDGE_CURVE ( 'NONE', #6575, #800, #49792, .T. ) ;
#14882=CARTESIAN_POINT ( 'NONE',  ( 1.975475456537005874E-15, -0.6249999972688137229, 5.000000000000000000 ) ) ;
#14884=CARTESIAN_POINT ( 'NONE',  ( 2.493747252781420335E-13, -43.12499999726882294, -5.000000000000000000 ) ) ;
#14885=CARTESIAN_POINT ( 'NONE',  ( -2.229367062499996610, -47.14583333196774362, 3.861377020970582219 ) ) ;
#14886=CARTESIAN_POINT ( 'NONE',  ( -4.458734124999999437, -30.56249999863440436, 0.000000000000000000 ) ) ;
#14888=( BOUNDED_CURVE ( )  B_SPLINE_CURVE ( 2, ( #32553, #37382, #47969, #13251, #3302, #2988, #42202, #3924, #52178 ),
 .UNSPECIFIED., .F., .F. ) 
 B_SPLINE_CURVE_WITH_KNOTS ( ( 3, 2, 2, 2, 3 ),
 ( 0.5410714285714285365, 0.5416666666666666297, 0.5428571428571428159, 0.5440476190476190022, 0.5446428571428570953 ),
 .UNSPECIFIED. ) 
 CURVE ( )  GEOMETRIC_REPRESENTATION_ITEM ( )  RATIONAL_B_SPLINE_CURVE ( ( 0.9330127018922194093, 0.9330127018922194093, 1.000000000000000000, 0.8660254037844387076, 1.000000000000000000, 0.8660254037844387076, 1.000000000000000000, 0.9330127018922194093, 0.9330127018922194093 ) ) 
 REPRESENTATION_ITEM ( '' )  );
#14890=CARTESIAN_POINT ( 'NONE',  ( 5.000000000000000000, 24.58333333333333215, -2.886751345948129988 ) ) ;
#14893=CARTESIAN_POINT ( 'NONE',  ( -4.458734124999998549, -36.22916666530106511, 2.574251347313722516 ) ) ;
#14894=CARTESIAN_POINT ( 'NONE',  ( -2.499999999999996447, -72.70833333060214443, 4.330127018922195425 ) ) ;
#14895=EDGE_CURVE ( 'NONE', #46124, #43789, #62954, .T. ) ;
#14899=CARTESIAN_POINT ( 'NONE',  ( -4.458734124999999437, -72.56249999863439371, 0.000000000000000000 ) ) ;
#14903=CARTESIAN_POINT ( 'NONE',  ( 0.000000000000000000, -120.0000000000000000, 0.000000000000000000 ) ) ;
#14904=CARTESIAN_POINT ( 'NONE',  ( 5.000000000000000000, -24.41666666666666430, -2.886751345948129988 ) ) ;
#14907=AXIS2_PLACEMENT_3D ( 'NONE', #5302, #59985, #36168 ) ;
#14911=CARTESIAN_POINT ( 'NONE',  ( -5.000000000000000000, 22.04166666939785202, -2.886751345948128211 ) ) ;
#14914=AXIS2_PLACEMENT_3D ( 'NONE', #57448, #13372, #61957 ) ;
#14918=CARTESIAN_POINT ( 'NONE',  ( -1.339745962155610925, -76.79465819873853150, 5.000000000000000000 ) ) ;
#14921=CARTESIAN_POINT ( 'NONE',  ( -6.972266317189433020E-16, -0.1249999972688142225, -5.000000000000000000 ) ) ;
#14922=CARTESIAN_POINT ( 'NONE',  ( 2.229367062499998831, -19.64583333196774007, -3.861377020970580887 ) ) ;
#14923=CARTESIAN_POINT ( 'NONE',  ( 6.123233995736766282E-16, -120.0000000000000000, -5.000000000000000000 ) ) ;
#14927=VERTEX_POINT ( 'NONE', #57992 ) ;
#14930=VERTEX_POINT ( 'NONE', #44124 ) ;
#14932=CARTESIAN_POINT ( 'NONE',  ( -1.339745962155613812, -68.08034179853028434, -5.000000000000000000 ) ) ;
#14939=EDGE_CURVE ( 'NONE', #62925, #47452, #49283, .T. ) ;
#14940=ORIENTED_EDGE ( 'NONE', *, *, #56329, .T. ) ;
#14944=CARTESIAN_POINT ( 'NONE',  ( 2.229367062499998831, 17.35416666803225993, -3.861377020970580887 ) ) ;
#14945=CARTESIAN_POINT ( 'NONE',  ( -1.339745962155610925, -84.79465819873851729, 5.000000000000000000 ) ) ;
#14946=VERTEX_POINT ( 'NONE', #52850 ) ;
#14949=DIRECTION ( 'NONE',  ( 0.4999999999999951150, 0.000000000000000000, -0.8660254037844414832 ) ) ;
#14952=CARTESIAN_POINT ( 'NONE',  ( 2.229367062499998831, -61.64583333196774362, -3.861377020970580887 ) ) ;
#14954=CARTESIAN_POINT ( 'NONE',  ( 2.229367062499998831, 15.35416666803225993, -3.861377020970580887 ) ) ;
#14956=AXIS2_PLACEMENT_3D ( 'NONE', #26283, #16002, #55254 ) ;
#14957=CARTESIAN_POINT ( 'NONE',  ( -6.000000000000000000, -120.0000000000000000, 1.499999999999999556 ) ) ;
#14958=CARTESIAN_POINT ( 'NONE',  ( 4.458734124999999437, -52.06249999863440792, -5.460374474430324690E-16 ) ) ;
#14959=CARTESIAN_POINT ( 'NONE',  ( 1.060575238724906964E-15, -11.62499999726881761, 5.773502691896257311 ) ) ;
#14962=CARTESIAN_POINT ( 'NONE',  ( 0.000000000000000000, -120.0000000000000000, 0.000000000000000000 ) ) ;
#14964=CARTESIAN_POINT ( 'NONE',  ( 2.229367062500001939, -106.9791666653010651, 3.861377020970579999 ) ) ;
#14965=CARTESIAN_POINT ( 'NONE',  ( 4.458734125000000326, -15.14583333196773474, 2.574251347313718519 ) ) ;
#14968=CARTESIAN_POINT ( 'NONE',  ( 4.458734124999999437, -98.81249999863440792, -5.460374474430324690E-16 ) ) ;
#14970=CARTESIAN_POINT ( 'NONE',  ( 2.229367062500001939, -98.22916666530105090, 3.861377020970579999 ) ) ;
#14972=CARTESIAN_POINT ( 'NONE',  ( -5.000000000000000000, -57.95833333060215153, -2.886751345948128211 ) ) ;
#14973=CARTESIAN_POINT ( 'NONE',  ( 1.975475456537005874E-15, -5.750000000000000000, 5.000000000000000000 ) ) ;
#14974=( BOUNDED_CURVE ( )  B_SPLINE_CURVE ( 2, ( #54972, #45952, #60128, #35042, #1598, #16375, #35994, #59485, #21522 ),
 .UNSPECIFIED., .F., .F. ) 
 B_SPLINE_CURVE_WITH_KNOTS ( ( 3, 2, 2, 2, 3 ),
 ( 0.008928571428571429811, 0.009523809523809524669, 0.01071428571428571438, 0.01190476190476190410, 0.01250000000000000069 ),
 .UNSPECIFIED. ) 
 CURVE ( )  GEOMETRIC_REPRESENTATION_ITEM ( )  RATIONAL_B_SPLINE_CURVE ( ( 0.9330127018922192983, 0.9330127018922194093, 1.000000000000000000, 0.8660254037844387076, 1.000000000000000000, 0.8660254037844387076, 1.000000000000000000, 0.9330127018922191873, 0.9330127018922192983 ) ) 
 REPRESENTATION_ITEM ( '' )  );
#14977=CARTESIAN_POINT ( 'NONE',  ( 9.457646018065525792E-16, -19.06249999863440792, 5.148502694627439702 ) ) ;
#14978=CARTESIAN_POINT ( 'NONE',  ( 4.458734125000001214, 7.854166668032260823, 2.574251347313718519 ) ) ;
#14979=CARTESIAN_POINT ( 'NONE',  ( -4.458734124999999437, -59.56249999863440081, 0.000000000000000000 ) ) ;
#14980=CARTESIAN_POINT ( 'NONE',  ( 1.339745962155612702, -94.16965819600731891, -5.000000000000000000 ) ) ;
#14982=CARTESIAN_POINT ( 'NONE',  ( 0.000000000000000000, -120.0000000000000000, 0.000000000000000000 ) ) ;
#14984=CARTESIAN_POINT ( 'NONE',  ( 5.000000000000000000, -3.500000000000003109, -6.123233995736766282E-16 ) ) ;
#14985=VERTEX_POINT ( 'NONE', #24202 ) ;
#14990=CARTESIAN_POINT ( 'NONE',  ( -2.229367062500000163, -90.47916666530106511, -3.861377020970580443 ) ) ;
#14991=CARTESIAN_POINT ( 'NONE',  ( 2.229367062499998831, 19.10416666803225993, -3.861377020970580887 ) ) ;
#14997=CARTESIAN_POINT ( 'NONE',  ( 5.000000000000000888, -74.58333333333332860, 2.886751345948126879 ) ) ;
#15000=CARTESIAN_POINT ( 'NONE',  ( 2.499999999999998668, -102.3333333333333286, -4.330127018922193649 ) ) ;
#15002=VECTOR ( 'NONE', #45794, 1000.000000000000000 ) ;
#15003=CARTESIAN_POINT ( 'NONE',  ( 1.975475456537005874E-15, -4.749999999999999112, 5.000000000000000000 ) ) ;
#15015=CARTESIAN_POINT ( 'NONE',  ( -4.458734124999999437, -56.64583333196773651, -2.574251347313719407 ) ) ;
#15026=CARTESIAN_POINT ( 'NONE',  ( -2.229367062500000163, -102.7291666653010651, -3.861377020970580443 ) ) ;
#15028=VERTEX_POINT ( 'NONE', #49597 ) ;
#15032=CARTESIAN_POINT ( 'NONE',  ( -4.458734124999999437, -43.31249999863440081, 0.000000000000000000 ) ) ;
#15034=EDGE_CURVE ( 'NONE', #20024, #1425, #54752, .T. ) ;
#15038=CARTESIAN_POINT ( 'NONE',  ( -2.229367062499996610, -15.14583333196773474, 3.861377020970582219 ) ) ;
#15039=CARTESIAN_POINT ( 'NONE',  ( 5.000000000000000000, -102.4166666666666572, -2.886751345948129988 ) ) ;
#15041=CARTESIAN_POINT ( 'NONE',  ( -1.975475456537005874E-15, 28.37500000273118772, 5.000000000000000000 ) ) ;
#15042=CARTESIAN_POINT ( 'NONE',  ( 4.458734125000001214, -34.14583333196772941, 2.574251347313718519 ) ) ;
#15043=CARTESIAN_POINT ( 'NONE',  ( 1.060575238724906964E-15, 6.375000002731185056, 5.773502691896257311 ) ) ;
#15047=ADVANCED_FACE ( 'NONE', ( #35444 ), #59254, .T. ) ;
#15051=CARTESIAN_POINT ( 'NONE',  ( 4.458734124999999437, 6.937500001365594748, -5.460374474430324690E-16 ) ) ;
#15052=( BOUNDED_CURVE ( )  B_SPLINE_CURVE ( 2, ( #59643, #59968, #60607, #40645, #10100, #40959, #50620, #5600, #1753 ),
 .UNSPECIFIED., .F., .F. ) 
 B_SPLINE_CURVE_WITH_KNOTS ( ( 3, 2, 2, 2, 3 ),
 ( 0.7446428571428571619, 0.7452380952380952550, 0.7464285714285714413, 0.7476190476190476275, 0.7482142857142857206 ),
 .UNSPECIFIED. ) 
 CURVE ( )  GEOMETRIC_REPRESENTATION_ITEM ( )  RATIONAL_B_SPLINE_CURVE ( ( 0.9330127018922194093, 0.9330127018922194093, 1.000000000000000000, 0.8660254037844387076, 1.000000000000000000, 0.8660254037844387076, 1.000000000000000000, 0.9330127018922194093, 0.9330127018922194093 ) ) 
 REPRESENTATION_ITEM ( '' )  );
#15057=CARTESIAN_POINT ( 'NONE',  ( -1.339745962155613812, -76.20534180126146850, -5.000000000000000000 ) ) ;
#15058=CARTESIAN_POINT ( 'NONE',  ( 2.499999999999998668, -98.33333333333332860, -4.330127018922193649 ) ) ;
#15059=CARTESIAN_POINT ( 'NONE',  ( -2.229367062500000163, -31.47916666530107577, -3.861377020970580443 ) ) ;
#15060=CARTESIAN_POINT ( 'NONE',  ( 2.500000000000002220, -95.66666666666664298, 4.330127018922192761 ) ) ;
#15061=CARTESIAN_POINT ( 'NONE',  ( 4.458734124999998549, -82.97916666530107932, -2.574251347313721627 ) ) ;
#15062=VECTOR ( 'NONE', #36309, 1000.000000000000000 ) ;
#15067=ADVANCED_FACE ( 'NONE', ( #55392 ), #11308, .T. ) ;
#15068=CARTESIAN_POINT ( 'NONE',  ( -2.229367062500000163, -1.479166665301071770, -3.861377020970580443 ) ) ;
#15069=CARTESIAN_POINT ( 'NONE',  ( 4.458734125000001214, 20.85416666803226349, 2.574251347313718519 ) ) ;
#15070=CARTESIAN_POINT ( 'NONE',  ( -2.229367062500000163, -44.72916666530106511, -3.861377020970580443 ) ) ;
#15073=CARTESIAN_POINT ( 'NONE',  ( 4.458734124999999437, -67.81249999863440792, -5.460374474430324690E-16 ) ) ;
#15074=CARTESIAN_POINT ( 'NONE',  ( 1.060575238724906964E-15, -106.6249999972688016, 5.773502691896257311 ) ) ;
#15076=CARTESIAN_POINT ( 'NONE',  ( 1.339745962155615144, -58.58034179853029855, 4.999999999999999112 ) ) ;
#15079=CARTESIAN_POINT ( 'NONE',  ( 2.499999999999998668, -59.33333333333333570, -4.330127018922193649 ) ) ;
#15082=ORIENTED_EDGE ( 'NONE', *, *, #40113, .T. ) ;
#15085=CARTESIAN_POINT ( 'NONE',  ( -1.339745962155610925, -98.79465819873853150, 5.000000000000000000 ) ) ;
#15092=ORIENTED_EDGE ( 'NONE', *, *, #10529, .F. ) ;
#15093=CARTESIAN_POINT ( 'NONE',  ( 5.000000000000000000, -35.29166666393547303, -2.886751345948130876 ) ) ;
#15095=EDGE_LOOP ( 'NONE', ( #18898, #20985, #48579, #36325 ) ) ;
#15099=CARTESIAN_POINT ( 'NONE',  ( 4.458734124999999437, -41.06249999863440081, -5.460374474430324690E-16 ) ) ;
#15100=CARTESIAN_POINT ( 'NONE',  ( 5.000000000000000888, -68.45833333060214443, 2.886751345948126879 ) ) ;
#15102=DIRECTION ( 'NONE',  ( 0.000000000000000000, 0.000000000000000000, 1.000000000000000000 ) ) ;
#15108=CARTESIAN_POINT ( 'NONE',  ( 2.500000000000002220, -89.66666666666665719, 4.330127018922192761 ) ) ;
#15110=CARTESIAN_POINT ( 'NONE',  ( 4.458734124999999437, -90.06249999863440792, -5.460374474430324690E-16 ) ) ;
#15113=CARTESIAN_POINT ( 'NONE',  ( -5.000000000000000000, -32.08333333333332860, -2.886751345948128211 ) ) ;
#15116=DIRECTION ( 'NONE',  ( -0.000000000000000000, 1.000000000000000000, -0.000000000000000000 ) ) ;
#15118=CARTESIAN_POINT ( 'NONE',  ( 4.458734124999999437, 3.187500001365594304, -5.460374474430324690E-16 ) ) ;
#15119=CARTESIAN_POINT ( 'NONE',  ( 5.000000000000000888, -50.45833333060213732, 2.886751345948126879 ) ) ;
#15120=CARTESIAN_POINT ( 'NONE',  ( 4.458734124999998549, -18.97916666530107221, -2.574251347313721627 ) ) ;
#15121=CARTESIAN_POINT ( 'NONE',  ( -6.972266317189433020E-16, -101.1249999972688158, -5.000000000000000000 ) ) ;
#15124=CARTESIAN_POINT ( 'NONE',  ( 2.229367062499998831, 21.10416666803226349, -3.861377020970580887 ) ) ;
#15126=CARTESIAN_POINT ( 'NONE',  ( 4.458734124999999437, -99.81249999863440792, -5.460374474430324690E-16 ) ) ;
#15129=CARTESIAN_POINT ( 'NONE',  ( 2.229367062499998831, -14.64583333196773474, -3.861377020970580887 ) ) ;
#15133=CARTESIAN_POINT ( 'NONE',  ( -5.000000000000000000, -40.95833333060215153, -2.886751345948128211 ) ) ;
#15135=CARTESIAN_POINT ( 'NONE',  ( 4.458734124999999437, 12.18750000136559564, -5.460374474430324690E-16 ) ) ;
#15136=CARTESIAN_POINT ( 'NONE',  ( -6.972266317189433020E-16, -84.24999999999998579, -5.000000000000000000 ) ) ;
#15137=CARTESIAN_POINT ( 'NONE',  ( 1.975475456537005874E-15, -87.75000000000001421, 5.000000000000000000 ) ) ;
#15139=CARTESIAN_POINT ( 'NONE',  ( -2.229367062500000163, -62.47916666530106511, -3.861377020970580443 ) ) ;
#15140=ORIENTED_EDGE ( 'NONE', *, *, #14881, .F. ) ;
#15142=VECTOR ( 'NONE', #34667, 1000.000000000000000 ) ;
#15143=CARTESIAN_POINT ( 'NONE',  ( -5.000000000000000000, 5.999999999999998224, 0.000000000000000000 ) ) ;
#15146=CARTESIAN_POINT ( 'NONE',  ( 9.457646018065525792E-16, -54.06249999863440081, 5.148502694627439702 ) ) ;
#15147=CARTESIAN_POINT ( 'NONE',  ( 5.000000000000000888, -87.45833333060214443, 2.886751345948126879 ) ) ;
#15148=AXIS2_PLACEMENT_3D ( 'NONE', #63663, #19580, #58819 ) ;
#15149=CARTESIAN_POINT ( 'NONE',  ( 4.458734124999998549, -35.72916666530107221, -2.574251347313721627 ) ) ;
#15150=DIRECTION ( 'NONE',  ( 0.000000000000000000, 0.000000000000000000, 1.000000000000000000 ) ) ;
#15152=CARTESIAN_POINT ( 'NONE',  ( -4.330127018922205195, 30.00000000000000000, -7.499999999999943157 ) ) ;
#15154=CARTESIAN_POINT ( 'NONE',  ( -5.000000000000000000, -43.00000000000000000, 0.000000000000000000 ) ) ;
#15155=CARTESIAN_POINT ( 'NONE',  ( 2.499999999999998668, -98.20833333060214443, -4.330127018922193649 ) ) ;
#15158=CARTESIAN_POINT ( 'NONE',  ( -2.229367062499996610, -100.1458333319677365, 3.861377020970582219 ) ) ;
#15159=CARTESIAN_POINT ( 'NONE',  ( -3.152548672688508926E-16, 1.187500001365596081, -5.148502694627439702 ) ) ;
#15160=DIRECTION ( 'NONE',  ( -0.000000000000000000, 1.000000000000000000, -0.000000000000000000 ) ) ;
#15166=EDGE_LOOP ( 'NONE', ( #61885, #59163, #13375, #9628 ) ) ;
#15173=CARTESIAN_POINT ( 'NONE',  ( -2.229367062500000163, -25.72916666530106866, -3.861377020970580443 ) ) ;
#15182=CARTESIAN_POINT ( 'NONE',  ( 8.660254037844342889, 45.00000000000000000, 0.000000000000000000 ) ) ;
#15184=CARTESIAN_POINT ( 'NONE',  ( -4.458734124999998549, -73.47916666530106511, 2.574251347313722516 ) ) ;
#15186=ORIENTED_EDGE ( 'NONE', *, *, #60858, .T. ) ;
#15188=VECTOR ( 'NONE', #21718, 1000.000000000000000 ) ;
#15189=CYLINDRICAL_SURFACE ( 'NONE', #44529, 5.000000000000000000 ) ;
#15192=CARTESIAN_POINT ( 'NONE',  ( 4.458734125000001214, -4.145833331967740065, 2.574251347313718519 ) ) ;
#15193=ORIENTED_EDGE ( 'NONE', *, *, #4707, .F. ) ;
#15200=EDGE_LOOP ( 'NONE', ( #10228, #11223, #4733, #47733 ) ) ;
#15201=CARTESIAN_POINT ( 'NONE',  ( 9.457646018065525792E-16, -83.06249999863439371, 5.148502694627439702 ) ) ;
#15203=CARTESIAN_POINT ( 'NONE',  ( 4.458734125000001214, 0.1041666680322607674, 2.574251347313718519 ) ) ;
#15204=CARTESIAN_POINT ( 'NONE',  ( 2.499999999999998668, -83.33333333333332860, -4.330127018922193649 ) ) ;
#15206=CARTESIAN_POINT ( 'NONE',  ( -4.458734124999999437, -65.56249999863440792, 0.000000000000000000 ) ) ;
#15207=CARTESIAN_POINT ( 'NONE',  ( -5.000000000000000000, -25.95833333060214798, -2.886751345948128211 ) ) ;
#15209=CARTESIAN_POINT ( 'NONE',  ( 2.229367062499998831, 28.35416666803225993, -3.861377020970580887 ) ) ;
#15210=DIRECTION ( 'NONE',  ( -0.000000000000000000, -1.000000000000000000, -0.000000000000000000 ) ) ;
#15212=CARTESIAN_POINT ( 'NONE',  ( 4.458734124999998549, -46.72916666530106511, -2.574251347313721627 ) ) ;
#15213=CARTESIAN_POINT ( 'NONE',  ( -2.229367062499996610, -30.39583333196773651, 3.861377020970582219 ) ) ;
#15216=CARTESIAN_POINT ( 'NONE',  ( 5.000000000000000888, 18.41666666666666430, 2.886751345948126879 ) ) ;
#15218=CARTESIAN_POINT ( 'NONE',  ( 2.500000000000002220, -54.54166666393548013, 4.330127018922192761 ) ) ;
#15219=CARTESIAN_POINT ( 'NONE',  ( 9.457646018065525792E-16, -35.06249999863440792, 5.148502694627439702 ) ) ;
#15220=CARTESIAN_POINT ( 'NONE',  ( 5.000000000000000000, -72.37499999726880162, -6.123233995736766282E-16 ) ) ;
#15222=CARTESIAN_POINT ( 'NONE',  ( 2.499999999999998668, -24.20833333060214443, -4.330127018922193649 ) ) ;
#15224=CARTESIAN_POINT ( 'NONE',  ( 9.457646018065525792E-16, -80.31249999863440792, 5.148502694627439702 ) ) ;
#15228=DIRECTION ( 'NONE',  ( 0.000000000000000000, 0.000000000000000000, 1.000000000000000000 ) ) ;
#15229=CARTESIAN_POINT ( 'NONE',  ( 5.000000000000000888, -27.58333333333333215, 2.886751345948126879 ) ) ;
#15231=ORIENTED_EDGE ( 'NONE', *, *, #25554, .F. ) ;
#15233=ORIENTED_EDGE ( 'NONE', *, *, #58244, .F. ) ;
#15235=( BOUNDED_CURVE ( )  B_SPLINE_CURVE ( 2, ( #39438, #33677, #24659, #53297, #23727, #19827, #9848, #49419, #20156 ),
 .UNSPECIFIED., .F., .F. ) 
 B_SPLINE_CURVE_WITH_KNOTS ( ( 3, 2, 2, 2, 3 ),
 ( 0.9553571428571429047, 0.9559523809523809978, 0.9571428571428571841, 0.9583333333333333703, 0.9589285714285714635 ),
 .UNSPECIFIED. ) 
 CURVE ( )  GEOMETRIC_REPRESENTATION_ITEM ( )  RATIONAL_B_SPLINE_CURVE ( ( 0.9330127018922194093, 0.9330127018922194093, 1.000000000000000000, 0.8660254037844387076, 1.000000000000000000, 0.8660254037844387076, 1.000000000000000000, 0.9330127018922194093, 0.9330127018922194093 ) ) 
 REPRESENTATION_ITEM ( '' )  );
#15236=CARTESIAN_POINT ( 'NONE',  ( 5.000000000000000888, 19.54166666939785202, 2.886751345948126879 ) ) ;
#15245=CARTESIAN_POINT ( 'NONE',  ( 2.500000000000002220, -91.54166666393547303, 4.330127018922192761 ) ) ;
#15247=DIRECTION ( 'NONE',  ( 0.000000000000000000, 0.000000000000000000, 1.000000000000000000 ) ) ;
#15248=CARTESIAN_POINT ( 'NONE',  ( -1.339745962155613812, -79.20534180126146850, -5.000000000000000000 ) ) ;
#15249=CARTESIAN_POINT ( 'NONE',  ( -4.458734124999999437, -20.31249999863440081, 0.000000000000000000 ) ) ;
#15250=CARTESIAN_POINT ( 'NONE',  ( -4.999999999999998224, -77.79166666393547303, 2.886751345948131764 ) ) ;
#15253=EDGE_CURVE ( 'NONE', #38618, #2392, #50166, .T. ) ;
#15259=EDGE_LOOP ( 'NONE', ( #38799, #13296, #11158, #43662 ) ) ;
#15260=CARTESIAN_POINT ( 'NONE',  ( 5.000000000000000888, -4.583333333333334814, 2.886751345948126879 ) ) ;
#15261=CYLINDRICAL_SURFACE ( 'NONE', #26543, 5.000000000000000000 ) ;
#15264=CARTESIAN_POINT ( 'NONE',  ( 5.000000000000000000, -23.29166666393548368, -2.886751345948130876 ) ) ;
#15268=ORIENTED_EDGE ( 'NONE', *, *, #8289, .T. ) ;
#15270=CARTESIAN_POINT ( 'NONE',  ( 1.975475456537005874E-15, -103.6249999972687874, 5.000000000000000000 ) ) ;
#15271=CARTESIAN_POINT ( 'NONE',  ( 4.458734124999998549, 11.27083333469892779, -2.574251347313721627 ) ) ;
#15274=DIRECTION ( 'NONE',  ( 0.000000000000000000, 0.000000000000000000, 1.000000000000000000 ) ) ;
#15276=( BOUNDED_CURVE ( )  B_SPLINE_CURVE ( 2, ( #27008, #2573, #18302, #37925, #36982, #37293, #22189, #46951, #12841 ),
 .UNSPECIFIED., .F., .F. ) 
 B_SPLINE_CURVE_WITH_KNOTS ( ( 3, 2, 2, 2, 3 ),
 ( 0.2482142857142857206, 0.2488095238095238138, 0.2500000000000000000, 0.2511904761904761862, 0.2517857142857142794 ),
 .UNSPECIFIED. ) 
 CURVE ( )  GEOMETRIC_REPRESENTATION_ITEM ( )  RATIONAL_B_SPLINE_CURVE ( ( 0.9330127018922194093, 0.9330127018922194093, 1.000000000000000000, 0.8660254037844387076, 1.000000000000000000, 0.8660254037844387076, 1.000000000000000000, 0.9330127018922194093, 0.9330127018922194093 ) ) 
 REPRESENTATION_ITEM ( '' )  );
#15277=CARTESIAN_POINT ( 'NONE',  ( -4.999999999999998224, -102.9166666666666714, 2.886751345948131764 ) ) ;
#15278=CARTESIAN_POINT ( 'NONE',  ( 2.229367062499998831, -67.64583333196773651, -3.861377020970580887 ) ) ;
#15279=CYLINDRICAL_SURFACE ( 'NONE', #51024, 5.000000000000000000 ) ;
#15280=CARTESIAN_POINT ( 'NONE',  ( 4.458734125000001214, 18.10416666803225638, 2.574251347313718519 ) ) ;
#15283=CARTESIAN_POINT ( 'NONE',  ( 4.458734125000001214, -49.14583333196772941, 2.574251347313718519 ) ) ;
#15284=EDGE_CURVE ( 'NONE', #32980, #62925, #43208, .T. ) ;
#15285=CARTESIAN_POINT ( 'NONE',  ( -3.535250795749689387E-16, -9.124999997268815832, -5.773502691896257311 ) ) ;
#15290=CARTESIAN_POINT ( 'NONE',  ( 4.458734124999998549, -17.97916666530106866, -2.574251347313721627 ) ) ;
#15293=CARTESIAN_POINT ( 'NONE',  ( -2.229367062499996610, -103.1458333319677365, 3.861377020970582219 ) ) ;
#15295=CARTESIAN_POINT ( 'NONE',  ( -4.458734124999999437, -97.64583333196772230, -2.574251347313719407 ) ) ;
#15296=CARTESIAN_POINT ( 'NONE',  ( -6.972266317189433020E-16, -12.24999999999999645, -5.000000000000000000 ) ) ;
#15297=CARTESIAN_POINT ( 'NONE',  ( -5.000000000000000000, -55.87499999726880162, 0.000000000000000000 ) ) ;
#15298=CARTESIAN_POINT ( 'NONE',  ( 1.339745962155612702, -62.16965819600734022, -5.000000000000000000 ) ) ;
#15302=CARTESIAN_POINT ( 'NONE',  ( 9.457646018065525792E-16, -17.06249999863440792, 5.148502694627439702 ) ) ;
#15303=CARTESIAN_POINT ( 'NONE',  ( 4.458734124999998549, 8.020833334698926009, -2.574251347313721627 ) ) ;
#15304=CARTESIAN_POINT ( 'NONE',  ( 2.229367062500001939, -66.22916666530106511, 3.861377020970579999 ) ) ;
#15305=CARTESIAN_POINT ( 'NONE',  ( 5.000000000000000000, -94.29166666393547303, -2.886751345948130876 ) ) ;
#15307=DIRECTION ( 'NONE',  ( -0.000000000000000000, 1.000000000000000000, -0.000000000000000000 ) ) ;
#15309=CARTESIAN_POINT ( 'NONE',  ( -2.500000000000000444, -5.166666666666666963, -4.330127018922193649 ) ) ;
#15311=ORIENTED_EDGE ( 'NONE', *, *, #55494, .F. ) ;
#15314=CARTESIAN_POINT ( 'NONE',  ( 5.000000000000000000, -66.50000000000000000, -6.123233995736766282E-16 ) ) ;
#15316=CARTESIAN_POINT ( 'NONE',  ( -2.229367062500000163, -88.47916666530106511, -3.861377020970580443 ) ) ;
#15317=CARTESIAN_POINT ( 'NONE',  ( 4.458734125000001214, 17.85416666803225993, 2.574251347313718519 ) ) ;
#15318=EDGE_CURVE ( 'NONE', #20975, #17776, #32840, .T. ) ;
#15323=CARTESIAN_POINT ( 'NONE',  ( 5.000000000000000888, -73.58333333333334281, 2.886751345948126879 ) ) ;
#15325=VERTEX_POINT ( 'NONE', #28004 ) ;
#15328=AXIS2_PLACEMENT_3D ( 'NONE', #17219, #41645, #51957 ) ;
#15329=FACE_OUTER_BOUND ( 'NONE', #41496, .T. ) ;
#15341=CARTESIAN_POINT ( 'NONE',  ( 2.229367062499998831, -64.89583333196773651, -3.861377020970580887 ) ) ;
#15351=CARTESIAN_POINT ( 'NONE',  ( -2.229367062499996610, -109.3958333319677365, 3.861377020970582219 ) ) ;
#15352=CARTESIAN_POINT ( 'NONE',  ( 5.000000000000000000, 20.49999999999999645, -6.123233995736766282E-16 ) ) ;
#15357=CARTESIAN_POINT ( 'NONE',  ( -3.152548672688508926E-16, -42.56249999863439371, -5.148502694627439702 ) ) ;
#15360=CARTESIAN_POINT ( 'NONE',  ( -4.458734124999997661, -49.22916666530106511, 2.574251347313722516 ) ) ;
#15361=CARTESIAN_POINT ( 'NONE',  ( 1.339745962155613146, 29.29465819873852084, 5.000000000000000888 ) ) ;
#15363=CARTESIAN_POINT ( 'NONE',  ( -2.229367062499996610, -14.14583333196774184, 3.861377020970582219 ) ) ;
#15365=CARTESIAN_POINT ( 'NONE',  ( -4.999999999999999112, -100.9166666666666430, 2.886751345948131764 ) ) ;
#15367=CARTESIAN_POINT ( 'NONE',  ( -2.229367062500000163, -31.72916666530107577, -3.861377020970580443 ) ) ;
#15368=CARTESIAN_POINT ( 'NONE',  ( 5.000000000000000000, 6.708333336064521646, -2.886751345948129988 ) ) ;
#15374=CARTESIAN_POINT ( 'NONE',  ( -6.000000000000000000, -120.0000000000000000, -1.500000000000000000 ) ) ;
#15375=CARTESIAN_POINT ( 'NONE',  ( 2.229367062499998831, -0.8958333319677401763, -3.861377020970580887 ) ) ;
#15377=CARTESIAN_POINT ( 'NONE',  ( -6.972266317189433020E-16, -57.25000000000000000, -5.000000000000000000 ) ) ;
#15378=CARTESIAN_POINT ( 'NONE',  ( 2.229367062499998831, -85.64583333196773651, -3.861377020970580887 ) ) ;
#15379=CARTESIAN_POINT ( 'NONE',  ( 9.457646018065525792E-16, -36.06249999863441502, 5.148502694627439702 ) ) ;
#15381=CARTESIAN_POINT ( 'NONE',  ( -4.458734124999998549, -80.47916666530106511, 2.574251347313722516 ) ) ;
#15387=CARTESIAN_POINT ( 'NONE',  ( -4.458734124999999437, -1.312499998634406140, 0.000000000000000000 ) ) ;
#15388=CARTESIAN_POINT ( 'NONE',  ( 2.229367062500001939, 21.77083333469892779, 3.861377020970579999 ) ) ;
#15389=CARTESIAN_POINT ( 'NONE',  ( 4.458734124999998549, -50.97916666530107221, -2.574251347313721627 ) ) ;
#15390=CARTESIAN_POINT ( 'NONE',  ( 1.339745962155612702, -15.29465819873851906, -5.000000000000000000 ) ) ;
#15395=CARTESIAN_POINT ( 'NONE',  ( -2.229367062499996610, -73.14583333196773651, 3.861377020970582219 ) ) ;
#15396=CARTESIAN_POINT ( 'NONE',  ( -5.000000000000000000, -102.9583333306021302, -2.886751345948128211 ) ) ;
#15403=CARTESIAN_POINT ( 'NONE',  ( -4.999999999999999112, -57.91666666666665719, 2.886751345948131764 ) ) ;
#15407=ORIENTED_EDGE ( 'NONE', *, *, #43238, .F. ) ;
#15409=EDGE_CURVE ( 'NONE', #7881, #19063, #48565, .T. ) ;
#15419=DIRECTION ( 'NONE',  ( -0.000000000000000000, 1.000000000000000000, -0.000000000000000000 ) ) ;
#15425=EDGE_CURVE ( 'NONE', #55214, #24763, #47724, .T. ) ;
#15427=CARTESIAN_POINT ( 'NONE',  ( 4.458734125000001214, -44.14583333196773651, 2.574251347313718519 ) ) ;
#15428=CARTESIAN_POINT ( 'NONE',  ( -6.972266317189433020E-16, -23.24999999999999645, -5.000000000000000000 ) ) ;
#15437=CARTESIAN_POINT ( 'NONE',  ( 1.243387493232115550E-13, -19.25000000000000000, -5.000000000000000000 ) ) ;
#15439=CARTESIAN_POINT ( 'NONE',  ( 2.229367062499998831, -86.89583333196773651, -3.861377020970580887 ) ) ;
#15440=ORIENTED_EDGE ( 'NONE', *, *, #8031, .T. ) ;
#15441=CARTESIAN_POINT ( 'NONE',  ( -2.500000000000000444, 13.95833333606451809, -4.330127018922193649 ) ) ;
#15442=LINE ( 'NONE', #9962, #15896 ) ;
#15444=( BOUNDED_CURVE ( )  B_SPLINE_CURVE ( 2, ( #2508, #42043, #47199, #36589, #11513, #60421, #56545, #56225, #12146 ),
 .UNSPECIFIED., .F., .F. ) 
 B_SPLINE_CURVE_WITH_KNOTS ( ( 3, 2, 2, 2, 3 ),
 ( 0.08392857142857143571, 0.08452380952380952883, 0.08571428571428571508, 0.08690476190476190133, 0.08750000000000000833 ),
 .UNSPECIFIED. ) 
 CURVE ( )  GEOMETRIC_REPRESENTATION_ITEM ( )  RATIONAL_B_SPLINE_CURVE ( ( 0.9330127018922192983, 0.9330127018922200755, 1.000000000000000000, 0.8660254037844387076, 1.000000000000000000, 0.8660254037844387076, 1.000000000000000000, 0.9330127018922185211, 0.9330127018922192983 ) ) 
 REPRESENTATION_ITEM ( '' )  );
#15445=CARTESIAN_POINT ( 'NONE',  ( 2.500000000000002220, -38.66666666666667140, 4.330127018922192761 ) ) ;
#15447=CARTESIAN_POINT ( 'NONE',  ( -4.458734124999999437, 3.604166668032260379, -2.574251347313719407 ) ) ;
#15449=CARTESIAN_POINT ( 'NONE',  ( 4.458734124999999437, -20.06249999863440081, -5.460374474430324690E-16 ) ) ;
#15452=CARTESIAN_POINT ( 'NONE',  ( -6.972266317189433020E-16, 3.875000002731185500, -5.000000000000000000 ) ) ;
#15454=CARTESIAN_POINT ( 'NONE',  ( -4.458734124999999437, 17.43750000136559208, 0.000000000000000000 ) ) ;
#15455=ORIENTED_EDGE ( 'NONE', *, *, #7134, .F. ) ;
#15456=CARTESIAN_POINT ( 'NONE',  ( 9.457646018065525792E-16, -98.06249999863440792, 5.148502694627439702 ) ) ;
#15458=CARTESIAN_POINT ( 'NONE',  ( 4.458734125000001214, -20.89583333196774007, 2.574251347313718519 ) ) ;
#15462=CARTESIAN_POINT ( 'NONE',  ( -4.999999999999999112, -43.79166666393546592, 2.886751345948131764 ) ) ;
#15464=CARTESIAN_POINT ( 'NONE',  ( -4.458734124999999437, 12.60416666803226349, -2.574251347313719407 ) ) ;
#15465=CARTESIAN_POINT ( 'NONE',  ( -2.499999999999996447, -8.708333330602144429, 4.330127018922195425 ) ) ;
#15468=CARTESIAN_POINT ( 'NONE',  ( -3.152548672688508926E-16, -59.56249999863440081, -5.148502694627439702 ) ) ;
#15469=ORIENTED_EDGE ( 'NONE', *, *, #26473, .F. ) ;
#15470=VECTOR ( 'NONE', #2830, 1000.000000000000000 ) ;
#15473=CARTESIAN_POINT ( 'NONE',  ( 2.500000000000002220, 4.333333333333331261, 4.330127018922192761 ) ) ;
#15476=CARTESIAN_POINT ( 'NONE',  ( 9.457646018065525792E-16, -59.06249999863439371, 5.148502694627439702 ) ) ;
#15477=CARTESIAN_POINT ( 'NONE',  ( -5.000000000000000000, -90.87499999726880162, 0.000000000000000000 ) ) ;
#15478=CARTESIAN_POINT ( 'NONE',  ( -4.458734124999999437, -33.31249999863440792, 0.000000000000000000 ) ) ;
#15479=FACE_OUTER_BOUND ( 'NONE', #47367, .T. ) ;
#15480=CARTESIAN_POINT ( 'NONE',  ( 1.975475456537005874E-15, -52.75000000000000000, 5.000000000000000000 ) ) ;
#15482=CARTESIAN_POINT ( 'NONE',  ( -5.000000000000000000, -49.00000000000000000, 0.000000000000000000 ) ) ;
#15484=CARTESIAN_POINT ( 'NONE',  ( 5.000000000000000000, -43.50000000000000000, -6.123233995736766282E-16 ) ) ;
#15486=CARTESIAN_POINT ( 'NONE',  ( 1.339745962155615144, -6.580341798530292330, 4.999999999999999112 ) ) ;
#15488=CARTESIAN_POINT ( 'NONE',  ( 4.458734124999998549, -103.7291666653010651, -2.574251347313721627 ) ) ;
#15489=CARTESIAN_POINT ( 'NONE',  ( 4.458734125000001214, 0.8541666680322613781, 2.574251347313718519 ) ) ;
#15490=CARTESIAN_POINT ( 'NONE',  ( 1.339745962155612702, -59.29465819873853150, -5.000000000000000000 ) ) ;
#15498=FACE_OUTER_BOUND ( 'NONE', #22388, .T. ) ;
#15500=CARTESIAN_POINT ( 'NONE',  ( 5.000000000000000000, -101.3749999972688158, -6.123233995736766282E-16 ) ) ;
#15502=EDGE_CURVE ( 'NONE', #27082, #29335, #32517, .T. ) ;
#15504=CARTESIAN_POINT ( 'NONE',  ( 4.458734125000001214, -24.14583333196773651, 2.574251347313718519 ) ) ;
#15512=ADVANCED_FACE ( 'NONE', ( #40504 ), #35695, .T. ) ;
#15515=VERTEX_POINT ( 'NONE', #20260 ) ;
#15516=CARTESIAN_POINT ( 'NONE',  ( -2.229367062499996610, -74.39583333196773651, 3.861377020970582219 ) ) ;
#15518=VERTEX_POINT ( 'NONE', #5777 ) ;
#15519=CARTESIAN_POINT ( 'NONE',  ( 1.975475456537005874E-15, 12.24999999999999822, 5.000000000000000000 ) ) ;
#15520=CARTESIAN_POINT ( 'NONE',  ( 5.000000000000000888, -31.45833333060214798, 2.886751345948126879 ) ) ;
#15521=VECTOR ( 'NONE', #15160, 1000.000000000000000 ) ;
#15523=CARTESIAN_POINT ( 'NONE',  ( -4.458734124999998549, -6.479166665301073103, 2.574251347313722516 ) ) ;
#15532=CARTESIAN_POINT ( 'NONE',  ( 2.229367062500001939, -83.97916666530106511, 3.861377020970579999 ) ) ;
#15534=CARTESIAN_POINT ( 'NONE',  ( -4.458734124999999437, 0.6041666680322611560, -2.574251347313719407 ) ) ;
#15535=DIRECTION ( 'NONE',  ( -0.000000000000000000, 1.000000000000000000, -0.000000000000000000 ) ) ;
#15536=CARTESIAN_POINT ( 'NONE',  ( -4.999999999999999112, -86.91666666666667140, 2.886751345948131764 ) ) ;
#15537=CARTESIAN_POINT ( 'NONE',  ( 1.975475456537005874E-15, -88.74999999999998579, 5.000000000000000000 ) ) ;
#15538=CARTESIAN_POINT ( 'NONE',  ( -2.229367062500000163, -67.72916666530106511, -3.861377020970580443 ) ) ;
#15539=CARTESIAN_POINT ( 'NONE',  ( 2.500000000000002220, -25.54166666393547658, 4.330127018922192761 ) ) ;
#15541=CARTESIAN_POINT ( 'NONE',  ( 5.000000000000000888, -110.4583333306021586, 2.886751345948126879 ) ) ;
#15542=CARTESIAN_POINT ( 'NONE',  ( 5.000000000000000000, -43.37499999726880873, -6.123233995736766282E-16 ) ) ;
#15543=CARTESIAN_POINT ( 'NONE',  ( -3.152548672688508926E-16, -46.56249999863440792, -5.148502694627439702 ) ) ;
#15544=CARTESIAN_POINT ( 'NONE',  ( 4.458734124999998549, -32.97916666530106511, -2.574251347313721627 ) ) ;
#15547=CARTESIAN_POINT ( 'NONE',  ( -3.535250795749689387E-16, 21.75000000000000000, -5.773502691896257311 ) ) ;
#15549=CARTESIAN_POINT ( 'NONE',  ( 0.000000000000000000, -120.0000000000000000, 5.000000000000000000 ) ) ;
#15550=CARTESIAN_POINT ( 'NONE',  ( 9.457646018065525792E-16, -39.06249999863440081, 5.148502694627439702 ) ) ;
#15551=CARTESIAN_POINT ( 'NONE',  ( 2.499999999999998668, -75.20833333060214443, -4.330127018922193649 ) ) ;
#15552=( BOUNDED_CURVE ( )  B_SPLINE_CURVE ( 2, ( #57157, #7940, #38151, #42651, #23047, #52937, #42336, #58074, #27544 ),
 .UNSPECIFIED., .F., .F. ) 
 B_SPLINE_CURVE_WITH_KNOTS ( ( 3, 2, 2, 2, 3 ),
 ( 0.1375000000000000111, 0.1380952380952381042, 0.1392857142857142905, 0.1404761904761904767, 0.1410714285714285698 ),
 .UNSPECIFIED. ) 
 CURVE ( )  GEOMETRIC_REPRESENTATION_ITEM ( )  RATIONAL_B_SPLINE_CURVE ( ( 0.9330127018922194093, 0.9330127018922194093, 1.000000000000000000, 0.8660254037844387076, 1.000000000000000000, 0.8660254037844387076, 1.000000000000000000, 0.9330127018922194093, 0.9330127018922194093 ) ) 
 REPRESENTATION_ITEM ( '' )  );
#15556=CARTESIAN_POINT ( 'NONE',  ( -2.229367062500000163, -78.72916666530106511, -3.861377020970580443 ) ) ;
#15559=CARTESIAN_POINT ( 'NONE',  ( 2.499999999999998668, 13.79166666939785202, -4.330127018922193649 ) ) ;
#15560=CARTESIAN_POINT ( 'NONE',  ( 5.000000000000000888, -29.58333333333332504, 2.886751345948126879 ) ) ;
#15562=ORIENTED_EDGE ( 'NONE', *, *, #31225, .F. ) ;
#15564=ORIENTED_EDGE ( 'NONE', *, *, #46332, .T. ) ;
#15566=CARTESIAN_POINT ( 'NONE',  ( -5.000000000000000000, 22.12500000273118417, 0.000000000000000000 ) ) ;
#15567=CARTESIAN_POINT ( 'NONE',  ( -5.000000000000000000, -60.87499999726880873, 0.000000000000000000 ) ) ;
#15575=CARTESIAN_POINT ( 'NONE',  ( 2.499999999999998668, -91.20833333060214443, -4.330127018922193649 ) ) ;
#15576=CARTESIAN_POINT ( 'NONE',  ( 5.000000000000000000, -11.37499999726881583, -6.123233995736766282E-16 ) ) ;
#15577=CARTESIAN_POINT ( 'NONE',  ( 5.000000000000000000, -56.37499999726880162, -6.123233995736766282E-16 ) ) ;
#15579=CARTESIAN_POINT ( 'NONE',  ( 2.229367062500001939, -23.97916666530107577, 3.861377020970579999 ) ) ;
#15580=CARTESIAN_POINT ( 'NONE',  ( -1.336351044127974539E-14, 24.37500000273118417, 5.000000000000000000 ) ) ;
#15584=ORIENTED_EDGE ( 'NONE', *, *, #38126, .T. ) ;
#15585=CARTESIAN_POINT ( 'NONE',  ( 1.339745962155600711, 13.29465819873851729, 5.000000000000007994 ) ) ;
#15588=CARTESIAN_POINT ( 'NONE',  ( -5.000000000000000000, -27.99999999999999645, 0.000000000000000000 ) ) ;
#15589=CARTESIAN_POINT ( 'NONE',  ( 2.500000000000002220, -9.541666663935483683, 4.330127018922192761 ) ) ;
#15591=ORIENTED_EDGE ( 'NONE', *, *, #61039, .T. ) ;
#15597=CARTESIAN_POINT ( 'NONE',  ( 4.458734124999998549, 14.27083333469892779, -2.574251347313721627 ) ) ;
#15602=CARTESIAN_POINT ( 'NONE',  ( 0.000000000000000000, -120.0000000000000000, 5.000000000000000000 ) ) ;
#15603=CARTESIAN_POINT ( 'NONE',  ( 4.458734124999999437, -62.81249999863440792, -5.460374474430324690E-16 ) ) ;
#15604=FACE_OUTER_BOUND ( 'NONE', #18590, .T. ) ;
#15605=CARTESIAN_POINT ( 'NONE',  ( -3.152548672688508926E-16, 16.43750000136559564, -5.148502694627439702 ) ) ;
#15606=EDGE_CURVE ( 'NONE', #42322, #26829, #45017, .T. ) ;
#15607=LINE ( 'NONE', #14957, #22787 ) ;
#15608=CARTESIAN_POINT ( 'NONE',  ( -2.229367062500000163, -49.72916666530107221, -3.861377020970580443 ) ) ;
#15609=CARTESIAN_POINT ( 'NONE',  ( 2.500000000000002220, -8.541666663935483683, 4.330127018922192761 ) ) ;
#15611=CARTESIAN_POINT ( 'NONE',  ( -2.499999999999996447, -65.70833333060213022, 4.330127018922195425 ) ) ;
#15613=CARTESIAN_POINT ( 'NONE',  ( 1.339745962155615144, -104.5803417985302701, 4.999999999999999112 ) ) ;
#15614=CARTESIAN_POINT ( 'NONE',  ( 9.457646018065525792E-16, -16.31249999863440436, 5.148502694627439702 ) ) ;
#15617=CARTESIAN_POINT ( 'NONE',  ( -1.339745962155610925, -46.66965819600733312, 5.000000000000000000 ) ) ;
#15618=CARTESIAN_POINT ( 'NONE',  ( 2.229367062499998831, -101.6458333319677365, -3.861377020970580887 ) ) ;
#15620=VERTEX_POINT ( 'NONE', #39539 ) ;
#15621=CARTESIAN_POINT ( 'NONE',  ( 9.457646018065525792E-16, -96.31249999863439371, 5.148502694627439702 ) ) ;
#15623=CARTESIAN_POINT ( 'NONE',  ( -5.000000000000000000, -59.87499999726880873, 0.000000000000000000 ) ) ;
#15624=CARTESIAN_POINT ( 'NONE',  ( -4.999999999999998224, 19.20833333606451632, 2.886751345948131764 ) ) ;
#15627=CARTESIAN_POINT ( 'NONE',  ( 4.458734124999998549, -16.72916666530107577, -2.574251347313721627 ) ) ;
#15628=CARTESIAN_POINT ( 'NONE',  ( 2.229367062499998831, 5.104166668032261711, -3.861377020970580887 ) ) ;
#15629=CARTESIAN_POINT ( 'NONE',  ( 4.458734124999999437, -63.06249999863440792, -5.460374474430324690E-16 ) ) ;
#15630=CARTESIAN_POINT ( 'NONE',  ( 2.500000000000002220, -94.54166666393547303, 4.330127018922192761 ) ) ;
#15634=CARTESIAN_POINT ( 'NONE',  ( -5.000000000000000000, -9.083333333333333925, -2.886751345948128211 ) ) ;
#15642=CARTESIAN_POINT ( 'NONE',  ( 0.000000000000000000, -120.0000000000000000, 0.000000000000000000 ) ) ;
#15644=DIRECTION ( 'NONE',  ( -0.4999999999999951705, 0.000000000000000000, 0.8660254037844414832 ) ) ;
#15646=CARTESIAN_POINT ( 'NONE',  ( 1.060575238724906964E-15, -74.75000000000000000, 5.773502691896257311 ) ) ;
#15648=ORIENTED_EDGE ( 'NONE', *, *, #33834, .F. ) ;
#15649=LINE ( 'NONE', #35265, #34548 ) ;
#15650=ORIENTED_EDGE ( 'NONE', *, *, #47358, .T. ) ;
#15658=CARTESIAN_POINT ( 'NONE',  ( 4.458734124999999437, -63.06249999863440792, -5.460374474430324690E-16 ) ) ;
#15661=DIRECTION ( 'NONE',  ( -0.000000000000000000, 1.000000000000000000, -0.000000000000000000 ) ) ;
#15662=ORIENTED_EDGE ( 'NONE', *, *, #45553, .T. ) ;
#15665=CARTESIAN_POINT ( 'NONE',  ( -6.972266317189433020E-16, -84.24999999999998579, -5.000000000000000000 ) ) ;
#15669=CARTESIAN_POINT ( 'NONE',  ( 9.457646018065525792E-16, 27.93750000136559208, 5.148502694627439702 ) ) ;
#15675=CARTESIAN_POINT ( 'NONE',  ( -4.458734124999997661, -45.22916666530106511, 2.574251347313722516 ) ) ;
#15678=CARTESIAN_POINT ( 'NONE',  ( 9.457646018065525792E-16, -50.06249999863440792, 5.148502694627439702 ) ) ;
#15679=CARTESIAN_POINT ( 'NONE',  ( -1.339745962155613812, -71.20534180126148271, -5.000000000000000000 ) ) ;
#15681=CARTESIAN_POINT ( 'NONE',  ( -4.458734124999999437, -16.39583333196773651, -2.574251347313719407 ) ) ;
#15682=CARTESIAN_POINT ( 'NONE',  ( 5.000000000000000000, -99.50000000000000000, -6.123233995736766282E-16 ) ) ;
#15684=CARTESIAN_POINT ( 'NONE',  ( 2.229367062499998831, -31.89583333196773651, -3.861377020970580887 ) ) ;
#15685=CARTESIAN_POINT ( 'NONE',  ( -2.499999999999996447, 6.291666669397851130, 4.330127018922195425 ) ) ;
#15686=CARTESIAN_POINT ( 'NONE',  ( -6.972266317189433020E-16, -75.12499999726880162, -5.000000000000000000 ) ) ;
#15690=CARTESIAN_POINT ( 'NONE',  ( 0.000000000000000000, -120.0000000000000000, 5.000000000000000000 ) ) ;
#15692=CARTESIAN_POINT ( 'NONE',  ( 4.458734124999998549, 1.020833334698927120, -2.574251347313721627 ) ) ;
#15696=CARTESIAN_POINT ( 'NONE',  ( 4.458734125000001214, -85.89583333196773651, 2.574251347313718519 ) ) ;
#15697=CARTESIAN_POINT ( 'NONE',  ( -3.152548672688508926E-16, -34.56249999863440792, -5.148502694627439702 ) ) ;
#15699=CARTESIAN_POINT ( 'NONE',  ( 1.975475456537005874E-15, -9.750000000000000000, 5.000000000000000000 ) ) ;
#15700=CARTESIAN_POINT ( 'NONE',  ( 9.457646018065525792E-16, -82.31249999863440792, 5.148502694627439702 ) ) ;
#15702=CARTESIAN_POINT ( 'NONE',  ( 1.975475456537005874E-15, -52.75000000000000000, 5.000000000000000000 ) ) ;
#15704=CARTESIAN_POINT ( 'NONE',  ( -4.458734124999999437, -0.3124999986344051406, 0.000000000000000000 ) ) ;
#15705=CARTESIAN_POINT ( 'NONE',  ( 4.458734124999998549, 22.02083333469892779, -2.574251347313721627 ) ) ;
#15706=EDGE_CURVE ( 'NONE', #18224, #49905, #31174, .T. ) ;
#15707=CARTESIAN_POINT ( 'NONE',  ( -3.152548672688508926E-16, -46.81249999863440792, -5.148502694627439702 ) ) ;
#15708=CARTESIAN_POINT ( 'NONE',  ( -5.000000000000000000, -45.87499999726880873, 0.000000000000000000 ) ) ;
#15713=CARTESIAN_POINT ( 'NONE',  ( -4.458734124999998549, -75.22916666530106511, 2.574251347313722516 ) ) ;
#15714=CARTESIAN_POINT ( 'NONE',  ( -4.999999999999999112, -110.7916666639354730, 2.886751345948131764 ) ) ;
#15716=CARTESIAN_POINT ( 'NONE',  ( -1.339745962155610925, -64.79465819873851729, 5.000000000000000000 ) ) ;
#15719=CARTESIAN_POINT ( 'NONE',  ( 5.000000000000000000, -61.41666666666665719, -2.886751345948129988 ) ) ;
#15720=CARTESIAN_POINT ( 'NONE',  ( -6.972266317189433020E-16, -90.12499999726880162, -5.000000000000000000 ) ) ;
#15723=CARTESIAN_POINT ( 'NONE',  ( -2.500000000000000444, -57.16666666666667140, -4.330127018922193649 ) ) ;
#15730=EDGE_CURVE ( 'NONE', #57534, #26333, #20901, .T. ) ;
#15734=CARTESIAN_POINT ( 'NONE',  ( 2.499999999999998668, -59.20833333060214443, -4.330127018922193649 ) ) ;
#15740=CARTESIAN_POINT ( 'NONE',  ( -4.458734124999998549, -45.47916666530105800, 2.574251347313722516 ) ) ;
#15741=LINE ( 'NONE', #20247, #20391 ) ;
#15750=CARTESIAN_POINT ( 'NONE',  ( 2.229367062499998831, -92.89583333196773651, -3.861377020970580887 ) ) ;
#15751=DIRECTION ( 'NONE',  ( 0.000000000000000000, 0.000000000000000000, 1.000000000000000000 ) ) ;
#15758=CARTESIAN_POINT ( 'NONE',  ( -3.152548672688508926E-16, -2.562499998634407028, -5.148502694627439702 ) ) ;
#15762=CARTESIAN_POINT ( 'NONE',  ( -6.972266317189433020E-16, 6.750000000000000000, -5.000000000000000000 ) ) ;
#15763=CARTESIAN_POINT ( 'NONE',  ( 9.457646018065525792E-16, -18.31249999863440436, 5.148502694627439702 ) ) ;
#15766=CARTESIAN_POINT ( 'NONE',  ( -5.000000000000000000, -73.87499999726880162, 0.000000000000000000 ) ) ;
#15768=CARTESIAN_POINT ( 'NONE',  ( -4.458734124999999437, 14.43750000136559386, 0.000000000000000000 ) ) ;
#15769=ORIENTED_EDGE ( 'NONE', *, *, #46703, .T. ) ;
#15771=DIRECTION ( 'NONE',  ( -0.000000000000000000, 1.000000000000000000, -0.000000000000000000 ) ) ;
#15772=CARTESIAN_POINT ( 'NONE',  ( 4.458734124999998549, -16.72916666530107577, -2.574251347313721627 ) ) ;
#15773=EDGE_CURVE ( 'NONE', #29768, #62355, #30054, .T. ) ;
#15776=CARTESIAN_POINT ( 'NONE',  ( -2.500000000000000444, -47.04166666393547303, -4.330127018922193649 ) ) ;
#15778=CARTESIAN_POINT ( 'NONE',  ( 4.458734125000000326, 16.10416666803225993, 2.574251347313718519 ) ) ;
#15779=CARTESIAN_POINT ( 'NONE',  ( 1.975475456537005874E-15, -41.74999999999999289, 5.000000000000000000 ) ) ;
#15781=DIRECTION ( 'NONE',  ( -0.000000000000000000, 1.000000000000000000, -0.000000000000000000 ) ) ;
#15783=CARTESIAN_POINT ( 'NONE',  ( 9.457646018065525792E-16, -65.06249999863440792, 5.148502694627439702 ) ) ;
#15784=EDGE_LOOP ( 'NONE', ( #27990, #60931, #25709, #19457 ) ) ;
#15786=CARTESIAN_POINT ( 'NONE',  ( 1.060575238724906964E-15, 3.249999999999999556, 5.773502691896257311 ) ) ;
#15789=CARTESIAN_POINT ( 'NONE',  ( -4.458734124999999437, -57.39583333196773651, -2.574251347313719407 ) ) ;
#15790=CARTESIAN_POINT ( 'NONE',  ( -5.000000000000000000, -94.95833333060213022, -2.886751345948128211 ) ) ;
#15791=CARTESIAN_POINT ( 'NONE',  ( -4.458734124999997661, -34.22916666530107221, 2.574251347313722516 ) ) ;
#15792=CARTESIAN_POINT ( 'NONE',  ( -6.972266317189433020E-16, 19.87500000273118417, -5.000000000000000000 ) ) ;
#15793=DIRECTION ( 'NONE',  ( 0.000000000000000000, 0.000000000000000000, 1.000000000000000000 ) ) ;
#15797=CARTESIAN_POINT ( 'NONE',  ( 5.000000000000000000, -42.49999999999999289, -6.123233995736766282E-16 ) ) ;
#15799=CARTESIAN_POINT ( 'NONE',  ( 1.339745962155612702, -86.16965819600731891, -5.000000000000000000 ) ) ;
#15800=ORIENTED_EDGE ( 'NONE', *, *, #42579, .F. ) ;
#15801=CARTESIAN_POINT ( 'NONE',  ( -4.458734124999999437, -105.3124999986344221, 0.000000000000000000 ) ) ;
#15802=CARTESIAN_POINT ( 'NONE',  ( -4.458734124999999437, 0.4375000013655955255, 0.000000000000000000 ) ) ;
#15803=CARTESIAN_POINT ( 'NONE',  ( -4.999999999999998224, -96.79166666393545881, 2.886751345948131764 ) ) ;
#15806=VECTOR ( 'NONE', #35220, 1000.000000000000000 ) ;
#15807=CARTESIAN_POINT ( 'NONE',  ( -4.999999999999998224, -25.91666666666666430, 2.886751345948131764 ) ) ;
#15812=CARTESIAN_POINT ( 'NONE',  ( 1.975475456537005874E-15, -6.749999999999999112, 5.000000000000000000 ) ) ;
#15815=CARTESIAN_POINT ( 'NONE',  ( 1.975475456537005874E-15, -101.7499999999999858, 5.000000000000000000 ) ) ;
#15817=CARTESIAN_POINT ( 'NONE',  ( 2.229367062500001939, -28.22916666530107221, 3.861377020970579999 ) ) ;
#15825=ORIENTED_EDGE ( 'NONE', *, *, #4348, .F. ) ;
#15828=CARTESIAN_POINT ( 'NONE',  ( -2.229367062499996610, -76.39583333196773651, 3.861377020970582219 ) ) ;
#15829=CARTESIAN_POINT ( 'NONE',  ( 6.123233995736766282E-16, -120.0000000000000000, -5.000000000000000000 ) ) ;
#15830=ORIENTED_EDGE ( 'NONE', *, *, #49097, .F. ) ;
#15831=CARTESIAN_POINT ( 'NONE',  ( 1.975475456537005874E-15, -14.62499999726881228, 5.000000000000000000 ) ) ;
#15835=CARTESIAN_POINT ( 'NONE',  ( -3.152548672688508926E-16, -1.812499998634406362, -5.148502694627439702 ) ) ;
#15839=CARTESIAN_POINT ( 'NONE',  ( 1.339745962155612702, -91.29465819873853150, -5.000000000000000000 ) ) ;
#15842=CARTESIAN_POINT ( 'NONE',  ( 5.000000000000000000, -47.37499999726880873, -6.123233995736766282E-16 ) ) ;
#15845=CARTESIAN_POINT ( 'NONE',  ( 4.458734124999998549, 29.02083333469893134, -2.574251347313721627 ) ) ;
#15846=ORIENTED_EDGE ( 'NONE', *, *, #2774, .T. ) ;
#15847=CARTESIAN_POINT ( 'NONE',  ( -4.458734124999999437, -82.31249999863440792, 0.000000000000000000 ) ) ;
#15848=CARTESIAN_POINT ( 'NONE',  ( 4.458734124999998549, -5.729166665301072214, -2.574251347313721627 ) ) ;
#15850=DIRECTION ( 'NONE',  ( 0.000000000000000000, 0.000000000000000000, 1.000000000000000000 ) ) ;
#15851=CARTESIAN_POINT ( 'NONE',  ( -4.458734124999999437, -72.56249999863439371, 0.000000000000000000 ) ) ;
#15852=CARTESIAN_POINT ( 'NONE',  ( -5.000000000000000000, -30.95833333060214443, -2.886751345948128211 ) ) ;
#15853=CARTESIAN_POINT ( 'NONE',  ( -4.458734124999999437, 29.68750000136559208, 0.000000000000000000 ) ) ;
#15854=CARTESIAN_POINT ( 'NONE',  ( 1.975475456537005874E-15, -3.750000000000001776, 5.000000000000000000 ) ) ;
#15857=CARTESIAN_POINT ( 'NONE',  ( 4.458734124999999437, -45.81249999863440081, -5.460374474430324690E-16 ) ) ;
#15858=CARTESIAN_POINT ( 'NONE',  ( -3.152548672688508926E-16, -33.81249999863440792, -5.148502694627439702 ) ) ;
#15861=CARTESIAN_POINT ( 'NONE',  ( -5.000000000000000000, 17.91666666666666430, -2.886751345948128211 ) ) ;
#15865=CARTESIAN_POINT ( 'NONE',  ( -4.458734124999999437, -43.39583333196774362, -2.574251347313719407 ) ) ;
#15866=CARTESIAN_POINT ( 'NONE',  ( -5.000000000000000000, -71.87499999726880162, 0.000000000000000000 ) ) ;
#15868=CARTESIAN_POINT ( 'NONE',  ( 6.123233995736766282E-16, -120.0000000000000000, -5.000000000000000000 ) ) ;
#15869=EDGE_CURVE ( 'NONE', #51679, #54583, #52249, .T. ) ;
#15871=CARTESIAN_POINT ( 'NONE',  ( -4.458734124999999437, -81.64583333196773651, -2.574251347313719407 ) ) ;
#15874=CARTESIAN_POINT ( 'NONE',  ( 5.000000000000000000, 13.70833333606451987, -2.886751345948130876 ) ) ;
#15875=CARTESIAN_POINT ( 'NONE',  ( -2.500000000000000444, -27.16666666666666430, -4.330127018922193649 ) ) ;
#15877=ORIENTED_EDGE ( 'NONE', *, *, #11497, .T. ) ;
#15879=VERTEX_POINT ( 'NONE', #46610 ) ;
#15881=CARTESIAN_POINT ( 'NONE',  ( -4.999999999999999112, 21.20833333606451987, 2.886751345948131764 ) ) ;
#15891=LINE ( 'NONE', #49340, #15002 ) ;
#15892=CARTESIAN_POINT ( 'NONE',  ( -4.458734124999999437, -15.64583333196773474, -2.574251347313719407 ) ) ;
#15896=VECTOR ( 'NONE', #35061, 1000.000000000000000 ) ;
#15898=VERTEX_POINT ( 'NONE', #2556 ) ;
#15899=CARTESIAN_POINT ( 'NONE',  ( -2.500000000000000444, 24.95833333606451987, -4.330127018922193649 ) ) ;
#15903=CARTESIAN_POINT ( 'NONE',  ( -1.339745962155613812, -86.20534180126146850, -5.000000000000000000 ) ) ;
#15905=VERTEX_POINT ( 'NONE', #37276 ) ;
#15906=CARTESIAN_POINT ( 'NONE',  ( -5.000000000000000000, -10.08333333333333393, -2.886751345948128211 ) ) ;
#15910=VERTEX_POINT ( 'NONE', #56271 ) ;
#15911=CARTESIAN_POINT ( 'NONE',  ( -5.000000000000000000, -109.8749999972688016, 0.000000000000000000 ) ) ;
#15912=CARTESIAN_POINT ( 'NONE',  ( -2.229367062500000163, 14.52083333469892779, -3.861377020970580443 ) ) ;
#15915=CARTESIAN_POINT ( 'NONE',  ( -6.972266317189433020E-16, -44.25000000000000000, -5.000000000000000000 ) ) ;
#15917=CARTESIAN_POINT ( 'NONE',  ( -2.229367062499996610, -64.14583333196773651, 3.861377020970582219 ) ) ;
#15918=CARTESIAN_POINT ( 'NONE',  ( -2.499999999999996447, -49.70833333060213732, 4.330127018922195425 ) ) ;
#15919=CARTESIAN_POINT ( 'NONE',  ( -2.229367062499996610, 10.85416666803225993, 3.861377020970582219 ) ) ;
#15923=CARTESIAN_POINT ( 'NONE',  ( -4.458734124999999437, -54.56249999863440081, 0.000000000000000000 ) ) ;
#15924=CARTESIAN_POINT ( 'NONE',  ( -4.999999999999999112, -8.791666663935483683, 2.886751345948131764 ) ) ;
#15929=CARTESIAN_POINT ( 'NONE',  ( -3.152548672688508926E-16, -18.81249999863440792, -5.148502694627439702 ) ) ;
#15930=ORIENTED_EDGE ( 'NONE', *, *, #35905, .F. ) ;
#15932=CARTESIAN_POINT ( 'NONE',  ( -2.229367062499996610, -102.1458333319677365, 3.861377020970582219 ) ) ;
#15934=ORIENTED_EDGE ( 'NONE', *, *, #14250, .T. ) ;
#15935=CARTESIAN_POINT ( 'NONE',  ( -3.152548672688508926E-16, -98.81249999863440792, -5.148502694627439702 ) ) ;
#15936=CARTESIAN_POINT ( 'NONE',  ( 4.458734124999998549, -25.72916666530107221, -2.574251347313721627 ) ) ;
#15937=CARTESIAN_POINT ( 'NONE',  ( 5.000000000000000888, -55.45833333060214443, 2.886751345948126879 ) ) ;
#15938=CARTESIAN_POINT ( 'NONE',  ( 1.975475456537005874E-15, -62.62499999726880873, 5.000000000000000000 ) ) ;
#15942=CARTESIAN_POINT ( 'NONE',  ( 2.229367062500001939, -25.97916666530106866, 3.861377020970579999 ) ) ;
#15943=CARTESIAN_POINT ( 'NONE',  ( -2.229367062500000163, -63.72916666530106511, -3.861377020970580443 ) ) ;
#15944=DIRECTION ( 'NONE',  ( 0.000000000000000000, 0.000000000000000000, 1.000000000000000000 ) ) ;
#15946=DIRECTION ( 'NONE',  ( -0.000000000000000000, 1.000000000000000000, -0.000000000000000000 ) ) ;
#15948=CARTESIAN_POINT ( 'NONE',  ( 1.060575238724906964E-15, -9.750000000000001776, 5.773502691896257311 ) ) ;
#15958=CARTESIAN_POINT ( 'NONE',  ( -6.972266317189433020E-16, -95.12499999726880162, -5.000000000000000000 ) ) ;
#15959=CARTESIAN_POINT ( 'NONE',  ( 0.000000000000000000, -120.0000000000000000, 0.000000000000000000 ) ) ;
#15961=CARTESIAN_POINT ( 'NONE',  ( -2.499999999999996447, -75.83333333333334281, 4.330127018922195425 ) ) ;
#15965=CARTESIAN_POINT ( 'NONE',  ( 6.123233995736766282E-16, -120.0000000000000000, -5.000000000000000000 ) ) ;
#15979=VERTEX_POINT ( 'NONE', #22493 ) ;
#15982=CARTESIAN_POINT ( 'NONE',  ( 9.457646018065525792E-16, -75.06249999863439371, 5.148502694627439702 ) ) ;
#15983=CARTESIAN_POINT ( 'NONE',  ( 4.458734124999999437, 27.18750000136559564, -5.460374474430324690E-16 ) ) ;
#15984=CARTESIAN_POINT ( 'NONE',  ( -6.972266317189433020E-16, 20.74999999999999645, -5.000000000000000000 ) ) ;
#15990=CARTESIAN_POINT ( 'NONE',  ( -3.152548672688508926E-16, -44.56249999863440081, -5.148502694627439702 ) ) ;
#15992=( BOUNDED_CURVE ( )  B_SPLINE_CURVE ( 2, ( #19240, #38855, #58798, #54294, #48826, #34675, #14729, #14415, #59450 ),
 .UNSPECIFIED., .F., .F. ) 
 B_SPLINE_CURVE_WITH_KNOTS ( ( 3, 2, 2, 2, 3 ),
 ( 0.3696428571428571619, 0.3702380952380952550, 0.3714285714285714413, 0.3726190476190476275, 0.3732142857142857206 ),
 .UNSPECIFIED. ) 
 CURVE ( )  GEOMETRIC_REPRESENTATION_ITEM ( )  RATIONAL_B_SPLINE_CURVE ( ( 0.9330127018922194093, 0.9330127018922194093, 1.000000000000000000, 0.8660254037844387076, 1.000000000000000000, 0.8660254037844387076, 1.000000000000000000, 0.9330127018922194093, 0.9330127018922194093 ) ) 
 REPRESENTATION_ITEM ( '' )  );
#15994=CARTESIAN_POINT ( 'NONE',  ( 4.458734124999998549, -48.72916666530106511, -2.574251347313721627 ) ) ;
#15996=CARTESIAN_POINT ( 'NONE',  ( -4.999999999999998224, -70.91666666666667140, 2.886751345948131764 ) ) ;
#15997=CARTESIAN_POINT ( 'NONE',  ( -4.458734124999999437, -18.39583333196774007, -2.574251347313719407 ) ) ;
#15998=CARTESIAN_POINT ( 'NONE',  ( -5.000000000000000000, -103.0000000000000142, 0.000000000000000000 ) ) ;
#16000=CARTESIAN_POINT ( 'NONE',  ( 4.458734124999999437, -36.06249999863440792, -5.460374474430324690E-16 ) ) ;
#16001=CARTESIAN_POINT ( 'NONE',  ( -5.000000000000000000, 6.041666669397850242, -2.886751345948128211 ) ) ;
#16002=DIRECTION ( 'NONE',  ( -0.000000000000000000, 1.000000000000000000, -0.000000000000000000 ) ) ;
#16007=CARTESIAN_POINT ( 'NONE',  ( -4.458734124999999437, -1.562499998634406140, 0.000000000000000000 ) ) ;
#16008=ORIENTED_EDGE ( 'NONE', *, *, #49514, .F. ) ;
#16009=CARTESIAN_POINT ( 'NONE',  ( 1.339745962155615144, -30.70534180126147916, 4.999999999999999112 ) ) ;
#16010=CARTESIAN_POINT ( 'NONE',  ( 5.000000000000000000, -57.41666666666667140, -2.886751345948130876 ) ) ;
#16011=CARTESIAN_POINT ( 'NONE',  ( -4.458734124999999437, -88.31249999863439371, 0.000000000000000000 ) ) ;
#16012=CARTESIAN_POINT ( 'NONE',  ( 2.229367062500001939, -33.97916666530107221, 3.861377020970579999 ) ) ;
#16014=CARTESIAN_POINT ( 'NONE',  ( 4.458734124999998549, -81.97916666530106511, -2.574251347313721627 ) ) ;
#16018=CARTESIAN_POINT ( 'NONE',  ( -2.229367062500000163, -7.479166665301073991, -3.861377020970580443 ) ) ;
#16019=CARTESIAN_POINT ( 'NONE',  ( -4.458734124999999437, 20.43750000136559208, 0.000000000000000000 ) ) ;
#16020=CARTESIAN_POINT ( 'NONE',  ( 2.229367062500001939, -49.22916666530107221, 3.861377020970579999 ) ) ;
#16021=CARTESIAN_POINT ( 'NONE',  ( 1.339745962155612702, -105.2946581987385173, -5.000000000000000000 ) ) ;
#16028=CARTESIAN_POINT ( 'NONE',  ( -2.229367062500000163, -74.47916666530106511, -3.861377020970580443 ) ) ;
#16029=CARTESIAN_POINT ( 'NONE',  ( -2.499999999999996447, -108.7083333306021444, 4.330127018922195425 ) ) ;
#16032=CYLINDRICAL_SURFACE ( 'NONE', #16255, 5.000000000000000000 ) ;
#16034=CARTESIAN_POINT ( 'NONE',  ( -5.000000000000000000, -59.08333333333334281, -2.886751345948128211 ) ) ;
#16037=ORIENTED_EDGE ( 'NONE', *, *, #8040, .F. ) ;
#16055=CARTESIAN_POINT ( 'NONE',  ( 4.458734125000001214, -49.14583333196772941, 2.574251347313718519 ) ) ;
#16056=DIRECTION ( 'NONE',  ( -0.000000000000000000, 1.000000000000000000, -0.000000000000000000 ) ) ;
#16062=ADVANCED_FACE ( 'NONE', ( #21539 ), #41767, .T. ) ;
#16066=CARTESIAN_POINT ( 'NONE',  ( -3.152548672688508926E-16, -96.81249999863440792, -5.148502694627439702 ) ) ;
#16067=CARTESIAN_POINT ( 'NONE',  ( -2.500000000000000444, -107.1666666666666572, -4.330127018922193649 ) ) ;
#16069=CARTESIAN_POINT ( 'NONE',  ( 1.339745962155612702, -19.16965819600733312, -5.000000000000000000 ) ) ;
#16072=AXIS2_PLACEMENT_3D ( 'NONE', #55199, #16276, #1496 ) ;
#16073=CARTESIAN_POINT ( 'NONE',  ( 1.975475456537005874E-15, 14.25000000000000000, 5.000000000000000000 ) ) ;
#16076=CARTESIAN_POINT ( 'NONE',  ( 4.458734125000001214, -0.8958333319677401763, 2.574251347313718519 ) ) ;
#16077=VECTOR ( 'NONE', #27865, 1000.000000000000000 ) ;
#16078=CARTESIAN_POINT ( 'NONE',  ( 5.000000000000000000, 6.583333333333333037, -2.886751345948130876 ) ) ;
#16079=CARTESIAN_POINT ( 'NONE',  ( -2.229367062500000163, -16.72916666530107577, -3.861377020970580443 ) ) ;
#16082=CARTESIAN_POINT ( 'NONE',  ( -6.972266317189433020E-16, -40.24999999999999289, -5.000000000000000000 ) ) ;
#16084=CARTESIAN_POINT ( 'NONE',  ( 2.229367062500001939, 17.77083333469892779, 3.861377020970579999 ) ) ;
#16085=ORIENTED_EDGE ( 'NONE', *, *, #25634, .F. ) ;
#16087=CARTESIAN_POINT ( 'NONE',  ( 1.975475456537005874E-15, -12.74999999999999822, 5.000000000000000000 ) ) ;
#16088=CARTESIAN_POINT ( 'NONE',  ( -4.458734124999999437, -19.31249999863440081, 0.000000000000000000 ) ) ;
#16093=CARTESIAN_POINT ( 'NONE',  ( 2.499999999999998668, -46.20833333060214443, -4.330127018922193649 ) ) ;
#16094=LINE ( 'NONE', #54700, #40170 ) ;
#16095=CARTESIAN_POINT ( 'NONE',  ( 2.229367062499998831, 10.35416666803225993, -3.861377020970580887 ) ) ;
#16097=DIRECTION ( 'NONE',  ( 0.000000000000000000, 0.000000000000000000, 1.000000000000000000 ) ) ;
#16099=CARTESIAN_POINT ( 'NONE',  ( 4.458734124999999437, -69.81249999863439371, -5.460374474430324690E-16 ) ) ;
#16101=CARTESIAN_POINT ( 'NONE',  ( -3.535250795749689387E-16, 3.750000000000000000, -5.773502691896257311 ) ) ;
#16103=CARTESIAN_POINT ( 'NONE',  ( 7.204675194429079505E-15, 25.87500000273118062, -5.000000000000000000 ) ) ;
#16104=CARTESIAN_POINT ( 'NONE',  ( 4.458734124999998549, -60.72916666530106511, -2.574251347313721627 ) ) ;
#16105=CARTESIAN_POINT ( 'NONE',  ( -5.000000000000000000, -93.95833333060213022, -2.886751345948128211 ) ) ;
#16107=CARTESIAN_POINT ( 'NONE',  ( -2.499999999999996447, -69.83333333333332860, 4.330127018922195425 ) ) ;
#16111=CARTESIAN_POINT ( 'NONE',  ( -3.535250795749689387E-16, -45.25000000000000000, -5.773502691896257311 ) ) ;
#16113=CARTESIAN_POINT ( 'NONE',  ( 2.229367062499998831, -108.6458333319677365, -3.861377020970580887 ) ) ;
#16114=CARTESIAN_POINT ( 'NONE',  ( 2.229367062499998831, -2.895833331967738289, -3.861377020970580887 ) ) ;
#16115=AXIS2_PLACEMENT_3D ( 'NONE', #22416, #41062, #57152 ) ;
#16116=CARTESIAN_POINT ( 'NONE',  ( 1.975475456537005874E-15, -30.62499999726881228, 5.000000000000000000 ) ) ;
#16121=( BOUNDED_CURVE ( )  B_SPLINE_CURVE ( 2, ( #14471, #53715, #28009, #59183, #10290, #45022, #59834, #1310, #49209 ),
 .UNSPECIFIED., .F., .F. ) 
 B_SPLINE_CURVE_WITH_KNOTS ( ( 3, 2, 2, 2, 3 ),
 ( 0.7946428571428570953, 0.7952380952380951884, 0.7964285714285713746, 0.7976190476190476719, 0.7982142857142857650 ),
 .UNSPECIFIED. ) 
 CURVE ( )  GEOMETRIC_REPRESENTATION_ITEM ( )  RATIONAL_B_SPLINE_CURVE ( ( 0.9330127018922194093, 0.9330127018922194093, 1.000000000000000000, 0.8660254037844387076, 1.000000000000000000, 0.8660254037844387076, 1.000000000000000000, 0.9330127018922194093, 0.9330127018922194093 ) ) 
 REPRESENTATION_ITEM ( '' )  );
#16123=EDGE_CURVE ( 'NONE', #11139, #53594, #54302, .T. ) ;
#16127=EDGE_LOOP ( 'NONE', ( #52588, #45230, #49890, #48221 ) ) ;
#16129=CARTESIAN_POINT ( 'NONE',  ( -4.999999999999998224, 28.20833333606451987, 2.886751345948131764 ) ) ;
#16131=EDGE_LOOP ( 'NONE', ( #60699, #36025, #56986, #60542 ) ) ;
#16132=CARTESIAN_POINT ( 'NONE',  ( 2.500000000000002220, -101.5416666639354588, 4.330127018922192761 ) ) ;
#16134=CARTESIAN_POINT ( 'NONE',  ( 4.458734124999999437, -33.06249999863440792, -5.460374474430324690E-16 ) ) ;
#16143=EDGE_CURVE ( 'NONE', #8862, #10824, #21060, .T. ) ;
#16144=CARTESIAN_POINT ( 'NONE',  ( 2.229367062499998831, -79.89583333196773651, -3.861377020970580887 ) ) ;
#16145=ORIENTED_EDGE ( 'NONE', *, *, #9091, .T. ) ;
#16146=FACE_OUTER_BOUND ( 'NONE', #62197, .T. ) ;
#16149=CARTESIAN_POINT ( 'NONE',  ( 4.458734124999999437, -4.062499998634408804, -5.460374474430324690E-16 ) ) ;
#16151=CARTESIAN_POINT ( 'NONE',  ( -1.339745962155613812, -85.20534180126148271, -5.000000000000000000 ) ) ;
#16152=CARTESIAN_POINT ( 'NONE',  ( -4.999999999999998224, 3.208333336064520758, 2.886751345948131764 ) ) ;
#16154=CARTESIAN_POINT ( 'NONE',  ( 2.499999999999998668, -27.33333333333333570, -4.330127018922193649 ) ) ;
#16158=CARTESIAN_POINT ( 'NONE',  ( 2.499999999999998668, -75.20833333060214443, -4.330127018922193649 ) ) ;
#16159=ORIENTED_EDGE ( 'NONE', *, *, #33355, .F. ) ;
#16160=CARTESIAN_POINT ( 'NONE',  ( -2.229367062500000163, -82.47916666530106511, -3.861377020970580443 ) ) ;
#16161=DIRECTION ( 'NONE',  ( 0.000000000000000000, 0.000000000000000000, 1.000000000000000000 ) ) ;
#16162=CARTESIAN_POINT ( 'NONE',  ( -4.458734124999998549, -2.229166665301068662, 2.574251347313722516 ) ) ;
#16166=CARTESIAN_POINT ( 'NONE',  ( -3.152548672688508926E-16, -72.81249999863439371, -5.148502694627439702 ) ) ;
#16168=CARTESIAN_POINT ( 'NONE',  ( -3.535250795749689387E-16, -32.12499999726880873, -5.773502691896257311 ) ) ;
#16170=CARTESIAN_POINT ( 'NONE',  ( -4.999999999999998224, -0.7916666639354794643, 2.886751345948131764 ) ) ;
#16173=CARTESIAN_POINT ( 'NONE',  ( -2.229367062500000163, -52.47916666530107221, -3.861377020970580443 ) ) ;
#16174=CARTESIAN_POINT ( 'NONE',  ( 4.458734124999998549, -33.97916666530107221, -2.574251347313721627 ) ) ;
#16177=CARTESIAN_POINT ( 'NONE',  ( 1.060575238724906964E-15, 19.25000000000000000, 5.773502691896257311 ) ) ;
#16179=CARTESIAN_POINT ( 'NONE',  ( 1.339745962155612702, -26.16965819600733312, -5.000000000000000000 ) ) ;
#16180=CARTESIAN_POINT ( 'NONE',  ( 9.457646018065525792E-16, -42.06249999863440081, 5.148502694627439702 ) ) ;
#16181=CARTESIAN_POINT ( 'NONE',  ( 2.500000000000002220, -80.54166666393547303, 4.330127018922192761 ) ) ;
#16185=CARTESIAN_POINT ( 'NONE',  ( 4.458734125000000326, -80.14583333196773651, 2.574251347313718519 ) ) ;
#16188=CARTESIAN_POINT ( 'NONE',  ( -4.999999999999999112, -25.91666666666666430, 2.886751345948131764 ) ) ;
#16190=ORIENTED_EDGE ( 'NONE', *, *, #34705, .T. ) ;
#16193=CARTESIAN_POINT ( 'NONE',  ( 5.000000000000000000, 20.62500000273118772, -6.123233995736766282E-16 ) ) ;
#16198=LINE ( 'NONE', #60280, #14359 ) ;
#16201=CARTESIAN_POINT ( 'NONE',  ( 1.339745962155615144, -99.58034179853028434, 4.999999999999999112 ) ) ;
#16202=CARTESIAN_POINT ( 'NONE',  ( 2.499999999999998668, -1.333333333333332149, -4.330127018922193649 ) ) ;
#16206=CARTESIAN_POINT ( 'NONE',  ( 1.975475456537005874E-15, -38.62499999726880873, 5.000000000000000000 ) ) ;
#16208=CARTESIAN_POINT ( 'NONE',  ( 2.229367062499998831, -11.89583333196774007, -3.861377020970580887 ) ) ;
#16210=VECTOR ( 'NONE', #13942, 1000.000000000000000 ) ;
#16222=CARTESIAN_POINT ( 'NONE',  ( 1.975475456537005874E-15, -21.75000000000000000, 5.000000000000000000 ) ) ;
#16223=CARTESIAN_POINT ( 'NONE',  ( 2.499999999999998668, -103.3333333333333286, -4.330127018922193649 ) ) ;
#16228=EDGE_CURVE ( 'NONE', #23523, #31695, #58436, .T. ) ;
#16233=ORIENTED_EDGE ( 'NONE', *, *, #37254, .F. ) ;
#16234=VECTOR ( 'NONE', #6505, 1000.000000000000000 ) ;
#16236=CARTESIAN_POINT ( 'NONE',  ( -2.500000000000000444, -110.0416666639354730, -4.330127018922193649 ) ) ;
#16237=CARTESIAN_POINT ( 'NONE',  ( -2.229367062500000163, 13.52083333469892779, -3.861377020970580443 ) ) ;
#16240=LINE ( 'NONE', #11401, #25430 ) ;
#16241=CARTESIAN_POINT ( 'NONE',  ( 2.500000000000002220, -25.66666666666666430, 4.330127018922192761 ) ) ;
#16242=ORIENTED_EDGE ( 'NONE', *, *, #50054, .F. ) ;
#16243=CARTESIAN_POINT ( 'NONE',  ( -4.458734124999997661, -66.22916666530106511, 2.574251347313722516 ) ) ;
#16245=CARTESIAN_POINT ( 'NONE',  ( 9.457646018065525792E-16, 10.93750000136559208, 5.148502694627439702 ) ) ;
#16247=CARTESIAN_POINT ( 'NONE',  ( -4.458734124999999437, -55.64583333196773651, -2.574251347313719407 ) ) ;
#16248=CARTESIAN_POINT ( 'NONE',  ( 5.000000000000000000, -17.29166666393548368, -2.886751345948129988 ) ) ;
#16252=CARTESIAN_POINT ( 'NONE',  ( 1.339745962155612702, -104.1696581960073331, -5.000000000000000000 ) ) ;
#16253=CARTESIAN_POINT ( 'NONE',  ( 4.458734125000000326, -14.14583333196774184, 2.574251347313718519 ) ) ;
#16254=ORIENTED_EDGE ( 'NONE', *, *, #41668, .T. ) ;
#16255=AXIS2_PLACEMENT_3D ( 'NONE', #50123, #46581, #45936 ) ;
#16257=CARTESIAN_POINT ( 'NONE',  ( 9.457646018065525792E-16, -105.0624999986344079, 5.148502694627439702 ) ) ;
#16259=ORIENTED_EDGE ( 'NONE', *, *, #2076, .T. ) ;
#16260=CARTESIAN_POINT ( 'NONE',  ( -4.458734124999999437, -101.5624999986344079, 0.000000000000000000 ) ) ;
#16261=VECTOR ( 'NONE', #40657, 1000.000000000000000 ) ;
#16262=CARTESIAN_POINT ( 'NONE',  ( -2.229367062499996610, -28.14583333196774007, 3.861377020970582219 ) ) ;
#16263=CARTESIAN_POINT ( 'NONE',  ( -2.500000000000000444, -61.04166666393547303, -4.330127018922193649 ) ) ;
#16266=CARTESIAN_POINT ( 'NONE',  ( -4.458734124999999437, -23.31249999863440436, 0.000000000000000000 ) ) ;
#16267=CARTESIAN_POINT ( 'NONE',  ( 4.458734124999999437, -64.06249999863440792, -5.460374474430324690E-16 ) ) ;
#16268=CARTESIAN_POINT ( 'NONE',  ( -5.000000000000000000, -39.95833333060214443, -2.886751345948128211 ) ) ;
#16272=CARTESIAN_POINT ( 'NONE',  ( 2.500000000000002220, -11.66666666666666607, 4.330127018922192761 ) ) ;
#16276=DIRECTION ( 'NONE',  ( -0.000000000000000000, 1.000000000000000000, -0.000000000000000000 ) ) ;
#16284=CARTESIAN_POINT ( 'NONE',  ( -2.499999999999996447, -78.83333333333332860, 4.330127018922195425 ) ) ;
#16287=CARTESIAN_POINT ( 'NONE',  ( -5.000000000000000000, -98.08333333333332860, -2.886751345948128211 ) ) ;
#16289=CARTESIAN_POINT ( 'NONE',  ( 7.204675194429079505E-15, 26.74999999999999645, -5.000000000000000000 ) ) ;
#16295=EDGE_LOOP ( 'NONE', ( #21198, #42556, #43882, #25228 ) ) ;
#16298=AXIS2_PLACEMENT_3D ( 'NONE', #6007, #55840, #54880 ) ;
#16300=ORIENTED_EDGE ( 'NONE', *, *, #5983, .F. ) ;
#16302=VECTOR ( 'NONE', #48940, 1000.000000000000000 ) ;
#16305=ORIENTED_EDGE ( 'NONE', *, *, #55150, .F. ) ;
#16307=EDGE_CURVE ( 'NONE', #49482, #41437, #56509, .T. ) ;
#16308=CARTESIAN_POINT ( 'NONE',  ( 2.229367062499998831, -74.64583333196773651, -3.861377020970580887 ) ) ;
#16309=CARTESIAN_POINT ( 'NONE',  ( 4.458734124999999437, -109.0624999986343937, -5.460374474430324690E-16 ) ) ;
#16311=ORIENTED_EDGE ( 'NONE', *, *, #14160, .F. ) ;
#16316=CARTESIAN_POINT ( 'NONE',  ( -2.229367062499996610, -44.14583333196774362, 3.861377020970582219 ) ) ;
#16319=CARTESIAN_POINT ( 'NONE',  ( 2.229367062499998831, -47.64583333196774362, -3.861377020970580887 ) ) ;
#16321=CARTESIAN_POINT ( 'NONE',  ( 4.458734124999999437, 27.18750000136559564, -5.460374474430324690E-16 ) ) ;
#16322=CARTESIAN_POINT ( 'NONE',  ( -2.229367062500000163, -17.47916666530106866, -3.861377020970580443 ) ) ;
#16324=CARTESIAN_POINT ( 'NONE',  ( 2.500000000000002220, -98.66666666666665719, 4.330127018922192761 ) ) ;
#16327=CARTESIAN_POINT ( 'NONE',  ( 4.458734124999998549, -37.97916666530107932, -2.574251347313721627 ) ) ;
#16328=CARTESIAN_POINT ( 'NONE',  ( 5.000000000000000000, 2.625000002731185500, -6.123233995736766282E-16 ) ) ;
#16331=CARTESIAN_POINT ( 'NONE',  ( 5.000000000000000000, 24.50000000000000000, -6.123233995736766282E-16 ) ) ;
#16333=CARTESIAN_POINT ( 'NONE',  ( -4.458734124999999437, -1.645833331967737401, -2.574251347313719407 ) ) ;
#16334=EDGE_LOOP ( 'NONE', ( #6071, #40400, #26907, #53856 ) ) ;
#16335=CARTESIAN_POINT ( 'NONE',  ( 5.000000000000000000, 24.62500000273118417, -6.123233995736766282E-16 ) ) ;
#16336=CARTESIAN_POINT ( 'NONE',  ( -1.339745962155610925, -75.79465819873853150, 5.000000000000000000 ) ) ;
#16337=CARTESIAN_POINT ( 'NONE',  ( 2.229367062500001939, -89.97916666530106511, 3.861377020970579999 ) ) ;
#16339=CARTESIAN_POINT ( 'NONE',  ( 2.229367062500001939, -86.22916666530107932, 3.861377020970579999 ) ) ;
#16343=CARTESIAN_POINT ( 'NONE',  ( -3.152548672688508926E-16, -7.562499998634404363, -5.148502694627439702 ) ) ;
#16344=CARTESIAN_POINT ( 'NONE',  ( -4.458734124999999437, 24.43750000136559208, 0.000000000000000000 ) ) ;
#16345=CARTESIAN_POINT ( 'NONE',  ( -4.458734124999999437, -47.56249999863440792, 0.000000000000000000 ) ) ;
#16354=CARTESIAN_POINT ( 'NONE',  ( 9.457646018065525792E-16, -76.06249999863440792, 5.148502694627439702 ) ) ;
#16355=CARTESIAN_POINT ( 'NONE',  ( 5.000000000000000888, -110.4583333306021586, 2.886751345948126879 ) ) ;
#16360=CARTESIAN_POINT ( 'NONE',  ( -5.000000000000000000, -63.08333333333332860, -2.886751345948128211 ) ) ;
#16364=CARTESIAN_POINT ( 'NONE',  ( -1.339745962155613812, -73.08034179853029855, -5.000000000000000000 ) ) ;
#16365=CARTESIAN_POINT ( 'NONE',  ( 1.975475456537005874E-15, -69.74999999999998579, 5.000000000000000000 ) ) ;
#16369=AXIS2_PLACEMENT_3D ( 'NONE', #36720, #37037, #2007 ) ;
#16375=CARTESIAN_POINT ( 'NONE',  ( 5.000000000000000888, 27.54166666939785557, 2.886751345948126879 ) ) ;
#16380=CARTESIAN_POINT ( 'NONE',  ( -2.229367062499996610, -46.39583333196774362, 3.861377020970582219 ) ) ;
#16381=CARTESIAN_POINT ( 'NONE',  ( -6.972266317189433020E-16, 24.87500000273118417, -5.000000000000000000 ) ) ;
#16382=( BOUNDED_CURVE ( )  B_SPLINE_CURVE ( 2, ( #3362, #8493, #42890, #7867, #46467, #47099, #36818, #62537, #3049 ),
 .UNSPECIFIED., .F., .F. ) 
 B_SPLINE_CURVE_WITH_KNOTS ( ( 3, 2, 2, 2, 3 ),
 ( 0.8482142857142856984, 0.8488095238095237915, 0.8499999999999999778, 0.8511904761904761640, 0.8517857142857142572 ),
 .UNSPECIFIED. ) 
 CURVE ( )  GEOMETRIC_REPRESENTATION_ITEM ( )  RATIONAL_B_SPLINE_CURVE ( ( 0.9330127018922194093, 0.9330127018922194093, 1.000000000000000000, 0.8660254037844387076, 1.000000000000000000, 0.8660254037844387076, 1.000000000000000000, 0.9330127018922194093, 0.9330127018922194093 ) ) 
 REPRESENTATION_ITEM ( '' )  );
#16388=CYLINDRICAL_SURFACE ( 'NONE', #607, 5.000000000000000000 ) ;
#16390=CARTESIAN_POINT ( 'NONE',  ( -4.458734124999999437, -95.64583333196772230, -2.574251347313719407 ) ) ;
#16391=DIRECTION ( 'NONE',  ( -0.000000000000000000, 1.000000000000000000, -0.000000000000000000 ) ) ;
#16399=CARTESIAN_POINT ( 'NONE',  ( 4.458734124999999437, -4.812499998634402587, -5.460374474430324690E-16 ) ) ;
#16401=CARTESIAN_POINT ( 'NONE',  ( -4.458734124999999437, -23.56249999863440436, 0.000000000000000000 ) ) ;
#16402=CARTESIAN_POINT ( 'NONE',  ( 2.499999999999998668, -72.33333333333332860, -4.330127018922193649 ) ) ;
#16406=( BOUNDED_CURVE ( )  B_SPLINE_CURVE ( 2, ( #17861, #61624, #62257, #8221, #17559, #4025, #18176, #3086, #61942 ),
 .UNSPECIFIED., .F., .F. ) 
 B_SPLINE_CURVE_WITH_KNOTS ( ( 3, 2, 2, 2, 3 ),
 ( 0.3160714285714285587, 0.3166666666666666519, 0.3178571428571428381, 0.3190476190476190244, 0.3196428571428571175 ),
 .UNSPECIFIED. ) 
 CURVE ( )  GEOMETRIC_REPRESENTATION_ITEM ( )  RATIONAL_B_SPLINE_CURVE ( ( 0.9330127018922194093, 0.9330127018922194093, 1.000000000000000000, 0.8660254037844387076, 1.000000000000000000, 0.8660254037844387076, 1.000000000000000000, 0.9330127018922194093, 0.9330127018922194093 ) ) 
 REPRESENTATION_ITEM ( '' )  );
#16407=CARTESIAN_POINT ( 'NONE',  ( -4.458734124999997661, 13.52083333469892779, 2.574251347313722516 ) ) ;
#16408=ORIENTED_EDGE ( 'NONE', *, *, #49952, .F. ) ;
#16409=CARTESIAN_POINT ( 'NONE',  ( 1.975475456537005874E-15, -13.62499999726881228, 5.000000000000000000 ) ) ;
#16410=CARTESIAN_POINT ( 'NONE',  ( -6.972266317189433020E-16, -21.24999999999999289, -5.000000000000000000 ) ) ;
#16411=CARTESIAN_POINT ( 'NONE',  ( -4.458734124999999437, -18.31249999863440792, 0.000000000000000000 ) ) ;
#16412=EDGE_CURVE ( 'NONE', #7881, #58981, #56013, .T. ) ;
#16416=CARTESIAN_POINT ( 'NONE',  ( 1.060575238724906964E-15, -45.62499999726880873, 5.773502691896257311 ) ) ;
#16417=CARTESIAN_POINT ( 'NONE',  ( -2.499999999999996447, -1.708333330602145761, 4.330127018922195425 ) ) ;
#16418=CARTESIAN_POINT ( 'NONE',  ( 4.458734125000000326, 10.10416666803226171, 2.574251347313718519 ) ) ;
#16419=DIRECTION ( 'NONE',  ( 0.000000000000000000, -1.000000000000000000, 0.000000000000000000 ) ) ;
#16422=CARTESIAN_POINT ( 'NONE',  ( 2.229367062500001939, -66.97916666530106511, 3.861377020970579999 ) ) ;
#16424=CARTESIAN_POINT ( 'NONE',  ( -2.500000000000000444, 0.8333333333333317050, -4.330127018922193649 ) ) ;
#16426=CARTESIAN_POINT ( 'NONE',  ( -1.339745962155614700, 26.33034180399265978, 4.999999999999999112 ) ) ;
#16427=CARTESIAN_POINT ( 'NONE',  ( 2.229367062499998831, -60.64583333196774362, -3.861377020970580887 ) ) ;
#16428=CARTESIAN_POINT ( 'NONE',  ( 2.500000000000002220, -94.54166666393547303, 4.330127018922192761 ) ) ;
#16430=CARTESIAN_POINT ( 'NONE',  ( -6.972266317189433020E-16, -80.24999999999998579, -5.000000000000000000 ) ) ;
#16431=CARTESIAN_POINT ( 'NONE',  ( 0.000000000000000000, -120.0000000000000000, 0.000000000000000000 ) ) ;
#16433=CARTESIAN_POINT ( 'NONE',  ( -4.999999999999998224, -90.79166666393547303, 2.886751345948131764 ) ) ;
#16434=CARTESIAN_POINT ( 'NONE',  ( -5.000000000000000000, -46.00000000000000000, 0.000000000000000000 ) ) ;
#16435=CARTESIAN_POINT ( 'NONE',  ( -6.972266317189433020E-16, -17.12499999726881583, -5.000000000000000000 ) ) ;
#16436=ORIENTED_EDGE ( 'NONE', *, *, #46497, .T. ) ;
#16437=CARTESIAN_POINT ( 'NONE',  ( 4.458734124999998549, -106.7291666653010651, -2.574251347313721627 ) ) ;
#16438=CARTESIAN_POINT ( 'NONE',  ( 4.458734124999999437, -4.062499998634408804, -5.460374474430324690E-16 ) ) ;
#16448=CARTESIAN_POINT ( 'NONE',  ( 5.000000000000000000, -22.37499999726881228, -6.123233995736766282E-16 ) ) ;
#16450=ORIENTED_EDGE ( 'NONE', *, *, #9423, .T. ) ;
#16453=CARTESIAN_POINT ( 'NONE',  ( -3.152548672688508926E-16, -29.81249999863440436, -5.148502694627439702 ) ) ;
#16461=VERTEX_POINT ( 'NONE', #32042 ) ;
#16462=CARTESIAN_POINT ( 'NONE',  ( 2.229367062499998831, -76.89583333196773651, -3.861377020970580887 ) ) ;
#16463=DIRECTION ( 'NONE',  ( 0.000000000000000000, 0.000000000000000000, 1.000000000000000000 ) ) ;
#16464=ORIENTED_EDGE ( 'NONE', *, *, #11829, .T. ) ;
#16465=LINE ( 'NONE', #20666, #41887 ) ;
#16468=CARTESIAN_POINT ( 'NONE',  ( -4.458734124999998549, -9.479166665301070438, 2.574251347313722516 ) ) ;
#16469=VERTEX_POINT ( 'NONE', #31094 ) ;
#16472=EDGE_LOOP ( 'NONE', ( #56444, #22989, #50219, #50128 ) ) ;
#16473=CARTESIAN_POINT ( 'NONE',  ( 2.500000000000002220, -91.66666666666665719, 4.330127018922192761 ) ) ;
#16475=VECTOR ( 'NONE', #53104, 1000.000000000000000 ) ;
#16476=CARTESIAN_POINT ( 'NONE',  ( -6.972266317189433020E-16, -64.24999999999998579, -5.000000000000000000 ) ) ;
#16480=CARTESIAN_POINT ( 'NONE',  ( -2.229367062499996610, -89.14583333196773651, 3.861377020970582219 ) ) ;
#16481=CARTESIAN_POINT ( 'NONE',  ( 5.000000000000000000, -29.37499999726881228, -6.123233995736766282E-16 ) ) ;
#16482=CARTESIAN_POINT ( 'NONE',  ( -2.229367062499996610, -4.145833331967739177, 3.861377020970582219 ) ) ;
#16484=EDGE_CURVE ( 'NONE', #17652, #30039, #49414, .T. ) ;
#16486=CARTESIAN_POINT ( 'NONE',  ( 1.060575238724906964E-15, -28.62499999726881228, 5.773502691896257311 ) ) ;
#16488=CARTESIAN_POINT ( 'NONE',  ( 4.458734125000000326, 24.10416666803225993, 2.574251347313718519 ) ) ;
#16489=CARTESIAN_POINT ( 'NONE',  ( 5.000000000000000000, -104.5000000000000142, -6.123233995736766282E-16 ) ) ;
#16491=CARTESIAN_POINT ( 'NONE',  ( -2.229367062500000163, -49.47916666530107221, -3.861377020970580443 ) ) ;
#16492=CARTESIAN_POINT ( 'NONE',  ( -4.458734124999999437, -35.56249999863440792, 0.000000000000000000 ) ) ;
#16494=CARTESIAN_POINT ( 'NONE',  ( 5.000000000000000000, 14.58333333333333215, -2.886751345948129988 ) ) ;
#16498=CARTESIAN_POINT ( 'NONE',  ( 4.458734125000001214, -40.89583333196773651, 2.574251347313718519 ) ) ;
#16499=CARTESIAN_POINT ( 'NONE',  ( 2.500000000000002220, -77.54166666393547303, 4.330127018922192761 ) ) ;
#16504=CARTESIAN_POINT ( 'NONE',  ( 4.458734124999999437, -84.06249999863439371, -5.460374474430324690E-16 ) ) ;
#16507=CARTESIAN_POINT ( 'NONE',  ( -2.500000000000000444, -29.16666666666666785, -4.330127018922193649 ) ) ;
#16511=ORIENTED_EDGE ( 'NONE', *, *, #51470, .F. ) ;
#16512=CARTESIAN_POINT ( 'NONE',  ( 9.457646018065525792E-16, -91.06249999863439371, 5.148502694627439702 ) ) ;
#16513=CARTESIAN_POINT ( 'NONE',  ( -2.229367062500000163, 12.27083333469892601, -3.861377020970580443 ) ) ;
#16514=CARTESIAN_POINT ( 'NONE',  ( -5.000000000000000000, 15.12500000273118417, 0.000000000000000000 ) ) ;
#16519=CARTESIAN_POINT ( 'NONE',  ( 1.339745962155612702, -61.16965819600733312, -5.000000000000000000 ) ) ;
#16523=CARTESIAN_POINT ( 'NONE',  ( -2.500000000000000444, -62.16666666666666430, -4.330127018922193649 ) ) ;
#16525=CARTESIAN_POINT ( 'NONE',  ( 1.975475456537005874E-15, -56.62499999726880162, 5.000000000000000000 ) ) ;
#16526=CARTESIAN_POINT ( 'NONE',  ( 2.229367062499998831, -16.89583333196773651, -3.861377020970580887 ) ) ;
#16527=LINE ( 'NONE', #36151, #12171 ) ;
#16537=FACE_OUTER_BOUND ( 'NONE', #48791, .T. ) ;
#16538=ORIENTED_EDGE ( 'NONE', *, *, #20941, .F. ) ;
#16539=CARTESIAN_POINT ( 'NONE',  ( -6.972266317189433020E-16, -28.25000000000000000, -5.000000000000000000 ) ) ;
#16540=CARTESIAN_POINT ( 'NONE',  ( -6.972266317189433020E-16, -86.25000000000001421, -5.000000000000000000 ) ) ;
#16542=ORIENTED_EDGE ( 'NONE', *, *, #30358, .T. ) ;
#16545=CARTESIAN_POINT ( 'NONE',  ( 1.339745962155612702, 15.70534180126147916, -5.000000000000000000 ) ) ;
#16547=ORIENTED_EDGE ( 'NONE', *, *, #8658, .T. ) ;
#16549=CARTESIAN_POINT ( 'NONE',  ( -4.458734124999998549, 15.77083333469892601, 2.574251347313722516 ) ) ;
#16554=CARTESIAN_POINT ( 'NONE',  ( 1.975475456537005874E-15, 5.249999999999999112, 5.000000000000000000 ) ) ;
#16556=CARTESIAN_POINT ( 'NONE',  ( 4.458734124999998549, -72.72916666530107932, -2.574251347313721627 ) ) ;
#16558=CARTESIAN_POINT ( 'NONE',  ( -4.458734124999999437, 10.60416666803225993, -2.574251347313719407 ) ) ;
#16559=CARTESIAN_POINT ( 'NONE',  ( -2.480964764533239819E-13, -60.62499999726880873, 5.000000000000000000 ) ) ;
#16560=EDGE_CURVE ( 'NONE', #42800, #53365, #62209, .T. ) ;
#16562=EDGE_CURVE ( 'NONE', #19510, #42943, #33936, .T. ) ;
#16563=CARTESIAN_POINT ( 'NONE',  ( 9.457646018065525792E-16, -56.31249999863440081, 5.148502694627439702 ) ) ;
#16564=CARTESIAN_POINT ( 'NONE',  ( 5.000000000000000888, -13.45833333060214976, 2.886751345948126879 ) ) ;
#16568=CARTESIAN_POINT ( 'NONE',  ( 4.458734124999998549, -19.97916666530107221, -2.574251347313721627 ) ) ;
#16569=ORIENTED_EDGE ( 'NONE', *, *, #3224, .F. ) ;
#16571=CARTESIAN_POINT ( 'NONE',  ( 4.458734124999998549, -102.7291666653010509, -2.574251347313721627 ) ) ;
#16574=CARTESIAN_POINT ( 'NONE',  ( -2.229367062500000163, -104.7291666653010651, -3.861377020970580443 ) ) ;
#16576=CARTESIAN_POINT ( 'NONE',  ( -4.458734124999998549, -28.22916666530106866, 2.574251347313722516 ) ) ;
#16577=CARTESIAN_POINT ( 'NONE',  ( 1.060575238724906964E-15, -64.62499999726881583, 5.773502691896257311 ) ) ;
#16581=CARTESIAN_POINT ( 'NONE',  ( 2.229367062500001939, -20.97916666530107221, 3.861377020970579999 ) ) ;
#16583=CARTESIAN_POINT ( 'NONE',  ( 4.458734125000000326, -66.14583333196773651, 2.574251347313718519 ) ) ;
#16585=CARTESIAN_POINT ( 'NONE',  ( -5.000000000000000000, -33.00000000000000000, 0.000000000000000000 ) ) ;
#16587=CARTESIAN_POINT ( 'NONE',  ( -2.499999999999996447, -11.83333333333333393, 4.330127018922195425 ) ) ;
#16589=ORIENTED_EDGE ( 'NONE', *, *, #8040, .T. ) ;
#16611=VERTEX_POINT ( 'NONE', #57458 ) ;
#16614=FACE_OUTER_BOUND ( 'NONE', #7997, .T. ) ;
#16615=ORIENTED_EDGE ( 'NONE', *, *, #45680, .T. ) ;
#16618=CARTESIAN_POINT ( 'NONE',  ( -2.499999999999996447, 23.29166666939785202, 4.330127018922195425 ) ) ;
#16619=ORIENTED_EDGE ( 'NONE', *, *, #38648, .T. ) ;
#16620=CARTESIAN_POINT ( 'NONE',  ( 9.457646018065525792E-16, -78.06249999863440792, 5.148502694627439702 ) ) ;
#16621=CARTESIAN_POINT ( 'NONE',  ( -4.458734124999999437, 28.60416666803226349, -2.574251347313719407 ) ) ;
#16623=ORIENTED_EDGE ( 'NONE', *, *, #62111, .F. ) ;
#16631=FACE_OUTER_BOUND ( 'NONE', #24265, .T. ) ;
#16632=CARTESIAN_POINT ( 'NONE',  ( -4.458734124999997661, -51.22916666530107932, 2.574251347313722516 ) ) ;
#16634=CARTESIAN_POINT ( 'NONE',  ( 2.229367062499998831, 28.35416666803225993, -3.861377020970580887 ) ) ;
#16635=CARTESIAN_POINT ( 'NONE',  ( 1.060575238724906964E-15, -107.7499999999999858, 5.773502691896257311 ) ) ;
#16638=CARTESIAN_POINT ( 'NONE',  ( -4.458734124999998549, -41.47916666530107221, 2.574251347313722516 ) ) ;
#16639=CARTESIAN_POINT ( 'NONE',  ( -2.499999999999996447, 3.291666669397851575, 4.330127018922195425 ) ) ;
#16644=CARTESIAN_POINT ( 'NONE',  ( -2.229367062500000163, -97.47916666530105090, -3.861377020970580443 ) ) ;
#16645=CARTESIAN_POINT ( 'NONE',  ( -4.458734124999997661, -2.479166665301069106, 2.574251347313722516 ) ) ;
#16649=CARTESIAN_POINT ( 'NONE',  ( 2.229367062499998831, -88.64583333196773651, -3.861377020970580887 ) ) ;
#16650=CYLINDRICAL_SURFACE ( 'NONE', #62365, 5.000000000000000000 ) ;
#16651=CARTESIAN_POINT ( 'NONE',  ( -4.458734124999999437, -85.56249999863439371, 0.000000000000000000 ) ) ;
#16655=CARTESIAN_POINT ( 'NONE',  ( -4.458734124999999437, -5.395833331967740953, -2.574251347313719407 ) ) ;
#16656=CARTESIAN_POINT ( 'NONE',  ( -4.458734124999999437, 15.35416666803225993, -2.574251347313719407 ) ) ;
#16657=CARTESIAN_POINT ( 'NONE',  ( -3.152548672688508926E-16, -45.81249999863440081, -5.148502694627439702 ) ) ;
#16662=ADVANCED_FACE ( 'NONE', ( #27847 ), #38749, .T. ) ;
#16664=EDGE_CURVE ( 'NONE', #15620, #63145, #24807, .T. ) ;
#16668=CARTESIAN_POINT ( 'NONE',  ( 2.229367062499998831, -72.64583333196773651, -3.861377020970580887 ) ) ;
#16669=CARTESIAN_POINT ( 'NONE',  ( 4.458734124999998549, 28.02083333469892779, -2.574251347313721627 ) ) ;
#16671=EDGE_CURVE ( 'NONE', #14946, #13464, #14090, .T. ) ;
#16672=CARTESIAN_POINT ( 'NONE',  ( -5.000000000000000000, -57.95833333060216574, -2.886751345948128211 ) ) ;
#16675=CARTESIAN_POINT ( 'NONE',  ( 2.499999999999998668, -66.33333333333332860, -4.330127018922193649 ) ) ;
#16676=CARTESIAN_POINT ( 'NONE',  ( -4.999999999999998224, -74.91666666666665719, 2.886751345948131764 ) ) ;
#16678=ORIENTED_EDGE ( 'NONE', *, *, #49262, .F. ) ;
#16679=CARTESIAN_POINT ( 'NONE',  ( -2.499999999999996447, -56.83333333333333570, 4.330127018922195425 ) ) ;
#16681=CARTESIAN_POINT ( 'NONE',  ( 0.000000000000000000, -120.0000000000000000, 5.000000000000000000 ) ) ;
#16684=APPLICATION_CONTEXT ( 'automotive_design' ) ;
#16685=CARTESIAN_POINT ( 'NONE',  ( 1.339745962155612702, -62.29465819873851729, -5.000000000000000000 ) ) ;
#16693=EDGE_LOOP ( 'NONE', ( #39071, #62638, #27848, #35700 ) ) ;
#16696=CARTESIAN_POINT ( 'NONE',  ( -2.229367062500000163, -47.72916666530106511, -3.861377020970580443 ) ) ;
#16697=DIRECTION ( 'NONE',  ( -0.000000000000000000, 1.000000000000000000, -0.000000000000000000 ) ) ;
#16704=( BOUNDED_CURVE ( )  B_SPLINE_CURVE ( 2, ( #45077, #6807, #29955, #21601, #60526, #1044, #1673, #54737, #16766 ),
 .UNSPECIFIED., .F., .F. ) 
 B_SPLINE_CURVE_WITH_KNOTS ( ( 3, 2, 2, 2, 3 ),
 ( 0.6053571428571428159, 0.6059523809523809090, 0.6071428571428570953, 0.6083333333333332815, 0.6089285714285714857 ),
 .UNSPECIFIED. ) 
 CURVE ( )  GEOMETRIC_REPRESENTATION_ITEM ( )  RATIONAL_B_SPLINE_CURVE ( ( 0.9330127018922194093, 0.9330127018922194093, 1.000000000000000000, 0.8660254037844387076, 1.000000000000000000, 0.8660254037844387076, 1.000000000000000000, 0.9330127018922130810, 0.9330127018922194093 ) ) 
 REPRESENTATION_ITEM ( '' )  );
#16708=CARTESIAN_POINT ( 'NONE',  ( 2.229367062500001939, -92.22916666530106511, 3.861377020970579999 ) ) ;
#16710=ORIENTED_EDGE ( 'NONE', *, *, #52376, .T. ) ;
#16713=CARTESIAN_POINT ( 'NONE',  ( 0.000000000000000000, -120.0000000000000000, 0.000000000000000000 ) ) ;
#16714=CARTESIAN_POINT ( 'NONE',  ( 2.229367062500001939, -3.979166665301070438, 3.861377020970579999 ) ) ;
#16717=CARTESIAN_POINT ( 'NONE',  ( -4.458734124999998549, -24.47916666530107577, 2.574251347313722516 ) ) ;
#16719=CARTESIAN_POINT ( 'NONE',  ( -6.972266317189433020E-16, -70.25000000000000000, -5.000000000000000000 ) ) ;
#16723=CARTESIAN_POINT ( 'NONE',  ( 2.229367062500001939, 15.77083333469892601, 3.861377020970579999 ) ) ;
#16726=CARTESIAN_POINT ( 'NONE',  ( -1.339745962155610925, -20.79465819873852084, 5.000000000000000000 ) ) ;
#16727=CARTESIAN_POINT ( 'NONE',  ( 1.060575238724906964E-15, -85.74999999999998579, 5.773502691896257311 ) ) ;
#16728=CARTESIAN_POINT ( 'NONE',  ( 4.458734125000001214, -16.89583333196773651, 2.574251347313718519 ) ) ;
#16729=LINE ( 'NONE', #56616, #3693 ) ;
#16732=CARTESIAN_POINT ( 'NONE',  ( 1.060575238724906964E-15, -47.62499999726881583, 5.773502691896257311 ) ) ;
#16734=CARTESIAN_POINT ( 'NONE',  ( 2.229367062499998831, 9.354166668032261711, -3.861377020970580887 ) ) ;
#16738=CARTESIAN_POINT ( 'NONE',  ( 4.458734124999998549, -67.72916666530107932, -2.574251347313721627 ) ) ;
#16740=CARTESIAN_POINT ( 'NONE',  ( -5.000000000000000000, 0.9166666666666664076, -2.886751345948128211 ) ) ;
#16742=CARTESIAN_POINT ( 'NONE',  ( 1.975475456537005874E-15, -2.750000000000000888, 5.000000000000000000 ) ) ;
#16743=CARTESIAN_POINT ( 'NONE',  ( 4.458734124999998549, -58.72916666530106511, -2.574251347313721627 ) ) ;
#16744=CARTESIAN_POINT ( 'NONE',  ( -3.535250795749689387E-16, -92.12499999726880162, -5.773502691896257311 ) ) ;
#16745=DIRECTION ( 'NONE',  ( 0.000000000000000000, 0.000000000000000000, 1.000000000000000000 ) ) ;
#16749=CARTESIAN_POINT ( 'NONE',  ( 5.000000000000000888, -46.58333333333334991, 2.886751345948126879 ) ) ;
#16750=CARTESIAN_POINT ( 'NONE',  ( -4.999999999999998224, 19.08333333333333570, 2.886751345948131764 ) ) ;
#16751=CARTESIAN_POINT ( 'NONE',  ( 0.000000000000000000, -120.0000000000000000, 0.000000000000000000 ) ) ;
#16753=CARTESIAN_POINT ( 'NONE',  ( 9.457646018065525792E-16, -105.0624999986344079, 5.148502694627439702 ) ) ;
#16754=CARTESIAN_POINT ( 'NONE',  ( 4.458734125000001214, -0.1458333319677394824, 2.574251347313718519 ) ) ;
#16755=( BOUNDED_CURVE ( )  B_SPLINE_CURVE ( 2, ( #51017, #44586, #35586, #1508, #54569, #10816, #30428, #59720, #36221 ),
 .UNSPECIFIED., .F., .F. ) 
 B_SPLINE_CURVE_WITH_KNOTS ( ( 3, 2, 2, 2, 3 ),
 ( 0.7803571428571428603, 0.7809523809523809534, 0.7821428571428571397, 0.7833333333333333259, 0.7839285714285714191 ),
 .UNSPECIFIED. ) 
 CURVE ( )  GEOMETRIC_REPRESENTATION_ITEM ( )  RATIONAL_B_SPLINE_CURVE ( ( 0.9330127018922194093, 0.9330127018922194093, 1.000000000000000000, 0.8660254037844387076, 1.000000000000000000, 0.8660254037844387076, 1.000000000000000000, 0.9330127018922194093, 0.9330127018922194093 ) ) 
 REPRESENTATION_ITEM ( '' )  );
#16763=DIRECTION ( 'NONE',  ( -0.000000000000000000, 1.000000000000000000, -0.000000000000000000 ) ) ;
#16765=ORIENTED_EDGE ( 'NONE', *, *, #21624, .F. ) ;
#16766=CARTESIAN_POINT ( 'NONE',  ( 2.493747252781420335E-13, -56.12499999726880873, -5.000000000000000000 ) ) ;
#16768=CARTESIAN_POINT ( 'NONE',  ( 4.458734125000001214, -31.14583333196773651, 2.574251347313718519 ) ) ;
#16769=CARTESIAN_POINT ( 'NONE',  ( 1.339745962155612702, -10.29465819873852084, -5.000000000000000000 ) ) ;
#16773=EDGE_CURVE ( 'NONE', #16917, #34735, #1363, .T. ) ;
#16776=CARTESIAN_POINT ( 'NONE',  ( 5.000000000000000888, -70.45833333060214443, 2.886751345948126879 ) ) ;
#16777=ORIENTED_EDGE ( 'NONE', *, *, #57115, .F. ) ;
#16778=CARTESIAN_POINT ( 'NONE',  ( 4.458734124999999437, -79.06249999863440792, -5.460374474430324690E-16 ) ) ;
#16779=CARTESIAN_POINT ( 'NONE',  ( -6.972266317189433020E-16, 3.749999999999999556, -5.000000000000000000 ) ) ;
#16783=DIRECTION ( 'NONE',  ( -0.000000000000000000, 1.000000000000000000, -0.000000000000000000 ) ) ;
#16785=CARTESIAN_POINT ( 'NONE',  ( -3.152548672688508926E-16, -11.81249999863440969, -5.148502694627439702 ) ) ;
#16787=CARTESIAN_POINT ( 'NONE',  ( -2.500000000000000444, -85.16666666666667140, -4.330127018922193649 ) ) ;
#16788=CARTESIAN_POINT ( 'NONE',  ( -5.000000000000000000, -92.87499999726881583, 0.000000000000000000 ) ) ;
#16789=VERTEX_POINT ( 'NONE', #6829 ) ;
#16790=CARTESIAN_POINT ( 'NONE',  ( 4.458734124999999437, -8.062499998634404363, -5.460374474430324690E-16 ) ) ;
#16791=CARTESIAN_POINT ( 'NONE',  ( 1.975475456537005874E-15, -32.62499999726880873, 5.000000000000000000 ) ) ;
#16797=CARTESIAN_POINT ( 'NONE',  ( 4.458734124999999437, -87.81249999863439371, -5.460374474430324690E-16 ) ) ;
#16798=CARTESIAN_POINT ( 'NONE',  ( 1.339745962155615144, -29.58034179853029499, 4.999999999999999112 ) ) ;
#16799=CARTESIAN_POINT ( 'NONE',  ( -3.152548672688508926E-16, -3.562499998634408360, -5.148502694627439702 ) ) ;
#16801=CARTESIAN_POINT ( 'NONE',  ( 2.500000000000002220, -32.54166666393547303, 4.330127018922192761 ) ) ;
#16802=CYLINDRICAL_SURFACE ( 'NONE', #35525, 5.000000000000000000 ) ;
#16803=CARTESIAN_POINT ( 'NONE',  ( -4.458734124999999437, 22.68750000136559564, 0.000000000000000000 ) ) ;
#16804=CARTESIAN_POINT ( 'NONE',  ( -6.972266317189433020E-16, -104.2500000000000000, -5.000000000000000000 ) ) ;
#16806=CARTESIAN_POINT ( 'NONE',  ( -4.458734124999999437, -53.31249999863439371, 0.000000000000000000 ) ) ;
#16807=CARTESIAN_POINT ( 'NONE',  ( -2.229367062500000163, -35.72916666530107221, -3.861377020970580443 ) ) ;
#16809=CARTESIAN_POINT ( 'NONE',  ( 5.000000000000000000, 16.58333333333333215, -2.886751345948129988 ) ) ;
#16811=CARTESIAN_POINT ( 'NONE',  ( 6.123233995736766282E-16, -120.0000000000000000, -5.000000000000000000 ) ) ;
#16812=CARTESIAN_POINT ( 'NONE',  ( -4.458734124999999437, -41.39583333196773651, -2.574251347313719407 ) ) ;
#16813=CARTESIAN_POINT ( 'NONE',  ( 2.499999999999998668, -78.20833333060214443, -4.330127018922193649 ) ) ;
#16816=LINE ( 'NONE', #42206, #14397 ) ;
#16818=CARTESIAN_POINT ( 'NONE',  ( 4.458734125000000326, -87.14583333196773651, 2.574251347313718519 ) ) ;
#16821=CARTESIAN_POINT ( 'NONE',  ( -5.000000000000000000, -32.08333333333333570, -2.886751345948128211 ) ) ;
#16823=EDGE_LOOP ( 'NONE', ( #11669, #60691, #35652, #30820, #5625, #44534, #19387, #10988, #9005, #25928, #25901, #18274 ) ) ;
#16825=ORIENTED_EDGE ( 'NONE', *, *, #33478, .T. ) ;
#16826=CARTESIAN_POINT ( 'NONE',  ( 2.229367062500001939, -92.97916666530106511, 3.861377020970579999 ) ) ;
#16827=CARTESIAN_POINT ( 'NONE',  ( 9.457646018065525792E-16, 14.68750000136559208, 5.148502694627439702 ) ) ;
#16828=CARTESIAN_POINT ( 'NONE',  ( -2.499999999999996447, 15.29166666939785202, 4.330127018922195425 ) ) ;
#16829=CARTESIAN_POINT ( 'NONE',  ( -1.339745962155610925, -34.66965819600733312, 5.000000000000000000 ) ) ;
#16836=CARTESIAN_POINT ( 'NONE',  ( 5.000000000000000000, -33.29166666393547303, -2.886751345948130876 ) ) ;
#16837=CARTESIAN_POINT ( 'NONE',  ( -5.000000000000000000, -74.87499999726880162, 0.000000000000000000 ) ) ;
#16840=CARTESIAN_POINT ( 'NONE',  ( 4.458734124999999437, -16.06249999863440436, -5.460374474430324690E-16 ) ) ;
#16849=ORIENTED_EDGE ( 'NONE', *, *, #23213, .F. ) ;
#16850=DIRECTION ( 'NONE',  ( -0.000000000000000000, 1.000000000000000000, -0.000000000000000000 ) ) ;
#16852=CARTESIAN_POINT ( 'NONE',  ( 9.457646018065525792E-16, -63.31249999863440081, 5.148502694627439702 ) ) ;
#16856=CARTESIAN_POINT ( 'NONE',  ( -6.972266317189433020E-16, -12.12499999726881583, -5.000000000000000000 ) ) ;
#16857=CARTESIAN_POINT ( 'NONE',  ( 0.000000000000000000, -120.0000000000000000, 0.000000000000000000 ) ) ;
#16864=ADVANCED_FACE ( 'NONE', ( #10124 ), #36091, .T. ) ;
#16865=AXIS2_PLACEMENT_3D ( 'NONE', #50035, #15307, #6616 ) ;
#16866=CARTESIAN_POINT ( 'NONE',  ( 2.229367062499998831, 6.354166668032262599, -3.861377020970580887 ) ) ;
#16871=CARTESIAN_POINT ( 'NONE',  ( 2.229367062500001939, -68.97916666530107932, 3.861377020970579999 ) ) ;
#16873=CARTESIAN_POINT ( 'NONE',  ( 9.457646018065525792E-16, 13.93750000136559564, 5.148502694627439702 ) ) ;
#16876=CARTESIAN_POINT ( 'NONE',  ( -6.972266317189433020E-16, -60.12499999726880873, -5.000000000000000000 ) ) ;
#16877=DIRECTION ( 'NONE',  ( -0.000000000000000000, 1.000000000000000000, -0.000000000000000000 ) ) ;
#16878=CARTESIAN_POINT ( 'NONE',  ( -2.229367062499996610, -52.39583333196773651, 3.861377020970582219 ) ) ;
#16879=CARTESIAN_POINT ( 'NONE',  ( 2.500000000000002220, -13.54166666393548013, 4.330127018922192761 ) ) ;
#16880=CARTESIAN_POINT ( 'NONE',  ( -1.339745962155610925, -32.66965819600733312, 5.000000000000000000 ) ) ;
#16883=CARTESIAN_POINT ( 'NONE',  ( 4.458734124999999437, -20.06249999863440081, -5.460374474430324690E-16 ) ) ;
#16884=ORIENTED_EDGE ( 'NONE', *, *, #7133, .F. ) ;
#16886=CARTESIAN_POINT ( 'NONE',  ( -4.458734124999998549, -109.2291666653010793, 2.574251347313722516 ) ) ;
#16888=ORIENTED_EDGE ( 'NONE', *, *, #7288, .F. ) ;
#16889=CARTESIAN_POINT ( 'NONE',  ( 4.458734124999998549, -102.9791666653010651, -2.574251347313721627 ) ) ;
#16890=CARTESIAN_POINT ( 'NONE',  ( -3.152548672688508926E-16, -26.56249999863440792, -5.148502694627439702 ) ) ;
#16891=CARTESIAN_POINT ( 'NONE',  ( -5.000000000000000000, -60.87499999726880873, 0.000000000000000000 ) ) ;
#16895=CARTESIAN_POINT ( 'NONE',  ( 4.458734124999998549, -23.72916666530107577, -2.574251347313721627 ) ) ;
#16896=CARTESIAN_POINT ( 'NONE',  ( 4.458734125000000326, -69.14583333196773651, 2.574251347313718519 ) ) ;
#16899=CARTESIAN_POINT ( 'NONE',  ( 2.499999999999998668, -32.20833333060215153, -4.330127018922193649 ) ) ;
#16901=CARTESIAN_POINT ( 'NONE',  ( -5.000000000000000000, -12.99999999999999822, 0.000000000000000000 ) ) ;
#16905=CARTESIAN_POINT ( 'NONE',  ( 5.000000000000000888, -90.58333333333332860, 2.886751345948126879 ) ) ;
#16908=VECTOR ( 'NONE', #4487, 1000.000000000000000 ) ;
#16915=ORIENTED_EDGE ( 'NONE', *, *, #16307, .F. ) ;
#16917=VERTEX_POINT ( 'NONE', #22256 ) ;
#16918=CARTESIAN_POINT ( 'NONE',  ( 5.000000000000000000, -85.41666666666665719, -2.886751345948130876 ) ) ;
#16931=( BOUNDED_CURVE ( )  B_SPLINE_CURVE ( 2, ( #53846, #18797, #4963, #62884, #63199, #48698, #10103, #156, #19109 ),
 .UNSPECIFIED., .F., .F. ) 
 B_SPLINE_CURVE_WITH_KNOTS ( ( 3, 2, 2, 2, 3 ),
 ( 0.7196428571428571397, 0.7202380952380952328, 0.7214285714285714191, 0.7226190476190476053, 0.7232142857142856984 ),
 .UNSPECIFIED. ) 
 CURVE ( )  GEOMETRIC_REPRESENTATION_ITEM ( )  RATIONAL_B_SPLINE_CURVE ( ( 0.9330127018922194093, 0.9330127018922194093, 1.000000000000000000, 0.8660254037844387076, 1.000000000000000000, 0.8660254037844387076, 1.000000000000000000, 0.9330127018922194093, 0.9330127018922194093 ) ) 
 REPRESENTATION_ITEM ( '' )  );
#16933=ORIENTED_EDGE ( 'NONE', *, *, #39284, .F. ) ;
#16936=CARTESIAN_POINT ( 'NONE',  ( -6.972266317189433020E-16, 22.87500000273118417, -5.000000000000000000 ) ) ;
#16939=CARTESIAN_POINT ( 'NONE',  ( 2.229367062500001939, -74.97916666530106511, 3.861377020970579999 ) ) ;
#16941=CARTESIAN_POINT ( 'NONE',  ( -2.229367062499996610, 24.85416666803225993, 3.861377020970582219 ) ) ;
#16942=CARTESIAN_POINT ( 'NONE',  ( -6.972266317189433020E-16, -18.25000000000000000, -5.000000000000000000 ) ) ;
#16944=CARTESIAN_POINT ( 'NONE',  ( -6.972266317189433020E-16, 4.875000002731184168, -5.000000000000000000 ) ) ;
#16948=FACE_OUTER_BOUND ( 'NONE', #12883, .T. ) ;
#16951=CARTESIAN_POINT ( 'NONE',  ( -2.229367062499996610, -57.14583333196773651, 3.861377020970582219 ) ) ;
#16953=CARTESIAN_POINT ( 'NONE',  ( -3.152548672688508926E-16, 28.43750000136559208, -5.148502694627439702 ) ) ;
#16954=CARTESIAN_POINT ( 'NONE',  ( -3.535250795749689387E-16, -107.2499999999999858, -5.773502691896257311 ) ) ;
#16957=CARTESIAN_POINT ( 'NONE',  ( 4.458734124999998549, -38.97916666530107221, -2.574251347313721627 ) ) ;
#16958=CARTESIAN_POINT ( 'NONE',  ( -2.500000000000000444, -0.04166666393548221214, -4.330127018922193649 ) ) ;
#16964=CARTESIAN_POINT ( 'NONE',  ( 2.229367062499998831, -98.64583333196773651, -3.861377020970580887 ) ) ;
#16965=CARTESIAN_POINT ( 'NONE',  ( 4.458734125000000326, -4.145833331967739177, 2.574251347313718519 ) ) ;
#16966=ORIENTED_EDGE ( 'NONE', *, *, #54232, .F. ) ;
#16968=CARTESIAN_POINT ( 'NONE',  ( -4.999999999999998224, -35.79166666393547303, 2.886751345948131764 ) ) ;
#16969=CARTESIAN_POINT ( 'NONE',  ( -4.458734124999999437, -94.31249999863440792, 0.000000000000000000 ) ) ;
#16971=CARTESIAN_POINT ( 'NONE',  ( -4.458734124999998549, -86.47916666530107932, 2.574251347313722516 ) ) ;
#16975=CARTESIAN_POINT ( 'NONE',  ( 4.458734124999999437, -6.812499998634404363, -5.460374474430324690E-16 ) ) ;
#16976=CARTESIAN_POINT ( 'NONE',  ( 2.229367062499998831, 15.10416666803225993, -3.861377020970580887 ) ) ;
#16977=CARTESIAN_POINT ( 'NONE',  ( 2.229367062500001939, -52.22916666530107221, 3.861377020970579999 ) ) ;
#16978=CARTESIAN_POINT ( 'NONE',  ( 1.339745962155615144, -11.70534180126147739, 4.999999999999999112 ) ) ;
#16981=ORIENTED_EDGE ( 'NONE', *, *, #35831, .T. ) ;
#16985=CARTESIAN_POINT ( 'NONE',  ( 4.458734125000001214, -79.89583333196773651, 2.574251347313718519 ) ) ;
#16986=CARTESIAN_POINT ( 'NONE',  ( 2.499999999999998668, -109.2083333306021444, -4.330127018922193649 ) ) ;
#16989=CARTESIAN_POINT ( 'NONE',  ( -6.972266317189433020E-16, -94.25000000000000000, -5.000000000000000000 ) ) ;
#16992=CARTESIAN_POINT ( 'NONE',  ( 5.000000000000000000, -65.41666666666665719, -2.886751345948129988 ) ) ;
#16993=DIRECTION ( 'NONE',  ( 0.000000000000000000, 0.000000000000000000, 1.000000000000000000 ) ) ;
#16995=VERTEX_POINT ( 'NONE', #26761 ) ;
#16996=CARTESIAN_POINT ( 'NONE',  ( 2.500000000000002220, -18.54166666393547658, 4.330127018922192761 ) ) ;
#16997=CARTESIAN_POINT ( 'NONE',  ( 1.975475456537005874E-15, 7.249999999999998224, 5.000000000000000000 ) ) ;
#17005=ORIENTED_EDGE ( 'NONE', *, *, #46814, .T. ) ;
#17008=VERTEX_POINT ( 'NONE', #21933 ) ;
#17011=CARTESIAN_POINT ( 'NONE',  ( 4.458734124999998549, -49.97916666530106511, -2.574251347313721627 ) ) ;
#17012=CARTESIAN_POINT ( 'NONE',  ( -2.499999999999996447, 0.2916666693978525737, 4.330127018922195425 ) ) ;
#17013=EDGE_CURVE ( 'NONE', #2252, #29860, #61813, .T. ) ;
#17017=EDGE_CURVE ( 'NONE', #58981, #50378, #7778, .T. ) ;
#17020=CARTESIAN_POINT ( 'NONE',  ( -1.339745962155610925, -58.66965819600732601, 5.000000000000000000 ) ) ;
#17023=CARTESIAN_POINT ( 'NONE',  ( 4.458734125000001214, -92.14583333196775072, 2.574251347313718519 ) ) ;
#17025=ORIENTED_EDGE ( 'NONE', *, *, #62903, .F. ) ;
#17027=DIRECTION ( 'NONE',  ( -0.000000000000000000, 1.000000000000000000, -0.000000000000000000 ) ) ;
#17030=CARTESIAN_POINT ( 'NONE',  ( 2.229367062499998831, -1.645833331967737401, -3.861377020970580887 ) ) ;
#17031=CARTESIAN_POINT ( 'NONE',  ( -4.458734124999999437, -94.64583333196773651, -2.574251347313719407 ) ) ;
#17034=CARTESIAN_POINT ( 'NONE',  ( 4.458734124999999437, -25.06249999863440792, -5.460374474430324690E-16 ) ) ;
#17035=CYLINDRICAL_SURFACE ( 'NONE', #51944, 5.000000000000000000 ) ;
#17039=CARTESIAN_POINT ( 'NONE',  ( 5.000000000000000888, 23.54166666939785202, 2.886751345948126879 ) ) ;
#17041=CARTESIAN_POINT ( 'NONE',  ( -4.458734124999999437, 11.43750000136559564, 0.000000000000000000 ) ) ;
#17045=CARTESIAN_POINT ( 'NONE',  ( -2.500000000000000444, -86.16666666666667140, -4.330127018922193649 ) ) ;
#17046=CARTESIAN_POINT ( 'NONE',  ( -4.458734124999999437, -23.31249999863440436, 0.000000000000000000 ) ) ;
#17051=CARTESIAN_POINT ( 'NONE',  ( -4.999999999999999112, -46.79166666393546592, 2.886751345948131764 ) ) ;
#17052=CARTESIAN_POINT ( 'NONE',  ( 5.000000000000000888, -24.58333333333333215, 2.886751345948126879 ) ) ;
#17053=CARTESIAN_POINT ( 'NONE',  ( -4.458734124999997661, 9.770833334698927786, 2.574251347313722516 ) ) ;
#17056=CARTESIAN_POINT ( 'NONE',  ( -2.229367062499996610, -68.14583333196773651, 3.861377020970582219 ) ) ;
#17058=CARTESIAN_POINT ( 'NONE',  ( 5.000000000000000000, -1.500000000000001332, -6.123233995736766282E-16 ) ) ;
#17060=CARTESIAN_POINT ( 'NONE',  ( -1.339745962155618253, 22.20534180126147916, 4.999999999999996447 ) ) ;
#17061=CARTESIAN_POINT ( 'NONE',  ( -3.152548672688508926E-16, -61.56249999863440792, -5.148502694627439702 ) ) ;
#17062=CARTESIAN_POINT ( 'NONE',  ( 5.000000000000000888, -92.45833333060215864, 2.886751345948126879 ) ) ;
#17064=DIRECTION ( 'NONE',  ( -0.000000000000000000, 1.000000000000000000, -0.000000000000000000 ) ) ;
#17068=CARTESIAN_POINT ( 'NONE',  ( 5.000000000000000000, -51.41666666666666430, -2.886751345948129988 ) ) ;
#17070=DIRECTION ( 'NONE',  ( 0.4999999999999948930, 0.000000000000000000, -0.8660254037844415942 ) ) ;
#17072=CARTESIAN_POINT ( 'NONE',  ( 4.458734124999999437, -105.8124999986344221, -5.460374474430324690E-16 ) ) ;
#17073=CARTESIAN_POINT ( 'NONE',  ( -2.229367062500000163, 0.2708333346989263979, -3.861377020970580443 ) ) ;
#17074=CARTESIAN_POINT ( 'NONE',  ( 1.975475456537005874E-15, 23.37500000273118417, 5.000000000000000000 ) ) ;
#17077=( BOUNDED_CURVE ( )  B_SPLINE_CURVE ( 2, ( #22860, #56952, #2300, #52121, #46343, #18010, #42451, #60830, #8064 ),
 .UNSPECIFIED., .F., .F. ) 
 B_SPLINE_CURVE_WITH_KNOTS ( ( 3, 2, 2, 2, 3 ),
 ( 0.9196428571428570953, 0.9202380952380951884, 0.9214285714285713746, 0.9226190476190476719, 0.9232142857142857650 ),
 .UNSPECIFIED. ) 
 CURVE ( )  GEOMETRIC_REPRESENTATION_ITEM ( )  RATIONAL_B_SPLINE_CURVE ( ( 0.9330127018922194093, 0.9330127018922194093, 1.000000000000000000, 0.8660254037844387076, 1.000000000000000000, 0.8660254037844387076, 1.000000000000000000, 0.9330127018922194093, 0.9330127018922194093 ) ) 
 REPRESENTATION_ITEM ( '' )  );
#17078=CARTESIAN_POINT ( 'NONE',  ( -2.500000000000000444, -31.04166666393548368, -4.330127018922193649 ) ) ;
#17088=CARTESIAN_POINT ( 'NONE',  ( -4.458734124999999437, -33.64583333196772941, -2.574251347313719407 ) ) ;
#17089=CARTESIAN_POINT ( 'NONE',  ( -4.999999999999998224, -86.91666666666667140, 2.886751345948131764 ) ) ;
#17097=CARTESIAN_POINT ( 'NONE',  ( -3.152548672688508926E-16, -79.81249999863440792, -5.148502694627439702 ) ) ;
#17098=CARTESIAN_POINT ( 'NONE',  ( 5.000000000000000000, 3.499999999999999556, -6.123233995736766282E-16 ) ) ;
#17099=ORIENTED_EDGE ( 'NONE', *, *, #46857, .F. ) ;
#17103=CARTESIAN_POINT ( 'NONE',  ( -2.229367062499996610, -10.39583333196773829, 3.861377020970582219 ) ) ;
#17107=CARTESIAN_POINT ( 'NONE',  ( -4.458734124999998549, -4.479166665301070438, 2.574251347313722516 ) ) ;
#17112=DIRECTION ( 'NONE',  ( -0.000000000000000000, 1.000000000000000000, -0.000000000000000000 ) ) ;
#17114=CARTESIAN_POINT ( 'NONE',  ( -2.229367062499996610, -85.14583333196773651, 3.861377020970582219 ) ) ;
#17115=CARTESIAN_POINT ( 'NONE',  ( 1.975475456537005874E-15, -20.62499999726881228, 5.000000000000000000 ) ) ;
#17116=CARTESIAN_POINT ( 'NONE',  ( 4.458734125000001214, -3.895833331967739621, 2.574251347313718519 ) ) ;
#17118=CARTESIAN_POINT ( 'NONE',  ( -5.000000000000000000, -31.95833333060214443, -2.886751345948128211 ) ) ;
#17120=CARTESIAN_POINT ( 'NONE',  ( -4.458734124999997661, 25.77083333469893134, 2.574251347313722516 ) ) ;
#17123=CARTESIAN_POINT ( 'NONE',  ( -2.229367062499996610, -50.14583333196772941, 3.861377020970582219 ) ) ;
#17124=CARTESIAN_POINT ( 'NONE',  ( 9.457646018065525792E-16, -38.31249999863440792, 5.148502694627439702 ) ) ;
#17126=( BOUNDED_CURVE ( )  B_SPLINE_CURVE ( 2, ( #28214, #22782, #33056, #51732, #3788, #23410, #16996, #32096, #2846 ),
 .UNSPECIFIED., .F., .F. ) 
 B_SPLINE_CURVE_WITH_KNOTS ( ( 3, 2, 2, 2, 3 ),
 ( 0.3375000000000000222, 0.3380952380952381153, 0.3392857142857143016, 0.3404761904761904878, 0.3410714285714285809 ),
 .UNSPECIFIED. ) 
 CURVE ( )  GEOMETRIC_REPRESENTATION_ITEM ( )  RATIONAL_B_SPLINE_CURVE ( ( 0.9330127018922194093, 0.9330127018922194093, 1.000000000000000000, 0.8660254037844387076, 1.000000000000000000, 0.8660254037844387076, 1.000000000000000000, 0.9330127018922194093, 0.9330127018922194093 ) ) 
 REPRESENTATION_ITEM ( '' )  );
#17128=CARTESIAN_POINT ( 'NONE',  ( 6.158835246850667461E-14, 8.875000002731182391, -4.999999999999999112 ) ) ;
#17129=CARTESIAN_POINT ( 'NONE',  ( -4.999999999999999112, 14.08333333333333393, 2.886751345948131764 ) ) ;
#17131=DIRECTION ( 'NONE',  ( 0.000000000000000000, 0.000000000000000000, 1.000000000000000000 ) ) ;
#17132=CARTESIAN_POINT ( 'NONE',  ( 4.458734125000001214, -42.89583333196773651, 2.574251347313718519 ) ) ;
#17133=CARTESIAN_POINT ( 'NONE',  ( 1.060575238724906964E-15, -76.62499999726881583, 5.773502691896257311 ) ) ;
#17135=VECTOR ( 'NONE', #36815, 1000.000000000000000 ) ;
#17137=CARTESIAN_POINT ( 'NONE',  ( -6.972266317189433020E-16, -27.24999999999999645, -5.000000000000000000 ) ) ;
#17138=CARTESIAN_POINT ( 'NONE',  ( 1.975475456537005874E-15, -76.62499999726880162, 5.000000000000000000 ) ) ;
#17139=CARTESIAN_POINT ( 'NONE',  ( -4.458734124999999437, -83.56249999863439371, 0.000000000000000000 ) ) ;
#17141=CARTESIAN_POINT ( 'NONE',  ( -2.499999999999996447, -31.83333333333333215, 4.330127018922195425 ) ) ;
#17145=ORIENTED_EDGE ( 'NONE', *, *, #30747, .F. ) ;
#17146=CARTESIAN_POINT ( 'NONE',  ( -4.458734124999999437, -88.39583333196773651, -2.574251347313719407 ) ) ;
#17147=CARTESIAN_POINT ( 'NONE',  ( 4.458734124999998549, 11.02083333469892779, -2.574251347313721627 ) ) ;
#17148=CARTESIAN_POINT ( 'NONE',  ( -2.500000000000000444, 13.95833333606451809, -4.330127018922193649 ) ) ;
#17153=CARTESIAN_POINT ( 'NONE',  ( -1.339745962155613812, -52.20534180126148271, -5.000000000000000000 ) ) ;
#17158=CARTESIAN_POINT ( 'NONE',  ( 2.500000000000002220, -107.6666666666666572, 4.330127018922192761 ) ) ;
#17159=( BOUNDED_CURVE ( )  B_SPLINE_CURVE ( 2, ( #52564, #8497, #47722, #3680, #3989, #23294, #18462, #33254, #52874 ),
 .UNSPECIFIED., .F., .F. ) 
 B_SPLINE_CURVE_WITH_KNOTS ( ( 3, 2, 2, 2, 3 ),
 ( 0.5089285714285713969, 0.5095238095238094900, 0.5107142857142856762, 0.5119047619047618625, 0.5124999999999999556 ),
 .UNSPECIFIED. ) 
 CURVE ( )  GEOMETRIC_REPRESENTATION_ITEM ( )  RATIONAL_B_SPLINE_CURVE ( ( 0.9330127018922194093, 0.9330127018922194093, 1.000000000000000000, 0.8660254037844387076, 1.000000000000000000, 0.8660254037844387076, 1.000000000000000000, 0.9330127018922194093, 0.9330127018922194093 ) ) 
 REPRESENTATION_ITEM ( '' )  );
#17160=CARTESIAN_POINT ( 'NONE',  ( 4.458734124999998549, -12.97916666530107044, -2.574251347313721627 ) ) ;
#17169=ORIENTED_EDGE ( 'NONE', *, *, #10671, .T. ) ;
#17170=CARTESIAN_POINT ( 'NONE',  ( -3.152548672688508926E-16, -62.81249999863440792, -5.148502694627439702 ) ) ;
#17173=ORIENTED_EDGE ( 'NONE', *, *, #51051, .F. ) ;
#17175=CARTESIAN_POINT ( 'NONE',  ( -4.999999999999998224, 27.20833333606451276, 2.886751345948131764 ) ) ;
#17181=VECTOR ( 'NONE', #56786, 1000.000000000000000 ) ;
#17182=CARTESIAN_POINT ( 'NONE',  ( 9.457646018065525792E-16, 9.937500001365592084, 5.148502694627439702 ) ) ;
#17185=CARTESIAN_POINT ( 'NONE',  ( -2.500000000000000444, -24.04166666393548368, -4.330127018922193649 ) ) ;
#17187=ORIENTED_EDGE ( 'NONE', *, *, #19220, .T. ) ;
#17188=CARTESIAN_POINT ( 'NONE',  ( 9.457646018065525792E-16, -73.06249999863439371, 5.148502694627439702 ) ) ;
#17189=CARTESIAN_POINT ( 'NONE',  ( -1.339745962155613812, -50.08034179853029855, -5.000000000000000000 ) ) ;
#17190=CARTESIAN_POINT ( 'NONE',  ( -2.229367062499996610, 13.85416666803226171, 3.861377020970582219 ) ) ;
#17191=CARTESIAN_POINT ( 'NONE',  ( -2.499999999999996447, -41.83333333333333570, 4.330127018922195425 ) ) ;
#17192=CARTESIAN_POINT ( 'NONE',  ( 9.457646018065525792E-16, -57.31249999863440081, 5.148502694627439702 ) ) ;
#17193=CARTESIAN_POINT ( 'NONE',  ( -2.499999999999996447, -15.70833333060214443, 4.330127018922195425 ) ) ;
#17194=LINE ( 'NONE', #46783, #9105 ) ;
#17197=CARTESIAN_POINT ( 'NONE',  ( 9.457646018065525792E-16, -34.06249999863440792, 5.148502694627439702 ) ) ;
#17198=CARTESIAN_POINT ( 'NONE',  ( 4.458734124999999437, -19.06249999863440792, -5.460374474430324690E-16 ) ) ;
#17199=ORIENTED_EDGE ( 'NONE', *, *, #20005, .T. ) ;
#17201=CARTESIAN_POINT ( 'NONE',  ( -3.152548672688508926E-16, -109.5624999986344079, -5.148502694627439702 ) ) ;
#17203=ORIENTED_EDGE ( 'NONE', *, *, #44904, .T. ) ;
#17204=CARTESIAN_POINT ( 'NONE',  ( -3.152548672688508926E-16, -101.8124999986344079, -5.148502694627439702 ) ) ;
#17206=CARTESIAN_POINT ( 'NONE',  ( -4.458734124999999437, -26.31249999863440792, 0.000000000000000000 ) ) ;
#17207=CARTESIAN_POINT ( 'NONE',  ( 2.500000000000002220, -62.54166666393547303, 4.330127018922192761 ) ) ;
#17210=CARTESIAN_POINT ( 'NONE',  ( 4.458734124999999437, -29.81249999863440436, -5.460374474430324690E-16 ) ) ;
#17211=CARTESIAN_POINT ( 'NONE',  ( -2.229367062500000163, -67.72916666530106511, -3.861377020970580443 ) ) ;
#17212=DIRECTION ( 'NONE',  ( 0.000000000000000000, 0.000000000000000000, 1.000000000000000000 ) ) ;
#17216=CARTESIAN_POINT ( 'NONE',  ( 5.000000000000000000, -14.49999999999999822, -6.123233995736766282E-16 ) ) ;
#17219=CARTESIAN_POINT ( 'NONE',  ( 0.000000000000000000, -120.0000000000000000, 0.000000000000000000 ) ) ;
#17221=CARTESIAN_POINT ( 'NONE',  ( 2.499999999999998668, -84.20833333060214443, -4.330127018922193649 ) ) ;
#17222=CYLINDRICAL_SURFACE ( 'NONE', #48383, 5.000000000000000000 ) ;
#17225=PLANE ( 'NONE',  #28506 ) ;
#17227=EDGE_CURVE ( 'NONE', #9589, #9483, #45308, .T. ) ;
#17228=CARTESIAN_POINT ( 'NONE',  ( -4.330127018922101279, 45.00000000000000000, 7.500000000000002665 ) ) ;
#17234=EDGE_LOOP ( 'NONE', ( #9505, #55140, #50694, #43347 ) ) ;
#17235=CARTESIAN_POINT ( 'NONE',  ( 1.975475456537005874E-15, 17.25000000000000000, 5.000000000000000000 ) ) ;
#17236=ORIENTED_EDGE ( 'NONE', *, *, #16671, .F. ) ;
#17242=EDGE_LOOP ( 'NONE', ( #55441, #6970, #26261, #54435 ) ) ;
#17244=ORIENTED_EDGE ( 'NONE', *, *, #36996, .T. ) ;
#17247=CARTESIAN_POINT ( 'NONE',  ( 1.339745962155729053, -55.29465819873851729, -4.999999999999933387 ) ) ;
#17253=( BOUNDED_CURVE ( )  B_SPLINE_CURVE ( 2, ( #24887, #4831, #33169, #24450, #53093, #63385, #29580, #37989, #4512 ),
 .UNSPECIFIED., .F., .F. ) 
 B_SPLINE_CURVE_WITH_KNOTS ( ( 3, 2, 2, 2, 3 ),
 ( 0.7125000000000000222, 0.7130952380952381153, 0.7142857142857143016, 0.7154761904761904878, 0.7160714285714285809 ),
 .UNSPECIFIED. ) 
 CURVE ( )  GEOMETRIC_REPRESENTATION_ITEM ( )  RATIONAL_B_SPLINE_CURVE ( ( 0.9330127018922194093, 0.9330127018922194093, 1.000000000000000000, 0.8660254037844387076, 1.000000000000000000, 0.8660254037844387076, 1.000000000000000000, 0.9330127018922194093, 0.9330127018922194093 ) ) 
 REPRESENTATION_ITEM ( '' )  );
#17254=EDGE_CURVE ( 'NONE', #61583, #21697, #56247, .T. ) ;
#17255=CARTESIAN_POINT ( 'NONE',  ( -2.229367062499996610, -76.14583333196773651, 3.861377020970582219 ) ) ;
#17256=CARTESIAN_POINT ( 'NONE',  ( -4.458734124999999437, 22.60416666803225993, -2.574251347313719407 ) ) ;
#17264=CARTESIAN_POINT ( 'NONE',  ( 2.229367062499998831, -54.64583333196773651, -3.861377020970580887 ) ) ;
#17268=CARTESIAN_POINT ( 'NONE',  ( -4.999999999999999112, -108.9166666666666572, 2.886751345948131764 ) ) ;
#17270=CARTESIAN_POINT ( 'NONE',  ( 4.458734124999998549, -40.97916666530107932, -2.574251347313721627 ) ) ;
#17271=CARTESIAN_POINT ( 'NONE',  ( -2.500000000000000444, 2.958333336064520314, -4.330127018922193649 ) ) ;
#17276=CARTESIAN_POINT ( 'NONE',  ( -4.458734124999997661, -105.2291666653010651, 2.574251347313722516 ) ) ;
#17277=CARTESIAN_POINT ( 'NONE',  ( 2.229367062500001939, -8.229166665301073991, 3.861377020970579999 ) ) ;
#17280=CARTESIAN_POINT ( 'NONE',  ( 2.229367062500001939, -91.97916666530106511, 3.861377020970579999 ) ) ;
#17282=CARTESIAN_POINT ( 'NONE',  ( 4.458734125000001214, -88.14583333196773651, 2.574251347313718519 ) ) ;
#17285=CARTESIAN_POINT ( 'NONE',  ( -6.972266317189433020E-16, -94.12499999726880162, -5.000000000000000000 ) ) ;
#17287=CARTESIAN_POINT ( 'NONE',  ( 2.229367062499998831, -7.645833331967735624, -3.861377020970580887 ) ) ;
#17288=CARTESIAN_POINT ( 'NONE',  ( 4.458734125000001214, 17.85416666803225993, 2.574251347313718519 ) ) ;
#17289=CARTESIAN_POINT ( 'NONE',  ( 2.229367062500001939, -55.22916666530107221, 3.861377020970579999 ) ) ;
#17291=CARTESIAN_POINT ( 'NONE',  ( -6.972266317189433020E-16, -37.25000000000000000, -5.000000000000000000 ) ) ;
#17296=CARTESIAN_POINT ( 'NONE',  ( 2.500000000000002220, -76.66666666666665719, 4.330127018922192761 ) ) ;
#17297=CARTESIAN_POINT ( 'NONE',  ( -2.229367062500000163, -81.47916666530106511, -3.861377020970580443 ) ) ;
#17298=CARTESIAN_POINT ( 'NONE',  ( 4.458734125000001214, 22.85416666803225993, 2.574251347313718519 ) ) ;
#17305=CARTESIAN_POINT ( 'NONE',  ( -5.000000000000000000, -67.08333333333332860, -2.886751345948128211 ) ) ;
#17306=( BOUNDED_CURVE ( )  B_SPLINE_CURVE ( 2, ( #20576, #55312, #24750, #974, #20891, #30851, #5132, #59168, #49510 ),
 .UNSPECIFIED., .F., .F. ) 
 B_SPLINE_CURVE_WITH_KNOTS ( ( 3, 2, 2, 2, 3 ),
 ( 0.3196428571428571175, 0.3202380952380952106, 0.3214285714285714524, 0.3226190476190476386, 0.3232142857142857317 ),
 .UNSPECIFIED. ) 
 CURVE ( )  GEOMETRIC_REPRESENTATION_ITEM ( )  RATIONAL_B_SPLINE_CURVE ( ( 0.9330127018922194093, 0.9330127018922194093, 1.000000000000000000, 0.8660254037844387076, 1.000000000000000000, 0.8660254037844387076, 1.000000000000000000, 0.9330127018922194093, 0.9330127018922194093 ) ) 
 REPRESENTATION_ITEM ( '' )  );
#17309=VERTEX_POINT ( 'NONE', #20876 ) ;
#17311=EDGE_CURVE ( 'NONE', #33407, #50926, #5079, .T. ) ;
#17314=CARTESIAN_POINT ( 'NONE',  ( 1.975475456537005874E-15, -52.62499999726880873, 5.000000000000000000 ) ) ;
#17318=VECTOR ( 'NONE', #60683, 1000.000000000000000 ) ;
#17328=CARTESIAN_POINT ( 'NONE',  ( 4.458734125000001214, -51.14583333196772941, 2.574251347313718519 ) ) ;
#17336=FACE_OUTER_BOUND ( 'NONE', #17242, .T. ) ;
#17339=CARTESIAN_POINT ( 'NONE',  ( 4.458734125000001214, -100.1458333319677365, 2.574251347313718519 ) ) ;
#17346=CARTESIAN_POINT ( 'NONE',  ( -4.458734124999999437, -7.312499998634404363, 0.000000000000000000 ) ) ;
#17347=CARTESIAN_POINT ( 'NONE',  ( 4.458734124999998549, -96.97916666530105090, -2.574251347313721627 ) ) ;
#17349=CARTESIAN_POINT ( 'NONE',  ( -2.229367062499996610, -21.39583333196774007, 3.861377020970582219 ) ) ;
#17350=CARTESIAN_POINT ( 'NONE',  ( -6.972266317189433020E-16, -46.24999999999999289, -5.000000000000000000 ) ) ;
#17357=( BOUNDED_CURVE ( )  B_SPLINE_CURVE ( 2, ( #31403, #50403, #51041, #26918, #2174, #26595, #40422, #61018, #16944 ),
 .UNSPECIFIED., .F., .F. ) 
 B_SPLINE_CURVE_WITH_KNOTS ( ( 3, 2, 2, 2, 3 ),
 ( 0.1696428571428571508, 0.1702380952380952439, 0.1714285714285714302, 0.1726190476190476164, 0.1732142857142857095 ),
 .UNSPECIFIED. ) 
 CURVE ( )  GEOMETRIC_REPRESENTATION_ITEM ( )  RATIONAL_B_SPLINE_CURVE ( ( 0.9330127018922194093, 0.9330127018922194093, 1.000000000000000000, 0.8660254037844387076, 1.000000000000000000, 0.8660254037844387076, 1.000000000000000000, 0.9330127018922194093, 0.9330127018922194093 ) ) 
 REPRESENTATION_ITEM ( '' )  );
#17358=CARTESIAN_POINT ( 'NONE',  ( 2.229367062499998831, 11.10416666803225993, -3.861377020970580887 ) ) ;
#17360=DIRECTION ( 'NONE',  ( -0.000000000000000000, 1.000000000000000000, -0.000000000000000000 ) ) ;
#17361=CARTESIAN_POINT ( 'NONE',  ( 5.000000000000000000, -66.29166666393547303, -2.886751345948130876 ) ) ;
#17362=CARTESIAN_POINT ( 'NONE',  ( 5.000000000000000000, -92.41666666666665719, -2.886751345948129988 ) ) ;
#17363=CARTESIAN_POINT ( 'NONE',  ( -2.229367062499996610, -22.14583333196773651, 3.861377020970582219 ) ) ;
#17365=CARTESIAN_POINT ( 'NONE',  ( -4.458734124999998549, -70.47916666530107932, 2.574251347313722516 ) ) ;
#17369=ADVANCED_FACE ( 'NONE', ( #42606 ), #17849, .T. ) ;
#17371=CARTESIAN_POINT ( 'NONE',  ( 5.000000000000000888, -52.45833333060213732, 2.886751345948126879 ) ) ;
#17373=CARTESIAN_POINT ( 'NONE',  ( 2.229367062499998831, 6.354166668032262599, -3.861377020970580887 ) ) ;
#17378=CARTESIAN_POINT ( 'NONE',  ( 4.458734125000001214, -72.89583333196775072, 2.574251347313718519 ) ) ;
#17382=CARTESIAN_POINT ( 'NONE',  ( -5.000000000000000000, -1.083333333333331927, -2.886751345948128211 ) ) ;
#17385=CARTESIAN_POINT ( 'NONE',  ( 9.457646018065525792E-16, -65.06249999863440792, 5.148502694627439702 ) ) ;
#17386=CARTESIAN_POINT ( 'NONE',  ( 2.500000000000002220, -98.54166666393545881, 4.330127018922192761 ) ) ;
#17391=ADVANCED_FACE ( 'NONE', ( #32323 ), #13023, .T. ) ;
#17394=CARTESIAN_POINT ( 'NONE',  ( -4.999999999999999112, -47.91666666666667140, 2.886751345948131764 ) ) ;
#17395=EDGE_CURVE ( 'NONE', #19443, #24216, #7168, .T. ) ;
#17396=FACE_OUTER_BOUND ( 'NONE', #20907, .T. ) ;
#17397=VERTEX_POINT ( 'NONE', #62244 ) ;
#17400=EDGE_CURVE ( 'NONE', #30363, #28142, #51127, .T. ) ;
#17404=CARTESIAN_POINT ( 'NONE',  ( -4.999999999999998224, -30.79166666393548013, 2.886751345948131764 ) ) ;
#17410=ORIENTED_EDGE ( 'NONE', *, *, #7587, .T. ) ;
#17414=CARTESIAN_POINT ( 'NONE',  ( 4.458734124999998549, -33.97916666530107221, -2.574251347313721627 ) ) ;
#17424=CARTESIAN_POINT ( 'NONE',  ( -2.229367062500000163, -82.72916666530106511, -3.861377020970580443 ) ) ;
#17426=ORIENTED_EDGE ( 'NONE', *, *, #20404, .F. ) ;
#17427=CARTESIAN_POINT ( 'NONE',  ( -2.499999999999996447, -94.70833333060213022, 4.330127018922195425 ) ) ;
#17430=CARTESIAN_POINT ( 'NONE',  ( -3.152548672688508926E-16, -6.812499998634404363, -5.148502694627439702 ) ) ;
#17431=ORIENTED_EDGE ( 'NONE', *, *, #24057, .T. ) ;
#17434=CARTESIAN_POINT ( 'NONE',  ( -4.458734124999998549, -9.479166665301070438, 2.574251347313722516 ) ) ;
#17435=DIRECTION ( 'NONE',  ( 0.000000000000000000, 0.000000000000000000, 1.000000000000000000 ) ) ;
#17437=CARTESIAN_POINT ( 'NONE',  ( 1.339745962155612702, -64.29465819873851729, -5.000000000000000000 ) ) ;
#17439=CARTESIAN_POINT ( 'NONE',  ( -4.458734124999997661, 26.52083333469892779, 2.574251347313722516 ) ) ;
#17441=CARTESIAN_POINT ( 'NONE',  ( 2.229367062500001939, -85.97916666530107932, 3.861377020970579999 ) ) ;
#17442=CARTESIAN_POINT ( 'NONE',  ( -2.500000000000000444, -78.16666666666665719, -4.330127018922193649 ) ) ;
#17443=CARTESIAN_POINT ( 'NONE',  ( -4.458734124999999437, -7.395833331967734736, -2.574251347313719407 ) ) ;
#17444=CARTESIAN_POINT ( 'NONE',  ( -2.500000000000000444, 19.83333333333333570, -4.330127018922193649 ) ) ;
#17445=DIRECTION ( 'NONE',  ( -0.000000000000000000, 1.000000000000000000, -0.000000000000000000 ) ) ;
#17446=( BOUNDED_CURVE ( )  B_SPLINE_CURVE ( 2, ( #1360, #30272, #40564, #16129, #50860, #21597, #7120, #55052, #35120 ),
 .UNSPECIFIED., .F., .F. ) 
 B_SPLINE_CURVE_WITH_KNOTS ( ( 3, 2, 2, 2, 3 ),
 ( 0.005357142857142858060, 0.005952380952380952051, 0.007142857142857142634, 0.008333333333333333218, 0.008928571428571429811 ),
 .UNSPECIFIED. ) 
 CURVE ( )  GEOMETRIC_REPRESENTATION_ITEM ( )  RATIONAL_B_SPLINE_CURVE ( ( 0.9330127018922192983, 0.9330127018922194093, 1.000000000000000000, 0.8660254037844387076, 1.000000000000000000, 0.8660254037844387076, 1.000000000000000000, 0.9330127018922191873, 0.9330127018922192983 ) ) 
 REPRESENTATION_ITEM ( '' )  );
#17447=DIRECTION ( 'NONE',  ( -0.000000000000000000, 1.000000000000000000, -0.000000000000000000 ) ) ;
#17448=CARTESIAN_POINT ( 'NONE',  ( 1.060575238724906964E-15, -34.62499999726880873, 5.773502691896257311 ) ) ;
#17450=CARTESIAN_POINT ( 'NONE',  ( -4.458734124999999437, 25.68750000136559208, 0.000000000000000000 ) ) ;
#17451=CARTESIAN_POINT ( 'NONE',  ( -2.499999999999996447, -20.70833333060214798, 4.330127018922195425 ) ) ;
#17453=CARTESIAN_POINT ( 'NONE',  ( 9.457646018065525792E-16, -59.06249999863439371, 5.148502694627439702 ) ) ;
#17455=DIRECTION ( 'NONE',  ( -0.000000000000000000, 1.000000000000000000, -0.000000000000000000 ) ) ;
#17456=CARTESIAN_POINT ( 'NONE',  ( -2.499999999999996447, 15.16666666666666607, 4.330127018922195425 ) ) ;
#17460=CARTESIAN_POINT ( 'NONE',  ( -2.229367062500000163, -45.47916666530106511, -3.861377020970580443 ) ) ;
#17461=CARTESIAN_POINT ( 'NONE',  ( 5.000000000000000888, -79.45833333060214443, 2.886751345948126879 ) ) ;
#17464=( BOUNDED_CURVE ( )  B_SPLINE_CURVE ( 2, ( #27745, #18722, #38346, #3323, #41901, #62172, #61548, #17479, #18094 ),
 .UNSPECIFIED., .F., .F. ) 
 B_SPLINE_CURVE_WITH_KNOTS ( ( 3, 2, 2, 2, 3 ),
 ( 0.4982142857142857206, 0.4988095238095238138, 0.5000000000000000000, 0.5011904761904761862, 0.5017857142857142794 ),
 .UNSPECIFIED. ) 
 CURVE ( )  GEOMETRIC_REPRESENTATION_ITEM ( )  RATIONAL_B_SPLINE_CURVE ( ( 0.9330127018922194093, 0.9330127018922194093, 1.000000000000000000, 0.8660254037844387076, 1.000000000000000000, 0.8660254037844387076, 1.000000000000000000, 0.9330127018922194093, 0.9330127018922194093 ) ) 
 REPRESENTATION_ITEM ( '' )  );
#17465=CARTESIAN_POINT ( 'NONE',  ( -6.972266317189433020E-16, -36.25000000000000000, -5.000000000000000000 ) ) ;
#17466=CARTESIAN_POINT ( 'NONE',  ( -4.458734124999999437, -87.56249999863439371, 0.000000000000000000 ) ) ;
#17468=CARTESIAN_POINT ( 'NONE',  ( -3.535250795749689387E-16, -31.25000000000000000, -5.773502691896257311 ) ) ;
#17469=ORIENTED_EDGE ( 'NONE', *, *, #22773, .F. ) ;
#17470=ADVANCED_FACE ( 'NONE', ( #30016 ), #63494, .T. ) ;
#17473=CARTESIAN_POINT ( 'NONE',  ( 4.458734124999998549, -94.72916666530106511, -2.574251347313721627 ) ) ;
#17474=CARTESIAN_POINT ( 'NONE',  ( -3.152548672688508926E-16, 16.18750000136559564, -5.148502694627439702 ) ) ;
#17475=CARTESIAN_POINT ( 'NONE',  ( 5.000000000000000000, 17.70833333606451632, -2.886751345948129988 ) ) ;
#17476=CARTESIAN_POINT ( 'NONE',  ( -4.999999999999998224, -34.79166666393547303, 2.886751345948131764 ) ) ;
#17479=CARTESIAN_POINT ( 'NONE',  ( -1.339745962155613812, -40.20534180126147561, -5.000000000000000000 ) ) ;
#17480=CARTESIAN_POINT ( 'NONE',  ( -4.999999999999999112, -78.91666666666665719, 2.886751345948131764 ) ) ;
#17481=EDGE_CURVE ( 'NONE', #19195, #38618, #34512, .T. ) ;
#17482=CARTESIAN_POINT ( 'NONE',  ( 2.493747252781420335E-13, -43.12499999726882294, -5.000000000000000000 ) ) ;
#17483=FACE_OUTER_BOUND ( 'NONE', #53970, .T. ) ;
#17484=CARTESIAN_POINT ( 'NONE',  ( -5.000000000000000000, -25.95833333060214798, -2.886751345948128211 ) ) ;
#17489=CARTESIAN_POINT ( 'NONE',  ( -3.152548672688508926E-16, -20.81249999863440081, -5.148502694627439702 ) ) ;
#17498=CARTESIAN_POINT ( 'NONE',  ( 2.499999999999998668, -85.20833333060214443, -4.330127018922193649 ) ) ;
#17500=CARTESIAN_POINT ( 'NONE',  ( -2.229367062499996610, -62.39583333196774362, 3.861377020970582219 ) ) ;
#17502=CARTESIAN_POINT ( 'NONE',  ( -5.000000000000000000, -5.874999997268811391, 0.000000000000000000 ) ) ;
#17504=ORIENTED_EDGE ( 'NONE', *, *, #39698, .T. ) ;
#17505=AXIS2_PLACEMENT_3D ( 'NONE', #60329, #40042, #34575 ) ;
#17507=DIRECTION ( 'NONE',  ( 0.000000000000000000, 0.000000000000000000, 1.000000000000000000 ) ) ;
#17510=ORIENTED_EDGE ( 'NONE', *, *, #33833, .T. ) ;
#17512=CARTESIAN_POINT ( 'NONE',  ( 2.229367062500001939, 7.020833334698928674, 3.861377020970579999 ) ) ;
#17515=CARTESIAN_POINT ( 'NONE',  ( 5.000000000000000000, -77.50000000000000000, -6.123233995736766282E-16 ) ) ;
#17517=( BOUNDED_CURVE ( )  B_SPLINE_CURVE ( 2, ( #50262, #45438, #41232, #44792, #55733, #59933, #40607, #5891, #6845 ),
 .UNSPECIFIED., .F., .F. ) 
 B_SPLINE_CURVE_WITH_KNOTS ( ( 3, 2, 2, 2, 3 ),
 ( 0.04821428571428571647, 0.04880952380952380959, 0.05000000000000000278, 0.05119047619047618902, 0.05178571428571428908 ),
 .UNSPECIFIED. ) 
 CURVE ( )  GEOMETRIC_REPRESENTATION_ITEM ( )  RATIONAL_B_SPLINE_CURVE ( ( 0.9330127018922194093, 0.9330127018922197424, 1.000000000000000000, 0.8660254037844387076, 1.000000000000000000, 0.8660254037844387076, 1.000000000000000000, 0.9330127018922189652, 0.9330127018922194093 ) ) 
 REPRESENTATION_ITEM ( '' )  );
#17518=ORIENTED_EDGE ( 'NONE', *, *, #34267, .T. ) ;
#17519=CARTESIAN_POINT ( 'NONE',  ( 4.458734124999999437, -70.81249999863439371, -5.460374474430324690E-16 ) ) ;
#17520=CARTESIAN_POINT ( 'NONE',  ( -4.458734124999999437, 5.604166668032262599, -2.574251347313719407 ) ) ;
#17521=ADVANCED_FACE ( 'NONE', ( #14276 ), #48373, .T. ) ;
#17522=CARTESIAN_POINT ( 'NONE',  ( -2.500000000000000444, -42.16666666666667140, -4.330127018922193649 ) ) ;
#17523=CARTESIAN_POINT ( 'NONE',  ( 2.229367062499998831, -60.89583333196774362, -3.861377020970580887 ) ) ;
#17524=CARTESIAN_POINT ( 'NONE',  ( -3.535250795749689387E-16, -17.12499999726881583, -5.773502691896257311 ) ) ;
#17525=DIRECTION ( 'NONE',  ( 0.000000000000000000, 0.000000000000000000, 1.000000000000000000 ) ) ;
#17526=CARTESIAN_POINT ( 'NONE',  ( 1.975475456537005874E-15, -49.62499999726880873, 5.000000000000000000 ) ) ;
#17527=CARTESIAN_POINT ( 'NONE',  ( 1.339745962155615144, 19.41965820146970501, 4.999999999999999112 ) ) ;
#17529=CARTESIAN_POINT ( 'NONE',  ( -4.458734124999998549, -35.22916666530107221, 2.574251347313722516 ) ) ;
#17530=CARTESIAN_POINT ( 'NONE',  ( 4.458734125000000326, -24.14583333196774362, 2.574251347313718519 ) ) ;
#17532=CARTESIAN_POINT ( 'NONE',  ( -6.972266317189433020E-16, -36.25000000000000000, -5.000000000000000000 ) ) ;
#17533=CARTESIAN_POINT ( 'NONE',  ( 5.000000000000000888, 29.41666666666666785, 2.886751345948126879 ) ) ;
#17535=ORIENTED_EDGE ( 'NONE', *, *, #61829, .T. ) ;
#17536=CARTESIAN_POINT ( 'NONE',  ( -4.458734124999998549, -104.4791666653010651, 2.574251347313722516 ) ) ;
#17537=CARTESIAN_POINT ( 'NONE',  ( 4.458734125000001214, -33.89583333196773651, 2.574251347313718519 ) ) ;
#17538=CARTESIAN_POINT ( 'NONE',  ( -5.000000000000000000, -62.95833333060214443, -2.886751345948128211 ) ) ;
#17541=CARTESIAN_POINT ( 'NONE',  ( 4.458734124999999437, -26.81249999863440081, -5.460374474430324690E-16 ) ) ;
#17542=CARTESIAN_POINT ( 'NONE',  ( -2.229367062499996610, -69.39583333196773651, 3.861377020970582219 ) ) ;
#17545=CARTESIAN_POINT ( 'NONE',  ( 1.975475456537005874E-15, -32.74999999999999289, 5.000000000000000000 ) ) ;
#17547=CARTESIAN_POINT ( 'NONE',  ( 2.499999999999998668, -17.33333333333333215, -4.330127018922193649 ) ) ;
#17550=CARTESIAN_POINT ( 'NONE',  ( -6.972266317189433020E-16, -82.24999999999998579, -5.000000000000000000 ) ) ;
#17554=CARTESIAN_POINT ( 'NONE',  ( 6.158835246850667461E-14, -1.250000000000002442, -4.999999999999999112 ) ) ;
#17559=CARTESIAN_POINT ( 'NONE',  ( 5.000000000000000000, -14.49999999999999822, -6.123233995736766282E-16 ) ) ;
#17560=CARTESIAN_POINT ( 'NONE',  ( 1.339745962155612702, -87.16965819600731891, -5.000000000000000000 ) ) ;
#17563=CARTESIAN_POINT ( 'NONE',  ( -6.972266317189433020E-16, -30.12499999726880873, -5.000000000000000000 ) ) ;
#17564=VERTEX_POINT ( 'NONE', #58976 ) ;
#17565=DIRECTION ( 'NONE',  ( 0.000000000000000000, 0.000000000000000000, 1.000000000000000000 ) ) ;
#17569=VERTEX_POINT ( 'NONE', #43536 ) ;
#17572=CARTESIAN_POINT ( 'NONE',  ( 2.500000000000002220, -53.66666666666667140, 4.330127018922192761 ) ) ;
#17581=CARTESIAN_POINT ( 'NONE',  ( -4.458734124999999437, -82.39583333196773651, -2.574251347313719407 ) ) ;
#17582=CARTESIAN_POINT ( 'NONE',  ( -4.458734124999999437, 25.68750000136559208, 0.000000000000000000 ) ) ;
#17589=CARTESIAN_POINT ( 'NONE',  ( 0.000000000000000000, -120.0000000000000000, 5.000000000000000000 ) ) ;
#17590=CYLINDRICAL_SURFACE ( 'NONE', #8955, 5.000000000000000000 ) ;
#17591=CARTESIAN_POINT ( 'NONE',  ( 2.500000000000002220, -13.54166666393548013, 4.330127018922192761 ) ) ;
#17592=CARTESIAN_POINT ( 'NONE',  ( -4.458734124999999437, -55.39583333196773651, -2.574251347313719407 ) ) ;
#17595=CARTESIAN_POINT ( 'NONE',  ( 2.229367062499998831, 27.35416666803225993, -3.861377020970580887 ) ) ;
#17596=CARTESIAN_POINT ( 'NONE',  ( 2.499999999999998668, -104.3333333333333286, -4.330127018922193649 ) ) ;
#17598=CARTESIAN_POINT ( 'NONE',  ( -4.458734124999999437, -39.56249999863440081, 0.000000000000000000 ) ) ;
#17599=CARTESIAN_POINT ( 'NONE',  ( -2.499999999999996447, -0.7083333306021483144, 4.330127018922195425 ) ) ;
#17603=CARTESIAN_POINT ( 'NONE',  ( -4.458734124999999437, -100.3124999986344079, 0.000000000000000000 ) ) ;
#17604=CARTESIAN_POINT ( 'NONE',  ( 2.229367062500001939, -6.229166665301072214, 3.861377020970579999 ) ) ;
#17605=ORIENTED_EDGE ( 'NONE', *, *, #20483, .T. ) ;
#17606=CARTESIAN_POINT ( 'NONE',  ( 1.975475456537005874E-15, -85.62499999726880162, 5.000000000000000000 ) ) ;
#17607=CARTESIAN_POINT ( 'NONE',  ( 4.458734124999999437, -94.81249999863440792, -5.460374474430324690E-16 ) ) ;
#17609=CARTESIAN_POINT ( 'NONE',  ( -4.458734124999998549, -84.47916666530107932, 2.574251347313722516 ) ) ;
#17611=DIRECTION ( 'NONE',  ( -0.000000000000000000, 1.000000000000000000, -0.000000000000000000 ) ) ;
#17613=CARTESIAN_POINT ( 'NONE',  ( 4.458734124999998549, -12.72916666530106866, -2.574251347313721627 ) ) ;
#17614=CARTESIAN_POINT ( 'NONE',  ( -4.458734124999998549, 18.52083333469892779, 2.574251347313722516 ) ) ;
#17615=CARTESIAN_POINT ( 'NONE',  ( -4.458734124999997661, -53.47916666530107221, 2.574251347313722516 ) ) ;
#17623=CARTESIAN_POINT ( 'NONE',  ( 7.204675194429079505E-15, 26.87500000273118417, -5.000000000000000000 ) ) ;
#17624=CARTESIAN_POINT ( 'NONE',  ( 9.457646018065525792E-16, -79.06249999863440792, 5.148502694627439702 ) ) ;
#17625=CARTESIAN_POINT ( 'NONE',  ( 4.458734124999998549, 26.02083333469892779, -2.574251347313721627 ) ) ;
#17630=CARTESIAN_POINT ( 'NONE',  ( -3.535250795749689387E-16, -64.25000000000000000, -5.773502691896257311 ) ) ;
#17631=CARTESIAN_POINT ( 'NONE',  ( 4.648177544792955347E-16, 29.75000000000000355, -5.000000000000000000 ) ) ;
#17635=FACE_OUTER_BOUND ( 'NONE', #63392, .T. ) ;
#17638=CARTESIAN_POINT ( 'NONE',  ( -2.500000000000000444, 4.833333333333332149, -4.330127018922193649 ) ) ;
#17639=( BOUNDED_CURVE ( )  B_SPLINE_CURVE ( 2, ( #54868, #30411, #5993, #37165, #16585, #61929, #17848, #56471, #36205 ),
 .UNSPECIFIED., .F., .F. ) 
 B_SPLINE_CURVE_WITH_KNOTS ( ( 3, 2, 2, 2, 3 ),
 ( 0.4482142857142857317, 0.4488095238095238249, 0.4500000000000000111, 0.4511904761904761973, 0.4517857142857142905 ),
 .UNSPECIFIED. ) 
 CURVE ( )  GEOMETRIC_REPRESENTATION_ITEM ( )  RATIONAL_B_SPLINE_CURVE ( ( 0.9330127018922194093, 0.9330127018922194093, 1.000000000000000000, 0.8660254037844387076, 1.000000000000000000, 0.8660254037844387076, 1.000000000000000000, 0.9330127018922194093, 0.9330127018922194093 ) ) 
 REPRESENTATION_ITEM ( '' )  );
#17645=ORIENTED_EDGE ( 'NONE', *, *, #13796, .F. ) ;
#17649=CARTESIAN_POINT ( 'NONE',  ( -4.458734124999998549, -49.47916666530106511, 2.574251347313722516 ) ) ;
#17652=VERTEX_POINT ( 'NONE', #10082 ) ;
#17659=CARTESIAN_POINT ( 'NONE',  ( -2.229367062500000163, -98.72916666530105090, -3.861377020970580443 ) ) ;
#17666=CARTESIAN_POINT ( 'NONE',  ( -3.152548672688508926E-16, -5.562499998634402587, -5.148502694627439702 ) ) ;
#17667=CARTESIAN_POINT ( 'NONE',  ( -4.458734124999999437, -95.64583333196773651, -2.574251347313719407 ) ) ;
#17669=CARTESIAN_POINT ( 'NONE',  ( -4.458734124999998549, -20.47916666530107577, 2.574251347313722516 ) ) ;
#17676=CARTESIAN_POINT ( 'NONE',  ( 2.229367062499998831, 12.10416666803226171, -3.861377020970580887 ) ) ;
#17678=CARTESIAN_POINT ( 'NONE',  ( -5.000000000000000000, -52.95833333060214443, -2.886751345948128211 ) ) ;
#17679=CARTESIAN_POINT ( 'NONE',  ( 0.000000000000000000, -120.0000000000000000, 0.000000000000000000 ) ) ;
#17680=CARTESIAN_POINT ( 'NONE',  ( -5.000000000000000000, -89.00000000000000000, 0.000000000000000000 ) ) ;
#17681=CARTESIAN_POINT ( 'NONE',  ( -4.458734124999999437, -22.31249999863440436, 0.000000000000000000 ) ) ;
#17683=CARTESIAN_POINT ( 'NONE',  ( 9.457646018065525792E-16, -73.31249999863440792, 5.148502694627439702 ) ) ;
#17687=CARTESIAN_POINT ( 'NONE',  ( 4.458734124999999437, 2.187500001365593416, -5.460374474430324690E-16 ) ) ;
#17689=DIRECTION ( 'NONE',  ( -0.000000000000000000, 1.000000000000000000, -0.000000000000000000 ) ) ;
#17691=CARTESIAN_POINT ( 'NONE',  ( 9.457646018065525792E-16, -73.06249999863440792, 5.148502694627439702 ) ) ;
#17694=CARTESIAN_POINT ( 'NONE',  ( 1.060575238724906964E-15, -2.750000000000002220, 5.773502691896257311 ) ) ;
#17697=CARTESIAN_POINT ( 'NONE',  ( 2.229367062499998831, -62.64583333196774362, -3.861377020970580887 ) ) ;
#17698=CARTESIAN_POINT ( 'NONE',  ( -3.535250795749689387E-16, -98.12499999726881583, -5.773502691896257311 ) ) ;
#17700=ADVANCED_FACE ( 'NONE', ( #48679 ), #58029, .T. ) ;
#17701=CARTESIAN_POINT ( 'NONE',  ( -4.458734124999999437, -107.6458333319677223, -2.574251347313719407 ) ) ;
#17703=CARTESIAN_POINT ( 'NONE',  ( -2.500000000000000444, -48.16666666666666430, -4.330127018922193649 ) ) ;
#17705=FACE_OUTER_BOUND ( 'NONE', #23555, .T. ) ;
#17707=DIRECTION ( 'NONE',  ( -0.000000000000000000, 1.000000000000000000, -0.000000000000000000 ) ) ;
#17708=DIRECTION ( 'NONE',  ( -0.000000000000000000, 1.000000000000000000, -0.000000000000000000 ) ) ;
#17715=CARTESIAN_POINT ( 'NONE',  ( 1.339745962155612702, -100.1696581960073473, -5.000000000000000000 ) ) ;
#17717=ORIENTED_EDGE ( 'NONE', *, *, #63257, .F. ) ;
#17721=CARTESIAN_POINT ( 'NONE',  ( -4.458734124999999437, -34.64583333196773651, -2.574251347313719407 ) ) ;
#17730=CARTESIAN_POINT ( 'NONE',  ( -2.229367062499996610, -81.39583333196773651, 3.861377020970582219 ) ) ;
#17733=( BOUNDED_CURVE ( )  B_SPLINE_CURVE ( 2, ( #44829, #35197, #54495, #24904, #45153, #30682, #1119, #15248, #54159 ),
 .UNSPECIFIED., .F., .F. ) 
 B_SPLINE_CURVE_WITH_KNOTS ( ( 3, 2, 2, 2, 3 ),
 ( 0.7767857142857143016, 0.7773809523809523947, 0.7785714285714285809, 0.7797619047619047672, 0.7803571428571428603 ),
 .UNSPECIFIED. ) 
 CURVE ( )  GEOMETRIC_REPRESENTATION_ITEM ( )  RATIONAL_B_SPLINE_CURVE ( ( 0.9330127018922194093, 0.9330127018922194093, 1.000000000000000000, 0.8660254037844387076, 1.000000000000000000, 0.8660254037844387076, 1.000000000000000000, 0.9330127018922194093, 0.9330127018922194093 ) ) 
 REPRESENTATION_ITEM ( '' )  );
#17734=CYLINDRICAL_SURFACE ( 'NONE', #29088, 5.000000000000000000 ) ;
#17736=CARTESIAN_POINT ( 'NONE',  ( -4.458734124999997661, -37.22916666530107221, 2.574251347313722516 ) ) ;
#17737=CARTESIAN_POINT ( 'NONE',  ( 4.458734125000001214, -10.14583333196773829, 2.574251347313718519 ) ) ;
#17740=CARTESIAN_POINT ( 'NONE',  ( 6.123233995736766282E-16, -120.0000000000000000, -5.000000000000000000 ) ) ;
#17742=CARTESIAN_POINT ( 'NONE',  ( -4.458734124999998549, -5.479166665301072214, 2.574251347313722516 ) ) ;
#17744=CARTESIAN_POINT ( 'NONE',  ( -6.972266317189433020E-16, -85.12499999726880162, -5.000000000000000000 ) ) ;
#17748=CARTESIAN_POINT ( 'NONE',  ( -3.152548672688508926E-16, 26.18750000136560274, -5.148502694627439702 ) ) ;
#17750=CARTESIAN_POINT ( 'NONE',  ( 4.458734124999998549, -88.72916666530106511, -2.574251347313721627 ) ) ;
#17752=CARTESIAN_POINT ( 'NONE',  ( -2.229367062499996610, -11.14583333196773829, 3.861377020970582219 ) ) ;
#17756=CARTESIAN_POINT ( 'NONE',  ( -4.999999999999999112, -36.79166666393548013, 2.886751345948131764 ) ) ;
#17758=CARTESIAN_POINT ( 'NONE',  ( 4.458734124999998549, 23.27083333469892423, -2.574251347313721627 ) ) ;
#17760=CARTESIAN_POINT ( 'NONE',  ( -2.229367062499996610, -54.14583333196773651, 3.861377020970582219 ) ) ;
#17763=CARTESIAN_POINT ( 'NONE',  ( 5.000000000000000000, 17.58333333333333215, -2.886751345948129988 ) ) ;
#17765=CARTESIAN_POINT ( 'NONE',  ( 5.000000000000000000, -69.41666666666667140, -2.886751345948130876 ) ) ;
#17766=CARTESIAN_POINT ( 'NONE',  ( -4.458734124999999437, -49.31249999863440792, 0.000000000000000000 ) ) ;
#17767=CARTESIAN_POINT ( 'NONE',  ( 5.000000000000000000, -82.37499999726881583, -6.123233995736766282E-16 ) ) ;
#17770=CARTESIAN_POINT ( 'NONE',  ( 4.458734124999998549, -85.97916666530107932, -2.574251347313721627 ) ) ;
#17772=CARTESIAN_POINT ( 'NONE',  ( -2.500000000000000444, -34.16666666666666430, -4.330127018922193649 ) ) ;
#17773=CARTESIAN_POINT ( 'NONE',  ( -4.999999999999998224, 24.08333333333333215, 2.886751345948131764 ) ) ;
#17776=VERTEX_POINT ( 'NONE', #21019 ) ;
#17777=CARTESIAN_POINT ( 'NONE',  ( -4.458734124999999437, -97.39583333196773651, -2.574251347313719407 ) ) ;
#17778=CARTESIAN_POINT ( 'NONE',  ( 4.458734124999998549, 9.020833334698927786, -2.574251347313721627 ) ) ;
#17779=CARTESIAN_POINT ( 'NONE',  ( 2.500000000000002220, 17.45833333606451987, 4.330127018922192761 ) ) ;
#17780=CARTESIAN_POINT ( 'NONE',  ( -2.499999999999996447, -28.70833333060214798, 4.330127018922195425 ) ) ;
#17784=CARTESIAN_POINT ( 'NONE',  ( 5.000000000000000000, -78.41666666666667140, -2.886751345948129988 ) ) ;
#17785=CARTESIAN_POINT ( 'NONE',  ( 1.975475456537005874E-15, 20.24999999999999289, 5.000000000000000000 ) ) ;
#17787=CARTESIAN_POINT ( 'NONE',  ( 0.000000000000000000, -120.0000000000000000, 5.000000000000000000 ) ) ;
#17790=CARTESIAN_POINT ( 'NONE',  ( -2.499999999999996447, 14.16666666666666785, 4.330127018922195425 ) ) ;
#17791=CARTESIAN_POINT ( 'NONE',  ( 9.457646018065525792E-16, -18.31249999863440436, 5.148502694627439702 ) ) ;
#17792=CARTESIAN_POINT ( 'NONE',  ( 2.500000000000002220, -107.5416666639354730, 4.330127018922192761 ) ) ;
#17799=EDGE_CURVE ( 'NONE', #9375, #38618, #62587, .T. ) ;
#17800=ORIENTED_EDGE ( 'NONE', *, *, #1286, .F. ) ;
#17801=CYLINDRICAL_SURFACE ( 'NONE', #35363, 5.000000000000000000 ) ;
#17802=ORIENTED_EDGE ( 'NONE', *, *, #40450, .F. ) ;
#17803=CARTESIAN_POINT ( 'NONE',  ( -2.229367062500000163, -68.72916666530107932, -3.861377020970580443 ) ) ;
#17804=CARTESIAN_POINT ( 'NONE',  ( -6.972266317189433020E-16, -7.124999997268814056, -5.000000000000000000 ) ) ;
#17805=DIRECTION ( 'NONE',  ( -0.000000000000000000, 1.000000000000000000, -0.000000000000000000 ) ) ;
#17806=ORIENTED_EDGE ( 'NONE', *, *, #26651, .F. ) ;
#17812=CARTESIAN_POINT ( 'NONE',  ( -2.499999999999996447, 2.291666669397850686, 4.330127018922195425 ) ) ;
#17813=CARTESIAN_POINT ( 'NONE',  ( -4.458734124999999437, 10.68750000136559386, 0.000000000000000000 ) ) ;
#17814=ADVANCED_FACE ( 'NONE', ( #11037 ), #20381, .T. ) ;
#17817=CARTESIAN_POINT ( 'NONE',  ( 1.975475456537005874E-15, -78.62499999726881583, 5.000000000000000000 ) ) ;
#17818=FACE_OUTER_BOUND ( 'NONE', #34033, .T. ) ;
#17820=EDGE_CURVE ( 'NONE', #34481, #14927, #35179, .T. ) ;
#17821=CARTESIAN_POINT ( 'NONE',  ( 4.458734124999999437, -68.81249999863439371, -5.460374474430324690E-16 ) ) ;
#17823=CARTESIAN_POINT ( 'NONE',  ( 4.458734125000001214, 6.104166668032262599, 2.574251347313718519 ) ) ;
#17826=CARTESIAN_POINT ( 'NONE',  ( -3.152548672688508926E-16, -61.81249999863440081, -5.148502694627439702 ) ) ;
#17827=CARTESIAN_POINT ( 'NONE',  ( 5.000000000000000888, -21.45833333060215153, 2.886751345948126879 ) ) ;
#17831=CARTESIAN_POINT ( 'NONE',  ( 6.123233995736766282E-16, -120.0000000000000000, -5.000000000000000000 ) ) ;
#17832=CARTESIAN_POINT ( 'NONE',  ( 9.457646018065525792E-16, -43.06249999863440081, 5.148502694627439702 ) ) ;
#17833=CARTESIAN_POINT ( 'NONE',  ( -4.458734124999999437, -19.56249999863440081, 0.000000000000000000 ) ) ;
#17836=CARTESIAN_POINT ( 'NONE',  ( -2.229367062499996610, -108.1458333319677365, 3.861377020970582219 ) ) ;
#17839=CARTESIAN_POINT ( 'NONE',  ( -4.458734124999998549, -109.4791666653010651, 2.574251347313722516 ) ) ;
#17840=CARTESIAN_POINT ( 'NONE',  ( -4.458734124999998549, -34.22916666530107221, 2.574251347313722516 ) ) ;
#17841=CARTESIAN_POINT ( 'NONE',  ( 1.060575238724906964E-15, -66.62499999726881583, 5.773502691896257311 ) ) ;
#17844=CARTESIAN_POINT ( 'NONE',  ( 2.229367062500001939, -27.97916666530107221, 3.861377020970579999 ) ) ;
#17845=CARTESIAN_POINT ( 'NONE',  ( -4.458734124999999437, -70.64583333196773651, -2.574251347313719407 ) ) ;
#17848=CARTESIAN_POINT ( 'NONE',  ( -2.500000000000000444, -33.16666666666666430, -4.330127018922193649 ) ) ;
#17849=CYLINDRICAL_SURFACE ( 'NONE', #25621, 5.000000000000000000 ) ;
#17850=CARTESIAN_POINT ( 'NONE',  ( 5.000000000000000888, -14.58333333333333037, 2.886751345948126879 ) ) ;
#17853=CARTESIAN_POINT ( 'NONE',  ( 6.123233995736766282E-16, -120.0000000000000000, -5.000000000000000000 ) ) ;
#17855=CARTESIAN_POINT ( 'NONE',  ( 5.000000000000000000, -84.29166666393547303, -2.886751345948130876 ) ) ;
#17858=CARTESIAN_POINT ( 'NONE',  ( 0.000000000000000000, -114.9999999999999858, 0.000000000000000000 ) ) ;
#17861=CARTESIAN_POINT ( 'NONE',  ( -6.972266317189433020E-16, -14.24999999999999822, -5.000000000000000000 ) ) ;
#17864=ORIENTED_EDGE ( 'NONE', *, *, #26805, .T. ) ;
#17882=DIRECTION ( 'NONE',  ( -0.000000000000000000, 1.000000000000000000, -0.000000000000000000 ) ) ;
#17883=ORIENTED_EDGE ( 'NONE', *, *, #19663, .F. ) ;
#17884=CARTESIAN_POINT ( 'NONE',  ( -4.458734124999999437, -84.39583333196773651, -2.574251347313719407 ) ) ;
#17885=CARTESIAN_POINT ( 'NONE',  ( 4.458734124999999437, 25.18750000136559208, -5.460374474430324690E-16 ) ) ;
#17886=CARTESIAN_POINT ( 'NONE',  ( 2.500000000000002220, -12.54166666393548013, 4.330127018922192761 ) ) ;
#17888=CARTESIAN_POINT ( 'NONE',  ( 1.339745962155612702, 14.70534180126147916, -5.000000000000000000 ) ) ;
#17894=CARTESIAN_POINT ( 'NONE',  ( 4.458734125000000326, -52.89583333196772941, 2.574251347313718519 ) ) ;
#17895=CARTESIAN_POINT ( 'NONE',  ( -4.458734124999999437, 20.68750000136559208, 0.000000000000000000 ) ) ;
#17896=CARTESIAN_POINT ( 'NONE',  ( 2.499999999999998668, -106.3333333333333286, -4.330127018922193649 ) ) ;
#17898=CARTESIAN_POINT ( 'NONE',  ( 9.457646018065525792E-16, -42.31249999863440081, 5.148502694627439702 ) ) ;
#17899=CARTESIAN_POINT ( 'NONE',  ( -3.535250795749689387E-16, -4.124999997268816720, -5.773502691896257311 ) ) ;
#17901=CARTESIAN_POINT ( 'NONE',  ( -6.972266317189433020E-16, -70.12499999726880162, -5.000000000000000000 ) ) ;
#17903=CARTESIAN_POINT ( 'NONE',  ( -3.152548672688508926E-16, -101.5624999986343937, -5.148502694627439702 ) ) ;
#17905=CARTESIAN_POINT ( 'NONE',  ( -2.229367062499996610, -5.395833331967740953, 3.861377020970582219 ) ) ;
#17907=FACE_OUTER_BOUND ( 'NONE', #33974, .T. ) ;
#17908=CARTESIAN_POINT ( 'NONE',  ( 9.457646018065525792E-16, -92.06249999863439371, 5.148502694627439702 ) ) ;
#17910=CARTESIAN_POINT ( 'NONE',  ( -4.458734124999999437, -90.64583333196773651, -2.574251347313719407 ) ) ;
#17913=AXIS2_PLACEMENT_3D ( 'NONE', #44428, #388, #28996 ) ;
#17915=CARTESIAN_POINT ( 'NONE',  ( -4.458734124999999437, -10.39583333196773474, -2.574251347313719407 ) ) ;
#17916=CARTESIAN_POINT ( 'NONE',  ( -4.458734124999999437, 14.35416666803226171, -2.574251347313719407 ) ) ;
#17917=CARTESIAN_POINT ( 'NONE',  ( -3.152548672688508926E-16, -55.81249999863440081, -5.148502694627439702 ) ) ;
#17918=DIRECTION ( 'NONE',  ( 0.000000000000000000, 0.000000000000000000, 1.000000000000000000 ) ) ;
#17919=CARTESIAN_POINT ( 'NONE',  ( -6.972266317189433020E-16, 13.87500000273118594, -5.000000000000000000 ) ) ;
#17921=ORIENTED_EDGE ( 'NONE', *, *, #56601, .F. ) ;
#17924=CARTESIAN_POINT ( 'NONE',  ( 1.339745962155615144, -68.70534180126148271, 4.999999999999999112 ) ) ;
#17925=CARTESIAN_POINT ( 'NONE',  ( -4.458734124999998549, -80.22916666530106511, 2.574251347313722516 ) ) ;
#17926=CARTESIAN_POINT ( 'NONE',  ( 4.458734124999999437, 21.93750000136559208, -5.460374474430324690E-16 ) ) ;
#17930=CARTESIAN_POINT ( 'NONE',  ( 2.500000000000002220, -67.66666666666667140, 4.330127018922192761 ) ) ;
#17931=CYLINDRICAL_SURFACE ( 'NONE', #26450, 5.000000000000000000 ) ;
#17935=CARTESIAN_POINT ( 'NONE',  ( -2.499999999999996447, -79.70833333060213022, 4.330127018922195425 ) ) ;
#17948=EDGE_CURVE ( 'NONE', #56025, #15620, #57582, .T. ) ;
#17949=CARTESIAN_POINT ( 'NONE',  ( -3.152548672688508926E-16, -50.81249999863440792, -5.148502694627439702 ) ) ;
#17959=CARTESIAN_POINT ( 'NONE',  ( 9.457646018065525792E-16, -100.3124999986344079, 5.148502694627439702 ) ) ;
#17964=CARTESIAN_POINT ( 'NONE',  ( -2.229367062500000163, -5.479166665301072214, -3.861377020970580443 ) ) ;
#17965=CARTESIAN_POINT ( 'NONE',  ( 4.458734124999999437, -96.06249999863440792, -5.460374474430324690E-16 ) ) ;
#17967=CARTESIAN_POINT ( 'NONE',  ( -2.229367062499996610, -28.39583333196774007, 3.861377020970582219 ) ) ;
#17968=CARTESIAN_POINT ( 'NONE',  ( -5.000000000000000000, -67.00000000000000000, 0.000000000000000000 ) ) ;
#17971=CARTESIAN_POINT ( 'NONE',  ( 1.975475456537005874E-15, -90.74999999999998579, 5.000000000000000000 ) ) ;
#17972=CARTESIAN_POINT ( 'NONE',  ( 1.339745962155615144, -88.58034179853028434, 4.999999999999999112 ) ) ;
#17974=CARTESIAN_POINT ( 'NONE',  ( -4.458734124999999437, 9.437500001365593860, 0.000000000000000000 ) ) ;
#17975=VERTEX_POINT ( 'NONE', #61215 ) ;
#17976=CARTESIAN_POINT ( 'NONE',  ( 1.975475456537005874E-15, -82.62499999726878741, 5.000000000000000000 ) ) ;
#17977=DIRECTION ( 'NONE',  ( 0.000000000000000000, 0.000000000000000000, 1.000000000000000000 ) ) ;
#17978=CARTESIAN_POINT ( 'NONE',  ( -4.999999999999999112, -88.91666666666667140, 2.886751345948131764 ) ) ;
#17979=CARTESIAN_POINT ( 'NONE',  ( 4.458734124999998549, -24.72916666530106866, -2.574251347313721627 ) ) ;
#17981=CARTESIAN_POINT ( 'NONE',  ( 4.458734124999998549, -71.97916666530107932, -2.574251347313721627 ) ) ;
#17982=FACE_OUTER_BOUND ( 'NONE', #40241, .T. ) ;
#17984=( BOUNDED_CURVE ( )  B_SPLINE_CURVE ( 2, ( #14650, #19799, #34268, #38465, #9820, #53894, #33652, #9513, #14973 ),
 .UNSPECIFIED., .F., .F. ) 
 B_SPLINE_CURVE_WITH_KNOTS ( ( 3, 2, 2, 2, 3 ),
 ( 0.2517857142857142794, 0.2523809523809523725, 0.2535714285714285587, 0.2547619047619047450, 0.2553571428571428381 ),
 .UNSPECIFIED. ) 
 CURVE ( )  GEOMETRIC_REPRESENTATION_ITEM ( )  RATIONAL_B_SPLINE_CURVE ( ( 0.9330127018922194093, 0.9330127018922194093, 1.000000000000000000, 0.8660254037844387076, 1.000000000000000000, 0.8660254037844387076, 1.000000000000000000, 0.9330127018922194093, 0.9330127018922194093 ) ) 
 REPRESENTATION_ITEM ( '' )  );
#17986=CARTESIAN_POINT ( 'NONE',  ( 4.458734125000000326, 2.104166668032262599, 2.574251347313718519 ) ) ;
#17987=CYLINDRICAL_SURFACE ( 'NONE', #20158, 5.000000000000000000 ) ;
#17988=CARTESIAN_POINT ( 'NONE',  ( 1.975475456537005874E-15, 20.37500000273118417, 5.000000000000000000 ) ) ;
#17990=CARTESIAN_POINT ( 'NONE',  ( -2.229367062500000163, -74.47916666530106511, -3.861377020970580443 ) ) ;
#17992=CARTESIAN_POINT ( 'NONE',  ( 2.500000000000002220, -7.666666666666668739, 4.330127018922192761 ) ) ;
#17994=CARTESIAN_POINT ( 'NONE',  ( 1.975475456537005874E-15, -104.6249999972688016, 5.000000000000000000 ) ) ;
#17995=CARTESIAN_POINT ( 'NONE',  ( -4.458734124999999437, -63.31249999863440792, 0.000000000000000000 ) ) ;
#17996=CARTESIAN_POINT ( 'NONE',  ( -5.000000000000000000, -100.9583333306021444, -2.886751345948128211 ) ) ;
#18000=CARTESIAN_POINT ( 'NONE',  ( 5.000000000000000888, -41.58333333333333570, 2.886751345948126879 ) ) ;
#18003=CARTESIAN_POINT ( 'NONE',  ( 4.458734124999998549, -107.9791666653010651, -2.574251347313721627 ) ) ;
#18005=CARTESIAN_POINT ( 'NONE',  ( -5.000000000000000000, -49.08333333333332860, -2.886751345948128211 ) ) ;
#18009=CARTESIAN_POINT ( 'NONE',  ( 4.458734124999999437, -109.8124999986343937, -5.460374474430324690E-16 ) ) ;
#18010=CARTESIAN_POINT ( 'NONE',  ( -5.000000000000000000, -99.95833333060213022, -2.886751345948128211 ) ) ;
#18026=CARTESIAN_POINT ( 'NONE',  ( -4.458734124999998549, -36.47916666530107221, 2.574251347313722516 ) ) ;
#18027=CARTESIAN_POINT ( 'NONE',  ( -2.500000000000000444, -87.16666666666667140, -4.330127018922193649 ) ) ;
#18030=DIRECTION ( 'NONE',  ( -0.000000000000000000, 1.000000000000000000, -0.000000000000000000 ) ) ;
#18033=ADVANCED_FACE ( 'NONE', ( #57266 ), #13184, .T. ) ;
#18036=CARTESIAN_POINT ( 'NONE',  ( 2.229367062500001939, -86.22916666530107932, 3.861377020970579999 ) ) ;
#18044=CARTESIAN_POINT ( 'NONE',  ( 2.500000000000002220, 17.33333333333333215, 4.330127018922192761 ) ) ;
#18045=EDGE_CURVE ( 'NONE', #29318, #60194, #12034, .T. ) ;
#18046=CARTESIAN_POINT ( 'NONE',  ( -4.458734124999999437, -12.56249999863440259, 0.000000000000000000 ) ) ;
#18051=( BOUNDED_CURVE ( )  B_SPLINE_CURVE ( 2, ( #57248, #62699, #53028, #43371, #56926, #3838, #27640, #28893, #38247 ),
 .UNSPECIFIED., .F., .F. ) 
 B_SPLINE_CURVE_WITH_KNOTS ( ( 3, 2, 2, 2, 3 ),
 ( 0.7553571428571428381, 0.7559523809523809312, 0.7571428571428571175, 0.7583333333333333037, 0.7589285714285713969 ),
 .UNSPECIFIED. ) 
 CURVE ( )  GEOMETRIC_REPRESENTATION_ITEM ( )  RATIONAL_B_SPLINE_CURVE ( ( 0.9330127018922194093, 0.9330127018922194093, 1.000000000000000000, 0.8660254037844387076, 1.000000000000000000, 0.8660254037844387076, 1.000000000000000000, 0.9330127018922194093, 0.9330127018922194093 ) ) 
 REPRESENTATION_ITEM ( '' )  );
#18052=CARTESIAN_POINT ( 'NONE',  ( -4.458734124999999437, 28.43750000136559208, 0.000000000000000000 ) ) ;
#18054=CARTESIAN_POINT ( 'NONE',  ( 4.458734124999999437, -93.81249999863440792, -5.460374474430324690E-16 ) ) ;
#18055=CARTESIAN_POINT ( 'NONE',  ( -2.500000000000000444, -68.16666666666667140, -4.330127018922193649 ) ) ;
#18056=CARTESIAN_POINT ( 'NONE',  ( -2.500000000000000444, -70.04166666393547303, -4.330127018922193649 ) ) ;
#18057=CARTESIAN_POINT ( 'NONE',  ( 4.458734124999998549, -8.729166665301073991, -2.574251347313721627 ) ) ;
#18060=CARTESIAN_POINT ( 'NONE',  ( -4.999999999999998224, 15.08333333333333215, 2.886751345948131764 ) ) ;
#18061=CARTESIAN_POINT ( 'NONE',  ( -5.000000000000000000, -35.87499999726881583, 0.000000000000000000 ) ) ;
#18062=FACE_OUTER_BOUND ( 'NONE', #47597, .T. ) ;
#18063=CARTESIAN_POINT ( 'NONE',  ( -4.458734124999999437, 18.68750000136559564, 0.000000000000000000 ) ) ;
#18064=CARTESIAN_POINT ( 'NONE',  ( -1.339745962155613812, -4.205341801261476498, -5.000000000000000000 ) ) ;
#18066=CARTESIAN_POINT ( 'NONE',  ( -3.152548672688508926E-16, -56.56249999863439371, -5.148502694627439702 ) ) ;
#18069=CARTESIAN_POINT ( 'NONE',  ( 5.000000000000000000, 11.58333333333333570, -2.886751345948129988 ) ) ;
#18073=CARTESIAN_POINT ( 'NONE',  ( 4.458734124999999437, -48.81249999863440792, -5.460374474430324690E-16 ) ) ;
#18074=CARTESIAN_POINT ( 'NONE',  ( -4.999999999999999112, -85.79166666393547303, 2.886751345948131764 ) ) ;
#18075=EDGE_CURVE ( 'NONE', #55067, #60295, #586, .T. ) ;
#18078=CARTESIAN_POINT ( 'NONE',  ( 1.339745962155557191, -36.70534180126148271, 5.000000000000032863 ) ) ;
#18079=EDGE_CURVE ( 'NONE', #2056, #55022, #38262, .T. ) ;
#18080=CARTESIAN_POINT ( 'NONE',  ( -4.458734124999997661, -89.47916666530105090, 2.574251347313722516 ) ) ;
#18082=CARTESIAN_POINT ( 'NONE',  ( 5.000000000000000888, -30.58333333333332860, 2.886751345948126879 ) ) ;
#18087=CARTESIAN_POINT ( 'NONE',  ( 2.229367062499998831, -98.64583333196773651, -3.861377020970580887 ) ) ;
#18088=CARTESIAN_POINT ( 'NONE',  ( 4.458734124999998549, 10.02083333469892779, -2.574251347313721627 ) ) ;
#18089=CARTESIAN_POINT ( 'NONE',  ( -5.000000000000000000, 10.12500000273118594, 0.000000000000000000 ) ) ;
#18092=AXIS2_PLACEMENT_3D ( 'NONE', #8300, #47523, #41739 ) ;
#18094=CARTESIAN_POINT ( 'NONE',  ( -6.972266317189433020E-16, -40.24999999999999289, -5.000000000000000000 ) ) ;
#18095=CARTESIAN_POINT ( 'NONE',  ( -3.535250795749689387E-16, -81.25000000000001421, -5.773502691896257311 ) ) ;
#18097=CARTESIAN_POINT ( 'NONE',  ( 0.000000000000000000, -120.0000000000000000, 0.000000000000000000 ) ) ;
#18099=ADVANCED_FACE ( 'NONE', ( #53047 ), #28597, .T. ) ;
#18100=CARTESIAN_POINT ( 'NONE',  ( 1.339745962155615144, -109.7053418012614685, 4.999999999999999112 ) ) ;
#18103=CARTESIAN_POINT ( 'NONE',  ( 5.000000000000000888, 6.541666669397851130, 2.886751345948126879 ) ) ;
#18104=CARTESIAN_POINT ( 'NONE',  ( 4.458734125000001214, -19.14583333196774007, 2.574251347313718519 ) ) ;
#18105=CARTESIAN_POINT ( 'NONE',  ( -5.000000000000000000, -57.99999999999999289, 0.000000000000000000 ) ) ;
#18107=( BOUNDED_CURVE ( )  B_SPLINE_CURVE ( 2, ( #8420, #51845, #47642, #23202, #31909, #42815, #62457, #18377, #22904 ),
 .UNSPECIFIED., .F., .F. ) 
 B_SPLINE_CURVE_WITH_KNOTS ( ( 3, 2, 2, 2, 3 ),
 ( 0.4339285714285714413, 0.4345238095238095344, 0.4357142857142857206, 0.4369047619047619069, 0.4375000000000000000 ),
 .UNSPECIFIED. ) 
 CURVE ( )  GEOMETRIC_REPRESENTATION_ITEM ( )  RATIONAL_B_SPLINE_CURVE ( ( 0.9330127018922194093, 0.9330127018922194093, 1.000000000000000000, 0.8660254037844387076, 1.000000000000000000, 0.8660254037844387076, 1.000000000000000000, 0.9330127018922194093, 0.9330127018922194093 ) ) 
 REPRESENTATION_ITEM ( '' )  );
#18116=CARTESIAN_POINT ( 'NONE',  ( 4.458734125000001214, -67.14583333196773651, 2.574251347313718519 ) ) ;
#18117=CARTESIAN_POINT ( 'NONE',  ( 2.500000000000002220, -7.541666663935481907, 4.330127018922192761 ) ) ;
#18119=ORIENTED_EDGE ( 'NONE', *, *, #49952, .T. ) ;
#18123=ORIENTED_EDGE ( 'NONE', *, *, #10952, .T. ) ;
#18124=DIRECTION ( 'NONE',  ( 0.000000000000000000, 0.000000000000000000, 1.000000000000000000 ) ) ;
#18125=CARTESIAN_POINT ( 'NONE',  ( -4.458734124999998549, 10.77083333469892956, 2.574251347313722516 ) ) ;
#18130=AXIS2_PLACEMENT_3D ( 'NONE', #13514, #53681, #63664 ) ;
#18131=VERTEX_POINT ( 'NONE', #18940 ) ;
#18132=CARTESIAN_POINT ( 'NONE',  ( 4.458734124999998549, -75.72916666530106511, -2.574251347313721627 ) ) ;
#18134=CARTESIAN_POINT ( 'NONE',  ( -2.229367062500000163, 9.520833334698927786, -3.861377020970580443 ) ) ;
#18135=VECTOR ( 'NONE', #15419, 1000.000000000000000 ) ;
#18137=CARTESIAN_POINT ( 'NONE',  ( -2.229367062499996610, -62.39583333196774362, 3.861377020970582219 ) ) ;
#18138=CARTESIAN_POINT ( 'NONE',  ( 5.000000000000000888, -22.45833333060214088, 2.886751345948126879 ) ) ;
#18140=DIRECTION ( 'NONE',  ( -0.000000000000000000, 1.000000000000000000, -0.000000000000000000 ) ) ;
#18141=CARTESIAN_POINT ( 'NONE',  ( 2.500000000000002220, 19.45833333606451632, 4.330127018922192761 ) ) ;
#18142=LINE ( 'NONE', #17831, #33690 ) ;
#18144=CARTESIAN_POINT ( 'NONE',  ( -4.458734124999999437, -38.31249999863439371, 0.000000000000000000 ) ) ;
#18145=CARTESIAN_POINT ( 'NONE',  ( 4.458734125000000326, -25.14583333196774007, 2.574251347313718519 ) ) ;
#18147=CARTESIAN_POINT ( 'NONE',  ( -5.000000000000000000, 29.91666666666666430, -2.886751345948128211 ) ) ;
#18149=ORIENTED_EDGE ( 'NONE', *, *, #27611, .F. ) ;
#18150=CARTESIAN_POINT ( 'NONE',  ( -2.229367062500000163, -106.7291666653010651, -3.861377020970580443 ) ) ;
#18151=CARTESIAN_POINT ( 'NONE',  ( -2.229367062500000163, -29.47916666530107221, -3.861377020970580443 ) ) ;
#18152=CARTESIAN_POINT ( 'NONE',  ( -4.999999999999999112, -69.79166666393547303, 2.886751345948131764 ) ) ;
#18156=EDGE_CURVE ( 'NONE', #45293, #25630, #11649, .T. ) ;
#18157=CARTESIAN_POINT ( 'NONE',  ( -4.458734124999999437, -31.31249999863440436, 0.000000000000000000 ) ) ;
#18158=CARTESIAN_POINT ( 'NONE',  ( 4.458734124999999437, -69.06249999863439371, -5.460374474430324690E-16 ) ) ;
#18161=EDGE_CURVE ( 'NONE', #20917, #57302, #11205, .T. ) ;
#18162=CARTESIAN_POINT ( 'NONE',  ( 1.975475456537005874E-15, -106.7499999999999858, 5.000000000000000000 ) ) ;
#18164=CARTESIAN_POINT ( 'NONE',  ( 5.000000000000000000, -18.41666666666666430, -2.886751345948129988 ) ) ;
#18167=CARTESIAN_POINT ( 'NONE',  ( 1.975475456537005874E-15, -57.74999999999999289, 5.000000000000000000 ) ) ;
#18169=CARTESIAN_POINT ( 'NONE',  ( 2.500000000000002220, 25.45833333606451987, 4.330127018922192761 ) ) ;
#18170=DIRECTION ( 'NONE',  ( -0.000000000000000000, 1.000000000000000000, -0.000000000000000000 ) ) ;
#18172=EDGE_CURVE ( 'NONE', #61583, #17564, #13720, .T. ) ;
#18176=CARTESIAN_POINT ( 'NONE',  ( 2.500000000000002220, -14.66666666666666785, 4.330127018922192761 ) ) ;
#18182=VECTOR ( 'NONE', #50911, 1000.000000000000000 ) ;
#18185=EDGE_CURVE ( 'NONE', #62764, #19443, #60110, .T. ) ;
#18189=VECTOR ( 'NONE', #53189, 1000.000000000000000 ) ;
#18192=ORIENTED_EDGE ( 'NONE', *, *, #11795, .T. ) ;
#18195=CARTESIAN_POINT ( 'NONE',  ( 6.123233995736766282E-16, -120.0000000000000000, -5.000000000000000000 ) ) ;
#18198=CYLINDRICAL_SURFACE ( 'NONE', #14914, 5.000000000000000000 ) ;
#18202=CARTESIAN_POINT ( 'NONE',  ( 2.229367062500001939, -81.97916666530106511, 3.861377020970579999 ) ) ;
#18203=CARTESIAN_POINT ( 'NONE',  ( -4.458734124999999437, 23.60416666803225993, -2.574251347313719407 ) ) ;
#18206=CARTESIAN_POINT ( 'NONE',  ( 4.648177544792955347E-16, 28.87500000273118417, -5.000000000000000000 ) ) ;
#18211=CARTESIAN_POINT ( 'NONE',  ( -5.000000000000000000, -83.08333333333332860, -2.886751345948128211 ) ) ;
#18213=CARTESIAN_POINT ( 'NONE',  ( -4.458734124999997661, -56.22916666530107221, 2.574251347313722516 ) ) ;
#18215=CARTESIAN_POINT ( 'NONE',  ( -4.458734124999999437, 21.60416666803225993, -2.574251347313719407 ) ) ;
#18217=CARTESIAN_POINT ( 'NONE',  ( -3.152548672688508926E-16, -41.81249999863440081, -5.148502694627439702 ) ) ;
#18218=CARTESIAN_POINT ( 'NONE',  ( 5.000000000000000000, -5.374999997268811391, -6.123233995736766282E-16 ) ) ;
#18222=CARTESIAN_POINT ( 'NONE',  ( 4.458734124999999437, -103.8124999986344079, -5.460374474430324690E-16 ) ) ;
#18223=CARTESIAN_POINT ( 'NONE',  ( -4.458734124999997661, -7.479166665301073991, 2.574251347313722516 ) ) ;
#18224=VERTEX_POINT ( 'NONE', #5108 ) ;
#18226=CARTESIAN_POINT ( 'NONE',  ( 4.458734125000001214, -93.89583333196772230, 2.574251347313718519 ) ) ;
#18228=CARTESIAN_POINT ( 'NONE',  ( -4.458734124999998549, -90.47916666530106511, 2.574251347313722516 ) ) ;
#18232=VECTOR ( 'NONE', #15210, 1000.000000000000000 ) ;
#18233=CARTESIAN_POINT ( 'NONE',  ( -3.152548672688508926E-16, -13.56249999863440259, -5.148502694627439702 ) ) ;
#18234=CARTESIAN_POINT ( 'NONE',  ( 4.458734124999998549, 10.02083333469892779, -2.574251347313721627 ) ) ;
#18235=CARTESIAN_POINT ( 'NONE',  ( 4.458734124999998549, -52.97916666530107932, -2.574251347313721627 ) ) ;
#18236=( BOUNDED_CURVE ( )  B_SPLINE_CURVE ( 2, ( #4783, #19892, #44011, #59144, #39507, #950, #54637, #15076, #54314 ),
 .UNSPECIFIED., .F., .F. ) 
 B_SPLINE_CURVE_WITH_KNOTS ( ( 3, 2, 2, 2, 3 ),
 ( 0.6232142857142857206, 0.6238095238095238138, 0.6250000000000000000, 0.6261904761904761862, 0.6267857142857142794 ),
 .UNSPECIFIED. ) 
 CURVE ( )  GEOMETRIC_REPRESENTATION_ITEM ( )  RATIONAL_B_SPLINE_CURVE ( ( 0.9330127018922194093, 0.9330127018922194093, 1.000000000000000000, 0.8660254037844387076, 1.000000000000000000, 0.8660254037844387076, 1.000000000000000000, 0.9330127018922194093, 0.9330127018922194093 ) ) 
 REPRESENTATION_ITEM ( '' )  );
#18240=CARTESIAN_POINT ( 'NONE',  ( 1.339745962155615144, -84.70534180126146850, 4.999999999999999112 ) ) ;
#18243=UNCERTAINTY_MEASURE_WITH_UNIT (LENGTH_MEASURE( 1.000000000000000082E-05 ), #54126, 'distance_accuracy_value', 'NONE');
#18246=CARTESIAN_POINT ( 'NONE',  ( 4.458734124999998549, -80.72916666530106511, -2.574251347313721627 ) ) ;
#18247=CARTESIAN_POINT ( 'NONE',  ( 4.458734124999998549, 25.02083333469892423, -2.574251347313721627 ) ) ;
#18252=CARTESIAN_POINT ( 'NONE',  ( 2.499999999999998668, -72.33333333333332860, -4.330127018922193649 ) ) ;
#18254=ORIENTED_EDGE ( 'NONE', *, *, #53403, .F. ) ;
#18256=CARTESIAN_POINT ( 'NONE',  ( -5.000000000000000000, -90.08333333333332860, -2.886751345948128211 ) ) ;
#18260=FACE_OUTER_BOUND ( 'NONE', #38812, .T. ) ;
#18261=EDGE_CURVE ( 'NONE', #49758, #41892, #18236, .T. ) ;
#18264=ORIENTED_EDGE ( 'NONE', *, *, #21391, .F. ) ;
#18267=ORIENTED_EDGE ( 'NONE', *, *, #62976, .T. ) ;
#18270=CARTESIAN_POINT ( 'NONE',  ( 4.458734124999999437, -52.06249999863440792, -5.460374474430324690E-16 ) ) ;
#18273=CARTESIAN_POINT ( 'NONE',  ( -2.500000000000000444, 9.958333336064519870, -4.330127018922193649 ) ) ;
#18274=ORIENTED_EDGE ( 'NONE', *, *, #59361, .T. ) ;
#18279=ORIENTED_EDGE ( 'NONE', *, *, #23550, .T. ) ;
#18282=CARTESIAN_POINT ( 'NONE',  ( -4.458734124999998549, -100.4791666653010509, 2.574251347313722516 ) ) ;
#18288=( BOUNDED_CURVE ( )  B_SPLINE_CURVE ( 2, ( #16476, #17437, #36411, #36733, #26765, #60867, #30946, #46063, #41860 ),
 .UNSPECIFIED., .F., .F. ) 
 B_SPLINE_CURVE_WITH_KNOTS ( ( 3, 2, 2, 2, 3 ),
 ( 0.6732142857142857650, 0.6738095238095238582, 0.6750000000000000444, 0.6761904761904762307, 0.6767857142857143238 ),
 .UNSPECIFIED. ) 
 CURVE ( )  GEOMETRIC_REPRESENTATION_ITEM ( )  RATIONAL_B_SPLINE_CURVE ( ( 0.9330127018922194093, 0.9330127018922194093, 1.000000000000000000, 0.8660254037844387076, 1.000000000000000000, 0.8660254037844387076, 1.000000000000000000, 0.9330127018922194093, 0.9330127018922194093 ) ) 
 REPRESENTATION_ITEM ( '' )  );
#18289=CARTESIAN_POINT ( 'NONE',  ( -6.972266317189433020E-16, -86.25000000000001421, -5.000000000000000000 ) ) ;
#18290=CARTESIAN_POINT ( 'NONE',  ( 2.229367062499998831, -8.645833331967736513, -3.861377020970580887 ) ) ;
#18291=CARTESIAN_POINT ( 'NONE',  ( -2.229367062499996610, -97.39583333196773651, 3.861377020970582219 ) ) ;
#18293=CARTESIAN_POINT ( 'NONE',  ( 2.229367062499998831, -29.89583333196773296, -3.861377020970580887 ) ) ;
#18300=CARTESIAN_POINT ( 'NONE',  ( -2.229367062500000163, 12.27083333469892601, -3.861377020970580443 ) ) ;
#18301=ORIENTED_EDGE ( 'NONE', *, *, #60522, .F. ) ;
#18302=CARTESIAN_POINT ( 'NONE',  ( -2.499999999999996447, -4.833333333333335702, 4.330127018922195425 ) ) ;
#18303=CARTESIAN_POINT ( 'NONE',  ( 2.499999999999998668, -90.33333333333332860, -4.330127018922193649 ) ) ;
#18304=CARTESIAN_POINT ( 'NONE',  ( 4.458734124999999437, -24.81249999863440436, -5.460374474430324690E-16 ) ) ;
#18306=CARTESIAN_POINT ( 'NONE',  ( -4.458734124999998549, -75.47916666530107932, 2.574251347313722516 ) ) ;
#18310=CARTESIAN_POINT ( 'NONE',  ( 2.229367062500001939, 2.020833334698927786, 3.861377020970579999 ) ) ;
#18311=CARTESIAN_POINT ( 'NONE',  ( 4.458734125000001214, 26.85416666803225993, 2.574251347313718519 ) ) ;
#18312=CARTESIAN_POINT ( 'NONE',  ( 2.229367062500001939, -38.22916666530107221, 3.861377020970579999 ) ) ;
#18315=CARTESIAN_POINT ( 'NONE',  ( 9.457646018065525792E-16, -70.06249999863439371, 5.148502694627439702 ) ) ;
#18317=CARTESIAN_POINT ( 'NONE',  ( 5.000000000000000888, -5.583333333333336590, 2.886751345948126879 ) ) ;
#18320=CARTESIAN_POINT ( 'NONE',  ( -4.458734124999999437, -63.39583333196772941, -2.574251347313719407 ) ) ;
#18321=CARTESIAN_POINT ( 'NONE',  ( -5.000000000000000000, -99.95833333060213022, -2.886751345948128211 ) ) ;
#18325=CARTESIAN_POINT ( 'NONE',  ( 5.000000000000000000, 9.625000002731184168, -6.123233995736766282E-16 ) ) ;
#18326=CARTESIAN_POINT ( 'NONE',  ( -3.152548672688508926E-16, -103.8124999986343937, -5.148502694627439702 ) ) ;
#18328=CARTESIAN_POINT ( 'NONE',  ( 2.499999999999998668, -56.33333333333333570, -4.330127018922193649 ) ) ;
#18331=VERTEX_POINT ( 'NONE', #10252 ) ;
#18332=LINE ( 'NONE', #61466, #4766 ) ;
#18337=VECTOR ( 'NONE', #21396, 1000.000000000000000 ) ;
#18341=ORIENTED_EDGE ( 'NONE', *, *, #39203, .T. ) ;
#18344=ORIENTED_EDGE ( 'NONE', *, *, #12203, .T. ) ;
#18348=CARTESIAN_POINT ( 'NONE',  ( 4.458734124999998549, -35.97916666530107221, -2.574251347313721627 ) ) ;
#18355=CARTESIAN_POINT ( 'NONE',  ( 2.499999999999998668, -54.33333333333332860, -4.330127018922193649 ) ) ;
#18356=CARTESIAN_POINT ( 'NONE',  ( -2.229367062499996610, -85.39583333196773651, 3.861377020970582219 ) ) ;
#18358=EDGE_LOOP ( 'NONE', ( #49280, #53521, #35918, #3404 ) ) ;
#18364=VECTOR ( 'NONE', #25790, 1000.000000000000000 ) ;
#18366=ORIENTED_EDGE ( 'NONE', *, *, #33355, .T. ) ;
#18369=CARTESIAN_POINT ( 'NONE',  ( 4.458734124999999437, -10.06249999863440614, -5.460374474430324690E-16 ) ) ;
#18372=CARTESIAN_POINT ( 'NONE',  ( -4.999999999999998224, -95.79166666393547303, 2.886751345948131764 ) ) ;
#18374=CARTESIAN_POINT ( 'NONE',  ( -4.458734124999999437, 24.43750000136559208, 0.000000000000000000 ) ) ;
#18376=CARTESIAN_POINT ( 'NONE',  ( -2.229367062499996610, -94.14583333196772230, 3.861377020970582219 ) ) ;
#18377=CARTESIAN_POINT ( 'NONE',  ( -1.339745962155613812, -31.20534180126147916, -5.000000000000000000 ) ) ;
#18379=CARTESIAN_POINT ( 'NONE',  ( 9.457646018065525792E-16, -8.062499998634404363, 5.148502694627439702 ) ) ;
#18380=LINE ( 'NONE', #56689, #33427 ) ;
#18382=FACE_OUTER_BOUND ( 'NONE', #21764, .T. ) ;
#18385=CARTESIAN_POINT ( 'NONE',  ( 5.000000000000000888, -37.45833333060213732, 2.886751345948126879 ) ) ;
#18386=CARTESIAN_POINT ( 'NONE',  ( 5.000000000000000000, -49.29166666393547303, -2.886751345948130876 ) ) ;
#18387=CARTESIAN_POINT ( 'NONE',  ( 4.458734124999999437, 21.18750000136559208, -5.460374474430324690E-16 ) ) ;
#18388=CARTESIAN_POINT ( 'NONE',  ( -1.339745962155613812, -98.08034179853028434, -5.000000000000000000 ) ) ;
#18390=CARTESIAN_POINT ( 'NONE',  ( -4.458734124999998549, -59.22916666530106511, 2.574251347313722516 ) ) ;
#18393=CARTESIAN_POINT ( 'NONE',  ( -2.500000000000000444, 9.833333333333332149, -4.330127018922193649 ) ) ;
#18396=CARTESIAN_POINT ( 'NONE',  ( -2.229367062500000163, -49.47916666530107221, -3.861377020970580443 ) ) ;
#18397=CARTESIAN_POINT ( 'NONE',  ( -5.000000000000000000, -84.95833333060215864, -2.886751345948128211 ) ) ;
#18400=CARTESIAN_POINT ( 'NONE',  ( -1.230605004983934782E-13, -36.75000000000000711, 5.000000000000000000 ) ) ;
#18401=CARTESIAN_POINT ( 'NONE',  ( 9.457646018065525792E-16, -91.31249999863440792, 5.148502694627439702 ) ) ;
#18403=CARTESIAN_POINT ( 'NONE',  ( 2.500000000000002220, -37.66666666666666430, 4.330127018922192761 ) ) ;
#18407=ORIENTED_EDGE ( 'NONE', *, *, #41590, .F. ) ;
#18408=CARTESIAN_POINT ( 'NONE',  ( -4.458734124999999437, -95.31249999863440792, 0.000000000000000000 ) ) ;
#18409=CARTESIAN_POINT ( 'NONE',  ( -4.458734124999999437, 9.437500001365593860, 0.000000000000000000 ) ) ;
#18411=CARTESIAN_POINT ( 'NONE',  ( 5.000000000000000000, 10.62500000273118594, -6.123233995736766282E-16 ) ) ;
#18417=CARTESIAN_POINT ( 'NONE',  ( 1.339745962155612702, -40.16965819600733312, -5.000000000000000000 ) ) ;
#18418=CARTESIAN_POINT ( 'NONE',  ( 1.339745962155615144, -63.70534180126147561, 4.999999999999999112 ) ) ;
#18421=CARTESIAN_POINT ( 'NONE',  ( -1.339745962155618253, 24.33034180399266333, 4.999999999999996447 ) ) ;
#18422=CARTESIAN_POINT ( 'NONE',  ( -4.458734124999998549, -18.47916666530106866, 2.574251347313722516 ) ) ;
#18423=LINE ( 'NONE', #19360, #42967 ) ;
#18428=CIRCLE ( 'NONE', #34866, 5.000000000000000000 ) ;
#18434=CARTESIAN_POINT ( 'NONE',  ( -4.458734124999998549, -67.47916666530106511, 2.574251347313722516 ) ) ;
#18436=CARTESIAN_POINT ( 'NONE',  ( 1.975475456537005874E-15, -12.74999999999999822, 5.000000000000000000 ) ) ;
#18441=ADVANCED_FACE ( 'NONE', ( #40151 ), #59794, .T. ) ;
#18442=CARTESIAN_POINT ( 'NONE',  ( 2.229367062500001939, 1.770833334698927786, 3.861377020970579999 ) ) ;
#18443=EDGE_LOOP ( 'NONE', ( #38143, #38476, #30191, #22012 ) ) ;
#18445=CARTESIAN_POINT ( 'NONE',  ( -4.458734124999998549, 3.770833334698929562, 2.574251347313722516 ) ) ;
#18448=CARTESIAN_POINT ( 'NONE',  ( 2.499999999999998668, -92.20833333060214443, -4.330127018922193649 ) ) ;
#18450=EDGE_LOOP ( 'NONE', ( #7894, #50386, #39664, #10567 ) ) ;
#18451=ORIENTED_EDGE ( 'NONE', *, *, #10688, .F. ) ;
#18452=CARTESIAN_POINT ( 'NONE',  ( -4.458734124999997661, -77.22916666530106511, 2.574251347313722516 ) ) ;
#18455=CARTESIAN_POINT ( 'NONE',  ( -4.458734124999999437, 6.604166668032259047, -2.574251347313719407 ) ) ;
#18458=CARTESIAN_POINT ( 'NONE',  ( -4.458734124999999437, -58.64583333196774362, -2.574251347313719407 ) ) ;
#18459=CARTESIAN_POINT ( 'NONE',  ( -2.499999999999996447, -18.70833333060214798, 4.330127018922195425 ) ) ;
#18461=CARTESIAN_POINT ( 'NONE',  ( 1.339745962155612702, -96.16965819600731891, -5.000000000000000000 ) ) ;
#18462=CARTESIAN_POINT ( 'NONE',  ( 2.500000000000002220, -42.54166666393548013, 4.330127018922192761 ) ) ;
#18463=CARTESIAN_POINT ( 'NONE',  ( -6.972266317189433020E-16, -15.12499999726881050, -5.000000000000000000 ) ) ;
#18466=CARTESIAN_POINT ( 'NONE',  ( 4.458734124999999437, -40.81249999863440081, -5.460374474430324690E-16 ) ) ;
#18468=CARTESIAN_POINT ( 'NONE',  ( -4.458734124999999437, -28.56249999863440081, 0.000000000000000000 ) ) ;
#18470=CARTESIAN_POINT ( 'NONE',  ( 5.000000000000000000, 25.50000000000000000, -6.123233995736766282E-16 ) ) ;
#18473=CARTESIAN_POINT ( 'NONE',  ( -2.229367062500000163, -105.7291666653010651, -3.861377020970580443 ) ) ;
#18474=CARTESIAN_POINT ( 'NONE',  ( 2.229367062499998831, -30.64583333196773651, -3.861377020970580887 ) ) ;
#18475=CARTESIAN_POINT ( 'NONE',  ( 5.000000000000000888, -70.45833333060214443, 2.886751345948126879 ) ) ;
#18478=CARTESIAN_POINT ( 'NONE',  ( -4.458734124999999437, -28.31249999863440081, 0.000000000000000000 ) ) ;
#18479=CARTESIAN_POINT ( 'NONE',  ( -3.152548672688508926E-16, -73.81249999863440792, -5.148502694627439702 ) ) ;
#18482=CYLINDRICAL_SURFACE ( 'NONE', #47135, 5.000000000000000000 ) ;
#18483=CARTESIAN_POINT ( 'NONE',  ( 5.000000000000000000, 22.70833333606451632, -2.886751345948130876 ) ) ;
#18484=CARTESIAN_POINT ( 'NONE',  ( -2.499999999999996447, -21.83333333333332860, 4.330127018922195425 ) ) ;
#18487=CARTESIAN_POINT ( 'NONE',  ( 1.975475456537005874E-15, -102.6249999972688158, 5.000000000000000000 ) ) ;
#18489=CARTESIAN_POINT ( 'NONE',  ( -5.000000000000000000, 25.04166666939785557, -2.886751345948128211 ) ) ;
#18491=CARTESIAN_POINT ( 'NONE',  ( -1.339745962155610925, -110.6696581960073189, 5.000000000000000000 ) ) ;
#18494=DIRECTION ( 'NONE',  ( -0.000000000000000000, 1.000000000000000000, -0.000000000000000000 ) ) ;
#18496=CARTESIAN_POINT ( 'NONE',  ( 5.000000000000000888, 28.41666666666666430, 2.886751345948126879 ) ) ;
#18501=ORIENTED_EDGE ( 'NONE', *, *, #50054, .T. ) ;
#18513=CARTESIAN_POINT ( 'NONE',  ( -2.500000000000000444, -39.04166666393548013, -4.330127018922193649 ) ) ;
#18517=EDGE_CURVE ( 'NONE', #50534, #5841, #50765, .T. ) ;
#18519=CARTESIAN_POINT ( 'NONE',  ( 4.458734124999998549, -80.72916666530106511, -2.574251347313721627 ) ) ;
#18520=CARTESIAN_POINT ( 'NONE',  ( 4.458734124999999437, 18.18750000136559564, -5.460374474430324690E-16 ) ) ;
#18521=CARTESIAN_POINT ( 'NONE',  ( -5.000000000000000000, -17.95833333060214798, -2.886751345948128211 ) ) ;
#18522=EDGE_CURVE ( 'NONE', #58767, #49758, #3412, .T. ) ;
#18523=VERTEX_POINT ( 'NONE', #50457 ) ;
#18527=CARTESIAN_POINT ( 'NONE',  ( 5.000000000000000888, -74.45833333060214443, 2.886751345948126879 ) ) ;
#18530=CARTESIAN_POINT ( 'NONE',  ( 9.457646018065525792E-16, -59.06249999863440792, 5.148502694627439702 ) ) ;
#18532=CARTESIAN_POINT ( 'NONE',  ( -4.458734124999999437, 23.60416666803225993, -2.574251347313719407 ) ) ;
#18533=EDGE_CURVE ( 'NONE', #1494, #49961, #31765, .T. ) ;
#18536=CARTESIAN_POINT ( 'NONE',  ( -2.229367062499996610, -44.39583333196774362, 3.861377020970582219 ) ) ;
#18537=CARTESIAN_POINT ( 'NONE',  ( 2.500000000000002220, -5.541666663935480130, 4.330127018922192761 ) ) ;
#18540=CYLINDRICAL_SURFACE ( 'NONE', #10106, 5.000000000000000000 ) ;
#18542=CARTESIAN_POINT ( 'NONE',  ( 4.458734125000000326, -105.8958333319677365, 2.574251347313718519 ) ) ;
#18543=CARTESIAN_POINT ( 'NONE',  ( 2.229367062499998831, -8.895833331967736513, -3.861377020970580887 ) ) ;
#18545=CARTESIAN_POINT ( 'NONE',  ( -3.152548672688508926E-16, -99.56249999863440792, -5.148502694627439702 ) ) ;
#18546=EDGE_CURVE ( 'NONE', #12070, #54038, #2839, .T. ) ;
#18548=CARTESIAN_POINT ( 'NONE',  ( -4.458734124999999437, -93.56249999863440792, 0.000000000000000000 ) ) ;
#18549=CARTESIAN_POINT ( 'NONE',  ( -5.000000000000000000, -53.87499999726880162, 0.000000000000000000 ) ) ;
#18550=CARTESIAN_POINT ( 'NONE',  ( -2.499999999999996447, 19.29166666939785202, 4.330127018922195425 ) ) ;
#18552=CARTESIAN_POINT ( 'NONE',  ( -2.229367062499996610, -11.14583333196773829, 3.861377020970582219 ) ) ;
#18553=CARTESIAN_POINT ( 'NONE',  ( 2.229367062499998831, 9.104166668032261711, -3.861377020970580887 ) ) ;
#18554=CARTESIAN_POINT ( 'NONE',  ( 4.458734124999998549, -60.97916666530106511, -2.574251347313721627 ) ) ;
#18555=CARTESIAN_POINT ( 'NONE',  ( -6.972266317189433020E-16, -69.24999999999998579, -5.000000000000000000 ) ) ;
#18564=CARTESIAN_POINT ( 'NONE',  ( 4.458734125000001214, -86.89583333196773651, 2.574251347313718519 ) ) ;
#18565=CARTESIAN_POINT ( 'NONE',  ( 4.458734125000001214, 26.85416666803225993, 2.574251347313718519 ) ) ;
#18566=( BOUNDED_CURVE ( )  B_SPLINE_CURVE ( 2, ( #52466, #3886, #33459, #43418, #52145, #58220, #8403, #42797, #9017 ),
 .UNSPECIFIED., .F., .F. ) 
 B_SPLINE_CURVE_WITH_KNOTS ( ( 3, 2, 2, 2, 3 ),
 ( 0.3839285714285714524, 0.3845238095238095455, 0.3857142857142857317, 0.3869047619047619180, 0.3875000000000000111 ),
 .UNSPECIFIED. ) 
 CURVE ( )  GEOMETRIC_REPRESENTATION_ITEM ( )  RATIONAL_B_SPLINE_CURVE ( ( 0.9330127018922194093, 0.9330127018922194093, 1.000000000000000000, 0.8660254037844387076, 1.000000000000000000, 0.8660254037844387076, 1.000000000000000000, 0.9330127018922194093, 0.9330127018922194093 ) ) 
 REPRESENTATION_ITEM ( '' )  );
#18569=CARTESIAN_POINT ( 'NONE',  ( 0.000000000000000000, -120.0000000000000000, 0.000000000000000000 ) ) ;
#18571=CARTESIAN_POINT ( 'NONE',  ( 2.500000000000002220, -71.66666666666667140, 4.330127018922192761 ) ) ;
#18581=ORIENTED_EDGE ( 'NONE', *, *, #767, .T. ) ;
#18587=CARTESIAN_POINT ( 'NONE',  ( 4.458734124999998549, -56.97916666530107932, -2.574251347313721627 ) ) ;
#18589=CARTESIAN_POINT ( 'NONE',  ( 1.975475456537005874E-15, -58.62499999726880162, 5.000000000000000000 ) ) ;
#18590=EDGE_LOOP ( 'NONE', ( #17025, #18809, #26900, #24521 ) ) ;
#18591=VECTOR ( 'NONE', #32891, 1000.000000000000000 ) ;
#18596=ADVANCED_FACE ( 'NONE', ( #33668 ), #32410, .T. ) ;
#18599=CARTESIAN_POINT ( 'NONE',  ( 9.457646018065525792E-16, -98.31249999863440792, 5.148502694627439702 ) ) ;
#18604=CARTESIAN_POINT ( 'NONE',  ( 1.339745962155612702, -83.29465819873851729, -5.000000000000000000 ) ) ;
#18605=CARTESIAN_POINT ( 'NONE',  ( 4.458734124999998549, -7.729166665301073103, -2.574251347313721627 ) ) ;
#18606=CARTESIAN_POINT ( 'NONE',  ( -4.458734124999999437, -100.6458333319677365, -2.574251347313719407 ) ) ;
#18608=CARTESIAN_POINT ( 'NONE',  ( 9.457646018065525792E-16, -27.31249999863440436, 5.148502694627439702 ) ) ;
#18609=LINE ( 'NONE', #24699, #21129 ) ;
#18613=EDGE_CURVE ( 'NONE', #24693, #29631, #20303, .T. ) ;
#18614=CARTESIAN_POINT ( 'NONE',  ( 2.499999999999998668, -21.20833333060214798, -4.330127018922193649 ) ) ;
#18615=CARTESIAN_POINT ( 'NONE',  ( -2.500000000000000444, 16.83333333333333215, -4.330127018922193649 ) ) ;
#18617=CARTESIAN_POINT ( 'NONE',  ( -4.458734124999999437, 4.354166668032260823, -2.574251347313719407 ) ) ;
#18622=CARTESIAN_POINT ( 'NONE',  ( 2.500000000000002220, -92.66666666666665719, 4.330127018922192761 ) ) ;
#18623=CARTESIAN_POINT ( 'NONE',  ( -2.229367062499996610, -32.14583333196773651, 3.861377020970582219 ) ) ;
#18624=LINE ( 'NONE', #58168, #58268 ) ;
#18625=CARTESIAN_POINT ( 'NONE',  ( -4.458734124999998549, -77.47916666530106511, 2.574251347313722516 ) ) ;
#18627=CARTESIAN_POINT ( 'NONE',  ( -1.339745962155610925, -101.6696581960073473, 5.000000000000000000 ) ) ;
#18630=CARTESIAN_POINT ( 'NONE',  ( -4.458734124999999437, 1.604166668032262155, -2.574251347313719407 ) ) ;
#18631=CARTESIAN_POINT ( 'NONE',  ( 4.458734124999998549, 26.02083333469892779, -2.574251347313721627 ) ) ;
#18632=CARTESIAN_POINT ( 'NONE',  ( 2.229367062500001939, -40.22916666530107221, 3.861377020970579999 ) ) ;
#18637=CARTESIAN_POINT ( 'NONE',  ( -4.458734124999998549, -69.22916666530107932, 2.574251347313722516 ) ) ;
#18638=CARTESIAN_POINT ( 'NONE',  ( 1.060575238724906964E-15, -101.6249999972688158, 5.773502691896257311 ) ) ;
#18639=DIRECTION ( 'NONE',  ( -0.000000000000000000, 1.000000000000000000, -0.000000000000000000 ) ) ;
#18640=CARTESIAN_POINT ( 'NONE',  ( -5.000000000000000000, -64.08333333333332860, -2.886751345948128211 ) ) ;
#18641=CARTESIAN_POINT ( 'NONE',  ( -2.229367062500000163, -106.7291666653010651, -3.861377020970580443 ) ) ;
#18643=CARTESIAN_POINT ( 'NONE',  ( 2.500000000000002220, -53.66666666666667140, 4.330127018922192761 ) ) ;
#18646=ORIENTED_EDGE ( 'NONE', *, *, #43284, .F. ) ;
#18648=CARTESIAN_POINT ( 'NONE',  ( -5.000000000000000000, -110.4374999986343937, 0.000000000000000000 ) ) ;
#18662=CARTESIAN_POINT ( 'NONE',  ( -4.458734124999999437, -38.64583333196772941, -2.574251347313719407 ) ) ;
#18669=ADVANCED_FACE ( 'NONE', ( #27895 ), #63262, .T. ) ;
#18671=CARTESIAN_POINT ( 'NONE',  ( -2.229367062500000163, -85.72916666530107932, -3.861377020970580443 ) ) ;
#18672=CARTESIAN_POINT ( 'NONE',  ( 1.339745962155612702, -34.16965819600732601, -5.000000000000000000 ) ) ;
#18674=CARTESIAN_POINT ( 'NONE',  ( 5.000000000000000000, -43.41666666666666430, -2.886751345948130876 ) ) ;
#18676=ORIENTED_EDGE ( 'NONE', *, *, #24057, .F. ) ;
#18678=CARTESIAN_POINT ( 'NONE',  ( -4.458734124999999437, -11.56249999863440792, 0.000000000000000000 ) ) ;
#18679=DIRECTION ( 'NONE',  ( 0.000000000000000000, 0.000000000000000000, 1.000000000000000000 ) ) ;
#18683=CARTESIAN_POINT ( 'NONE',  ( 9.457646018065525792E-16, 23.68750000136559564, 5.148502694627439702 ) ) ;
#18685=CARTESIAN_POINT ( 'NONE',  ( -4.458734124999999437, -92.39583333196773651, -2.574251347313719407 ) ) ;
#18688=CARTESIAN_POINT ( 'NONE',  ( -4.458734124999999437, -8.312499998634406140, 0.000000000000000000 ) ) ;
#18689=CARTESIAN_POINT ( 'NONE',  ( 5.000000000000000888, -39.45833333060214443, 2.886751345948126879 ) ) ;
#18692=CARTESIAN_POINT ( 'NONE',  ( -2.499999999999996447, -38.70833333060213732, 4.330127018922195425 ) ) ;
#18694=CARTESIAN_POINT ( 'NONE',  ( -2.229367062500000163, 19.52083333469893134, -3.861377020970580443 ) ) ;
#18697=CARTESIAN_POINT ( 'NONE',  ( 4.458734125000001214, -57.89583333196773651, 2.574251347313718519 ) ) ;
#18699=DIRECTION ( 'NONE',  ( -0.000000000000000000, 1.000000000000000000, -0.000000000000000000 ) ) ;
#18700=CARTESIAN_POINT ( 'NONE',  ( -5.000000000000000000, 10.91666666666666607, -2.886751345948128211 ) ) ;
#18702=CARTESIAN_POINT ( 'NONE',  ( 2.499999999999998668, -69.33333333333332860, -4.330127018922193649 ) ) ;
#18703=CARTESIAN_POINT ( 'NONE',  ( 2.229367062499998831, -46.64583333196774362, -3.861377020970580887 ) ) ;
#18704=CARTESIAN_POINT ( 'NONE',  ( -5.000000000000000000, -82.87499999726881583, 0.000000000000000000 ) ) ;
#18706=CARTESIAN_POINT ( 'NONE',  ( -6.972266317189433020E-16, -17.25000000000000000, -5.000000000000000000 ) ) ;
#18707=CARTESIAN_POINT ( 'NONE',  ( -1.339745962155610925, -91.79465819873853150, 5.000000000000000000 ) ) ;
#18708=CARTESIAN_POINT ( 'NONE',  ( 4.458734124999999437, -91.06249999863440792, -5.460374474430324690E-16 ) ) ;
#18710=CARTESIAN_POINT ( 'NONE',  ( 1.060575238724906964E-15, -40.74999999999999289, 5.773502691896257311 ) ) ;
#18712=ORIENTED_EDGE ( 'NONE', *, *, #12228, .F. ) ;
#18715=CARTESIAN_POINT ( 'NONE',  ( -3.152548672688508926E-16, -94.56249999863440792, -5.148502694627439702 ) ) ;
#18716=CARTESIAN_POINT ( 'NONE',  ( -4.458734124999999437, 10.43750000136559386, 0.000000000000000000 ) ) ;
#18717=CARTESIAN_POINT ( 'NONE',  ( -5.000000000000000000, 11.12500000273118594, 0.000000000000000000 ) ) ;
#18718=CARTESIAN_POINT ( 'NONE',  ( 2.500000000000002220, -80.66666666666665719, 4.330127018922192761 ) ) ;
#18722=CARTESIAN_POINT ( 'NONE',  ( -1.339745962155610925, -39.79465819873851729, 5.000000000000000000 ) ) ;
#18726=CARTESIAN_POINT ( 'NONE',  ( 2.500000000000002220, -19.66666666666666430, 4.330127018922192761 ) ) ;
#18729=CARTESIAN_POINT ( 'NONE',  ( 4.458734125000001214, -21.14583333196774362, 2.574251347313718519 ) ) ;
#18730=CARTESIAN_POINT ( 'NONE',  ( -1.339745962155606929, 21.91965820146970501, -5.000000000000004441 ) ) ;
#18735=( BOUNDED_CURVE ( )  B_SPLINE_CURVE ( 2, ( #34397, #35697, #49205, #11239, #30863, #24444, #15441, #5145, #39860 ),
 .UNSPECIFIED., .F., .F. ) 
 B_SPLINE_CURVE_WITH_KNOTS ( ( 3, 2, 2, 2, 3 ),
 ( 0.1053571428571428575, 0.1059523809523809507, 0.1071428571428571369, 0.1083333333333333370, 0.1089285714285714302 ),
 .UNSPECIFIED. ) 
 CURVE ( )  GEOMETRIC_REPRESENTATION_ITEM ( )  RATIONAL_B_SPLINE_CURVE ( ( 0.9330127018922194093, 0.9330127018922194093, 1.000000000000000000, 0.8660254037844387076, 1.000000000000000000, 0.8660254037844387076, 1.000000000000000000, 0.9330127018922194093, 0.9330127018922194093 ) ) 
 REPRESENTATION_ITEM ( '' )  );
#18738=ORIENTED_EDGE ( 'NONE', *, *, #60858, .F. ) ;
#18741=CARTESIAN_POINT ( 'NONE',  ( 4.458734124999998549, -66.97916666530107932, -2.574251347313721627 ) ) ;
#18743=ORIENTED_EDGE ( 'NONE', *, *, #32681, .F. ) ;
#18746=CARTESIAN_POINT ( 'NONE',  ( 4.458734124999999437, 1.937500001365593416, -5.460374474430324690E-16 ) ) ;
#18749=CARTESIAN_POINT ( 'NONE',  ( 2.493747252781420335E-13, -55.24999999999999289, -5.000000000000000000 ) ) ;
#18755=CARTESIAN_POINT ( 'NONE',  ( -3.152548672688508926E-16, -77.56249999863440792, -5.148502694627439702 ) ) ;
#18756=CARTESIAN_POINT ( 'NONE',  ( 0.000000000000000000, -120.0000000000000000, 0.000000000000000000 ) ) ;
#18757=CARTESIAN_POINT ( 'NONE',  ( 2.229367062500001939, 8.020833334698926009, 3.861377020970579999 ) ) ;
#18759=CARTESIAN_POINT ( 'NONE',  ( -2.229367062500000163, -57.72916666530107932, -3.861377020970580443 ) ) ;
#18760=CARTESIAN_POINT ( 'NONE',  ( -3.535250795749689387E-16, -22.12499999726881228, -5.773502691896257311 ) ) ;
#18762=CARTESIAN_POINT ( 'NONE',  ( 1.975475456537005874E-15, -58.75000000000000000, 5.000000000000000000 ) ) ;
#18763=CARTESIAN_POINT ( 'NONE',  ( -4.999999999999998224, -105.7916666639354588, 2.886751345948131764 ) ) ;
#18765=CARTESIAN_POINT ( 'NONE',  ( -4.458734124999999437, -40.31249999863440081, 0.000000000000000000 ) ) ;
#18766=CARTESIAN_POINT ( 'NONE',  ( -4.458734124999997661, -24.47916666530107577, 2.574251347313722516 ) ) ;
#18767=CYLINDRICAL_SURFACE ( 'NONE', #55662, 5.000000000000000000 ) ;
#18768=CARTESIAN_POINT ( 'NONE',  ( 1.060575238724906964E-15, 27.25000000000000000, 5.773502691896257311 ) ) ;
#18770=ORIENTED_EDGE ( 'NONE', *, *, #44085, .F. ) ;
#18771=CARTESIAN_POINT ( 'NONE',  ( 2.229367062499998831, -105.8958333319677365, -3.861377020970580887 ) ) ;
#18772=CARTESIAN_POINT ( 'NONE',  ( 4.458734124999998549, -32.72916666530107221, -2.574251347313721627 ) ) ;
#18773=CARTESIAN_POINT ( 'NONE',  ( -3.535250795749689387E-16, -67.12499999726881583, -5.773502691896257311 ) ) ;
#18776=CARTESIAN_POINT ( 'NONE',  ( -2.229367062500000163, -75.72916666530106511, -3.861377020970580443 ) ) ;
#18780=CARTESIAN_POINT ( 'NONE',  ( 5.000000000000000888, -5.458333330602148870, 2.886751345948126879 ) ) ;
#18781=CARTESIAN_POINT ( 'NONE',  ( 5.000000000000000888, -23.58333333333333215, 2.886751345948126879 ) ) ;
#18785=CARTESIAN_POINT ( 'NONE',  ( 5.000000000000000000, 24.62500000273118417, -6.123233995736766282E-16 ) ) ;
#18786=CARTESIAN_POINT ( 'NONE',  ( 2.499999999999998668, -48.20833333060215153, -4.330127018922193649 ) ) ;
#18788=EDGE_CURVE ( 'NONE', #19094, #63269, #3155, .T. ) ;
#18791=CARTESIAN_POINT ( 'NONE',  ( -1.975475456537005874E-15, 28.25000000000000000, 5.000000000000000000 ) ) ;
#18794=CARTESIAN_POINT ( 'NONE',  ( 0.000000000000000000, -120.0000000000000000, 5.000000000000000000 ) ) ;
#18796=( BOUNDED_CURVE ( )  B_SPLINE_CURVE ( 2, ( #48590, #13568, #43448, #34421, #23535, #354, #24470, #29599, #8737 ),
 .UNSPECIFIED., .F., .F. ) 
 B_SPLINE_CURVE_WITH_KNOTS ( ( 3, 2, 2, 2, 3 ),
 ( 0.5732142857142856762, 0.5738095238095237693, 0.5749999999999999556, 0.5761904761904761418, 0.5767857142857142350 ),
 .UNSPECIFIED. ) 
 CURVE ( )  GEOMETRIC_REPRESENTATION_ITEM ( )  RATIONAL_B_SPLINE_CURVE ( ( 0.9330127018922194093, 0.9330127018922194093, 1.000000000000000000, 0.8660254037844387076, 1.000000000000000000, 0.8660254037844387076, 1.000000000000000000, 0.9330127018922194093, 0.9330127018922194093 ) ) 
 REPRESENTATION_ITEM ( '' )  );
#18797=CARTESIAN_POINT ( 'NONE',  ( -1.339745962155610925, -71.66965819600733312, 5.000000000000000000 ) ) ;
#18802=ORIENTED_EDGE ( 'NONE', *, *, #39652, .F. ) ;
#18806=DIRECTION ( 'NONE',  ( -0.000000000000000000, 1.000000000000000000, -0.000000000000000000 ) ) ;
#18809=ORIENTED_EDGE ( 'NONE', *, *, #32997, .F. ) ;
#18810=CARTESIAN_POINT ( 'NONE',  ( -5.000000000000000000, -38.87499999726880162, 0.000000000000000000 ) ) ;
#18815=EDGE_CURVE ( 'NONE', #50284, #62586, #47822, .T. ) ;
#18817=CARTESIAN_POINT ( 'NONE',  ( -4.458734124999999437, -84.31249999863439371, 0.000000000000000000 ) ) ;
#18818=CARTESIAN_POINT ( 'NONE',  ( -4.458734124999998549, 16.77083333469892779, 2.574251347313722516 ) ) ;
#18824=CARTESIAN_POINT ( 'NONE',  ( 2.500000000000002220, -74.54166666393547303, 4.330127018922192761 ) ) ;
#18826=CARTESIAN_POINT ( 'NONE',  ( 1.975475456537005874E-15, -13.62499999726881228, 5.000000000000000000 ) ) ;
#18827=CARTESIAN_POINT ( 'NONE',  ( -4.458734124999999437, -62.31249999863440792, 0.000000000000000000 ) ) ;
#18828=LINE ( 'NONE', #29101, #37656 ) ;
#18829=CARTESIAN_POINT ( 'NONE',  ( 4.458734124999999437, 25.18750000136559208, -5.460374474430324690E-16 ) ) ;
#18830=CARTESIAN_POINT ( 'NONE',  ( -2.499999999999996447, -109.8333333333333428, 4.330127018922195425 ) ) ;
#18832=CARTESIAN_POINT ( 'NONE',  ( 4.458734124999999437, -42.06249999863440081, -5.460374474430324690E-16 ) ) ;
#18833=EDGE_CURVE ( 'NONE', #4271, #50284, #51872, .T. ) ;
#18834=CARTESIAN_POINT ( 'NONE',  ( -2.499999999999996447, -1.708333330602145761, 4.330127018922195425 ) ) ;
#18836=FACE_OUTER_BOUND ( 'NONE', #23353, .T. ) ;
#18838=CARTESIAN_POINT ( 'NONE',  ( -2.229367062499996610, -109.1458333319677365, 3.861377020970582219 ) ) ;
#18839=CARTESIAN_POINT ( 'NONE',  ( 4.458734125000000326, -9.145833331967736513, 2.574251347313718519 ) ) ;
#18840=ORIENTED_EDGE ( 'NONE', *, *, #32707, .F. ) ;
#18842=CARTESIAN_POINT ( 'NONE',  ( 2.229367062499998831, -96.64583333196773651, -3.861377020970580887 ) ) ;
#18844=CARTESIAN_POINT ( 'NONE',  ( 4.458734124999999437, -92.06249999863440792, -5.460374474430324690E-16 ) ) ;
#18845=CARTESIAN_POINT ( 'NONE',  ( 2.500000000000002220, -53.54166666393548013, 4.330127018922192761 ) ) ;
#18846=CARTESIAN_POINT ( 'NONE',  ( 0.000000000000000000, -120.0000000000000000, 0.000000000000000000 ) ) ;
#18849=CARTESIAN_POINT ( 'NONE',  ( 9.457646018065525792E-16, -14.06249999863440436, 5.148502694627439702 ) ) ;
#18850=CARTESIAN_POINT ( 'NONE',  ( 2.229367062499998831, 13.10416666803226171, -3.861377020970580887 ) ) ;
#18851=CARTESIAN_POINT ( 'NONE',  ( 4.458734124999998549, -59.97916666530106511, -2.574251347313721627 ) ) ;
#18852=DIRECTION ( 'NONE',  ( 0.000000000000000000, 0.000000000000000000, 1.000000000000000000 ) ) ;
#18856=ORIENTED_EDGE ( 'NONE', *, *, #18517, .T. ) ;
#18859=FACE_OUTER_BOUND ( 'NONE', #5811, .T. ) ;
#18860=CARTESIAN_POINT ( 'NONE',  ( -1.339745962155613812, -67.08034179853029855, -5.000000000000000000 ) ) ;
#18861=CARTESIAN_POINT ( 'NONE',  ( 4.458734125000001214, -87.89583333196773651, 2.574251347313718519 ) ) ;
#18862=CARTESIAN_POINT ( 'NONE',  ( -2.229367062499996610, 17.60416666803225993, 3.861377020970582219 ) ) ;
#18864=AXIS2_PLACEMENT_3D ( 'NONE', #5721, #270, #588 ) ;
#18866=EDGE_CURVE ( 'NONE', #20917, #1494, #984, .T. ) ;
#18871=CARTESIAN_POINT ( 'NONE',  ( 5.000000000000000888, -69.58333333333332860, 2.886751345948126879 ) ) ;
#18874=LINE ( 'NONE', #38491, #37654 ) ;
#18881=EDGE_CURVE ( 'NONE', #34481, #13658, #9958, .T. ) ;
#18886=EDGE_CURVE ( 'NONE', #57924, #42260, #7542, .T. ) ;
#18891=CARTESIAN_POINT ( 'NONE',  ( 4.458734124999999437, -57.06249999863440081, -5.460374474430324690E-16 ) ) ;
#18898=ORIENTED_EDGE ( 'NONE', *, *, #27101, .F. ) ;
#18901=CARTESIAN_POINT ( 'NONE',  ( -4.458734124999999437, -102.6458333319677507, -2.574251347313719407 ) ) ;
#18906=CARTESIAN_POINT ( 'NONE',  ( 9.457646018065525792E-16, -40.06249999863440081, 5.148502694627439702 ) ) ;
#18907=LINE ( 'NONE', #38522, #43474 ) ;
#18908=CARTESIAN_POINT ( 'NONE',  ( 4.458734124999999437, -13.81249999863440259, -5.460374474430324690E-16 ) ) ;
#18909=CARTESIAN_POINT ( 'NONE',  ( -2.229367062499996610, -100.3958333319677365, 3.861377020970582219 ) ) ;
#18912=CARTESIAN_POINT ( 'NONE',  ( -3.152548672688508926E-16, -30.81249999863440436, -5.148502694627439702 ) ) ;
#18916=DIRECTION ( 'NONE',  ( -0.000000000000000000, 1.000000000000000000, -0.000000000000000000 ) ) ;
#18917=CARTESIAN_POINT ( 'NONE',  ( 1.975475456537005874E-15, 7.375000002731185944, 5.000000000000000000 ) ) ;
#18919=CARTESIAN_POINT ( 'NONE',  ( -4.458734124999997661, 3.520833334698929118, 2.574251347313722516 ) ) ;
#18922=CARTESIAN_POINT ( 'NONE',  ( -2.500000000000000444, -96.16666666666665719, -4.330127018922193649 ) ) ;
#18923=CARTESIAN_POINT ( 'NONE',  ( -4.458734124999999437, -29.31249999863440436, 0.000000000000000000 ) ) ;
#18924=CARTESIAN_POINT ( 'NONE',  ( -5.000000000000000000, 7.041666669397852019, -2.886751345948128211 ) ) ;
#18925=CARTESIAN_POINT ( 'NONE',  ( -4.458734124999999437, -76.56249999863440792, 0.000000000000000000 ) ) ;
#18929=CARTESIAN_POINT ( 'NONE',  ( -4.458734124999999437, 3.687500001365594748, 0.000000000000000000 ) ) ;
#18930=CARTESIAN_POINT ( 'NONE',  ( -4.458734124999999437, 26.35416666803226349, -2.574251347313719407 ) ) ;
#18931=CARTESIAN_POINT ( 'NONE',  ( -4.458734124999997661, -44.47916666530106511, 2.574251347313722516 ) ) ;
#18936=CARTESIAN_POINT ( 'NONE',  ( -2.229367062499996610, -69.14583333196773651, 3.861377020970582219 ) ) ;
#18937=CARTESIAN_POINT ( 'NONE',  ( -5.000000000000000000, -103.8749999972688158, 0.000000000000000000 ) ) ;
#18939=EDGE_CURVE ( 'NONE', #24503, #31719, #25284, .T. ) ;
#18940=CARTESIAN_POINT ( 'NONE',  ( -6.972266317189433020E-16, -92.12499999726878741, -5.000000000000000000 ) ) ;
#18941=CARTESIAN_POINT ( 'NONE',  ( 2.229367062500001939, -107.2291666653010651, 3.861377020970579999 ) ) ;
#18943=CARTESIAN_POINT ( 'NONE',  ( -5.000000000000000000, -55.99999999999999289, 0.000000000000000000 ) ) ;
#18945=ORIENTED_EDGE ( 'NONE', *, *, #30823, .F. ) ;
#18947=EDGE_CURVE ( 'NONE', #5972, #50310, #40396, .T. ) ;
#18948=CARTESIAN_POINT ( 'NONE',  ( 2.499999999999998668, -27.20833333060214798, -4.330127018922193649 ) ) ;
#18951=ADVANCED_FACE ( 'NONE', ( #40070 ), #59712, .T. ) ;
#18958=CARTESIAN_POINT ( 'NONE',  ( 5.000000000000000888, -98.58333333333332860, 2.886751345948126879 ) ) ;
#18960=ORIENTED_EDGE ( 'NONE', *, *, #44729, .T. ) ;
#18965=CARTESIAN_POINT ( 'NONE',  ( -2.229367062500000163, -41.72916666530107932, -3.861377020970580443 ) ) ;
#18968=EDGE_CURVE ( 'NONE', #26333, #25814, #29290, .T. ) ;
#18975=CARTESIAN_POINT ( 'NONE',  ( 2.229367062499998831, -90.89583333196773651, -3.861377020970580887 ) ) ;
#18981=( BOUNDED_CURVE ( )  B_SPLINE_CURVE ( 2, ( #13282, #57050, #42546, #62185, #18105, #36462, #56089, #47690, #48626 ),
 .UNSPECIFIED., .F., .F. ) 
 B_SPLINE_CURVE_WITH_KNOTS ( ( 3, 2, 2, 2, 3 ),
 ( 0.6267857142857142794, 0.6273809523809523725, 0.6285714285714285587, 0.6297619047619047450, 0.6303571428571428381 ),
 .UNSPECIFIED. ) 
 CURVE ( )  GEOMETRIC_REPRESENTATION_ITEM ( )  RATIONAL_B_SPLINE_CURVE ( ( 0.9330127018922194093, 0.9330127018922194093, 1.000000000000000000, 0.8660254037844387076, 1.000000000000000000, 0.8660254037844387076, 1.000000000000000000, 0.9330127018922194093, 0.9330127018922194093 ) ) 
 REPRESENTATION_ITEM ( '' )  );
#18986=CARTESIAN_POINT ( 'NONE',  ( -4.458734124999999437, -13.56249999863440259, 0.000000000000000000 ) ) ;
#18988=CARTESIAN_POINT ( 'NONE',  ( -1.339745962155727277, -95.66965819600733312, 4.999999999999933387 ) ) ;
#18990=CARTESIAN_POINT ( 'NONE',  ( 4.458734124999998549, 23.02083333469892423, -2.574251347313721627 ) ) ;
#18992=CARTESIAN_POINT ( 'NONE',  ( -4.458734124999999437, -90.39583333196772230, -2.574251347313719407 ) ) ;
#18995=CARTESIAN_POINT ( 'NONE',  ( -4.458734124999999437, -16.39583333196773651, -2.574251347313719407 ) ) ;
#18996=CARTESIAN_POINT ( 'NONE',  ( 5.000000000000000000, -39.37499999726880162, -6.123233995736766282E-16 ) ) ;
#18997=CARTESIAN_POINT ( 'NONE',  ( -1.339745962155613812, -73.20534180126146850, -5.000000000000000000 ) ) ;
#19000=CARTESIAN_POINT ( 'NONE',  ( -2.499999999999996447, -39.70833333060214443, 4.330127018922195425 ) ) ;
#19002=CARTESIAN_POINT ( 'NONE',  ( 4.458734124999998549, 18.27083333469893134, -2.574251347313721627 ) ) ;
#19004=( BOUNDED_CURVE ( )  B_SPLINE_CURVE ( 2, ( #54875, #20784, #862, #40388, #35895, #35255, #12075, #46179, #40065 ),
 .UNSPECIFIED., .F., .F. ) 
 B_SPLINE_CURVE_WITH_KNOTS ( ( 3, 2, 2, 2, 3 ),
 ( 0.4803571428571428714, 0.4809523809523809645, 0.4821428571428571508, 0.4833333333333333370, 0.4839285714285714302 ),
 .UNSPECIFIED. ) 
 CURVE ( )  GEOMETRIC_REPRESENTATION_ITEM ( )  RATIONAL_B_SPLINE_CURVE ( ( 0.9330127018922194093, 0.9330127018922194093, 1.000000000000000000, 0.8660254037844387076, 1.000000000000000000, 0.8660254037844387076, 1.000000000000000000, 0.9330127018922194093, 0.9330127018922194093 ) ) 
 REPRESENTATION_ITEM ( '' )  );
#19005=ORIENTED_EDGE ( 'NONE', *, *, #59025, .T. ) ;
#19007=CARTESIAN_POINT ( 'NONE',  ( -3.152548672688508926E-16, -63.56249999863440792, -5.148502694627439702 ) ) ;
#19010=CARTESIAN_POINT ( 'NONE',  ( 5.000000000000000000, 10.49999999999999822, -6.123233995736766282E-16 ) ) ;
#19013=CARTESIAN_POINT ( 'NONE',  ( 4.458734124999998549, -55.72916666530107221, -2.574251347313721627 ) ) ;
#19014=CARTESIAN_POINT ( 'NONE',  ( -3.535250795749689387E-16, -82.12499999726883004, -5.773502691896257311 ) ) ;
#19016=CYLINDRICAL_SURFACE ( 'NONE', #39052, 5.000000000000000000 ) ;
#19017=DIRECTION ( 'NONE',  ( -0.000000000000000000, 1.000000000000000000, -0.000000000000000000 ) ) ;
#19018=CARTESIAN_POINT ( 'NONE',  ( 2.229367062499998831, -88.89583333196773651, -3.861377020970580887 ) ) ;
#19020=CARTESIAN_POINT ( 'NONE',  ( 5.000000000000000888, -38.58333333333332860, 2.886751345948126879 ) ) ;
#19021=CARTESIAN_POINT ( 'NONE',  ( 5.000000000000000000, -98.37499999726881583, -6.123233995736766282E-16 ) ) ;
#19024=CARTESIAN_POINT ( 'NONE',  ( -4.458734124999999437, -100.3958333319677365, -2.574251347313719407 ) ) ;
#19025=CARTESIAN_POINT ( 'NONE',  ( 4.458734124999999437, 7.937500001365595637, -5.460374474430324690E-16 ) ) ;
#19026=CARTESIAN_POINT ( 'NONE',  ( 5.000000000000000888, 12.54166666939785202, 2.886751345948126879 ) ) ;
#19031=PLANE ( 'NONE',  #2 ) ;
#19035=CARTESIAN_POINT ( 'NONE',  ( 0.000000000000000000, -120.0000000000000000, 5.000000000000000000 ) ) ;
#19038=CARTESIAN_POINT ( 'NONE',  ( -5.000000000000000000, 24.12500000273118417, 0.000000000000000000 ) ) ;
#19039=CARTESIAN_POINT ( 'NONE',  ( 4.458734124999998549, -26.97916666530107221, -2.574251347313721627 ) ) ;
#19049=VERTEX_POINT ( 'NONE', #30750 ) ;
#19052=CARTESIAN_POINT ( 'NONE',  ( -4.458734124999999437, -71.64583333196773651, -2.574251347313719407 ) ) ;
#19054=VERTEX_POINT ( 'NONE', #2451 ) ;
#19056=CARTESIAN_POINT ( 'NONE',  ( 4.458734124999998549, -0.9791666653010713262, -2.574251347313721627 ) ) ;
#19061=CARTESIAN_POINT ( 'NONE',  ( 1.339745962155615144, -92.58034179853028434, 4.999999999999999112 ) ) ;
#19063=VERTEX_POINT ( 'NONE', #55533 ) ;
#19064=CARTESIAN_POINT ( 'NONE',  ( -3.152548672688508926E-16, -78.56249999863440792, -5.148502694627439702 ) ) ;
#19066=CARTESIAN_POINT ( 'NONE',  ( 2.229367062499998831, 2.354166668032262599, -3.861377020970580887 ) ) ;
#19068=CARTESIAN_POINT ( 'NONE',  ( 4.458734124999998549, -67.97916666530107932, -2.574251347313721627 ) ) ;
#19069=CARTESIAN_POINT ( 'NONE',  ( 5.000000000000000888, -20.45833333060214798, 2.886751345948126879 ) ) ;
#19071=CARTESIAN_POINT ( 'NONE',  ( 2.500000000000002220, -44.54166666393547303, 4.330127018922192761 ) ) ;
#19072=CARTESIAN_POINT ( 'NONE',  ( -5.000000000000000000, -59.08333333333332860, -2.886751345948128211 ) ) ;
#19073=CARTESIAN_POINT ( 'NONE',  ( 1.975475456537005874E-15, 14.37500000273118417, 5.000000000000000000 ) ) ;
#19074=CYLINDRICAL_SURFACE ( 'NONE', #31594, 5.000000000000000000 ) ;
#19075=CARTESIAN_POINT ( 'NONE',  ( -2.229367062499996610, -41.14583333196773651, 3.861377020970582219 ) ) ;
#19076=CARTESIAN_POINT ( 'NONE',  ( -4.458734124999999437, -24.56249999863440436, 0.000000000000000000 ) ) ;
#19079=CARTESIAN_POINT ( 'NONE',  ( -2.500000000000000444, 23.83333333333333215, -4.330127018922193649 ) ) ;
#19081=CARTESIAN_POINT ( 'NONE',  ( 4.458734124999999437, -107.0624999986343937, -5.460374474430324690E-16 ) ) ;
#19082=CARTESIAN_POINT ( 'NONE',  ( 4.458734124999998549, -36.72916666530107221, -2.574251347313721627 ) ) ;
#19083=CARTESIAN_POINT ( 'NONE',  ( -5.000000000000000000, -65.95833333060213022, -2.886751345948128211 ) ) ;
#19087=CARTESIAN_POINT ( 'NONE',  ( 2.229367062500001939, -75.22916666530106511, 3.861377020970579999 ) ) ;
#19090=DIRECTION ( 'NONE',  ( -0.000000000000000000, 1.000000000000000000, -0.000000000000000000 ) ) ;
#19092=CARTESIAN_POINT ( 'NONE',  ( -3.535250795749689387E-16, -21.24999999999999645, -5.773502691896257311 ) ) ;
#19094=VERTEX_POINT ( 'NONE', #17228 ) ;
#19096=CARTESIAN_POINT ( 'NONE',  ( -5.000000000000000000, -49.08333333333332860, -2.886751345948128211 ) ) ;
#19098=CARTESIAN_POINT ( 'NONE',  ( 5.000000000000000000, 27.70833333606451987, -2.886751345948129988 ) ) ;
#19101=( BOUNDED_CURVE ( )  B_SPLINE_CURVE ( 2, ( #44348, #14132, #14449, #10269, #311, #18958, #58205, #48548, #63359 ),
 .UNSPECIFIED., .F., .F. ) 
 B_SPLINE_CURVE_WITH_KNOTS ( ( 3, 2, 2, 2, 3 ),
 ( 0.9160714285714285365, 0.9166666666666666297, 0.9178571428571428159, 0.9190476190476190022, 0.9196428571428570953 ),
 .UNSPECIFIED. ) 
 CURVE ( )  GEOMETRIC_REPRESENTATION_ITEM ( )  RATIONAL_B_SPLINE_CURVE ( ( 0.9330127018922194093, 0.9330127018922194093, 1.000000000000000000, 0.8660254037844387076, 1.000000000000000000, 0.8660254037844387076, 1.000000000000000000, 0.9330127018922194093, 0.9330127018922194093 ) ) 
 REPRESENTATION_ITEM ( '' )  );
#19102=DIRECTION ( 'NONE',  ( -0.000000000000000000, 1.000000000000000000, -0.000000000000000000 ) ) ;
#19105=CARTESIAN_POINT ( 'NONE',  ( 1.975475456537005874E-15, -76.75000000000000000, 5.000000000000000000 ) ) ;
#19107=CARTESIAN_POINT ( 'NONE',  ( -1.339745962155610925, -87.66965819600731891, 5.000000000000000000 ) ) ;
#19108=CARTESIAN_POINT ( 'NONE',  ( -4.458734124999998549, -19.22916666530106866, 2.574251347313722516 ) ) ;
#19109=CARTESIAN_POINT ( 'NONE',  ( -6.972266317189433020E-16, -72.12499999726878741, -5.000000000000000000 ) ) ;
#19112=( BOUNDED_CURVE ( )  B_SPLINE_CURVE ( 2, ( #13893, #19661, #29297, #48926, #38343, #24495, #18718, #54074, #14830 ),
 .UNSPECIFIED., .F., .F. ) 
 B_SPLINE_CURVE_WITH_KNOTS ( ( 3, 2, 2, 2, 3 ),
 ( 0.7874999999999999778, 0.7880952380952380709, 0.7892857142857142572, 0.7904761904761904434, 0.7910714285714285365 ),
 .UNSPECIFIED. ) 
 CURVE ( )  GEOMETRIC_REPRESENTATION_ITEM ( )  RATIONAL_B_SPLINE_CURVE ( ( 0.9330127018922194093, 0.9330127018922194093, 1.000000000000000000, 0.8660254037844387076, 1.000000000000000000, 0.8660254037844387076, 1.000000000000000000, 0.9330127018922194093, 0.9330127018922194093 ) ) 
 REPRESENTATION_ITEM ( '' )  );
#19114=ORIENTED_EDGE ( 'NONE', *, *, #30448, .F. ) ;
#19117=CARTESIAN_POINT ( 'NONE',  ( 5.000000000000000000, -87.50000000000000000, -6.123233995736766282E-16 ) ) ;
#19118=CARTESIAN_POINT ( 'NONE',  ( -2.499999999999996447, -67.70833333060214443, 4.330127018922195425 ) ) ;
#19120=ORIENTED_EDGE ( 'NONE', *, *, #1962, .F. ) ;
#19122=VECTOR ( 'NONE', #44572, 1000.000000000000000 ) ;
#19125=CARTESIAN_POINT ( 'NONE',  ( -6.972266317189433020E-16, -53.12499999726880162, -5.000000000000000000 ) ) ;
#19127=VECTOR ( 'NONE', #17707, 1000.000000000000000 ) ;
#19130=CARTESIAN_POINT ( 'NONE',  ( 2.500000000000002220, -103.5416666639354730, 4.330127018922192761 ) ) ;
#19131=CARTESIAN_POINT ( 'NONE',  ( -2.229367062500000163, 18.52083333469892779, -3.861377020970580443 ) ) ;
#19133=VERTEX_POINT ( 'NONE', #2761 ) ;
#19137=CARTESIAN_POINT ( 'NONE',  ( 2.499999999999998668, -39.33333333333332860, -4.330127018922193649 ) ) ;
#19139=CARTESIAN_POINT ( 'NONE',  ( -4.458734124999997661, -59.22916666530106511, 2.574251347313722516 ) ) ;
#19141=CARTESIAN_POINT ( 'NONE',  ( 4.458734124999998549, 25.27083333469892779, -2.574251347313721627 ) ) ;
#19143=CARTESIAN_POINT ( 'NONE',  ( 2.499999999999998668, -109.3333333333333428, -4.330127018922193649 ) ) ;
#19144=CARTESIAN_POINT ( 'NONE',  ( -4.458734124999999437, -48.64583333196773651, -2.574251347313719407 ) ) ;
#19145=CARTESIAN_POINT ( 'NONE',  ( 2.500000000000002220, -2.541666663935477466, 4.330127018922192761 ) ) ;
#19147=DIRECTION ( 'NONE',  ( -0.000000000000000000, 1.000000000000000000, -0.000000000000000000 ) ) ;
#19149=CARTESIAN_POINT ( 'NONE',  ( 2.229367062500001939, -107.9791666653010651, 3.861377020970579999 ) ) ;
#19150=CARTESIAN_POINT ( 'NONE',  ( 4.458734125000000326, -13.14583333196774184, 2.574251347313718519 ) ) ;
#19151=ORIENTED_EDGE ( 'NONE', *, *, #16307, .T. ) ;
#19153=CARTESIAN_POINT ( 'NONE',  ( 4.458734125000001214, -99.89583333196772230, 2.574251347313718519 ) ) ;
#19155=CARTESIAN_POINT ( 'NONE',  ( -2.229367062499996610, -93.39583333196773651, 3.861377020970582219 ) ) ;
#19156=CARTESIAN_POINT ( 'NONE',  ( -4.999999999999999112, -49.79166666393547303, 2.886751345948131764 ) ) ;
#19161=CARTESIAN_POINT ( 'NONE',  ( -3.152548672688508926E-16, -15.56249999863440614, -5.148502694627439702 ) ) ;
#19162=CARTESIAN_POINT ( 'NONE',  ( -3.152548672688508926E-16, 13.18750000136559208, -5.148502694627439702 ) ) ;
#19164=CARTESIAN_POINT ( 'NONE',  ( -2.229367062500000163, -56.72916666530107221, -3.861377020970580443 ) ) ;
#19167=CARTESIAN_POINT ( 'NONE',  ( 1.339745962155612702, -8.169658196007333117, -5.000000000000000000 ) ) ;
#19169=ORIENTED_EDGE ( 'NONE', *, *, #1696, .F. ) ;
#19171=( BOUNDED_CURVE ( )  B_SPLINE_CURVE ( 2, ( #37725, #29552, #8462, #35041, #24744, #54653, #30188, #5761, #49816 ),
 .UNSPECIFIED., .F., .F. ) 
 B_SPLINE_CURVE_WITH_KNOTS ( ( 3, 2, 2, 2, 3 ),
 ( 0.7482142857142857206, 0.7488095238095238138, 0.7500000000000000000, 0.7511904761904761862, 0.7517857142857142794 ),
 .UNSPECIFIED. ) 
 CURVE ( )  GEOMETRIC_REPRESENTATION_ITEM ( )  RATIONAL_B_SPLINE_CURVE ( ( 0.9330127018922194093, 0.9330127018922194093, 1.000000000000000000, 0.8660254037844387076, 1.000000000000000000, 0.8660254037844387076, 1.000000000000000000, 0.9330127018922194093, 0.9330127018922194093 ) ) 
 REPRESENTATION_ITEM ( '' )  );
#19174=CARTESIAN_POINT ( 'NONE',  ( -5.000000000000000000, -91.95833333060214443, -2.886751345948128211 ) ) ;
#19175=DIRECTION ( 'NONE',  ( -0.000000000000000000, 1.000000000000000000, -0.000000000000000000 ) ) ;
#19176=CARTESIAN_POINT ( 'NONE',  ( -2.229367062500000163, -86.47916666530107932, -3.861377020970580443 ) ) ;
#19177=CARTESIAN_POINT ( 'NONE',  ( -4.458734124999998549, 20.52083333469892423, 2.574251347313722516 ) ) ;
#19182=CARTESIAN_POINT ( 'NONE',  ( 0.000000000000000000, -120.0000000000000000, 5.000000000000000000 ) ) ;
#19184=CARTESIAN_POINT ( 'NONE',  ( 5.000000000000000888, -71.58333333333332860, 2.886751345948126879 ) ) ;
#19187=CARTESIAN_POINT ( 'NONE',  ( 5.000000000000000000, -102.4166666666666572, -2.886751345948130876 ) ) ;
#19190=CYLINDRICAL_SURFACE ( 'NONE', #38822, 5.000000000000000000 ) ;
#19195=VERTEX_POINT ( 'NONE', #48386 ) ;
#19201=CYLINDRICAL_SURFACE ( 'NONE', #43276, 5.000000000000000000 ) ;
#19202=CARTESIAN_POINT ( 'NONE',  ( 9.457646018065525792E-16, -55.31249999863439371, 5.148502694627439702 ) ) ;
#19211=CARTESIAN_POINT ( 'NONE',  ( 9.457646018065525792E-16, -104.3124999986344221, 5.148502694627439702 ) ) ;
#19213=VERTEX_POINT ( 'NONE', #43237 ) ;
#19216=CARTESIAN_POINT ( 'NONE',  ( -3.152548672688508926E-16, -40.56249999863440081, -5.148502694627439702 ) ) ;
#19220=EDGE_CURVE ( 'NONE', #43789, #60902, #43241, .T. ) ;
#19222=CARTESIAN_POINT ( 'NONE',  ( 2.229367062499998831, -14.64583333196773474, -3.861377020970580887 ) ) ;
#19224=CARTESIAN_POINT ( 'NONE',  ( 2.229367062500001939, -100.2291666653010651, 3.861377020970579999 ) ) ;
#19225=EDGE_LOOP ( 'NONE', ( #5829, #24964, #30700, #36093 ) ) ;
#19227=CARTESIAN_POINT ( 'NONE',  ( 2.229367062499998831, -26.89583333196774007, -3.861377020970580887 ) ) ;
#19228=CARTESIAN_POINT ( 'NONE',  ( -4.999999999999998224, 12.08333333333333215, 2.886751345948131764 ) ) ;
#19231=CARTESIAN_POINT ( 'NONE',  ( 1.975475456537005874E-15, -15.75000000000000000, 5.000000000000000000 ) ) ;
#19234=CARTESIAN_POINT ( 'NONE',  ( -3.152548672688508926E-16, 4.187500001365595637, -5.148502694627439702 ) ) ;
#19237=CARTESIAN_POINT ( 'NONE',  ( -2.500000000000000444, -98.16666666666665719, -4.330127018922193649 ) ) ;
#19238=CARTESIAN_POINT ( 'NONE',  ( 4.458734125000001214, -30.89583333196773296, 2.574251347313718519 ) ) ;
#19240=CARTESIAN_POINT ( 'NONE',  ( 1.975475456537005874E-15, -22.62499999726880873, 5.000000000000000000 ) ) ;
#19241=CARTESIAN_POINT ( 'NONE',  ( 4.458734125000001214, -75.14583333196775072, 2.574251347313718519 ) ) ;
#19243=DIRECTION ( 'NONE',  ( -0.000000000000000000, 1.000000000000000000, -0.000000000000000000 ) ) ;
#19245=CARTESIAN_POINT ( 'NONE',  ( -4.458734124999999437, -4.395833331967740065, -2.574251347313719407 ) ) ;
#19246=CARTESIAN_POINT ( 'NONE',  ( -2.229367062500000163, 28.27083333469892779, -3.861377020970580443 ) ) ;
#19248=CARTESIAN_POINT ( 'NONE',  ( 4.458734125000000326, -44.14583333196774362, 2.574251347313718519 ) ) ;
#19251=EDGE_CURVE ( 'NONE', #22002, #43496, #47759, .T. ) ;
#19253=CARTESIAN_POINT ( 'NONE',  ( 4.458734125000001214, -71.89583333196773651, 2.574251347313718519 ) ) ;
#19254=CARTESIAN_POINT ( 'NONE',  ( -5.000000000000000000, -106.9583333306021302, -2.886751345948128211 ) ) ;
#19259=CARTESIAN_POINT ( 'NONE',  ( -2.500000000000000444, -53.16666666666666430, -4.330127018922193649 ) ) ;
#19273=ORIENTED_EDGE ( 'NONE', *, *, #50161, .F. ) ;
#19274=CARTESIAN_POINT ( 'NONE',  ( 1.975475456537005874E-15, 5.250000000000000000, 5.000000000000000000 ) ) ;
#19275=CARTESIAN_POINT ( 'NONE',  ( 1.975475456537005874E-15, -45.62499999726880873, 5.000000000000000000 ) ) ;
#19277=ORIENTED_EDGE ( 'NONE', *, *, #12203, .F. ) ;
#19281=CARTESIAN_POINT ( 'NONE',  ( 9.457646018065525792E-16, -40.31249999863440081, 5.148502694627439702 ) ) ;
#19282=VECTOR ( 'NONE', #57920, 1000.000000000000000 ) ;
#19291=CARTESIAN_POINT ( 'NONE',  ( -2.229367062500000163, -89.72916666530106511, -3.861377020970580443 ) ) ;
#19297=CARTESIAN_POINT ( 'NONE',  ( -5.000000000000000000, -105.0833333333333286, -2.886751345948128211 ) ) ;
#19298=VERTEX_POINT ( 'NONE', #52595 ) ;
#19303=CARTESIAN_POINT ( 'NONE',  ( 2.229367062499998831, -9.895833331967738289, -3.861377020970580887 ) ) ;
#19305=CYLINDRICAL_SURFACE ( 'NONE', #39425, 5.000000000000000000 ) ;
#19307=CARTESIAN_POINT ( 'NONE',  ( -2.500000000000000444, -74.04166666393547303, -4.330127018922193649 ) ) ;
#19309=CARTESIAN_POINT ( 'NONE',  ( -4.458734124999997661, 22.52083333469892423, 2.574251347313722516 ) ) ;
#19311=CARTESIAN_POINT ( 'NONE',  ( 4.458734124999998549, -92.72916666530106511, -2.574251347313721627 ) ) ;
#19313=CARTESIAN_POINT ( 'NONE',  ( -1.339745962155610925, -103.6696581960073331, 5.000000000000000000 ) ) ;
#19314=CARTESIAN_POINT ( 'NONE',  ( -2.229367062500000163, -16.47916666530107577, -3.861377020970580443 ) ) ;
#19315=CARTESIAN_POINT ( 'NONE',  ( -5.000000000000000000, -109.9999999999999858, 0.000000000000000000 ) ) ;
#19317=CARTESIAN_POINT ( 'NONE',  ( 5.000000000000000000, -42.37499999726880873, -6.123233995736766282E-16 ) ) ;
#19319=CARTESIAN_POINT ( 'NONE',  ( 9.457646018065525792E-16, 18.93750000136559564, 5.148502694627439702 ) ) ;
#19320=CARTESIAN_POINT ( 'NONE',  ( -2.916731409357579869E-14, 12.37500000273118594, 5.000000000000000888 ) ) ;
#19324=EDGE_CURVE ( 'NONE', #29404, #32980, #10869, .T. ) ;
#19325=CARTESIAN_POINT ( 'NONE',  ( -4.458734124999999437, -61.31249999863440081, 0.000000000000000000 ) ) ;
#19328=CARTESIAN_POINT ( 'NONE',  ( 5.000000000000000888, 12.41666666666666607, 2.886751345948126879 ) ) ;
#19332=CARTESIAN_POINT ( 'NONE',  ( -3.152548672688508926E-16, -54.56249999863439371, -5.148502694627439702 ) ) ;
#19333=CARTESIAN_POINT ( 'NONE',  ( -4.999999999999999112, -90.79166666393545881, 2.886751345948131764 ) ) ;
#19335=DIRECTION ( 'NONE',  ( -0.000000000000000000, 1.000000000000000000, -0.000000000000000000 ) ) ;
#19337=CARTESIAN_POINT ( 'NONE',  ( -2.229367062499996610, -89.39583333196773651, 3.861377020970582219 ) ) ;
#19339=CARTESIAN_POINT ( 'NONE',  ( -2.500000000000000444, -39.16666666666667140, -4.330127018922193649 ) ) ;
#19342=ORIENTED_EDGE ( 'NONE', *, *, #17948, .F. ) ;
#19343=CARTESIAN_POINT ( 'NONE',  ( -4.458734124999999437, -101.3124999986344079, 0.000000000000000000 ) ) ;
#19344=CARTESIAN_POINT ( 'NONE',  ( -4.458734124999999437, 5.437500001365592972, 0.000000000000000000 ) ) ;
#19354=( BOUNDED_CURVE ( )  B_SPLINE_CURVE ( 2, ( #318, #54979, #19916, #39530, #45326, #15100, #45646, #5449, #34387 ),
 .UNSPECIFIED., .F., .F. ) 
 B_SPLINE_CURVE_WITH_KNOTS ( ( 3, 2, 2, 2, 3 ),
 ( 0.6946428571428571175, 0.6952380952380952106, 0.6964285714285713969, 0.6976190476190475831, 0.6982142857142856762 ),
 .UNSPECIFIED. ) 
 CURVE ( )  GEOMETRIC_REPRESENTATION_ITEM ( )  RATIONAL_B_SPLINE_CURVE ( ( 0.9330127018922194093, 0.9330127018922194093, 1.000000000000000000, 0.8660254037844387076, 1.000000000000000000, 0.8660254037844387076, 1.000000000000000000, 0.9330127018922194093, 0.9330127018922194093 ) ) 
 REPRESENTATION_ITEM ( '' )  );
#19355=CARTESIAN_POINT ( 'NONE',  ( -4.999999999999998224, 25.08333333333333215, 2.886751345948131764 ) ) ;
#19359=CARTESIAN_POINT ( 'NONE',  ( -4.458734124999999437, -26.56249999863440792, 0.000000000000000000 ) ) ;
#19360=CARTESIAN_POINT ( 'NONE',  ( 0.000000000000000000, -120.0000000000000000, 5.000000000000000000 ) ) ;
#19364=AXIS2_PLACEMENT_3D ( 'NONE', #21758, #11452, #60041 ) ;
#19371=CARTESIAN_POINT ( 'NONE',  ( 2.229367062500001939, -73.22916666530107932, 3.861377020970579999 ) ) ;
#19378=CARTESIAN_POINT ( 'NONE',  ( -4.458734124999998549, 1.520833334698927342, 2.574251347313722516 ) ) ;
#19379=VERTEX_POINT ( 'NONE', #24257 ) ;
#19380=VECTOR ( 'NONE', #30015, 1000.000000000000000 ) ;
#19382=( BOUNDED_CURVE ( )  B_SPLINE_CURVE ( 2, ( #61155, #37019, #61470, #17404, #3866, #41502, #17078, #31866, #23165 ),
 .UNSPECIFIED., .F., .F. ) 
 B_SPLINE_CURVE_WITH_KNOTS ( ( 3, 2, 2, 2, 3 ),
 ( 0.4267857142857142683, 0.4273809523809523614, 0.4285714285714285476, 0.4297619047619047894, 0.4303571428571428825 ),
 .UNSPECIFIED. ) 
 CURVE ( )  GEOMETRIC_REPRESENTATION_ITEM ( )  RATIONAL_B_SPLINE_CURVE ( ( 0.9330127018922194093, 0.9330127018922194093, 1.000000000000000000, 0.8660254037844387076, 1.000000000000000000, 0.8660254037844387076, 1.000000000000000000, 0.9330127018922194093, 0.9330127018922194093 ) ) 
 REPRESENTATION_ITEM ( '' )  );
#19385=CARTESIAN_POINT ( 'NONE',  ( 2.500000000000002220, -92.54166666393547303, 4.330127018922192761 ) ) ;
#19387=ORIENTED_EDGE ( 'NONE', *, *, #60987, .T. ) ;
#19388=CARTESIAN_POINT ( 'NONE',  ( 2.229367062499998831, -74.64583333196773651, -3.861377020970580887 ) ) ;
#19390=CARTESIAN_POINT ( 'NONE',  ( -4.458734124999998549, 2.770833334698928674, 2.574251347313722516 ) ) ;
#19392=CARTESIAN_POINT ( 'NONE',  ( -4.458734124999998549, -64.47916666530106511, 2.574251347313722516 ) ) ;
#19393=CARTESIAN_POINT ( 'NONE',  ( -5.000000000000000000, -23.87499999726881228, 0.000000000000000000 ) ) ;
#19394=CARTESIAN_POINT ( 'NONE',  ( 1.975475456537005874E-15, -96.62499999726880162, 5.000000000000000000 ) ) ;
#19395=CARTESIAN_POINT ( 'NONE',  ( 1.339745962155612702, -28.16965819600733312, -5.000000000000000000 ) ) ;
#19396=CARTESIAN_POINT ( 'NONE',  ( -1.339745962155610925, -64.66965819600733312, 5.000000000000000000 ) ) ;
#19398=CARTESIAN_POINT ( 'NONE',  ( 4.458734124999999437, -46.81249999863440792, -5.460374474430324690E-16 ) ) ;
#19400=CARTESIAN_POINT ( 'NONE',  ( 4.458734124999998549, -24.97916666530106511, -2.574251347313721627 ) ) ;
#19402=VECTOR ( 'NONE', #20149, 1000.000000000000000 ) ;
#19405=CARTESIAN_POINT ( 'NONE',  ( -3.535250795749689387E-16, 27.75000000000000000, -5.773502691896257311 ) ) ;
#19408=DIRECTION ( 'NONE',  ( -0.8660254037844410391, -0.4999999999999958367, -0.000000000000000000 ) ) ;
#19410=CARTESIAN_POINT ( 'NONE',  ( -4.458734124999999437, -39.31249999863440081, 0.000000000000000000 ) ) ;
#19411=CARTESIAN_POINT ( 'NONE',  ( 5.000000000000000000, -74.29166666393547303, -2.886751345948129988 ) ) ;
#19415=CARTESIAN_POINT ( 'NONE',  ( 4.458734124999998549, -74.97916666530106511, -2.574251347313721627 ) ) ;
#19420=CARTESIAN_POINT ( 'NONE',  ( 1.060575238724906964E-15, -23.75000000000000000, 5.773502691896257311 ) ) ;
#19427=CARTESIAN_POINT ( 'NONE',  ( 1.339745962155615144, -48.58034179853029855, 4.999999999999999112 ) ) ;
#19434=CARTESIAN_POINT ( 'NONE',  ( -2.500000000000000444, -88.04166666393548724, -4.330127018922193649 ) ) ;
#19435=CARTESIAN_POINT ( 'NONE',  ( 1.339745962155627135, 18.70534180126147916, -4.999999999999991118 ) ) ;
#19436=CARTESIAN_POINT ( 'NONE',  ( 9.457646018065525792E-16, -22.06249999863440436, 5.148502694627439702 ) ) ;
#19443=VERTEX_POINT ( 'NONE', #60600 ) ;
#19444=CARTESIAN_POINT ( 'NONE',  ( 1.339745962155615144, -87.70534180126146850, 4.999999999999999112 ) ) ;
#19445=CARTESIAN_POINT ( 'NONE',  ( -5.000000000000000000, -3.000000000000002665, 0.000000000000000000 ) ) ;
#19447=ORIENTED_EDGE ( 'NONE', *, *, #7146, .T. ) ;
#19450=AXIS2_PLACEMENT_3D ( 'NONE', #63341, #32807, #34054 ) ;
#19454=CARTESIAN_POINT ( 'NONE',  ( 5.000000000000000000, -103.2916666639354730, -2.886751345948130876 ) ) ;
#19455=CARTESIAN_POINT ( 'NONE',  ( -4.458734124999999437, 19.68750000136559208, 0.000000000000000000 ) ) ;
#19457=ORIENTED_EDGE ( 'NONE', *, *, #13894, .F. ) ;
#19460=CARTESIAN_POINT ( 'NONE',  ( 1.975475456537005874E-15, -39.75000000000000000, 5.000000000000000000 ) ) ;
#19462=CARTESIAN_POINT ( 'NONE',  ( -2.229367062500000163, -58.47916666530106511, -3.861377020970580443 ) ) ;
#19464=CARTESIAN_POINT ( 'NONE',  ( 2.229367062500001939, 16.02083333469892779, 3.861377020970579999 ) ) ;
#19466=CARTESIAN_POINT ( 'NONE',  ( 9.457646018065525792E-16, -48.31249999863440081, 5.148502694627439702 ) ) ;
#19467=CARTESIAN_POINT ( 'NONE',  ( -2.500000000000000444, -8.041666663935481907, -4.330127018922193649 ) ) ;
#19468=CARTESIAN_POINT ( 'NONE',  ( 1.339745962155615144, -31.70534180126147916, 4.999999999999999112 ) ) ;
#19470=CARTESIAN_POINT ( 'NONE',  ( 0.000000000000000000, -120.0000000000000000, 0.000000000000000000 ) ) ;
#19471=CARTESIAN_POINT ( 'NONE',  ( 9.457646018065525792E-16, -106.0624999986343937, 5.148502694627439702 ) ) ;
#19472=CARTESIAN_POINT ( 'NONE',  ( -4.458734124999999437, -9.562499998634406140, 0.000000000000000000 ) ) ;
#19475=CARTESIAN_POINT ( 'NONE',  ( 4.458734124999999437, -96.81249999863440792, -5.460374474430324690E-16 ) ) ;
#19478=CARTESIAN_POINT ( 'NONE',  ( 4.458734124999998549, -97.97916666530105090, -2.574251347313721627 ) ) ;
#19480=CARTESIAN_POINT ( 'NONE',  ( 1.060575238724906964E-15, -49.62499999726880873, 5.773502691896257311 ) ) ;
#19482=( BOUNDED_CURVE ( )  B_SPLINE_CURVE ( 2, ( #22320, #37425, #17498, #21691, #47079, #32275, #51282, #56425, #36160 ),
 .UNSPECIFIED., .F., .F. ) 
 B_SPLINE_CURVE_WITH_KNOTS ( ( 3, 2, 2, 2, 3 ),
 ( 0.8160714285714285587, 0.8166666666666666519, 0.8178571428571428381, 0.8190476190476190244, 0.8196428571428571175 ),
 .UNSPECIFIED. ) 
 CURVE ( )  GEOMETRIC_REPRESENTATION_ITEM ( )  RATIONAL_B_SPLINE_CURVE ( ( 0.9330127018922194093, 0.9330127018922194093, 1.000000000000000000, 0.8660254037844387076, 1.000000000000000000, 0.8660254037844387076, 1.000000000000000000, 0.9330127018922194093, 0.9330127018922194093 ) ) 
 REPRESENTATION_ITEM ( '' )  );
#19485=CARTESIAN_POINT ( 'NONE',  ( 2.229367062499998831, -20.64583333196774007, -3.861377020970580887 ) ) ;
#19486=CARTESIAN_POINT ( 'NONE',  ( -4.458734124999999437, 9.437500001365593860, 0.000000000000000000 ) ) ;
#19487=CARTESIAN_POINT ( 'NONE',  ( -2.229367062500000163, -60.72916666530106511, -3.861377020970580443 ) ) ;
#19488=CARTESIAN_POINT ( 'NONE',  ( -6.972266317189433020E-16, -94.12499999726880162, -5.000000000000000000 ) ) ;
#19491=CARTESIAN_POINT ( 'NONE',  ( 5.000000000000000888, -7.583333333333330373, 2.886751345948126879 ) ) ;
#19496=CARTESIAN_POINT ( 'NONE',  ( 1.975475456537005874E-15, -66.62499999726881583, 5.000000000000000000 ) ) ;
#19497=CARTESIAN_POINT ( 'NONE',  ( 2.229367062499998831, -87.64583333196773651, -3.861377020970580887 ) ) ;
#19498=CARTESIAN_POINT ( 'NONE',  ( -2.229367062499996610, 20.60416666803225993, 3.861377020970582219 ) ) ;
#19503=CARTESIAN_POINT ( 'NONE',  ( -5.000000000000000000, -7.083333333333330373, -2.886751345948128211 ) ) ;
#19506=CARTESIAN_POINT ( 'NONE',  ( 5.000000000000000000, -74.50000000000000000, -6.123233995736766282E-16 ) ) ;
#19510=VERTEX_POINT ( 'NONE', #11680 ) ;
#19522=CARTESIAN_POINT ( 'NONE',  ( 1.975475456537005874E-15, -93.62499999726881583, 5.000000000000000000 ) ) ;
#19523=CARTESIAN_POINT ( 'NONE',  ( 2.229367062500001939, -58.22916666530107932, 3.861377020970579999 ) ) ;
#19525=DIRECTION ( 'NONE',  ( -0.000000000000000000, 1.000000000000000000, -0.000000000000000000 ) ) ;
#19532=CARTESIAN_POINT ( 'NONE',  ( -4.458734124999999437, -107.6458333319677365, -2.574251347313719407 ) ) ;
#19533=CARTESIAN_POINT ( 'NONE',  ( -5.000000000000000000, -68.95833333060214443, -2.886751345948128211 ) ) ;
#19534=EDGE_LOOP ( 'NONE', ( #27212, #10730, #21631, #37474 ) ) ;
#19538=CARTESIAN_POINT ( 'NONE',  ( -2.229367062499996610, -37.14583333196773651, 3.861377020970582219 ) ) ;
#19542=DIRECTION ( 'NONE',  ( -0.000000000000000000, 1.000000000000000000, -0.000000000000000000 ) ) ;
#19543=CARTESIAN_POINT ( 'NONE',  ( 9.457646018065525792E-16, -14.06249999863440259, 5.148502694627439702 ) ) ;
#19544=CARTESIAN_POINT ( 'NONE',  ( 4.458734124999998549, -98.97916666530105090, -2.574251347313721627 ) ) ;
#19547=CARTESIAN_POINT ( 'NONE',  ( 4.458734124999999437, -32.06249999863440792, -5.460374474430324690E-16 ) ) ;
#19551=CARTESIAN_POINT ( 'NONE',  ( 1.975475456537005874E-15, -17.75000000000000355, 5.000000000000000000 ) ) ;
#19554=CARTESIAN_POINT ( 'NONE',  ( 4.458734124999998549, 7.020833334698928674, -2.574251347313721627 ) ) ;
#19556=ORIENTED_EDGE ( 'NONE', *, *, #11474, .T. ) ;
#19559=CARTESIAN_POINT ( 'NONE',  ( -5.000000000000000000, -97.08333333333332860, -2.886751345948128211 ) ) ;
#19560=CARTESIAN_POINT ( 'NONE',  ( -2.229367062500000163, -29.47916666530107221, -3.861377020970580443 ) ) ;
#19561=CARTESIAN_POINT ( 'NONE',  ( -6.972266317189433020E-16, -95.25000000000000000, -5.000000000000000000 ) ) ;
#19562=CARTESIAN_POINT ( 'NONE',  ( 2.229367062500001939, -77.22916666530106511, 3.861377020970579999 ) ) ;
#19566=CARTESIAN_POINT ( 'NONE',  ( 9.457646018065525792E-16, -1.062499998634405696, 5.148502694627439702 ) ) ;
#19567=CARTESIAN_POINT ( 'NONE',  ( 4.458734125000001214, 27.85416666803225993, 2.574251347313718519 ) ) ;
#19568=CARTESIAN_POINT ( 'NONE',  ( -4.458734124999999437, -45.56249999863440081, 0.000000000000000000 ) ) ;
#19571=VERTEX_POINT ( 'NONE', #1113 ) ;
#19573=CARTESIAN_POINT ( 'NONE',  ( -4.458734124999999437, -69.39583333196773651, -2.574251347313719407 ) ) ;
#19574=CARTESIAN_POINT ( 'NONE',  ( -2.500000000000000444, -105.0416666639354730, -4.330127018922193649 ) ) ;
#19576=CARTESIAN_POINT ( 'NONE',  ( -5.000000000000000000, 9.999999999999998224, 0.000000000000000000 ) ) ;
#19577=CARTESIAN_POINT ( 'NONE',  ( 2.229367062500001939, -110.2291666653010651, 3.861377020970579999 ) ) ;
#19579=CARTESIAN_POINT ( 'NONE',  ( -4.999999999999999112, -59.91666666666665719, 2.886751345948131764 ) ) ;
#19580=DIRECTION ( 'NONE',  ( -0.000000000000000000, 1.000000000000000000, -0.000000000000000000 ) ) ;
#19582=VERTEX_POINT ( 'NONE', #20720 ) ;
#19584=( BOUNDED_CURVE ( )  B_SPLINE_CURVE ( 2, ( #50888, #45743, #10686, #16152, #6830, #31579, #46380, #50568, #35778 ),
 .UNSPECIFIED., .F., .F. ) 
 B_SPLINE_CURVE_WITH_KNOTS ( ( 3, 2, 2, 2, 3 ),
 ( 0.1839285714285714413, 0.1845238095238095344, 0.1857142857142857206, 0.1869047619047619069, 0.1875000000000000000 ),
 .UNSPECIFIED. ) 
 CURVE ( )  GEOMETRIC_REPRESENTATION_ITEM ( )  RATIONAL_B_SPLINE_CURVE ( ( 0.9330127018922194093, 0.9330127018922209636, 1.000000000000000000, 0.8660254037844387076, 1.000000000000000000, 0.8660254037844387076, 1.000000000000000000, 0.9330127018922194093, 0.9330127018922194093 ) ) 
 REPRESENTATION_ITEM ( '' )  );
#19585=CARTESIAN_POINT ( 'NONE',  ( -1.339745962155599601, 12.79465819873851906, -5.000000000000007994 ) ) ;
#19594=ORIENTED_EDGE ( 'NONE', *, *, #58893, .F. ) ;
#19595=CARTESIAN_POINT ( 'NONE',  ( 2.500000000000002220, 5.333333333333332149, 4.330127018922192761 ) ) ;
#19596=CARTESIAN_POINT ( 'NONE',  ( 6.123233995736766282E-16, -120.0000000000000000, -5.000000000000000000 ) ) ;
#19602=CARTESIAN_POINT ( 'NONE',  ( -4.458734124999998549, -39.47916666530107932, 2.574251347313722516 ) ) ;
#19611=EDGE_CURVE ( 'NONE', #7250, #23647, #16198, .T. ) ;
#19612=CARTESIAN_POINT ( 'NONE',  ( 4.458734124999999437, -87.06249999863439371, -5.460374474430324690E-16 ) ) ;
#19615=CARTESIAN_POINT ( 'NONE',  ( 5.000000000000000000, -19.29166666393548013, -2.886751345948130876 ) ) ;
#19616=CYLINDRICAL_SURFACE ( 'NONE', #28238, 5.000000000000000000 ) ;
#19618=CARTESIAN_POINT ( 'NONE',  ( 2.499999999999998668, -38.33333333333332860, -4.330127018922193649 ) ) ;
#19621=CARTESIAN_POINT ( 'NONE',  ( -4.458734124999998549, 0.7708333346989267865, 2.574251347313722516 ) ) ;
#19622=CARTESIAN_POINT ( 'NONE',  ( 5.000000000000000888, -78.58333333333334281, 2.886751345948126879 ) ) ;
#19623=CARTESIAN_POINT ( 'NONE',  ( -2.229367062499996610, -15.39583333196773651, 3.861377020970582219 ) ) ;
#19628=CARTESIAN_POINT ( 'NONE',  ( 4.458734124999998549, 19.02083333469892779, -2.574251347313721627 ) ) ;
#19630=CARTESIAN_POINT ( 'NONE',  ( 4.458734124999998549, -97.72916666530105090, -2.574251347313721627 ) ) ;
#19631=FACE_OUTER_BOUND ( 'NONE', #11634, .T. ) ;
#19632=CARTESIAN_POINT ( 'NONE',  ( -2.229367062499996610, -14.14583333196774184, 3.861377020970582219 ) ) ;
#19633=CARTESIAN_POINT ( 'NONE',  ( -6.972266317189433020E-16, -99.12499999726880162, -5.000000000000000000 ) ) ;
#19637=CARTESIAN_POINT ( 'NONE',  ( 5.000000000000000888, -42.45833333060214443, 2.886751345948126879 ) ) ;
#19638=CARTESIAN_POINT ( 'NONE',  ( 1.975475456537005874E-15, -67.62499999726881583, 5.000000000000000000 ) ) ;
#19639=CARTESIAN_POINT ( 'NONE',  ( -3.152548672688508926E-16, 16.43750000136559564, -5.148502694627439702 ) ) ;
#19640=CARTESIAN_POINT ( 'NONE',  ( -1.339745962155613812, -95.20534180126148271, -5.000000000000000000 ) ) ;
#19643=CARTESIAN_POINT ( 'NONE',  ( -4.458734124999999437, -63.31249999863440792, 0.000000000000000000 ) ) ;
#19645=FACE_OUTER_BOUND ( 'NONE', #41957, .T. ) ;
#19646=CARTESIAN_POINT ( 'NONE',  ( -5.000000000000000000, 6.916666666666664298, -2.886751345948128211 ) ) ;
#19648=CARTESIAN_POINT ( 'NONE',  ( -4.999999999999998224, -59.79166666393547303, 2.886751345948131764 ) ) ;
#19649=CARTESIAN_POINT ( 'NONE',  ( -4.458734124999999437, -53.39583333196773651, -2.574251347313719407 ) ) ;
#19650=CARTESIAN_POINT ( 'NONE',  ( -5.000000000000000000, -88.87499999726880162, 0.000000000000000000 ) ) ;
#19651=CARTESIAN_POINT ( 'NONE',  ( 4.458734125000000326, -31.89583333196773651, 2.574251347313718519 ) ) ;
#19655=CARTESIAN_POINT ( 'NONE',  ( -2.500000000000000444, -40.16666666666667140, -4.330127018922193649 ) ) ;
#19656=CYLINDRICAL_SURFACE ( 'NONE', #32604, 5.000000000000000000 ) ;
#19657=LINE ( 'NONE', #39269, #20200 ) ;
#19658=ORIENTED_EDGE ( 'NONE', *, *, #5512, .F. ) ;
#19659=CARTESIAN_POINT ( 'NONE',  ( 2.229367062499998831, -103.6458333319677365, -3.861377020970580887 ) ) ;
#19660=CARTESIAN_POINT ( 'NONE',  ( 2.229367062500001939, 0.7708333346989268975, 3.861377020970579999 ) ) ;
#19661=CARTESIAN_POINT ( 'NONE',  ( 1.339745962155612702, -80.29465819873850307, -5.000000000000000000 ) ) ;
#19663=EDGE_CURVE ( 'NONE', #20660, #54885, #32545, .T. ) ;
#19667=EDGE_CURVE ( 'NONE', #52091, #26939, #21967, .T. ) ;
#19676=CARTESIAN_POINT ( 'NONE',  ( 4.458734124999998549, -22.97916666530107221, -2.574251347313721627 ) ) ;
#19684=( BOUNDED_CURVE ( )  B_SPLINE_CURVE ( 2, ( #5470, #39866, #25407, #45347, #1314, #15119, #993, #50498, #19936 ),
 .UNSPECIFIED., .F., .F. ) 
 B_SPLINE_CURVE_WITH_KNOTS ( ( 3, 2, 2, 2, 3 ),
 ( 0.5660714285714285587, 0.5666666666666666519, 0.5678571428571428381, 0.5690476190476190244, 0.5696428571428571175 ),
 .UNSPECIFIED. ) 
 CURVE ( )  GEOMETRIC_REPRESENTATION_ITEM ( )  RATIONAL_B_SPLINE_CURVE ( ( 0.9330127018922194093, 0.9330127018922194093, 1.000000000000000000, 0.8660254037844387076, 1.000000000000000000, 0.8660254037844387076, 1.000000000000000000, 0.9330127018922194093, 0.9330127018922194093 ) ) 
 REPRESENTATION_ITEM ( '' )  );
#19686=ORIENTED_EDGE ( 'NONE', *, *, #46687, .T. ) ;
#19687=CARTESIAN_POINT ( 'NONE',  ( -5.000000000000000000, -82.95833333060214443, -2.886751345948128211 ) ) ;
#19690=CARTESIAN_POINT ( 'NONE',  ( -3.152548672688508926E-16, -75.81249999863440792, -5.148502694627439702 ) ) ;
#19694=CARTESIAN_POINT ( 'NONE',  ( 5.000000000000000000, 12.58333333333333215, -2.886751345948130876 ) ) ;
#19695=CARTESIAN_POINT ( 'NONE',  ( 0.000000000000000000, -120.0000000000000000, 5.000000000000000000 ) ) ;
#19697=CARTESIAN_POINT ( 'NONE',  ( 9.457646018065525792E-16, 2.687500001365594304, 5.148502694627439702 ) ) ;
#19698=VERTEX_POINT ( 'NONE', #61867 ) ;
#19699=CARTESIAN_POINT ( 'NONE',  ( 6.123233995736766282E-16, -120.0000000000000000, -5.000000000000000000 ) ) ;
#19700=CARTESIAN_POINT ( 'NONE',  ( -2.480964764533239819E-13, -107.7500000000000000, 5.000000000000000000 ) ) ;
#19703=CARTESIAN_POINT ( 'NONE',  ( 5.000000000000000888, -47.45833333060215153, 2.886751345948126879 ) ) ;
#19706=CARTESIAN_POINT ( 'NONE',  ( -4.458734124999999437, -83.31249999863439371, 0.000000000000000000 ) ) ;
#19708=CARTESIAN_POINT ( 'NONE',  ( -3.152548672688508926E-16, 3.437500001365594748, -5.148502694627439702 ) ) ;
#19709=CARTESIAN_POINT ( 'NONE',  ( -2.499999999999996447, -85.83333333333332860, 4.330127018922195425 ) ) ;
#19711=CARTESIAN_POINT ( 'NONE',  ( -2.229367062500000163, -64.72916666530106511, -3.861377020970580443 ) ) ;
#19712=CARTESIAN_POINT ( 'NONE',  ( -2.499999999999996447, -25.70833333060214798, 4.330127018922195425 ) ) ;
#19713=CARTESIAN_POINT ( 'NONE',  ( 2.493747252781420335E-13, -42.25000000000000711, -5.000000000000000000 ) ) ;
#19714=CARTESIAN_POINT ( 'NONE',  ( 2.229367062500001939, 28.02083333469892779, 3.861377020970579999 ) ) ;
#19716=CARTESIAN_POINT ( 'NONE',  ( 2.500000000000002220, -3.541666663935478354, 4.330127018922192761 ) ) ;
#19717=CARTESIAN_POINT ( 'NONE',  ( 4.458734124999998549, -44.72916666530106511, -2.574251347313721627 ) ) ;
#19718=CARTESIAN_POINT ( 'NONE',  ( 9.457646018065525792E-16, -33.31249999863440792, 5.148502694627439702 ) ) ;
#19720=DIRECTION ( 'NONE',  ( -0.000000000000000000, 1.000000000000000000, -0.000000000000000000 ) ) ;
#19721=CARTESIAN_POINT ( 'NONE',  ( -5.000000000000000000, 24.91666666666666430, -2.886751345948128211 ) ) ;
#19724=CARTESIAN_POINT ( 'NONE',  ( -2.229367062500000163, -35.47916666530107221, -3.861377020970580443 ) ) ;
#19725=CARTESIAN_POINT ( 'NONE',  ( 2.499999999999998668, -74.20833333060214443, -4.330127018922193649 ) ) ;
#19728=CARTESIAN_POINT ( 'NONE',  ( 4.458734124999999437, -75.06249999863440792, -5.460374474430324690E-16 ) ) ;
#19731=( BOUNDED_CURVE ( )  B_SPLINE_CURVE ( 2, ( #61090, #52916, #17012, #31799, #60456, #62270, #12185, #32990, #8542 ),
 .UNSPECIFIED., .F., .F. ) 
 B_SPLINE_CURVE_WITH_KNOTS ( ( 3, 2, 2, 2, 3 ),
 ( 0.2053571428571428492, 0.2059523809523809423, 0.2071428571428571563, 0.2083333333333333426, 0.2089285714285714357 ),
 .UNSPECIFIED. ) 
 CURVE ( )  GEOMETRIC_REPRESENTATION_ITEM ( )  RATIONAL_B_SPLINE_CURVE ( ( 0.9330127018922194093, 0.9330127018922194093, 1.000000000000000000, 0.8660254037844387076, 1.000000000000000000, 0.8660254037844387076, 1.000000000000000000, 0.9330127018922194093, 0.9330127018922194093 ) ) 
 REPRESENTATION_ITEM ( '' )  );
#19733=CARTESIAN_POINT ( 'NONE',  ( 2.499999999999998668, -24.33333333333333215, -4.330127018922193649 ) ) ;
#19737=ORIENTED_EDGE ( 'NONE', *, *, #13729, .F. ) ;
#19739=( BOUNDED_CURVE ( )  B_SPLINE_CURVE ( 2, ( #14302, #4971, #19118, #53548, #9472, #39373, #59004, #14932, #34539 ),
 .UNSPECIFIED., .F., .F. ) 
 B_SPLINE_CURVE_WITH_KNOTS ( ( 3, 2, 2, 2, 3 ),
 ( 0.6910714285714285587, 0.6916666666666666519, 0.6928571428571428381, 0.6940476190476190244, 0.6946428571428571175 ),
 .UNSPECIFIED. ) 
 CURVE ( )  GEOMETRIC_REPRESENTATION_ITEM ( )  RATIONAL_B_SPLINE_CURVE ( ( 0.9330127018922194093, 0.9330127018922194093, 1.000000000000000000, 0.8660254037844387076, 1.000000000000000000, 0.8660254037844387076, 1.000000000000000000, 0.9330127018922194093, 0.9330127018922194093 ) ) 
 REPRESENTATION_ITEM ( '' )  );
#19740=CARTESIAN_POINT ( 'NONE',  ( 2.499999999999998668, 23.79166666939785202, -4.330127018922193649 ) ) ;
#19741=LINE ( 'NONE', #44820, #10365 ) ;
#19746=EDGE_CURVE ( 'NONE', #1698, #63455, #47991, .T. ) ;
#19748=CARTESIAN_POINT ( 'NONE',  ( 6.123233995736766282E-16, -120.0000000000000000, -5.000000000000000000 ) ) ;
#19750=CARTESIAN_POINT ( 'NONE',  ( -1.339745962155610925, 5.205341801261479162, 5.000000000000000000 ) ) ;
#19751=CARTESIAN_POINT ( 'NONE',  ( -2.229367062499996610, -19.14583333196774007, 3.861377020970582219 ) ) ;
#19764=EDGE_CURVE ( 'NONE', #14049, #57389, #17464, .T. ) ;
#19767=CARTESIAN_POINT ( 'NONE',  ( -2.500000000000000444, 10.83333333333333393, -4.330127018922193649 ) ) ;
#19773=CARTESIAN_POINT ( 'NONE',  ( 0.000000000000000000, -120.0000000000000000, 5.000000000000000000 ) ) ;
#19774=CARTESIAN_POINT ( 'NONE',  ( -4.458734124999998549, 17.77083333469892779, 2.574251347313722516 ) ) ;
#19775=CARTESIAN_POINT ( 'NONE',  ( -6.972266317189433020E-16, -10.12499999726881406, -5.000000000000000000 ) ) ;
#19776=VERTEX_POINT ( 'NONE', #39594 ) ;
#19782=CARTESIAN_POINT ( 'NONE',  ( -2.229367062500000163, -59.47916666530106511, -3.861377020970580443 ) ) ;
#19784=CARTESIAN_POINT ( 'NONE',  ( -2.229367062500000163, 15.52083333469892779, -3.861377020970580443 ) ) ;
#19786=CARTESIAN_POINT ( 'NONE',  ( 4.458734124999998549, -46.97916666530106511, -2.574251347313721627 ) ) ;
#19787=CARTESIAN_POINT ( 'NONE',  ( 5.000000000000000888, -11.45833333060214798, 2.886751345948126879 ) ) ;
#19788=CARTESIAN_POINT ( 'NONE',  ( 5.000000000000000888, -25.45833333060214443, 2.886751345948126879 ) ) ;
#19790=CARTESIAN_POINT ( 'NONE',  ( -6.972266317189433020E-16, -74.25000000000000000, -5.000000000000000000 ) ) ;
#19791=CARTESIAN_POINT ( 'NONE',  ( -4.458734124999999437, -109.3958333319677365, -2.574251347313719407 ) ) ;
#19792=CARTESIAN_POINT ( 'NONE',  ( 2.229367062500001939, -9.229166665301075767, 3.861377020970579999 ) ) ;
#19794=CARTESIAN_POINT ( 'NONE',  ( 4.458734125000001214, -98.89583333196775072, 2.574251347313718519 ) ) ;
#19796=CARTESIAN_POINT ( 'NONE',  ( 4.458734124999999437, -95.06249999863440792, -5.460374474430324690E-16 ) ) ;
#19798=CARTESIAN_POINT ( 'NONE',  ( -5.000000000000000000, -56.95833333060214443, -2.886751345948128211 ) ) ;
#19799=CARTESIAN_POINT ( 'NONE',  ( 1.339745962155612702, -5.294658198738519950, -5.000000000000000000 ) ) ;
#19802=CARTESIAN_POINT ( 'NONE',  ( 2.229367062500001939, -17.97916666530106866, 3.861377020970579999 ) ) ;
#19803=CARTESIAN_POINT ( 'NONE',  ( -4.458734124999998549, 7.520833334698926009, 2.574251347313722516 ) ) ;
#19804=CARTESIAN_POINT ( 'NONE',  ( -2.229367062499996610, -58.39583333196773651, 3.861377020970582219 ) ) ;
#19809=CARTESIAN_POINT ( 'NONE',  ( -5.000000000000000000, -4.999999999999997335, 0.000000000000000000 ) ) ;
#19810=ORIENTED_EDGE ( 'NONE', *, *, #7146, .F. ) ;
#19813=CARTESIAN_POINT ( 'NONE',  ( -6.972266317189433020E-16, -9.250000000000000000, -5.000000000000000000 ) ) ;
#19815=CARTESIAN_POINT ( 'NONE',  ( 4.458734125000001214, -82.89583333196772230, 2.574251347313718519 ) ) ;
#19816=CARTESIAN_POINT ( 'NONE',  ( 2.229367062500001939, 19.77083333469892779, 3.861377020970579999 ) ) ;
#19818=CARTESIAN_POINT ( 'NONE',  ( -5.000000000000000000, -88.87499999726880162, 0.000000000000000000 ) ) ;
#19820=CARTESIAN_POINT ( 'NONE',  ( 5.000000000000000000, 20.62500000273118772, -6.123233995736766282E-16 ) ) ;
#19822=CARTESIAN_POINT ( 'NONE',  ( -5.000000000000000000, -78.08333333333332860, -2.886751345948128211 ) ) ;
#19827=CARTESIAN_POINT ( 'NONE',  ( -5.000000000000000000, -104.0833333333333428, -2.886751345948128211 ) ) ;
#19832=ORIENTED_EDGE ( 'NONE', *, *, #31168, .T. ) ;
#19839=CARTESIAN_POINT ( 'NONE',  ( 9.457646018065525792E-16, -56.31249999863440081, 5.148502694627439702 ) ) ;
#19842=ORIENTED_EDGE ( 'NONE', *, *, #59431, .T. ) ;
#19845=CARTESIAN_POINT ( 'NONE',  ( 0.000000000000000000, -120.0000000000000000, 0.000000000000000000 ) ) ;
#19846=ORIENTED_EDGE ( 'NONE', *, *, #26810, .T. ) ;
#19849=CARTESIAN_POINT ( 'NONE',  ( -4.458734124999999437, -105.5624999986344221, 0.000000000000000000 ) ) ;
#19854=CARTESIAN_POINT ( 'NONE',  ( -2.229367062500000163, -38.47916666530107221, -3.861377020970580443 ) ) ;
#19858=CARTESIAN_POINT ( 'NONE',  ( 4.458734124999999437, -11.81249999863440081, -5.460374474430324690E-16 ) ) ;
#19859=( BOUNDED_CURVE ( )  B_SPLINE_CURVE ( 2, ( #9186, #52935, #52320, #43273, #13069, #62913, #17591, #42963, #18826 ),
 .UNSPECIFIED., .F., .F. ) 
 B_SPLINE_CURVE_WITH_KNOTS ( ( 3, 2, 2, 2, 3 ),
 ( 0.3017857142857142683, 0.3023809523809523614, 0.3035714285714285476, 0.3047619047619047894, 0.3053571428571428825 ),
 .UNSPECIFIED. ) 
 CURVE ( )  GEOMETRIC_REPRESENTATION_ITEM ( )  RATIONAL_B_SPLINE_CURVE ( ( 0.9330127018922194093, 0.9330127018922194093, 1.000000000000000000, 0.8660254037844387076, 1.000000000000000000, 0.8660254037844387076, 1.000000000000000000, 0.9330127018922194093, 0.9330127018922194093 ) ) 
 REPRESENTATION_ITEM ( '' )  );
#19860=CARTESIAN_POINT ( 'NONE',  ( -5.000000000000000000, -101.0833333333333286, -2.886751345948128211 ) ) ;
#19863=CARTESIAN_POINT ( 'NONE',  ( -3.152548672688508926E-16, -33.81249999863440792, -5.148502694627439702 ) ) ;
#19864=CARTESIAN_POINT ( 'NONE',  ( 2.500000000000002220, 5.458333336064518981, 4.330127018922192761 ) ) ;
#19870=CARTESIAN_POINT ( 'NONE',  ( 0.000000000000000000, -120.0000000000000000, 0.000000000000000000 ) ) ;
#19871=CARTESIAN_POINT ( 'NONE',  ( 2.229367062500001939, 5.770833334698927786, 3.861377020970579999 ) ) ;
#19873=CARTESIAN_POINT ( 'NONE',  ( 0.000000000000000000, -120.0000000000000000, 5.000000000000000000 ) ) ;
#19874=CARTESIAN_POINT ( 'NONE',  ( 2.500000000000002220, 2.333333333333333037, 4.330127018922192761 ) ) ;
#19875=CARTESIAN_POINT ( 'NONE',  ( -4.999999999999999112, -95.91666666666664298, 2.886751345948131764 ) ) ;
#19876=CARTESIAN_POINT ( 'NONE',  ( -2.229367062500000163, -28.47916666530107221, -3.861377020970580443 ) ) ;
#19878=CARTESIAN_POINT ( 'NONE',  ( 2.229367062500001939, -81.22916666530106511, 3.861377020970579999 ) ) ;
#19883=CARTESIAN_POINT ( 'NONE',  ( 2.229367062500001939, -0.9791666653010712151, 3.861377020970579999 ) ) ;
#19884=CARTESIAN_POINT ( 'NONE',  ( 4.458734124999998549, 21.02083333469892779, -2.574251347313721627 ) ) ;
#19885=CARTESIAN_POINT ( 'NONE',  ( -4.458734124999999437, -42.56249999863440081, 0.000000000000000000 ) ) ;
#19889=CARTESIAN_POINT ( 'NONE',  ( -3.152548672688508926E-16, -67.56249999863440792, -5.148502694627439702 ) ) ;
#19890=CARTESIAN_POINT ( 'NONE',  ( -2.499999999999996447, -105.7083333306021444, 4.330127018922195425 ) ) ;
#19892=CARTESIAN_POINT ( 'NONE',  ( 1.339745962155612702, -58.16965819600732601, -5.000000000000000000 ) ) ;
#19893=CARTESIAN_POINT ( 'NONE',  ( 0.000000000000000000, -120.0000000000000000, 0.000000000000000000 ) ) ;
#19895=CARTESIAN_POINT ( 'NONE',  ( -4.999999999999999112, -56.91666666666667140, 2.886751345948131764 ) ) ;
#19896=CARTESIAN_POINT ( 'NONE',  ( 1.975475456537005874E-15, -31.62499999726880873, 5.000000000000000000 ) ) ;
#19899=CARTESIAN_POINT ( 'NONE',  ( -6.972266317189433020E-16, -27.24999999999999645, -5.000000000000000000 ) ) ;
#19908=CARTESIAN_POINT ( 'NONE',  ( -4.999999999999998224, -23.91666666666666785, 2.886751345948131764 ) ) ;
#19911=ORIENTED_EDGE ( 'NONE', *, *, #37272, .F. ) ;
#19915=CARTESIAN_POINT ( 'NONE',  ( 2.229367062499998831, -39.89583333196773651, -3.861377020970580887 ) ) ;
#19916=CARTESIAN_POINT ( 'NONE',  ( 2.499999999999998668, -68.20833333060214443, -4.330127018922193649 ) ) ;
#19922=AXIS2_PLACEMENT_3D ( 'NONE', #5955, #42179, #40352 ) ;
#19925=CARTESIAN_POINT ( 'NONE',  ( -4.458734124999999437, -90.56249999863440792, 0.000000000000000000 ) ) ;
#19926=DIRECTION ( 'NONE',  ( -0.000000000000000000, 1.000000000000000000, -0.000000000000000000 ) ) ;
#19927=ORIENTED_EDGE ( 'NONE', *, *, #43975, .T. ) ;
#19928=CARTESIAN_POINT ( 'NONE',  ( 5.000000000000000888, -19.45833333060214798, 2.886751345948126879 ) ) ;
#19933=CARTESIAN_POINT ( 'NONE',  ( 5.000000000000000888, -38.58333333333332149, 2.886751345948126879 ) ) ;
#19935=CARTESIAN_POINT ( 'NONE',  ( -2.229367062499996610, 1.854166668032262377, 3.861377020970582219 ) ) ;
#19936=CARTESIAN_POINT ( 'NONE',  ( 1.975475456537005874E-15, -50.62499999726881583, 5.000000000000000000 ) ) ;
#19937=CARTESIAN_POINT ( 'NONE',  ( 9.457646018065525792E-16, -15.31249999863440436, 5.148502694627439702 ) ) ;
#19940=LINE ( 'NONE', #34742, #55198 ) ;
#19942=CARTESIAN_POINT ( 'NONE',  ( 4.458734125000000326, 20.85416666803226349, 2.574251347313718519 ) ) ;
#19944=CARTESIAN_POINT ( 'NONE',  ( 2.229367062499998831, -99.64583333196773651, -3.861377020970580887 ) ) ;
#19945=CARTESIAN_POINT ( 'NONE',  ( -2.499999999999996447, -33.70833333060213732, 4.330127018922195425 ) ) ;
#19947=CARTESIAN_POINT ( 'NONE',  ( 0.000000000000000000, -120.0000000000000000, 5.000000000000000000 ) ) ;
#19948=CARTESIAN_POINT ( 'NONE',  ( -3.152548672688508926E-16, -12.56249999863440081, -5.148502694627439702 ) ) ;
#19949=EDGE_CURVE ( 'NONE', #63218, #44248, #60626, .T. ) ;
#19952=CARTESIAN_POINT ( 'NONE',  ( -4.999999999999998224, -87.91666666666667140, 2.886751345948131764 ) ) ;
#19953=CARTESIAN_POINT ( 'NONE',  ( -4.999999999999999112, -40.79166666393548724, 2.886751345948131764 ) ) ;
#19955=CARTESIAN_POINT ( 'NONE',  ( -3.152548672688508926E-16, 11.43750000136559564, -5.148502694627439702 ) ) ;
#19956=CARTESIAN_POINT ( 'NONE',  ( -5.000000000000000000, -8.874999997268814056, 0.000000000000000000 ) ) ;
#19959=CARTESIAN_POINT ( 'NONE',  ( -4.458734124999999437, -61.39583333196774362, -2.574251347313719407 ) ) ;
#19962=( BOUNDED_CURVE ( )  B_SPLINE_CURVE ( 2, ( #11639, #31260, #36736, #56367, #59922, #15845, #37995, #37057, #27081, #52789, #32213, #32855, #18052, #56684, #12600, #57315, #27388, #42812, #3285, #46696, #7785, #52161, #51842, #13232, #42496, #47021, #38309, #52484, #37365, #32532, #2970, #31905, #51534, #22587, #2644, #17439, #57627, #42184, #7471, #17748, #22263, #61824, #56996, #12910, #8417, #41863, #8104, #27708, #47335, #61510, #28020, #22901, #47639, #23522, #62133, #8722, #37673, #3594, #62454, #23199, #18374, #13556, #33174, #28335, #47950, #3903, #12290, #43123, #62763, #18683, #5476, #33793, #49218, #5158, #49535, #54037, #29908, #18990, #14796, #29587, #28, #23833, #57937, #19309, #9035, #24778, #53724, #9975, #44382, #44699, #48893, #4519, #24144, #44062, #33479, #58558, #39238, #342, #38924, #43436, #15124, #38605, #4837, #19942, #43747, #39554, #34408, #59196, #34745, #63391, #53410, #54372, #20273, #28955, #28646, #9655, #48578, #25091, #10299, #9341, #63080, #664, #58238, #13855, #53100, #19628, #48261, #58864, #4219, #29264, #14166, #14478, #24457, #34099, #25413, #26369, #10932, #50819, #45671, #10611, #16084, #1629, #40207, #11570, #15454, #26693, #35071, #45353, #35708, #11252, #50173, #30547, #55336, #45031, #999, #5795, #20916, #40836, #36024, #30877, #55970, #59843, #50504, #36339, #16723, #46310, #2267, #6756, #40519, #45987, #1320, #6125, #41151, #6447, #31190, #54689, #1953, #20603, #30224, #11882, #15768, #60163, #60481, #49849, #60797, #26056, #31500, #51145, #35385, #21230, #7080, #16407, #55004, #55656, #21554, #25739, #39874, #59519, #46949, #42103, #36980, #32137, #47566, #61117, #46625, #8345, #18300, #21871, #17676, #27006, #57555, #51772, #2571, #27320, #3208, #41788, #17041, #8646, #27943, #22828, #17358, #13158, #36658, #3517, #22187, #56286, #62377, #61432, #42418, #27635, #56608, #12525, #62061, #7716, #52413, #12839, #12213, #2896, #22509, #47871, #17974, #52090, #61749, #41466, #37598, #37291, #56920, #32458, #31830, #51461, #8028, #7399, #47263, #23128, #57242, #32780, #42732, #37923, #13481, #33097, #52712, #28259, #23450, #63011, #14093, #9271, #13784, #63635, #62693, #19554, #15051, #38243, #44309, #48193, #58485, #34343, #33719, #39168, #24386, #29508, #24705, #273, #33406, #3832, #19871, #63312, #57862, #34669, #43364, #58793, #14723, #59121, #53969, #39485, #28572, #43987, #9899, #9588, #54288, #29194, #43055, #18617, #49140, #19234, #5084, #10227, #29832, #53021, #8962, #4146, #23765, #18919, #38533, #48820, #58161, #53338, #28887, #48508, #4446, #24075, #43671, #38850, #14410, #34032, #53653, #4757, #49778, #6054, #6682, #59766, #49465, #60407, #6372, #20198, #40444, #40759, #59445, #5404, #60085, #1551, #30801, #15692, #35312, #35631, #25021, #50099, #50430, #21154, #10858, #34998, #26289, #11806, #44631, #11178, #39801, #54932, #30473, #35955, #20841, #1874, #45911, #21479, #591, #20527, #15375, #1241, #40125, #41077, #11500, #44962, #54613, #60722, #16007, #16333, #55260, #50738, #25664, #10537, #30149, #45275, #5724, #55581, #25978, #16645, #25338, #31116, #45593, #36268, #55893, #922, #7640, #42347, #23057, #37849, #22434, #27244, #62301, #21798, #51061, #32063, #47186, #22113, #46869, #16965, #36576, #61042, #12452, #32386, #27554, #2812, #47489, #61985, #31752, #42030, #27869, #8267, #57482, #31423, #17905, #51699, #37526, #57167, #12763, #26938, #56206, #52011, #61671, #22749, #17604, #13082, #7953, #56846, #36901, #3129, #41393, #32703, #37220, #3442, #52332, #51385, #42662, #12130, #7005, #18223, #26614, #46231, #2194, #7327, #46554, #2497, #41706, #61354, #17277, #56531, #52637, #38163, #63554, #9812, #13400, #9198, #18543, #43288, #57787, #18839, #19792, #39399, #43904, #14016, #19472, #38457, #4069, #14642, #28810, #4678, #28182, #39086, #13707, #47798, #53887, #33329, #33955, #53576, #23377, #34259, #58085, #29422, #49053, #52948, #63236, #5002, #53263, #8885, #14334, #43593, #28498, #33021, #9503, #33643, #48429, #48117, #8571, #58716, #3755, #23688, #24621, #44228, #42977, #4373, #62924, #193, #23989, #19150, #38767, #58406, #62619, #29112, #48735, #24300, #5326, #55177, #54204, #20441, #44550, #16253, #21398, #59035, #20759, #49382, #44874, #25256, #45513, #30394, #11416, #35873, #24944, #14965, #55501, #54851, #506, #6599, #34912, #21077, #54535, #20114, #31035, #50017, #50344, #5970, #60327, #15614, #39718, #34573, #40040, #10142, #30721, #10784, #11096, #6291, #45834, #50660, #26214, #1160, #29749, #35232, #25896, #1796, #59355, #25580, #45193, #15290, #10455, #30070, #59682, #1475, #49699, #5643, #836, #40365, #60005, #15929, #35552, #40682, #17198, #57086, #7876, #41315, #36825, #37455, #17833, #2420, #61276, #56128, #60645, #16568, #16883, #31343, #46157, #22674, #51311, #36190, #46473, #13005, #7249, #2119, #22032, #22354, #55811, #36499, #26861, #41623, #50985, #37148, #11727, #56772, #52252, #6925, #32625, #21720, #31991, #27479, #56456, #12378, #47107, #51625, #8192, #27794, #26534, #41003, #47419, #7559, #60963, #3371, #12051, #32305, #51934, #31675, #12692, #27171, #46788, #61596, #3056, #2734, #41951, #17530, #42273, #61913, #58333, #18766, #19076, #14259, #9742, #58647, #63480, #19400, #23299, #18145, #24228, #28732, #42899, #33881, #62227, #53812, #13325, #42589, #23616, #38696, #32945, #29347, #52878, #28428, #62547, #43212, #43834, #33260, #22988, #53501, #43521, #57404, #13945, #9431, #52569, #48981, #37773, #29041, #62853, #48664, #48042, #13639, #39018, #38393, #4605, #8502, #14567, #47728, #28112, #34189, #18468, #63165, #48358, #3685, #38088, #3993, #57714, #8813, #58017, #9124, #33572, #53191, #4302, #23919, #35164, #44474, #30963, #5894, #10389, #49939, #24549, #433, #15213, #29999, #14886, #25501, #20693, #49631, #54128, #25826, #4930, #44153, #30318, #58960, #54463, #34839, #55096, #39966, #21006, #45441, #34493, #124, #1404, #759, #10066, #59282, #60255, #30643, #20039, #29679, #40611, #59612, #59936, #15544, #6213, #25181, #49309, #19718, #5567, #39327, #40298, #20367, #1085, #15858, #55422, #16174, #35799, #5251, #24873, #11340, #10711, #39643, #35480, #44795, #54780, #45120, #11022, #50265, #21955, #60882, #41235, #26780, #36113, #55736, #16492, #8659, #16807, #50588, #62391, #7482, #21323, #41551, #42748, #60567, #6528, #61202, #3531, #6848, #45761, #38254, #37937, #31919, #46079, #11652, #27095, #13495, #31272, #1715, #28272, #26462, #47580, #56380, #50906, #2037, #51546, #21642, #18312, #17124, #40924, #36427, #56055, #13799, #23140, #51235, #57570, #26142, #33111, #11971, #7171, #31601, #46398, #2347, #36750, #12304, #52727, #47887, #3845, #23465, #43068, #62706, #18632, #57875, #59134, #54301, #63330, #63024, #33420, #29847, #29208, #23777, #44644, #9285, #24718, #44322, #25034, #29521, #5417, #58178, #53984, #5100, #39180, #10243, #58805, #53038, #4773, #286, #48833, #49155, #19885, #20214, #604, #49479, #39816, #33732, #28586, #34682, #14737, #53350, #39498, #8976, #59457, #48207, #38863, #9600, #24400, #43379, #4160, #19248, #58499, #28901, #53667, #18931, #43684, #38547, #15070, #9913, #14107, #44002, #48521, #4462, #24089, #63649, #14423, #34045, #19568, #34354, #6066, #16657, #11192, #6696, #30162, #41089, #40138, #49791, #55906, #35324, #35967, #21167, #59782, #15707, #60420, #30489, #45925, #6386, #5737, #36282, #55273, #54945, #16345, #45610, #10872, #41405, #55593, #40460, #35647, #50111, #35014, #54628, #25680, #25355, #20541, #60736, #45288, #10552, #20857, #51079, #1254, #60099, #16020, #11512, #44973, #30814, #50446, #25991, #938, #31128, #1566, #50751, #26625, #40774, #11817, #26302, #1888, #21491, #31436, #7017, #46245, #2206, #21810, #15389, #7652, #23067, #36588, #22125, #47503, #57493, #61057, #56857, #2507, #33033, #27255, #41717, #2826, #42358, #16977, #46882, #47198, #56224, #61684, #61997, #13096, #22445, #46567, #18235, #23390, #12145, #22762, #51397, #42042, #17615, #3453, #32397, #13412, #37860, #26950, #31764, #32074, #7339, #12775, #51711, #52649, #42672, #56544, #61368, #8584, #52023, #52343, #7967, #62311, #37231, #17289, #36914, #27565, #12463, #32715, #3142, #28194, #17917, #47809, #37539, #8277, #57178, #27881, #3766, #53900, #34588, #49396, #33969, #19164, #10157, #33344, #62632, #43606, #58729, #52959, #38781, #28512, #48130, #8897, #24003, #43920, #39101, #58420, #59051, #9825, #43301, #14347, #39413, #19804, #5340, #42990, #29436, #63249, #49069, #4384, #44242, #53589, #34274, #57798, #5016, #4081, #13719, #14979, #62937, #63567, #48749, #23704, #18851, #24313, #58099, #24635, #9519, #38472, #14028, #33657, #53275, #19487, #29126, #9210, #18554, #14655, #38176, #4691, #206, #54219, #29762, #28823, #48444, #11430, #59698, #35886, #30735, #59370, #1174, #55516, #25271, #60339, #521, #11739, #20131, #30408, #20774, #60020, #35246, #15629, #40379, #10470, #30083, #54547, #5990, #25908, #21090, #15943, #41015, #31048, #35565, #16267, #34926, #44563, #55189, #40694, #44892, #39731, #31357, #50672, #6304, #20456, #49713, #45526, #11110, #6613, #50356, #26226, #1487, #45846, #1808, #5658, #852, #21412, #40054, #60659, #16583, #15304, #54865, #10796, #50998, #36202, #25595, #55824, #24958, #50032, #45208, #7888, #57101, #3069, #46169, #46487, #60975, #12063, #52267, #17211, #2131, #12390, #21733, #22686, #27807, #22044, #22366, #61608, #36838, #56468, #56785, #41329, #7572, #51949, #42286, #18158, #16896, #47432, #51323, #17542, #37468, #32004, #61926, #27492, #32637, #3384, #51638, #2435, #23001, #32957, #41637, #36512, #41966, #61289, #17845, #13019, #62239, #8204, #42602, #31688, #47121, #37786, #12704, #57416, #32318, #13337, #6938, #26549, #56143, #7261, #27185, #46800, #26874, #37162, #2747, #28440, #48992, #14899, #23628, #3697, #4311, #43223, #44167, #14578, #48054, #57725, #4939, #23931, #43844, #43532, #53823, #9135, #18479, #52582, #63176, #53513, #39029, #48369, #134, #38101, #58656, #62864, #63490, #58344, #23311, #28743, #19415, #19728, #58972, #19087, #38706, #39341, #42912, #8513, #14272, #18776, #38403, #33891, #13651, #33271, #52890, #33582, #9442, #48675, #29051, #24562, #34200, #8826, #4615, #28123, #29359, #47741, #62560, #9752, #4007, #58026, #13955, #24240, #53201, #39656, #55109, #25514, #25836, #1096, #60267, #11034, #59948, #39978, #30657, #44485, #35812, #15556, #11352, #55436, #5264, #30013, #59293, #60584, #50279, #35176, #45452, #20705, #6224, #10401, #35491, #21017, #1418, #44809, #16185, #10078, #15224, #40624, #30974, #34508, #59624, #49320, #50598, #6540, #49641, #49955, #45132, #771, #20378, #40310, #29689, #54794, #15871, #26153, #10722, #20052, #45772, #30329, #1730, #24884, #34853, #21334, #5907, #446, #40934, #54474, #54139, #5578, #25194, #31930, #7497, #26791, #46411, #2667, #55747, #17139, #61534, #32241, #41562, #2049, #42523, #16504, #41888, #6860, #2360, #21969, #2995, #51558, #32562, #57024, #46089, #36125, #12939, #12319, #26475, #27732, #56067, #7812, #27414, #8129, #52184, #27109, #47045, #46722, #17770, #36763, #21657, #11664, #61213, #31283, #51870, #22289, #12625, #22612, #3308, #47360, #22929, #50918, #16818, #41248, #42207, #60894, #36437, #17466, #56391, #11986, #31612, #51248, #37088, #61853, #7183, #56706, #37389, #52814, #3619, #3932, #33818, #13580, #62160, #19018, #38631, #42840, #43149, #28982, #9371, #19337, #18080, #58274, #23551, #14193, #47978, #33199, #48605, #62789, #53438, #32881, #4544, #23226, #52509, #24169, #9061, #28357, #4243, #8444, #43773, #18708, #63419, #37703, #18401, #53129, #57341, #38333, #38022, #23858, #28671, #57654, #13257, #28047, #57962, #48291, #47667, #62483, #8752, #13883, #33511, #43461, #63107, #3505, #41457, #42408, #26997, #3199, #61738, #26685, #32127, #22817, #47557, #62367, #46938, #51763, #31491, #61423, #7707, #27311, #2562, #46616, #2886, #61107, #17031, #21862, #36969, #56910, #52081, #22499, #8335, #62050, #56277, #42095, #52403, #32769, #17667, #8019, #12201, #51135, #42723, #17965, #37282, #51453, #36646, #12829, #32449, #47254, #27624, #37589, #57232, #13149, #17347, #27934, #2258, #23119, #7390, #18291, #55961, #46301, #22176, #31820, #11873, #7070, #56598, #41777, #12516, #9576, #13774, #38837, #24376, #34022, #48184, #63622, #13472, #62685, #19544, #4137, #33088, #43353, #52702, #53643, #58782, #53010, #53329, #28878, #23758, #63001, #24065, #8637, #38524, #19224, #29183, #18909, #23443, #14712, #18606, #48499, #4748, #58152, #48810, #58474, #39157, #34330, #14082, #33397, #53956, #262, #8952, #28248, #9263, #28563, #29497, #9888, #33710, #43045, #49129, #38234, #14400, #43977, #43661, #5072, #3822, #37914, #24692, #4436, #47862, #44298, #63302, #57544, #57854, #47287, #32808, #42762, #18326, #57583, #28286, #43388, #47898, #22537, #13510, #23475, #8986, #37950, #33743, #8057, #28598, #57267, #33430, #3854, #56945, #62404, #53049, #14117, #28910, #33126, #9294, #61774, #27972, #52743, #8672, #52437, #13185, #43078, #27659, #3237, #52113, #3545, #62716, #18641, #38263, #38559, #48216, #22853, #57885, #18941, #42133, #13811, #4171, #42444, #17701, #48533, #23786, #63033, #18003, #62086, #58188, #53360, #37315, #12866, #32484, #37626, #8371, #47593, #23153, #14432, #49169, #44985, #25365, #4784, #54315, #5747, #44330, #24411, #5426, #34690, #44012, #30501, #25043, #29532, #24728, #19577, #24099, #43695, #63660, #58508 ),
 .UNSPECIFIED., .F., .F. ) 
 B_SPLINE_CURVE_WITH_KNOTS ( ( 3, 2, 2, 2, 2, 2, 2, 2, 2, 2, 2, 2, 2, 2, 2, 2, 2, 2, 2, 2, 2, 2, 2, 2, 2, 2, 2, 2, 2, 2, 2, 2, 2, 2, 2, 2, 2, 2, 2, 2, 2, 2, 2, 2, 2, 2, 2, 2, 2, 2, 2, 2, 2, 2, 2, 2, 2, 2, 2, 2, 2, 2, 2, 2, 2, 2, 2, 2, 2, 2, 2, 2, 2, 2, 2, 2, 2, 2, 2, 2, 2, 2, 2, 2, 2, 2, 2, 2, 2, 2, 2, 2, 2, 2, 2, 2, 2, 2, 2, 2, 2, 2, 2, 2, 2, 2, 2, 2, 2, 2, 2, 2, 2, 2, 2, 2, 2, 2, 2, 2, 2, 2, 2, 2, 2, 2, 2, 2, 2, 2, 2, 2, 2, 2, 2, 2, 2, 2, 2, 2, 2, 2, 2, 2, 2, 2, 2, 2, 2, 2, 2, 2, 2, 2, 2, 2, 2, 2, 2, 2, 2, 2, 2, 2, 2, 2, 2, 2, 2, 2, 2, 2, 2, 2, 2, 2, 2, 2, 2, 2, 2, 2, 2, 2, 2, 2, 2, 2, 2, 2, 2, 2, 2, 2, 2, 2, 2, 2, 2, 2, 2, 2, 2, 2, 2, 2, 2, 2, 2, 2, 2, 2, 2, 2, 2, 2, 2, 2, 2, 2, 2, 2, 2, 2, 2, 2, 2, 2, 2, 2, 2, 2, 2, 2, 2, 2, 2, 2, 2, 2, 2, 2, 2, 2, 2, 2, 2, 2, 2, 2, 2, 2, 2, 2, 2, 2, 2, 2, 2, 2, 2, 2, 2, 2, 2, 2, 2, 2, 2, 2, 2, 2, 2, 2, 2, 2, 2, 2, 2, 2, 2, 2, 2, 2, 2, 2, 2, 2, 2, 2, 2, 2, 2, 2, 2, 2, 2, 2, 2, 2, 2, 2, 2, 2, 2, 2, 2, 2, 2, 2, 2, 2, 2, 2, 2, 2, 2, 2, 2, 2, 2, 2, 2, 2, 2, 2, 2, 2, 2, 2, 2, 2, 2, 2, 2, 2, 2, 2, 2, 2, 2, 2, 2, 2, 2, 2, 2, 2, 2, 2, 2, 2, 2, 2, 2, 2, 2, 2, 2, 2, 2, 2, 2, 2, 2, 2, 2, 2, 2, 2, 2, 2, 2, 2, 2, 2, 2, 2, 2, 2, 2, 2, 2, 2, 2, 2, 2, 2, 2, 2, 2, 2, 2, 2, 2, 2, 2, 2, 2, 2, 2, 2, 2, 2, 2, 2, 2, 2, 2, 2, 2, 2, 2, 2, 2, 2, 2, 2, 2, 2, 2, 2, 2, 2, 2, 2, 2, 2, 2, 2, 2, 2, 2, 2, 2, 2, 2, 2, 2, 2, 2, 2, 2, 2, 2, 2, 2, 2, 2, 2, 2, 2, 2, 2, 2, 2, 2, 2, 2, 2, 2, 2, 2, 2, 2, 2, 2, 2, 2, 2, 2, 2, 2, 2, 2, 2, 2, 2, 2, 2, 2, 2, 2, 2, 2, 2, 2, 2, 2, 2, 2, 2, 2, 2, 2, 2, 2, 2, 2, 2, 2, 2, 2, 2, 2, 2, 2, 2, 2, 2, 2, 2, 2, 2, 2, 2, 2, 2, 2, 2, 2, 2, 2, 2, 2, 2, 2, 2, 2, 2, 2, 2, 2, 2, 2, 2, 2, 2, 2, 2, 2, 2, 2, 2, 2, 2, 2, 2, 2, 2, 2, 2, 2, 2, 2, 2, 2, 2, 2, 2, 2, 2, 2, 2, 2, 2, 2, 2, 2, 2, 2, 2, 2, 2, 2, 2, 2, 2, 2, 2, 2, 2, 2, 2, 2, 2, 2, 2, 2, 2, 2, 2, 2, 2, 2, 2, 2, 2, 2, 2, 2, 2, 2, 2, 2, 2, 2, 2, 2, 2, 2, 2, 2, 2, 2, 2, 2, 2, 2, 2, 2, 2, 2, 2, 2, 2, 2, 2, 2, 2, 2, 2, 2, 2, 2, 2, 2, 2, 2, 2, 2, 2, 2, 2, 2, 2, 2, 2, 2, 2, 2, 2, 2, 2, 2, 2, 2, 2, 2, 2, 2, 2, 2, 2, 2, 2, 2, 2, 2, 2, 2, 2, 2, 2, 2, 2, 2, 2, 2, 2, 2, 2, 2, 2, 2, 2, 2, 2, 2, 2, 2, 2, 2, 2, 2, 2, 2, 2, 2, 2, 2, 2, 2, 2, 2, 2, 2, 2, 2, 2, 2, 2, 2, 2, 2, 2, 2, 2, 2, 2, 2, 2, 2, 2, 2, 2, 2, 2, 2, 2, 2, 2, 2, 2, 2, 2, 2, 2, 2, 2, 2, 2, 2, 2, 2, 2, 2, 2, 2, 2, 2, 2, 2, 2, 2, 2, 2, 2, 2, 2, 2, 2, 2, 2, 2, 2, 2, 2, 2, 2, 2, 2, 2, 2, 2, 2, 2, 2, 2, 2, 2, 2, 2, 2, 2, 2, 2, 2, 2, 2, 2, 2, 2, 2, 2, 2, 2, 2, 2, 2, 2, 2, 2, 2, 2, 2, 2, 2, 2, 2, 2, 2, 2, 2, 2, 2, 2, 2, 2, 2, 2, 2, 2, 2, 2, 2, 2, 2, 2, 2, 2, 2, 2, 2, 2, 2, 2, 2, 2, 2, 3 ),
 ( 0.000000000000000000, 0.001190476190476190584, 0.002380952380952381167, 0.003571428571428571317, 0.004761904761904762334, 0.005952380952380952051, 0.007142857142857142634, 0.008333333333333333218, 0.009523809523809524669, 0.01071428571428571438, 0.01190476190476190410, 0.01309523809523809555, 0.01428571428571428527, 0.01547619047619047672, 0.01666666666666666644, 0.01785714285714285615, 0.01904761904761904934, 0.02023809523809523905, 0.02142857142857142877, 0.02261904761904761849, 0.02380952380952380820, 0.02500000000000000139, 0.02619047619047619110, 0.02738095238095238082, 0.02857142857142857054, 0.02976190476190476025, 0.03095238095238095344, 0.03214285714285713969, 0.03333333333333333287, 0.03452380952380952606, 0.03571428571428571230, 0.03690476190476190549, 0.03809523809523809867, 0.03928571428571428492, 0.04047619047619047811, 0.04166666666666666435, 0.04285714285714285754, 0.04404761904761905073, 0.04523809523809523697, 0.04642857142857143016, 0.04761904761904761640, 0.04880952380952380959, 0.05000000000000000278, 0.05119047619047618902, 0.05238095238095238221, 0.05357142857142856845, 0.05476190476190476164, 0.05595238095238095483, 0.05714285714285714107, 0.05833333333333333426, 0.05952380952380952051, 0.06071428571428571369, 0.06190476190476190688, 0.06309523809523809312, 0.06428571428571427937, 0.06547619047619047949, 0.06666666666666666574, 0.06785714285714285199, 0.06904761904761905211, 0.07023809523809523836, 0.07142857142857142461, 0.07261904761904762473, 0.07380952380952381098, 0.07499999999999999722, 0.07619047619047619735, 0.07738095238095238360, 0.07857142857142856984, 0.07976190476190475609, 0.08095238095238095621, 0.08214285714285714246, 0.08333333333333332871, 0.08452380952380952883, 0.08571428571428571508, 0.08690476190476190133, 0.08809523809523810145, 0.08928571428571428770, 0.09047619047619047394, 0.09166666666666666019, 0.09285714285714286031, 0.09404761904761904656, 0.09523809523809523281, 0.09642857142857143293, 0.09761904761904761918, 0.09880952380952380543, 0.1000000000000000056, 0.1011904761904761918, 0.1023809523809523780, 0.1035714285714285782, 0.1047619047619047644, 0.1059523809523809507, 0.1071428571428571369, 0.1083333333333333370, 0.1095238095238095233, 0.1107142857142857095, 0.1119047619047619097, 0.1130952380952380959, 0.1142857142857142821, 0.1154761904761904823, 0.1166666666666666685, 0.1178571428571428548, 0.1190476190476190410, 0.1202380952380952411, 0.1214285714285714274, 0.1226190476190476136, 0.1238095238095238138, 0.1250000000000000000, 0.1261904761904761862, 0.1273809523809523725, 0.1285714285714285587, 0.1297619047619047727, 0.1309523809523809590, 0.1321428571428571452, 0.1333333333333333315, 0.1345238095238095177, 0.1357142857142857040, 0.1369047619047619180, 0.1380952380952381042, 0.1392857142857142905, 0.1404761904761904767, 0.1416666666666666630, 0.1428571428571428492, 0.1440476190476190355, 0.1452380952380952495, 0.1464285714285714357, 0.1476190476190476220, 0.1488095238095238082, 0.1499999999999999944, 0.1511904761904761807, 0.1523809523809523947, 0.1535714285714285809, 0.1547619047619047672, 0.1559523809523809534, 0.1571428571428571397, 0.1583333333333333259, 0.1595238095238095122, 0.1607142857142857262, 0.1619047619047619124, 0.1630952380952380987, 0.1642857142857142849, 0.1654761904761904712, 0.1666666666666666574, 0.1678571428571428437, 0.1690476190476190577, 0.1702380952380952439, 0.1714285714285714302, 0.1726190476190476164, 0.1738095238095238027, 0.1749999999999999889, 0.1761904761904762029, 0.1773809523809523891, 0.1785714285714285754, 0.1797619047619047616, 0.1809523809523809479, 0.1821428571428571341, 0.1833333333333333204, 0.1845238095238095344, 0.1857142857142857206, 0.1869047619047619069, 0.1880952380952380931, 0.1892857142857142794, 0.1904761904761904656, 0.1916666666666666796, 0.1928571428571428659, 0.1940476190476190521, 0.1952380952380952384, 0.1964285714285714246, 0.1976190476190476109, 0.1988095238095237971, 0.2000000000000000111, 0.2011904761904761973, 0.2023809523809523836, 0.2035714285714285698, 0.2047619047619047561, 0.2059523809523809423, 0.2071428571428571563, 0.2083333333333333426, 0.2095238095238095288, 0.2107142857142857151, 0.2119047619047619013, 0.2130952380952380876, 0.2142857142857142738, 0.2154761904761904878, 0.2166666666666666741, 0.2178571428571428603, 0.2190476190476190466, 0.2202380952380952328, 0.2214285714285714191, 0.2226190476190476053, 0.2238095238095238193, 0.2250000000000000056, 0.2261904761904761918, 0.2273809523809523780, 0.2285714285714285643, 0.2297619047619047505, 0.2309523809523809645, 0.2321428571428571508, 0.2333333333333333370, 0.2345238095238095233, 0.2357142857142857095, 0.2369047619047618958, 0.2380952380952380820, 0.2392857142857142960, 0.2404761904761904823, 0.2416666666666666685, 0.2428571428571428548, 0.2440476190476190410, 0.2452380952380952273, 0.2464285714285714413, 0.2476190476190476275, 0.2488095238095238138, 0.2500000000000000000, 0.2511904761904761862, 0.2523809523809523725, 0.2535714285714285587, 0.2547619047619047450, 0.2559523809523809312, 0.2571428571428571175, 0.2583333333333333592, 0.2595238095238095455, 0.2607142857142857317, 0.2619047619047619180, 0.2630952380952381042, 0.2642857142857142905, 0.2654761904761904767, 0.2666666666666666630, 0.2678571428571428492, 0.2690476190476190355, 0.2702380952380952217, 0.2714285714285714080, 0.2726190476190475942, 0.2738095238095238360, 0.2750000000000000222, 0.2761904761904762085, 0.2773809523809523947, 0.2785714285714285809, 0.2797619047619047672, 0.2809523809523809534, 0.2821428571428571397, 0.2833333333333333259, 0.2845238095238095122, 0.2857142857142856984, 0.2869047619047618847, 0.2880952380952380709, 0.2892857142857143127, 0.2904761904761904989, 0.2916666666666666852, 0.2928571428571428714, 0.2940476190476190577, 0.2952380952380952439, 0.2964285714285714302, 0.2976190476190476164, 0.2988095238095238027, 0.2999999999999999889, 0.3011904761904761751, 0.3023809523809523614, 0.3035714285714285476, 0.3047619047619047894, 0.3059523809523809756, 0.3071428571428571619, 0.3083333333333333481, 0.3095238095238095344, 0.3107142857142857206, 0.3119047619047619069, 0.3130952380952380931, 0.3142857142857142794, 0.3154761904761904656, 0.3166666666666666519, 0.3178571428571428381, 0.3190476190476190244, 0.3202380952380952106, 0.3214285714285714524, 0.3226190476190476386, 0.3238095238095238249, 0.3250000000000000111, 0.3261904761904761973, 0.3273809523809523836, 0.3285714285714285698, 0.3297619047619047561, 0.3309523809523809423, 0.3321428571428571286, 0.3333333333333333148, 0.3345238095238095011, 0.3357142857142856873, 0.3369047619047619291, 0.3380952380952381153, 0.3392857142857143016, 0.3404761904761904878, 0.3416666666666666741, 0.3428571428571428603, 0.3440476190476190466, 0.3452380952380952328, 0.3464285714285714191, 0.3476190476190476053, 0.3488095238095237915, 0.3499999999999999778, 0.3511904761904761640, 0.3523809523809524058, 0.3535714285714285920, 0.3547619047619047783, 0.3559523809523809645, 0.3571428571428571508, 0.3583333333333333370, 0.3595238095238095233, 0.3607142857142857095, 0.3619047619047618958, 0.3630952380952380820, 0.3642857142857142683, 0.3654761904761904545, 0.3666666666666666408, 0.3678571428571428825, 0.3690476190476190688, 0.3702380952380952550, 0.3714285714285714413, 0.3726190476190476275, 0.3738095238095238138, 0.3750000000000000000, 0.3761904761904761862, 0.3773809523809523725, 0.3785714285714285587, 0.3797619047619047450, 0.3809523809523809312, 0.3821428571428571175, 0.3833333333333333592, 0.3845238095238095455, 0.3857142857142857317, 0.3869047619047619180, 0.3880952380952381042, 0.3892857142857142905, 0.3904761904761904767, 0.3916666666666666630, 0.3928571428571428492, 0.3940476190476190355, 0.3952380952380952217, 0.3964285714285714080, 0.3976190476190475942, 0.3988095238095238360, 0.4000000000000000222, 0.4011904761904762085, 0.4023809523809523947, 0.4035714285714285809, 0.4047619047619047672, 0.4059523809523809534, 0.4071428571428571397, 0.4083333333333333259, 0.4095238095238095122, 0.4107142857142856984, 0.4119047619047618847, 0.4130952380952380709, 0.4142857142857143127, 0.4154761904761904989, 0.4166666666666666852, 0.4178571428571428714, 0.4190476190476190577, 0.4202380952380952439, 0.4214285714285714302, 0.4226190476190476164, 0.4238095238095238027, 0.4249999999999999889, 0.4261904761904761751, 0.4273809523809523614, 0.4285714285714285476, 0.4297619047619047894, 0.4309523809523809756, 0.4321428571428571619, 0.4333333333333333481, 0.4345238095238095344, 0.4357142857142857206, 0.4369047619047619069, 0.4380952380952380931, 0.4392857142857142794, 0.4404761904761904656, 0.4416666666666666519, 0.4428571428571428381, 0.4440476190476190244, 0.4452380952380952106, 0.4464285714285714524, 0.4476190476190476386, 0.4488095238095238249, 0.4500000000000000111, 0.4511904761904761973, 0.4523809523809523836, 0.4535714285714285698, 0.4547619047619047561, 0.4559523809523809423, 0.4571428571428571286, 0.4583333333333333148, 0.4595238095238095011, 0.4607142857142856873, 0.4619047619047619291, 0.4630952380952381153, 0.4642857142857143016, 0.4654761904761904878, 0.4666666666666666741, 0.4678571428571428603, 0.4690476190476190466, 0.4702380952380952328, 0.4714285714285714191, 0.4726190476190476053, 0.4738095238095237915, 0.4749999999999999778, 0.4761904761904761640, 0.4773809523809524058, 0.4785714285714285920, 0.4797619047619047783, 0.4809523809523809645, 0.4821428571428571508, 0.4833333333333333370, 0.4845238095238095233, 0.4857142857142857095, 0.4869047619047618958, 0.4880952380952380820, 0.4892857142857142683, 0.4904761904761904545, 0.4916666666666666408, 0.4928571428571428825, 0.4940476190476190688, 0.4952380952380952550, 0.4964285714285714413, 0.4976190476190476275, 0.4988095238095238138, 0.5000000000000000000, 0.5011904761904761862, 0.5023809523809523725, 0.5035714285714285587, 0.5047619047619047450, 0.5059523809523809312, 0.5071428571428571175, 0.5083333333333333037, 0.5095238095238094900, 0.5107142857142856762, 0.5119047619047618625, 0.5130952380952380487, 0.5142857142857142350, 0.5154761904761904212, 0.5166666666666667185, 0.5178571428571429047, 0.5190476190476190910, 0.5202380952380952772, 0.5214285714285714635, 0.5226190476190476497, 0.5238095238095238360, 0.5250000000000000222, 0.5261904761904762085, 0.5273809523809523947, 0.5285714285714285809, 0.5297619047619047672, 0.5309523809523809534, 0.5321428571428571397, 0.5333333333333333259, 0.5345238095238095122, 0.5357142857142856984, 0.5369047619047618847, 0.5380952380952380709, 0.5392857142857142572, 0.5404761904761904434, 0.5416666666666666297, 0.5428571428571428159, 0.5440476190476190022, 0.5452380952380951884, 0.5464285714285713746, 0.5476190476190476719, 0.5488095238095238582, 0.5500000000000000444, 0.5511904761904762307, 0.5523809523809524169, 0.5535714285714286031, 0.5547619047619047894, 0.5559523809523809756, 0.5571428571428571619, 0.5583333333333333481, 0.5595238095238095344, 0.5607142857142857206, 0.5619047619047619069, 0.5630952380952380931, 0.5642857142857142794, 0.5654761904761904656, 0.5666666666666666519, 0.5678571428571428381, 0.5690476190476190244, 0.5702380952380952106, 0.5714285714285713969, 0.5726190476190475831, 0.5738095238095237693, 0.5749999999999999556, 0.5761904761904761418, 0.5773809523809523281, 0.5785714285714286254, 0.5797619047619048116, 0.5809523809523809978, 0.5821428571428571841, 0.5833333333333333703, 0.5845238095238095566, 0.5857142857142857428, 0.5869047619047619291, 0.5880952380952381153, 0.5892857142857143016, 0.5904761904761904878, 0.5916666666666666741, 0.5928571428571428603, 0.5940476190476190466, 0.5952380952380952328, 0.5964285714285714191, 0.5976190476190476053, 0.5988095238095237915, 0.5999999999999999778, 0.6011904761904761640, 0.6023809523809523503, 0.6035714285714285365, 0.6047619047619047228, 0.6059523809523809090, 0.6071428571428570953, 0.6083333333333332815, 0.6095238095238095788, 0.6107142857142857650, 0.6119047619047619513, 0.6130952380952381375, 0.6142857142857143238, 0.6154761904761905100, 0.6166666666666666963, 0.6178571428571428825, 0.6190476190476190688, 0.6202380952380952550, 0.6214285714285714413, 0.6226190476190476275, 0.6238095238095238138, 0.6250000000000000000, 0.6261904761904761862, 0.6273809523809523725, 0.6285714285714285587, 0.6297619047619047450, 0.6309523809523809312, 0.6321428571428571175, 0.6333333333333333037, 0.6345238095238094900, 0.6357142857142856762, 0.6369047619047618625, 0.6380952380952380487, 0.6392857142857142350, 0.6404761904761904212, 0.6416666666666667185, 0.6428571428571429047, 0.6440476190476190910, 0.6452380952380952772, 0.6464285714285714635, 0.6476190476190476497, 0.6488095238095238360, 0.6500000000000000222, 0.6511904761904762085, 0.6523809523809523947, 0.6535714285714285809, 0.6547619047619047672, 0.6559523809523809534, 0.6571428571428571397, 0.6583333333333333259, 0.6595238095238095122, 0.6607142857142856984, 0.6619047619047618847, 0.6630952380952380709, 0.6642857142857142572, 0.6654761904761904434, 0.6666666666666666297, 0.6678571428571428159, 0.6690476190476190022, 0.6702380952380951884, 0.6714285714285713746, 0.6726190476190476719, 0.6738095238095238582, 0.6750000000000000444, 0.6761904761904762307, 0.6773809523809524169, 0.6785714285714286031, 0.6797619047619047894, 0.6809523809523809756, 0.6821428571428571619, 0.6833333333333333481, 0.6845238095238095344, 0.6857142857142857206, 0.6869047619047619069, 0.6880952380952380931, 0.6892857142857142794, 0.6904761904761904656, 0.6916666666666666519, 0.6928571428571428381, 0.6940476190476190244, 0.6952380952380952106, 0.6964285714285713969, 0.6976190476190475831, 0.6988095238095237693, 0.6999999999999999556, 0.7011904761904761418, 0.7023809523809523281, 0.7035714285714286254, 0.7047619047619048116, 0.7059523809523809978, 0.7071428571428571841, 0.7083333333333333703, 0.7095238095238095566, 0.7107142857142857428, 0.7119047619047619291, 0.7130952380952381153, 0.7142857142857143016, 0.7154761904761904878, 0.7166666666666666741, 0.7178571428571428603, 0.7190476190476190466, 0.7202380952380952328, 0.7214285714285714191, 0.7226190476190476053, 0.7238095238095237915, 0.7249999999999999778, 0.7261904761904761640, 0.7273809523809523503, 0.7285714285714285365, 0.7297619047619047228, 0.7309523809523809090, 0.7321428571428570953, 0.7333333333333332815, 0.7345238095238095788, 0.7357142857142857650, 0.7369047619047619513, 0.7380952380952381375, 0.7392857142857143238, 0.7404761904761905100, 0.7416666666666666963, 0.7428571428571428825, 0.7440476190476190688, 0.7452380952380952550, 0.7464285714285714413, 0.7476190476190476275, 0.7488095238095238138, 0.7500000000000000000, 0.7511904761904761862, 0.7523809523809523725, 0.7535714285714285587, 0.7547619047619047450, 0.7559523809523809312, 0.7571428571428571175, 0.7583333333333333037, 0.7595238095238094900, 0.7607142857142856762, 0.7619047619047618625, 0.7630952380952380487, 0.7642857142857142350, 0.7654761904761904212, 0.7666666666666667185, 0.7678571428571429047, 0.7690476190476190910, 0.7702380952380952772, 0.7714285714285714635, 0.7726190476190476497, 0.7738095238095238360, 0.7750000000000000222, 0.7761904761904762085, 0.7773809523809523947, 0.7785714285714285809, 0.7797619047619047672, 0.7809523809523809534, 0.7821428571428571397, 0.7833333333333333259, 0.7845238095238095122, 0.7857142857142856984, 0.7869047619047618847, 0.7880952380952380709, 0.7892857142857142572, 0.7904761904761904434, 0.7916666666666666297, 0.7928571428571428159, 0.7940476190476190022, 0.7952380952380951884, 0.7964285714285713746, 0.7976190476190476719, 0.7988095238095238582, 0.8000000000000000444, 0.8011904761904762307, 0.8023809523809524169, 0.8035714285714286031, 0.8047619047619047894, 0.8059523809523809756, 0.8071428571428571619, 0.8083333333333333481, 0.8095238095238095344, 0.8107142857142857206, 0.8119047619047619069, 0.8130952380952380931, 0.8142857142857142794, 0.8154761904761904656, 0.8166666666666666519, 0.8178571428571428381, 0.8190476190476190244, 0.8202380952380952106, 0.8214285714285713969, 0.8226190476190475831, 0.8238095238095237693, 0.8249999999999999556, 0.8261904761904761418, 0.8273809523809523281, 0.8285714285714286254, 0.8297619047619048116, 0.8309523809523809978, 0.8321428571428571841, 0.8333333333333333703, 0.8345238095238095566, 0.8357142857142857428, 0.8369047619047619291, 0.8380952380952381153, 0.8392857142857143016, 0.8404761904761904878, 0.8416666666666666741, 0.8428571428571428603, 0.8440476190476190466, 0.8452380952380952328, 0.8464285714285714191, 0.8476190476190476053, 0.8488095238095237915, 0.8499999999999999778, 0.8511904761904761640, 0.8523809523809523503, 0.8535714285714285365, 0.8547619047619047228, 0.8559523809523809090, 0.8571428571428570953, 0.8583333333333332815, 0.8595238095238095788, 0.8607142857142857650, 0.8619047619047619513, 0.8630952380952381375, 0.8642857142857143238, 0.8654761904761905100, 0.8666666666666666963, 0.8678571428571428825, 0.8690476190476190688, 0.8702380952380952550, 0.8714285714285714413, 0.8726190476190476275, 0.8738095238095238138, 0.8750000000000000000, 0.8761904761904761862, 0.8773809523809523725, 0.8785714285714285587, 0.8797619047619047450, 0.8809523809523809312, 0.8821428571428571175, 0.8833333333333333037, 0.8845238095238094900, 0.8857142857142856762, 0.8869047619047618625, 0.8880952380952380487, 0.8892857142857142350, 0.8904761904761904212, 0.8916666666666667185, 0.8928571428571429047, 0.8940476190476190910, 0.8952380952380952772, 0.8964285714285714635, 0.8976190476190476497, 0.8988095238095238360, 0.9000000000000000222, 0.9011904761904762085, 0.9023809523809523947, 0.9035714285714285809, 0.9047619047619047672, 0.9059523809523809534, 0.9071428571428571397, 0.9083333333333333259, 0.9095238095238095122, 0.9107142857142856984, 0.9119047619047618847, 0.9130952380952380709, 0.9142857142857142572, 0.9154761904761904434, 0.9166666666666666297, 0.9178571428571428159, 0.9190476190476190022, 0.9202380952380951884, 0.9214285714285713746, 0.9226190476190476719, 0.9238095238095238582, 0.9250000000000000444, 0.9261904761904762307, 0.9273809523809524169, 0.9285714285714286031, 0.9297619047619047894, 0.9309523809523809756, 0.9321428571428571619, 0.9333333333333333481, 0.9345238095238095344, 0.9357142857142857206, 0.9369047619047619069, 0.9380952380952380931, 0.9392857142857142794, 0.9404761904761904656, 0.9416666666666666519, 0.9428571428571428381, 0.9440476190476190244, 0.9452380952380952106, 0.9464285714285713969, 0.9476190476190475831, 0.9488095238095237693, 0.9499999999999999556, 0.9511904761904761418, 0.9523809523809523281, 0.9535714285714286254, 0.9547619047619048116, 0.9559523809523809978, 0.9571428571428571841, 0.9583333333333333703, 0.9595238095238095566, 0.9607142857142857428, 0.9619047619047619291, 0.9630952380952381153, 0.9642857142857143016, 0.9654761904761904878, 0.9666666666666666741, 0.9678571428571428603, 0.9690476190476190466, 0.9702380952380952328, 0.9714285714285714191, 0.9726190476190476053, 0.9738095238095237915, 0.9749999999999999778, 0.9761904761904761640, 0.9773809523809523503, 0.9785714285714285365, 0.9797619047619047228, 0.9809523809523809090, 0.9821428571428570953, 0.9833333333333332815, 0.9845238095238095788, 0.9857142857142857650, 0.9869047619047619513, 0.9880952380952381375, 0.9892857142857143238, 0.9904761904761905100, 0.9916666666666666963, 0.9928571428571428825, 0.9940476190476190688, 0.9952380952380952550, 0.9964285714285714413, 0.9976190476190476275, 0.9988095238095238138, 1.000000000000000000 ),
 .UNSPECIFIED. ) 
 CURVE ( )  GEOMETRIC_REPRESENTATION_ITEM ( )  RATIONAL_B_SPLINE_CURVE ( ( 1.000000000000000000, 0.8660254037844387076, 1.000000000000000000, 0.8660254037844387076, 1.000000000000000000, 0.8660254037844387076, 1.000000000000000000, 0.8660254037844387076, 1.000000000000000000, 0.8660254037844387076, 1.000000000000000000, 0.8660254037844387076, 1.000000000000000000, 0.8660254037844387076, 1.000000000000000000, 0.8660254037844387076, 1.000000000000000000, 0.8660254037844387076, 1.000000000000000000, 0.8660254037844387076, 1.000000000000000000, 0.8660254037844387076, 1.000000000000000000, 0.8660254037844387076, 1.000000000000000000, 0.8660254037844387076, 1.000000000000000000, 0.8660254037844387076, 1.000000000000000000, 0.8660254037844387076, 1.000000000000000000, 0.8660254037844387076, 1.000000000000000000, 0.8660254037844387076, 1.000000000000000000, 0.8660254037844387076, 1.000000000000000000, 0.8660254037844387076, 1.000000000000000000, 0.8660254037844387076, 1.000000000000000000, 0.8660254037844387076, 1.000000000000000000, 0.8660254037844387076, 1.000000000000000000, 0.8660254037844387076, 1.000000000000000000, 0.8660254037844387076, 1.000000000000000000, 0.8660254037844387076, 1.000000000000000000, 0.8660254037844387076, 1.000000000000000000, 0.8660254037844387076, 1.000000000000000000, 0.8660254037844387076, 1.000000000000000000, 0.8660254037844387076, 1.000000000000000000, 0.8660254037844387076, 1.000000000000000000, 0.8660254037844387076, 1.000000000000000000, 0.8660254037844387076, 1.000000000000000000, 0.8660254037844387076, 1.000000000000000000, 0.8660254037844387076, 1.000000000000000000, 0.8660254037844387076, 1.000000000000000000, 0.8660254037844387076, 1.000000000000000000, 0.8660254037844387076, 1.000000000000000000, 0.8660254037844387076, 1.000000000000000000, 0.8660254037844387076, 1.000000000000000000, 0.8660254037844387076, 1.000000000000000000, 0.8660254037844387076, 1.000000000000000000, 0.8660254037844387076, 1.000000000000000000, 0.8660254037844387076, 1.000000000000000000, 0.8660254037844387076, 1.000000000000000000, 0.8660254037844387076, 1.000000000000000000, 0.8660254037844387076, 1.000000000000000000, 0.8660254037844387076, 1.000000000000000000, 0.8660254037844387076, 1.000000000000000000, 0.8660254037844387076, 1.000000000000000000, 0.8660254037844387076, 1.000000000000000000, 0.8660254037844387076, 1.000000000000000000, 0.8660254037844387076, 1.000000000000000000, 0.8660254037844387076, 1.000000000000000000, 0.8660254037844387076, 1.000000000000000000, 0.8660254037844387076, 1.000000000000000000, 0.8660254037844387076, 1.000000000000000000, 0.8660254037844387076, 1.000000000000000000, 0.8660254037844387076, 1.000000000000000000, 0.8660254037844387076, 1.000000000000000000, 0.8660254037844387076, 1.000000000000000000, 0.8660254037844387076, 1.000000000000000000, 0.8660254037844387076, 1.000000000000000000, 0.8660254037844387076, 1.000000000000000000, 0.8660254037844387076, 1.000000000000000000, 0.8660254037844387076, 1.000000000000000000, 0.8660254037844387076, 1.000000000000000000, 0.8660254037844387076, 1.000000000000000000, 0.8660254037844387076, 1.000000000000000000, 0.8660254037844387076, 1.000000000000000000, 0.8660254037844387076, 1.000000000000000000, 0.8660254037844387076, 1.000000000000000000, 0.8660254037844387076, 1.000000000000000000, 0.8660254037844387076, 1.000000000000000000, 0.8660254037844387076, 1.000000000000000000, 0.8660254037844387076, 1.000000000000000000, 0.8660254037844387076, 1.000000000000000000, 0.8660254037844387076, 1.000000000000000000, 0.8660254037844387076, 1.000000000000000000, 0.8660254037844387076, 1.000000000000000000, 0.8660254037844387076, 1.000000000000000000, 0.8660254037844387076, 1.000000000000000000, 0.8660254037844387076, 1.000000000000000000, 0.8660254037844387076, 1.000000000000000000, 0.8660254037844387076, 1.000000000000000000, 0.8660254037844387076, 1.000000000000000000, 0.8660254037844387076, 1.000000000000000000, 0.8660254037844387076, 1.000000000000000000, 0.8660254037844387076, 1.000000000000000000, 0.8660254037844387076, 1.000000000000000000, 0.8660254037844387076, 1.000000000000000000, 0.8660254037844387076, 1.000000000000000000, 0.8660254037844387076, 1.000000000000000000, 0.8660254037844387076, 1.000000000000000000, 0.8660254037844387076, 1.000000000000000000, 0.8660254037844387076, 1.000000000000000000, 0.8660254037844387076, 1.000000000000000000, 0.8660254037844387076, 1.000000000000000000, 0.8660254037844387076, 1.000000000000000000, 0.8660254037844387076, 1.000000000000000000, 0.8660254037844387076, 1.000000000000000000, 0.8660254037844387076, 1.000000000000000000, 0.8660254037844387076, 1.000000000000000000, 0.8660254037844387076, 1.000000000000000000, 0.8660254037844387076, 1.000000000000000000, 0.8660254037844387076, 1.000000000000000000, 0.8660254037844387076, 1.000000000000000000, 0.8660254037844387076, 1.000000000000000000, 0.8660254037844387076, 1.000000000000000000, 0.8660254037844387076, 1.000000000000000000, 0.8660254037844387076, 1.000000000000000000, 0.8660254037844387076, 1.000000000000000000, 0.8660254037844387076, 1.000000000000000000, 0.8660254037844387076, 1.000000000000000000, 0.8660254037844387076, 1.000000000000000000, 0.8660254037844387076, 1.000000000000000000, 0.8660254037844387076, 1.000000000000000000, 0.8660254037844387076, 1.000000000000000000, 0.8660254037844387076, 1.000000000000000000, 0.8660254037844387076, 1.000000000000000000, 0.8660254037844387076, 1.000000000000000000, 0.8660254037844387076, 1.000000000000000000, 0.8660254037844387076, 1.000000000000000000, 0.8660254037844387076, 1.000000000000000000, 0.8660254037844387076, 1.000000000000000000, 0.8660254037844387076, 1.000000000000000000, 0.8660254037844387076, 1.000000000000000000, 0.8660254037844387076, 1.000000000000000000, 0.8660254037844387076, 1.000000000000000000, 0.8660254037844387076, 1.000000000000000000, 0.8660254037844387076, 1.000000000000000000, 0.8660254037844387076, 1.000000000000000000, 0.8660254037844387076, 1.000000000000000000, 0.8660254037844387076, 1.000000000000000000, 0.8660254037844387076, 1.000000000000000000, 0.8660254037844387076, 1.000000000000000000, 0.8660254037844387076, 1.000000000000000000, 0.8660254037844387076, 1.000000000000000000, 0.8660254037844387076, 1.000000000000000000, 0.8660254037844387076, 1.000000000000000000, 0.8660254037844387076, 1.000000000000000000, 0.8660254037844387076, 1.000000000000000000, 0.8660254037844387076, 1.000000000000000000, 0.8660254037844387076, 1.000000000000000000, 0.8660254037844387076, 1.000000000000000000, 0.8660254037844387076, 1.000000000000000000, 0.8660254037844387076, 1.000000000000000000, 0.8660254037844387076, 1.000000000000000000, 0.8660254037844387076, 1.000000000000000000, 0.8660254037844387076, 1.000000000000000000, 0.8660254037844387076, 1.000000000000000000, 0.8660254037844387076, 1.000000000000000000, 0.8660254037844387076, 1.000000000000000000, 0.8660254037844387076, 1.000000000000000000, 0.8660254037844387076, 1.000000000000000000, 0.8660254037844387076, 1.000000000000000000, 0.8660254037844387076, 1.000000000000000000, 0.8660254037844387076, 1.000000000000000000, 0.8660254037844387076, 1.000000000000000000, 0.8660254037844387076, 1.000000000000000000, 0.8660254037844387076, 1.000000000000000000, 0.8660254037844387076, 1.000000000000000000, 0.8660254037844387076, 1.000000000000000000, 0.8660254037844387076, 1.000000000000000000, 0.8660254037844387076, 1.000000000000000000, 0.8660254037844387076, 1.000000000000000000, 0.8660254037844387076, 1.000000000000000000, 0.8660254037844387076, 1.000000000000000000, 0.8660254037844387076, 1.000000000000000000, 0.8660254037844387076, 1.000000000000000000, 0.8660254037844387076, 1.000000000000000000, 0.8660254037844387076, 1.000000000000000000, 0.8660254037844387076, 1.000000000000000000, 0.8660254037844387076, 1.000000000000000000, 0.8660254037844387076, 1.000000000000000000, 0.8660254037844387076, 1.000000000000000000, 0.8660254037844387076, 1.000000000000000000, 0.8660254037844387076, 1.000000000000000000, 0.8660254037844387076, 1.000000000000000000, 0.8660254037844387076, 1.000000000000000000, 0.8660254037844387076, 1.000000000000000000, 0.8660254037844387076, 1.000000000000000000, 0.8660254037844387076, 1.000000000000000000, 0.8660254037844387076, 1.000000000000000000, 0.8660254037844387076, 1.000000000000000000, 0.8660254037844387076, 1.000000000000000000, 0.8660254037844387076, 1.000000000000000000, 0.8660254037844387076, 1.000000000000000000, 0.8660254037844387076, 1.000000000000000000, 0.8660254037844387076, 1.000000000000000000, 0.8660254037844387076, 1.000000000000000000, 0.8660254037844387076, 1.000000000000000000, 0.8660254037844387076, 1.000000000000000000, 0.8660254037844387076, 1.000000000000000000, 0.8660254037844387076, 1.000000000000000000, 0.8660254037844387076, 1.000000000000000000, 0.8660254037844387076, 1.000000000000000000, 0.8660254037844387076, 1.000000000000000000, 0.8660254037844387076, 1.000000000000000000, 0.8660254037844387076, 1.000000000000000000, 0.8660254037844387076, 1.000000000000000000, 0.8660254037844387076, 1.000000000000000000, 0.8660254037844387076, 1.000000000000000000, 0.8660254037844387076, 1.000000000000000000, 0.8660254037844387076, 1.000000000000000000, 0.8660254037844387076, 1.000000000000000000, 0.8660254037844387076, 1.000000000000000000, 0.8660254037844387076, 1.000000000000000000, 0.8660254037844387076, 1.000000000000000000, 0.8660254037844387076, 1.000000000000000000, 0.8660254037844387076, 1.000000000000000000, 0.8660254037844387076, 1.000000000000000000, 0.8660254037844387076, 1.000000000000000000, 0.8660254037844387076, 1.000000000000000000, 0.8660254037844387076, 1.000000000000000000, 0.8660254037844387076, 1.000000000000000000, 0.8660254037844387076, 1.000000000000000000, 0.8660254037844387076, 1.000000000000000000, 0.8660254037844387076, 1.000000000000000000, 0.8660254037844387076, 1.000000000000000000, 0.8660254037844387076, 1.000000000000000000, 0.8660254037844387076, 1.000000000000000000, 0.8660254037844387076, 1.000000000000000000, 0.8660254037844387076, 1.000000000000000000, 0.8660254037844387076, 1.000000000000000000, 0.8660254037844387076, 1.000000000000000000, 0.8660254037844387076, 1.000000000000000000, 0.8660254037844387076, 1.000000000000000000, 0.8660254037844387076, 1.000000000000000000, 0.8660254037844387076, 1.000000000000000000, 0.8660254037844387076, 1.000000000000000000, 0.8660254037844387076, 1.000000000000000000, 0.8660254037844387076, 1.000000000000000000, 0.8660254037844387076, 1.000000000000000000, 0.8660254037844387076, 1.000000000000000000, 0.8660254037844387076, 1.000000000000000000, 0.8660254037844387076, 1.000000000000000000, 0.8660254037844387076, 1.000000000000000000, 0.8660254037844387076, 1.000000000000000000, 0.8660254037844387076, 1.000000000000000000, 0.8660254037844387076, 1.000000000000000000, 0.8660254037844387076, 1.000000000000000000, 0.8660254037844387076, 1.000000000000000000, 0.8660254037844387076, 1.000000000000000000, 0.8660254037844387076, 1.000000000000000000, 0.8660254037844387076, 1.000000000000000000, 0.8660254037844387076, 1.000000000000000000, 0.8660254037844387076, 1.000000000000000000, 0.8660254037844387076, 1.000000000000000000, 0.8660254037844387076, 1.000000000000000000, 0.8660254037844387076, 1.000000000000000000, 0.8660254037844387076, 1.000000000000000000, 0.8660254037844387076, 1.000000000000000000, 0.8660254037844387076, 1.000000000000000000, 0.8660254037844387076, 1.000000000000000000, 0.8660254037844387076, 1.000000000000000000, 0.8660254037844387076, 1.000000000000000000, 0.8660254037844387076, 1.000000000000000000, 0.8660254037844387076, 1.000000000000000000, 0.8660254037844387076, 1.000000000000000000, 0.8660254037844387076, 1.000000000000000000, 0.8660254037844387076, 1.000000000000000000, 0.8660254037844387076, 1.000000000000000000, 0.8660254037844387076, 1.000000000000000000, 0.8660254037844387076, 1.000000000000000000, 0.8660254037844387076, 1.000000000000000000, 0.8660254037844387076, 1.000000000000000000, 0.8660254037844387076, 1.000000000000000000, 0.8660254037844387076, 1.000000000000000000, 0.8660254037844387076, 1.000000000000000000, 0.8660254037844387076, 1.000000000000000000, 0.8660254037844387076, 1.000000000000000000, 0.8660254037844387076, 1.000000000000000000, 0.8660254037844387076, 1.000000000000000000, 0.8660254037844387076, 1.000000000000000000, 0.8660254037844387076, 1.000000000000000000, 0.8660254037844387076, 1.000000000000000000, 0.8660254037844387076, 1.000000000000000000, 0.8660254037844387076, 1.000000000000000000, 0.8660254037844387076, 1.000000000000000000, 0.8660254037844387076, 1.000000000000000000, 0.8660254037844387076, 1.000000000000000000, 0.8660254037844387076, 1.000000000000000000, 0.8660254037844387076, 1.000000000000000000, 0.8660254037844387076, 1.000000000000000000, 0.8660254037844387076, 1.000000000000000000, 0.8660254037844387076, 1.000000000000000000, 0.8660254037844387076, 1.000000000000000000, 0.8660254037844387076, 1.000000000000000000, 0.8660254037844387076, 1.000000000000000000, 0.8660254037844387076, 1.000000000000000000, 0.8660254037844387076, 1.000000000000000000, 0.8660254037844387076, 1.000000000000000000, 0.8660254037844387076, 1.000000000000000000, 0.8660254037844387076, 1.000000000000000000, 0.8660254037844387076, 1.000000000000000000, 0.8660254037844387076, 1.000000000000000000, 0.8660254037844387076, 1.000000000000000000, 0.8660254037844387076, 1.000000000000000000, 0.8660254037844387076, 1.000000000000000000, 0.8660254037844387076, 1.000000000000000000, 0.8660254037844387076, 1.000000000000000000, 0.8660254037844387076, 1.000000000000000000, 0.8660254037844387076, 1.000000000000000000, 0.8660254037844387076, 1.000000000000000000, 0.8660254037844387076, 1.000000000000000000, 0.8660254037844387076, 1.000000000000000000, 0.8660254037844387076, 1.000000000000000000, 0.8660254037844387076, 1.000000000000000000, 0.8660254037844387076, 1.000000000000000000, 0.8660254037844387076, 1.000000000000000000, 0.8660254037844387076, 1.000000000000000000, 0.8660254037844387076, 1.000000000000000000, 0.8660254037844387076, 1.000000000000000000, 0.8660254037844387076, 1.000000000000000000, 0.8660254037844387076, 1.000000000000000000, 0.8660254037844387076, 1.000000000000000000, 0.8660254037844387076, 1.000000000000000000, 0.8660254037844387076, 1.000000000000000000, 0.8660254037844387076, 1.000000000000000000, 0.8660254037844387076, 1.000000000000000000, 0.8660254037844387076, 1.000000000000000000, 0.8660254037844387076, 1.000000000000000000, 0.8660254037844387076, 1.000000000000000000, 0.8660254037844387076, 1.000000000000000000, 0.8660254037844387076, 1.000000000000000000, 0.8660254037844387076, 1.000000000000000000, 0.8660254037844387076, 1.000000000000000000, 0.8660254037844387076, 1.000000000000000000, 0.8660254037844387076, 1.000000000000000000, 0.8660254037844387076, 1.000000000000000000, 0.8660254037844387076, 1.000000000000000000, 0.8660254037844387076, 1.000000000000000000, 0.8660254037844387076, 1.000000000000000000, 0.8660254037844387076, 1.000000000000000000, 0.8660254037844387076, 1.000000000000000000, 0.8660254037844387076, 1.000000000000000000, 0.8660254037844387076, 1.000000000000000000, 0.8660254037844387076, 1.000000000000000000, 0.8660254037844387076, 1.000000000000000000, 0.8660254037844387076, 1.000000000000000000, 0.8660254037844387076, 1.000000000000000000, 0.8660254037844387076, 1.000000000000000000, 0.8660254037844387076, 1.000000000000000000, 0.8660254037844387076, 1.000000000000000000, 0.8660254037844387076, 1.000000000000000000, 0.8660254037844387076, 1.000000000000000000, 0.8660254037844387076, 1.000000000000000000, 0.8660254037844387076, 1.000000000000000000, 0.8660254037844387076, 1.000000000000000000, 0.8660254037844387076, 1.000000000000000000, 0.8660254037844387076, 1.000000000000000000, 0.8660254037844387076, 1.000000000000000000, 0.8660254037844387076, 1.000000000000000000, 0.8660254037844387076, 1.000000000000000000, 0.8660254037844387076, 1.000000000000000000, 0.8660254037844387076, 1.000000000000000000, 0.8660254037844387076, 1.000000000000000000, 0.8660254037844387076, 1.000000000000000000, 0.8660254037844387076, 1.000000000000000000, 0.8660254037844387076, 1.000000000000000000, 0.8660254037844387076, 1.000000000000000000, 0.8660254037844387076, 1.000000000000000000, 0.8660254037844387076, 1.000000000000000000, 0.8660254037844387076, 1.000000000000000000, 0.8660254037844387076, 1.000000000000000000, 0.8660254037844387076, 1.000000000000000000, 0.8660254037844387076, 1.000000000000000000, 0.8660254037844387076, 1.000000000000000000, 0.8660254037844387076, 1.000000000000000000, 0.8660254037844387076, 1.000000000000000000, 0.8660254037844387076, 1.000000000000000000, 0.8660254037844387076, 1.000000000000000000, 0.8660254037844387076, 1.000000000000000000, 0.8660254037844387076, 1.000000000000000000, 0.8660254037844387076, 1.000000000000000000, 0.8660254037844387076, 1.000000000000000000, 0.8660254037844387076, 1.000000000000000000, 0.8660254037844387076, 1.000000000000000000, 0.8660254037844387076, 1.000000000000000000, 0.8660254037844387076, 1.000000000000000000, 0.8660254037844387076, 1.000000000000000000, 0.8660254037844387076, 1.000000000000000000, 0.8660254037844387076, 1.000000000000000000, 0.8660254037844387076, 1.000000000000000000, 0.8660254037844387076, 1.000000000000000000, 0.8660254037844387076, 1.000000000000000000, 0.8660254037844387076, 1.000000000000000000, 0.8660254037844387076, 1.000000000000000000, 0.8660254037844387076, 1.000000000000000000, 0.8660254037844387076, 1.000000000000000000, 0.8660254037844387076, 1.000000000000000000, 0.8660254037844387076, 1.000000000000000000, 0.8660254037844387076, 1.000000000000000000, 0.8660254037844387076, 1.000000000000000000, 0.8660254037844387076, 1.000000000000000000, 0.8660254037844387076, 1.000000000000000000, 0.8660254037844387076, 1.000000000000000000, 0.8660254037844387076, 1.000000000000000000, 0.8660254037844387076, 1.000000000000000000, 0.8660254037844387076, 1.000000000000000000, 0.8660254037844387076, 1.000000000000000000, 0.8660254037844387076, 1.000000000000000000, 0.8660254037844387076, 1.000000000000000000, 0.8660254037844387076, 1.000000000000000000, 0.8660254037844387076, 1.000000000000000000, 0.8660254037844387076, 1.000000000000000000, 0.8660254037844387076, 1.000000000000000000, 0.8660254037844387076, 1.000000000000000000, 0.8660254037844387076, 1.000000000000000000, 0.8660254037844387076, 1.000000000000000000, 0.8660254037844387076, 1.000000000000000000, 0.8660254037844387076, 1.000000000000000000, 0.8660254037844387076, 1.000000000000000000, 0.8660254037844387076, 1.000000000000000000, 0.8660254037844387076, 1.000000000000000000, 0.8660254037844387076, 1.000000000000000000, 0.8660254037844387076, 1.000000000000000000, 0.8660254037844387076, 1.000000000000000000, 0.8660254037844387076, 1.000000000000000000, 0.8660254037844387076, 1.000000000000000000, 0.8660254037844387076, 1.000000000000000000, 0.8660254037844387076, 1.000000000000000000, 0.8660254037844387076, 1.000000000000000000, 0.8660254037844387076, 1.000000000000000000, 0.8660254037844387076, 1.000000000000000000, 0.8660254037844387076, 1.000000000000000000, 0.8660254037844387076, 1.000000000000000000, 0.8660254037844387076, 1.000000000000000000, 0.8660254037844387076, 1.000000000000000000, 0.8660254037844387076, 1.000000000000000000, 0.8660254037844387076, 1.000000000000000000, 0.8660254037844387076, 1.000000000000000000, 0.8660254037844387076, 1.000000000000000000, 0.8660254037844387076, 1.000000000000000000, 0.8660254037844387076, 1.000000000000000000, 0.8660254037844387076, 1.000000000000000000, 0.8660254037844387076, 1.000000000000000000, 0.8660254037844387076, 1.000000000000000000, 0.8660254037844387076, 1.000000000000000000, 0.8660254037844387076, 1.000000000000000000, 0.8660254037844387076, 1.000000000000000000, 0.8660254037844387076, 1.000000000000000000, 0.8660254037844387076, 1.000000000000000000, 0.8660254037844387076, 1.000000000000000000, 0.8660254037844387076, 1.000000000000000000, 0.8660254037844387076, 1.000000000000000000, 0.8660254037844387076, 1.000000000000000000, 0.8660254037844387076, 1.000000000000000000, 0.8660254037844387076, 1.000000000000000000, 0.8660254037844387076, 1.000000000000000000, 0.8660254037844387076, 1.000000000000000000, 0.8660254037844387076, 1.000000000000000000, 0.8660254037844387076, 1.000000000000000000, 0.8660254037844387076, 1.000000000000000000, 0.8660254037844387076, 1.000000000000000000, 0.8660254037844387076, 1.000000000000000000, 0.8660254037844387076, 1.000000000000000000, 0.8660254037844387076, 1.000000000000000000, 0.8660254037844387076, 1.000000000000000000, 0.8660254037844387076, 1.000000000000000000, 0.8660254037844387076, 1.000000000000000000, 0.8660254037844387076, 1.000000000000000000, 0.8660254037844387076, 1.000000000000000000, 0.8660254037844387076, 1.000000000000000000, 0.8660254037844387076, 1.000000000000000000, 0.8660254037844387076, 1.000000000000000000, 0.8660254037844387076, 1.000000000000000000, 0.8660254037844387076, 1.000000000000000000, 0.8660254037844387076, 1.000000000000000000, 0.8660254037844387076, 1.000000000000000000, 0.8660254037844387076, 1.000000000000000000, 0.8660254037844387076, 1.000000000000000000, 0.8660254037844387076, 1.000000000000000000, 0.8660254037844387076, 1.000000000000000000, 0.8660254037844387076, 1.000000000000000000, 0.8660254037844387076, 1.000000000000000000, 0.8660254037844387076, 1.000000000000000000, 0.8660254037844387076, 1.000000000000000000, 0.8660254037844387076, 1.000000000000000000, 0.8660254037844387076, 1.000000000000000000, 0.8660254037844387076, 1.000000000000000000, 0.8660254037844387076, 1.000000000000000000, 0.8660254037844387076, 1.000000000000000000, 0.8660254037844387076, 1.000000000000000000, 0.8660254037844387076, 1.000000000000000000, 0.8660254037844387076, 1.000000000000000000, 0.8660254037844387076, 1.000000000000000000, 0.8660254037844387076, 1.000000000000000000, 0.8660254037844387076, 1.000000000000000000, 0.8660254037844387076, 1.000000000000000000, 0.8660254037844387076, 1.000000000000000000, 0.8660254037844387076, 1.000000000000000000, 0.8660254037844387076, 1.000000000000000000, 0.8660254037844387076, 1.000000000000000000, 0.8660254037844387076, 1.000000000000000000, 0.8660254037844387076, 1.000000000000000000, 0.8660254037844387076, 1.000000000000000000, 0.8660254037844387076, 1.000000000000000000, 0.8660254037844387076, 1.000000000000000000, 0.8660254037844387076, 1.000000000000000000, 0.8660254037844387076, 1.000000000000000000, 0.8660254037844387076, 1.000000000000000000, 0.8660254037844387076, 1.000000000000000000, 0.8660254037844387076, 1.000000000000000000, 0.8660254037844387076, 1.000000000000000000, 0.8660254037844387076, 1.000000000000000000, 0.8660254037844387076, 1.000000000000000000, 0.8660254037844387076, 1.000000000000000000, 0.8660254037844387076, 1.000000000000000000, 0.8660254037844387076, 1.000000000000000000, 0.8660254037844387076, 1.000000000000000000, 0.8660254037844387076, 1.000000000000000000, 0.8660254037844387076, 1.000000000000000000, 0.8660254037844387076, 1.000000000000000000, 0.8660254037844387076, 1.000000000000000000, 0.8660254037844387076, 1.000000000000000000, 0.8660254037844387076, 1.000000000000000000, 0.8660254037844387076, 1.000000000000000000, 0.8660254037844387076, 1.000000000000000000, 0.8660254037844387076, 1.000000000000000000, 0.8660254037844387076, 1.000000000000000000, 0.8660254037844387076, 1.000000000000000000, 0.8660254037844387076, 1.000000000000000000, 0.8660254037844387076, 1.000000000000000000, 0.8660254037844387076, 1.000000000000000000, 0.8660254037844387076, 1.000000000000000000, 0.8660254037844387076, 1.000000000000000000, 0.8660254037844387076, 1.000000000000000000, 0.8660254037844387076, 1.000000000000000000, 0.8660254037844387076, 1.000000000000000000, 0.8660254037844387076, 1.000000000000000000, 0.8660254037844387076, 1.000000000000000000, 0.8660254037844387076, 1.000000000000000000, 0.8660254037844387076, 1.000000000000000000, 0.8660254037844387076, 1.000000000000000000, 0.8660254037844387076, 1.000000000000000000, 0.8660254037844387076, 1.000000000000000000, 0.8660254037844387076, 1.000000000000000000, 0.8660254037844387076, 1.000000000000000000, 0.8660254037844387076, 1.000000000000000000, 0.8660254037844387076, 1.000000000000000000, 0.8660254037844387076, 1.000000000000000000, 0.8660254037844387076, 1.000000000000000000, 0.8660254037844387076, 1.000000000000000000, 0.8660254037844387076, 1.000000000000000000, 0.8660254037844387076, 1.000000000000000000, 0.8660254037844387076, 1.000000000000000000, 0.8660254037844387076, 1.000000000000000000, 0.8660254037844387076, 1.000000000000000000, 0.8660254037844387076, 1.000000000000000000, 0.8660254037844387076, 1.000000000000000000, 0.8660254037844387076, 1.000000000000000000, 0.8660254037844387076, 1.000000000000000000, 0.8660254037844387076, 1.000000000000000000, 0.8660254037844387076, 1.000000000000000000, 0.8660254037844387076, 1.000000000000000000, 0.8660254037844387076, 1.000000000000000000, 0.8660254037844387076, 1.000000000000000000, 0.8660254037844387076, 1.000000000000000000, 0.8660254037844387076, 1.000000000000000000, 0.8660254037844387076, 1.000000000000000000, 0.8660254037844387076, 1.000000000000000000, 0.8660254037844387076, 1.000000000000000000, 0.8660254037844387076, 1.000000000000000000, 0.8660254037844387076, 1.000000000000000000, 0.8660254037844387076, 1.000000000000000000, 0.8660254037844387076, 1.000000000000000000, 0.8660254037844387076, 1.000000000000000000, 0.8660254037844387076, 1.000000000000000000, 0.8660254037844387076, 1.000000000000000000, 0.8660254037844387076, 1.000000000000000000, 0.8660254037844387076, 1.000000000000000000, 0.8660254037844387076, 1.000000000000000000, 0.8660254037844387076, 1.000000000000000000, 0.8660254037844387076, 1.000000000000000000, 0.8660254037844387076, 1.000000000000000000, 0.8660254037844387076, 1.000000000000000000, 0.8660254037844387076, 1.000000000000000000, 0.8660254037844387076, 1.000000000000000000, 0.8660254037844387076, 1.000000000000000000, 0.8660254037844387076, 1.000000000000000000, 0.8660254037844387076, 1.000000000000000000, 0.8660254037844387076, 1.000000000000000000, 0.8660254037844387076, 1.000000000000000000, 0.8660254037844387076, 1.000000000000000000, 0.8660254037844387076, 1.000000000000000000, 0.8660254037844387076, 1.000000000000000000, 0.8660254037844387076, 1.000000000000000000, 0.8660254037844387076, 1.000000000000000000, 0.8660254037844387076, 1.000000000000000000, 0.8660254037844387076, 1.000000000000000000, 0.8660254037844387076, 1.000000000000000000, 0.8660254037844387076, 1.000000000000000000, 0.8660254037844387076, 1.000000000000000000, 0.8660254037844387076, 1.000000000000000000, 0.8660254037844387076, 1.000000000000000000, 0.8660254037844387076, 1.000000000000000000, 0.8660254037844387076, 1.000000000000000000, 0.8660254037844387076, 1.000000000000000000, 0.8660254037844387076, 1.000000000000000000, 0.8660254037844387076, 1.000000000000000000, 0.8660254037844387076, 1.000000000000000000, 0.8660254037844387076, 1.000000000000000000, 0.8660254037844387076, 1.000000000000000000, 0.8660254037844387076, 1.000000000000000000, 0.8660254037844387076, 1.000000000000000000, 0.8660254037844387076, 1.000000000000000000, 0.8660254037844387076, 1.000000000000000000, 0.8660254037844387076, 1.000000000000000000, 0.8660254037844387076, 1.000000000000000000, 0.8660254037844387076, 1.000000000000000000, 0.8660254037844387076, 1.000000000000000000, 0.8660254037844387076, 1.000000000000000000, 0.8660254037844387076, 1.000000000000000000, 0.8660254037844387076, 1.000000000000000000, 0.8660254037844387076, 1.000000000000000000, 0.8660254037844387076, 1.000000000000000000, 0.8660254037844387076, 1.000000000000000000, 0.8660254037844387076, 1.000000000000000000, 0.8660254037844387076, 1.000000000000000000, 0.8660254037844387076, 1.000000000000000000, 0.8660254037844387076, 1.000000000000000000, 0.8660254037844387076, 1.000000000000000000, 0.8660254037844387076, 1.000000000000000000, 0.8660254037844387076, 1.000000000000000000, 0.8660254037844387076, 1.000000000000000000, 0.8660254037844387076, 1.000000000000000000, 0.8660254037844387076, 1.000000000000000000, 0.8660254037844387076, 1.000000000000000000, 0.8660254037844387076, 1.000000000000000000, 0.8660254037844387076, 1.000000000000000000, 0.8660254037844387076, 1.000000000000000000, 0.8660254037844387076, 1.000000000000000000, 0.8660254037844387076, 1.000000000000000000, 0.8660254037844387076, 1.000000000000000000, 0.8660254037844387076, 1.000000000000000000, 0.8660254037844387076, 1.000000000000000000, 0.8660254037844387076, 1.000000000000000000, 0.8660254037844387076, 1.000000000000000000, 0.8660254037844387076, 1.000000000000000000, 0.8660254037844387076, 1.000000000000000000, 0.8660254037844387076, 1.000000000000000000, 0.8660254037844387076, 1.000000000000000000, 0.8660254037844387076, 1.000000000000000000, 0.8660254037844387076, 1.000000000000000000, 0.8660254037844387076, 1.000000000000000000, 0.8660254037844387076, 1.000000000000000000, 0.8660254037844387076, 1.000000000000000000, 0.8660254037844387076, 1.000000000000000000, 0.8660254037844387076, 1.000000000000000000, 0.8660254037844387076, 1.000000000000000000, 0.8660254037844387076, 1.000000000000000000, 0.8660254037844387076, 1.000000000000000000, 0.8660254037844387076, 1.000000000000000000, 0.8660254037844387076, 1.000000000000000000, 0.8660254037844387076, 1.000000000000000000, 0.8660254037844387076, 1.000000000000000000, 0.8660254037844387076, 1.000000000000000000, 0.8660254037844387076, 1.000000000000000000, 0.8660254037844387076, 1.000000000000000000, 0.8660254037844387076, 1.000000000000000000, 0.8660254037844387076, 1.000000000000000000, 0.8660254037844387076, 1.000000000000000000, 0.8660254037844387076, 1.000000000000000000, 0.8660254037844387076, 1.000000000000000000, 0.8660254037844387076, 1.000000000000000000, 0.8660254037844387076, 1.000000000000000000, 0.8660254037844387076, 1.000000000000000000, 0.8660254037844387076, 1.000000000000000000, 0.8660254037844387076, 1.000000000000000000, 0.8660254037844387076, 1.000000000000000000, 0.8660254037844387076, 1.000000000000000000, 0.8660254037844387076, 1.000000000000000000, 0.8660254037844387076, 1.000000000000000000, 0.8660254037844387076, 1.000000000000000000, 0.8660254037844387076, 1.000000000000000000, 0.8660254037844387076, 1.000000000000000000, 0.8660254037844387076, 1.000000000000000000, 0.8660254037844387076, 1.000000000000000000, 0.8660254037844387076, 1.000000000000000000, 0.8660254037844387076, 1.000000000000000000, 0.8660254037844387076, 1.000000000000000000, 0.8660254037844387076, 1.000000000000000000, 0.8660254037844387076, 1.000000000000000000, 0.8660254037844387076, 1.000000000000000000, 0.8660254037844387076, 1.000000000000000000, 0.8660254037844387076, 1.000000000000000000, 0.8660254037844387076, 1.000000000000000000, 0.8660254037844387076, 1.000000000000000000, 0.8660254037844387076, 1.000000000000000000, 0.8660254037844387076, 1.000000000000000000, 0.8660254037844387076, 1.000000000000000000, 0.8660254037844387076, 1.000000000000000000, 0.8660254037844387076, 1.000000000000000000, 0.8660254037844387076, 1.000000000000000000, 0.8660254037844387076, 1.000000000000000000, 0.8660254037844387076, 1.000000000000000000, 0.8660254037844387076, 1.000000000000000000, 0.8660254037844387076, 1.000000000000000000, 0.8660254037844387076, 1.000000000000000000, 0.8660254037844387076, 1.000000000000000000, 0.8660254037844387076, 1.000000000000000000, 0.8660254037844387076, 1.000000000000000000, 0.8660254037844387076, 1.000000000000000000, 0.8660254037844387076, 1.000000000000000000, 0.8660254037844387076, 1.000000000000000000, 0.8660254037844387076, 1.000000000000000000, 0.8660254037844387076, 1.000000000000000000, 0.8660254037844387076, 1.000000000000000000, 0.8660254037844387076, 1.000000000000000000, 0.8660254037844387076, 1.000000000000000000, 0.8660254037844387076, 1.000000000000000000, 0.8660254037844387076, 1.000000000000000000, 0.8660254037844387076, 1.000000000000000000, 0.8660254037844387076, 1.000000000000000000, 0.8660254037844387076, 1.000000000000000000, 0.8660254037844387076, 1.000000000000000000, 0.8660254037844387076, 1.000000000000000000, 0.8660254037844387076, 1.000000000000000000, 0.8660254037844387076, 1.000000000000000000, 0.8660254037844387076, 1.000000000000000000, 0.8660254037844387076, 1.000000000000000000, 0.8660254037844387076, 1.000000000000000000, 0.8660254037844387076, 1.000000000000000000, 0.8660254037844387076, 1.000000000000000000, 0.8660254037844387076, 1.000000000000000000, 0.8660254037844387076, 1.000000000000000000, 0.8660254037844387076, 1.000000000000000000, 0.8660254037844387076, 1.000000000000000000, 0.8660254037844387076, 1.000000000000000000, 0.8660254037844387076, 1.000000000000000000, 0.8660254037844387076, 1.000000000000000000, 0.8660254037844387076, 1.000000000000000000, 0.8660254037844387076, 1.000000000000000000, 0.8660254037844387076, 1.000000000000000000, 0.8660254037844387076, 1.000000000000000000, 0.8660254037844387076, 1.000000000000000000, 0.8660254037844387076, 1.000000000000000000, 0.8660254037844387076, 1.000000000000000000, 0.8660254037844387076, 1.000000000000000000, 0.8660254037844387076, 1.000000000000000000, 0.8660254037844387076, 1.000000000000000000, 0.8660254037844387076, 1.000000000000000000, 0.8660254037844387076, 1.000000000000000000, 0.8660254037844387076, 1.000000000000000000, 0.8660254037844387076, 1.000000000000000000, 0.8660254037844387076, 1.000000000000000000, 0.8660254037844387076, 1.000000000000000000, 0.8660254037844387076, 1.000000000000000000, 0.8660254037844387076, 1.000000000000000000, 0.8660254037844387076, 1.000000000000000000, 0.8660254037844387076, 1.000000000000000000, 0.8660254037844387076, 1.000000000000000000, 0.8660254037844387076, 1.000000000000000000, 0.8660254037844387076, 1.000000000000000000, 0.8660254037844387076, 1.000000000000000000, 0.8660254037844387076, 1.000000000000000000, 0.8660254037844387076, 1.000000000000000000, 0.8660254037844387076, 1.000000000000000000, 0.8660254037844387076, 1.000000000000000000, 0.8660254037844387076, 1.000000000000000000, 0.8660254037844387076, 1.000000000000000000, 0.8660254037844387076, 1.000000000000000000, 0.8660254037844387076, 1.000000000000000000, 0.8660254037844387076, 1.000000000000000000, 0.8660254037844387076, 1.000000000000000000, 0.8660254037844387076, 1.000000000000000000, 0.8660254037844387076, 1.000000000000000000, 0.8660254037844387076, 1.000000000000000000, 0.8660254037844387076, 1.000000000000000000, 0.8660254037844387076, 1.000000000000000000, 0.8660254037844387076, 1.000000000000000000, 0.8660254037844387076, 1.000000000000000000, 0.8660254037844387076, 1.000000000000000000, 0.8660254037844387076, 1.000000000000000000, 0.8660254037844387076, 1.000000000000000000, 0.8660254037844387076, 1.000000000000000000, 0.8660254037844387076, 1.000000000000000000, 0.8660254037844387076, 1.000000000000000000, 0.8660254037844387076, 1.000000000000000000, 0.8660254037844387076, 1.000000000000000000, 0.8660254037844387076, 1.000000000000000000, 0.8660254037844387076, 1.000000000000000000, 0.8660254037844387076, 1.000000000000000000, 0.8660254037844387076, 1.000000000000000000, 0.8660254037844387076, 1.000000000000000000, 0.8660254037844387076, 1.000000000000000000, 0.8660254037844387076, 1.000000000000000000, 0.8660254037844387076, 1.000000000000000000, 0.8660254037844387076, 1.000000000000000000, 0.8660254037844387076, 1.000000000000000000, 0.8660254037844387076, 1.000000000000000000, 0.8660254037844387076, 1.000000000000000000, 0.8660254037844387076, 1.000000000000000000, 0.8660254037844387076, 1.000000000000000000, 0.8660254037844387076, 1.000000000000000000, 0.8660254037844387076, 1.000000000000000000, 0.8660254037844387076, 1.000000000000000000, 0.8660254037844387076, 1.000000000000000000, 0.8660254037844387076, 1.000000000000000000, 0.8660254037844387076, 1.000000000000000000, 0.8660254037844387076, 1.000000000000000000, 0.8660254037844387076, 1.000000000000000000, 0.8660254037844387076, 1.000000000000000000, 0.8660254037844387076, 1.000000000000000000, 0.8660254037844387076, 1.000000000000000000, 0.8660254037844387076, 1.000000000000000000, 0.8660254037844387076, 1.000000000000000000, 0.8660254037844387076, 1.000000000000000000, 0.8660254037844387076, 1.000000000000000000, 0.8660254037844387076, 1.000000000000000000, 0.8660254037844387076, 1.000000000000000000, 0.8660254037844387076, 1.000000000000000000, 0.8660254037844387076, 1.000000000000000000, 0.8660254037844387076, 1.000000000000000000, 0.8660254037844387076, 1.000000000000000000, 0.8660254037844387076, 1.000000000000000000, 0.8660254037844387076, 1.000000000000000000, 0.8660254037844387076, 1.000000000000000000, 0.8660254037844387076, 1.000000000000000000, 0.8660254037844387076, 1.000000000000000000, 0.8660254037844387076, 1.000000000000000000, 0.8660254037844387076, 1.000000000000000000, 0.8660254037844387076, 1.000000000000000000, 0.8660254037844387076, 1.000000000000000000, 0.8660254037844387076, 1.000000000000000000, 0.8660254037844387076, 1.000000000000000000, 0.8660254037844387076, 1.000000000000000000, 0.8660254037844387076, 1.000000000000000000, 0.8660254037844387076, 1.000000000000000000, 0.8660254037844387076, 1.000000000000000000, 0.8660254037844387076, 1.000000000000000000, 0.8660254037844387076, 1.000000000000000000, 0.8660254037844387076, 1.000000000000000000, 0.8660254037844387076, 1.000000000000000000, 0.8660254037844387076, 1.000000000000000000, 0.8660254037844387076, 1.000000000000000000, 0.8660254037844387076, 1.000000000000000000, 0.8660254037844387076, 1.000000000000000000, 0.8660254037844387076, 1.000000000000000000 ) ) 
 REPRESENTATION_ITEM ( '' )  );
#19964=CARTESIAN_POINT ( 'NONE',  ( -2.500000000000000444, 6.833333333333333925, -4.330127018922193649 ) ) ;
#19966=CARTESIAN_POINT ( 'NONE',  ( -1.339745962155613812, -60.08034179853027723, -5.000000000000000000 ) ) ;
#19967=CARTESIAN_POINT ( 'NONE',  ( -3.152548672688508926E-16, -52.56249999863440792, -5.148502694627439702 ) ) ;
#19968=CARTESIAN_POINT ( 'NONE',  ( -2.500000000000000444, -89.04166666393547303, -4.330127018922193649 ) ) ;
#19969=CARTESIAN_POINT ( 'NONE',  ( 2.229367062499998831, -35.64583333196772941, -3.861377020970580887 ) ) ;
#19971=CARTESIAN_POINT ( 'NONE',  ( -2.500000000000000444, 19.95833333606451987, -4.330127018922193649 ) ) ;
#19977=CARTESIAN_POINT ( 'NONE',  ( -2.500000000000000444, -41.16666666666667140, -4.330127018922193649 ) ) ;
#19980=CARTESIAN_POINT ( 'NONE',  ( -3.152548672688508926E-16, -103.5624999986344221, -5.148502694627439702 ) ) ;
#19981=CARTESIAN_POINT ( 'NONE',  ( 4.458734124999999437, 2.937500001365594304, -5.460374474430324690E-16 ) ) ;
#19982=CYLINDRICAL_SURFACE ( 'NONE', #1124, 5.000000000000000000 ) ;
#19991=CARTESIAN_POINT ( 'NONE',  ( 1.975475456537005874E-15, 19.25000000000000000, 5.000000000000000000 ) ) ;
#19992=ORIENTED_EDGE ( 'NONE', *, *, #10952, .F. ) ;
#19996=CARTESIAN_POINT ( 'NONE',  ( -4.458734124999999437, -23.56249999863440436, 0.000000000000000000 ) ) ;
#20004=ORIENTED_EDGE ( 'NONE', *, *, #62997, .T. ) ;
#20005=EDGE_CURVE ( 'NONE', #62925, #45741, #30591, .T. ) ;
#20008=CARTESIAN_POINT ( 'NONE',  ( 2.229367062499998831, -70.89583333196773651, -3.861377020970580887 ) ) ;
#20011=VERTEX_POINT ( 'NONE', #44741 ) ;
#20015=CARTESIAN_POINT ( 'NONE',  ( -4.458734124999999437, -5.562499998634402587, 0.000000000000000000 ) ) ;
#20024=VERTEX_POINT ( 'NONE', #58286 ) ;
#20025=CARTESIAN_POINT ( 'NONE',  ( -4.458734124999997661, -82.22916666530106511, 2.574251347313722516 ) ) ;
#20027=CARTESIAN_POINT ( 'NONE',  ( -3.152548672688508926E-16, 2.437500001365594304, -5.148502694627439702 ) ) ;
#20029=CARTESIAN_POINT ( 'NONE',  ( 1.060575238724906964E-15, -82.75000000000001421, 5.773502691896257311 ) ) ;
#20031=CARTESIAN_POINT ( 'NONE',  ( 4.458734125000001214, -64.14583333196773651, 2.574251347313718519 ) ) ;
#20032=CARTESIAN_POINT ( 'NONE',  ( 5.000000000000000888, -27.45833333060214798, 2.886751345948126879 ) ) ;
#20036=CARTESIAN_POINT ( 'NONE',  ( 1.975475456537005874E-15, -64.62499999726880162, 5.000000000000000000 ) ) ;
#20038=CARTESIAN_POINT ( 'NONE',  ( -4.458734124999999437, -46.31249999863440792, 0.000000000000000000 ) ) ;
#20039=CARTESIAN_POINT ( 'NONE',  ( -4.458734124999999437, -32.56249999863440792, 0.000000000000000000 ) ) ;
#20042=CARTESIAN_POINT ( 'NONE',  ( 5.000000000000000000, 18.58333333333333215, -2.886751345948129988 ) ) ;
#20044=CARTESIAN_POINT ( 'NONE',  ( 1.339745962155612702, -54.16965819600732601, -5.000000000000000000 ) ) ;
#20045=CARTESIAN_POINT ( 'NONE',  ( 9.457646018065525792E-16, -36.06249999863441502, 5.148502694627439702 ) ) ;
#20046=CARTESIAN_POINT ( 'NONE',  ( -5.000000000000000000, -75.95833333060215864, -2.886751345948128211 ) ) ;
#20052=CARTESIAN_POINT ( 'NONE',  ( 2.229367062499998831, -81.89583333196773651, -3.861377020970580887 ) ) ;
#20054=CARTESIAN_POINT ( 'NONE',  ( -6.972266317189433020E-16, 18.87500000273119127, -5.000000000000000000 ) ) ;
#20056=CARTESIAN_POINT ( 'NONE',  ( 1.060575238724906964E-15, -25.75000000000000000, 5.773502691896257311 ) ) ;
#20058=ORIENTED_EDGE ( 'NONE', *, *, #30369, .F. ) ;
#20060=ORIENTED_EDGE ( 'NONE', *, *, #56942, .F. ) ;
#20062=CARTESIAN_POINT ( 'NONE',  ( -2.499999999999996447, 22.29166666939785202, 4.330127018922195425 ) ) ;
#20067=( BOUNDED_CURVE ( )  B_SPLINE_CURVE ( 2, ( #5019, #19167, #39416, #23394, #24638, #63570, #14031, #47813, #43609 ),
 .UNSPECIFIED., .F., .F. ) 
 B_SPLINE_CURVE_WITH_KNOTS ( ( 3, 2, 2, 2, 3 ),
 ( 0.2660714285714285698, 0.2666666666666666630, 0.2678571428571428492, 0.2690476190476190355, 0.2696428571428571286 ),
 .UNSPECIFIED. ) 
 CURVE ( )  GEOMETRIC_REPRESENTATION_ITEM ( )  RATIONAL_B_SPLINE_CURVE ( ( 0.9330127018922194093, 0.9330127018922194093, 1.000000000000000000, 0.8660254037844387076, 1.000000000000000000, 0.8660254037844387076, 1.000000000000000000, 0.9330127018922194093, 0.9330127018922194093 ) ) 
 REPRESENTATION_ITEM ( '' )  );
#20072=CARTESIAN_POINT ( 'NONE',  ( -4.458734124999999437, -22.39583333196773651, -2.574251347313719407 ) ) ;
#20082=CARTESIAN_POINT ( 'NONE',  ( 1.339745962155612702, -4.294658198738519062, -5.000000000000000000 ) ) ;
#20083=CARTESIAN_POINT ( 'NONE',  ( -1.339745962155613812, -29.20534180126147916, -5.000000000000000000 ) ) ;
#20085=ORIENTED_EDGE ( 'NONE', *, *, #4279, .T. ) ;
#20088=CARTESIAN_POINT ( 'NONE',  ( 5.000000000000000000, -86.41666666666667140, -2.886751345948130876 ) ) ;
#20092=CARTESIAN_POINT ( 'NONE',  ( -4.458734124999999437, 12.60416666803225993, -2.574251347313719407 ) ) ;
#20098=CARTESIAN_POINT ( 'NONE',  ( -6.972266317189433020E-16, -39.25000000000000000, -5.000000000000000000 ) ) ;
#20100=CARTESIAN_POINT ( 'NONE',  ( -2.229367062500000163, -67.47916666530106511, -3.861377020970580443 ) ) ;
#20102=CARTESIAN_POINT ( 'NONE',  ( -3.152548672688508926E-16, 19.43750000136559208, -5.148502694627439702 ) ) ;
#20103=AXIS2_PLACEMENT_3D ( 'NONE', #43981, #14717, #8956 ) ;
#20104=CARTESIAN_POINT ( 'NONE',  ( -5.000000000000000000, 18.00000000000000000, 0.000000000000000000 ) ) ;
#20105=ADVANCED_FACE ( 'NONE', ( #383, #63120 ), #19031, .F. ) ;
#20107=CARTESIAN_POINT ( 'NONE',  ( -2.229367062500000163, -50.72916666530107221, -3.861377020970580443 ) ) ;
#20108=CARTESIAN_POINT ( 'NONE',  ( 1.060575238724906964E-15, -10.62499999726881583, 5.773502691896257311 ) ) ;
#20114=CARTESIAN_POINT ( 'NONE',  ( -3.152548672688508926E-16, -15.81249999863440436, -5.148502694627439702 ) ) ;
#20119=CARTESIAN_POINT ( 'NONE',  ( 2.229367062500001939, -104.9791666653010651, 3.861377020970579999 ) ) ;
#20121=CARTESIAN_POINT ( 'NONE',  ( -2.229367062499996610, -96.39583333196773651, 3.861377020970582219 ) ) ;
#20122=CARTESIAN_POINT ( 'NONE',  ( -2.499999999999996447, -7.833333333333331261, 4.330127018922195425 ) ) ;
#20123=CARTESIAN_POINT ( 'NONE',  ( -2.500000000000000444, -56.04166666393548013, -4.330127018922193649 ) ) ;
#20125=DIRECTION ( 'NONE',  ( -0.000000000000000000, 1.000000000000000000, -0.000000000000000000 ) ) ;
#20126=EDGE_CURVE ( 'NONE', #5147, #49482, #58835, .T. ) ;
#20129=CARTESIAN_POINT ( 'NONE',  ( 2.229367062499998831, -17.64583333196773651, -3.861377020970580887 ) ) ;
#20130=CARTESIAN_POINT ( 'NONE',  ( 4.458734124999999437, 4.937500001365595637, -5.460374474430324690E-16 ) ) ;
#20131=CARTESIAN_POINT ( 'NONE',  ( -4.458734124999999437, -62.64583333196774362, -2.574251347313719407 ) ) ;
#20135=CARTESIAN_POINT ( 'NONE',  ( -4.999999999999999112, -6.916666666666667851, 2.886751345948131764 ) ) ;
#20140=CARTESIAN_POINT ( 'NONE',  ( -1.336351044127974539E-14, 21.37500000273118417, 5.000000000000000000 ) ) ;
#20141=EDGE_CURVE ( 'NONE', #21367, #31465, #30913, .T. ) ;
#20145=CARTESIAN_POINT ( 'NONE',  ( -4.458734124999999437, -93.39583333196773651, -2.574251347313719407 ) ) ;
#20146=CARTESIAN_POINT ( 'NONE',  ( 4.458734124999999437, 17.93750000136559208, -5.460374474430324690E-16 ) ) ;
#20149=DIRECTION ( 'NONE',  ( -0.000000000000000000, 1.000000000000000000, -0.000000000000000000 ) ) ;
#20151=CARTESIAN_POINT ( 'NONE',  ( 2.499999999999998668, -73.33333333333332860, -4.330127018922193649 ) ) ;
#20153=ORIENTED_EDGE ( 'NONE', *, *, #43546, .F. ) ;
#20155=ORIENTED_EDGE ( 'NONE', *, *, #58619, .T. ) ;
#20156=CARTESIAN_POINT ( 'NONE',  ( -6.972266317189433020E-16, -104.2500000000000000, -5.000000000000000000 ) ) ;
#20158=AXIS2_PLACEMENT_3D ( 'NONE', #2585, #56932, #1965 ) ;
#20160=EDGE_LOOP ( 'NONE', ( #58127, #14401, #15186, #4147 ) ) ;
#20166=CARTESIAN_POINT ( 'NONE',  ( -2.229367062499996610, -64.39583333196773651, 3.861377020970582219 ) ) ;
#20169=CARTESIAN_POINT ( 'NONE',  ( 2.500000000000002220, 3.458333336064517205, 4.330127018922192761 ) ) ;
#20170=ORIENTED_EDGE ( 'NONE', *, *, #58688, .F. ) ;
#20173=CARTESIAN_POINT ( 'NONE',  ( -5.000000000000000000, -83.99999999999998579, 0.000000000000000000 ) ) ;
#20177=CARTESIAN_POINT ( 'NONE',  ( -4.458734124999998549, -110.4791666653010793, 2.574251347313722516 ) ) ;
#20178=CARTESIAN_POINT ( 'NONE',  ( 2.500000000000002220, 20.33333333333333215, 4.330127018922192761 ) ) ;
#20179=ORIENTED_EDGE ( 'NONE', *, *, #47645, .T. ) ;
#20183=CARTESIAN_POINT ( 'NONE',  ( -4.458734124999999437, -46.39583333196774362, -2.574251347313719407 ) ) ;
#20186=CARTESIAN_POINT ( 'NONE',  ( -2.229367062499996610, -48.14583333196772941, 3.861377020970582219 ) ) ;
#20187=DIRECTION ( 'NONE',  ( 0.000000000000000000, 0.000000000000000000, 1.000000000000000000 ) ) ;
#20188=CARTESIAN_POINT ( 'NONE',  ( 2.229367062500001939, -14.97916666530107399, 3.861377020970579999 ) ) ;
#20189=CARTESIAN_POINT ( 'NONE',  ( 5.000000000000000000, -100.4166666666666572, -2.886751345948129988 ) ) ;
#20191=CARTESIAN_POINT ( 'NONE',  ( -4.458734124999998549, -34.47916666530107221, 2.574251347313722516 ) ) ;
#20192=CARTESIAN_POINT ( 'NONE',  ( -5.000000000000000000, 8.041666669397852019, -2.886751345948128211 ) ) ;
#20197=CYLINDRICAL_SURFACE ( 'NONE', #28467, 5.000000000000000000 ) ;
#20198=CARTESIAN_POINT ( 'NONE',  ( 9.457646018065525792E-16, 1.687500001365593194, 5.148502694627439702 ) ) ;
#20199=ORIENTED_EDGE ( 'NONE', *, *, #17013, .T. ) ;
#20200=VECTOR ( 'NONE', #13888, 1000.000000000000000 ) ;
#20201=CARTESIAN_POINT ( 'NONE',  ( 2.499999999999998668, 16.79166666939785202, -4.330127018922193649 ) ) ;
#20202=CARTESIAN_POINT ( 'NONE',  ( -4.999999999999999112, -93.91666666666667140, 2.886751345948131764 ) ) ;
#20203=CARTESIAN_POINT ( 'NONE',  ( -4.458734124999999437, -37.39583333196773651, -2.574251347313719407 ) ) ;
#20204=CARTESIAN_POINT ( 'NONE',  ( -2.500000000000000444, -36.16666666666666430, -4.330127018922193649 ) ) ;
#20205=CARTESIAN_POINT ( 'NONE',  ( 4.458734125000001214, -79.14583333196772230, 2.574251347313718519 ) ) ;
#20209=AXIS2_PLACEMENT_3D ( 'NONE', #18846, #23997, #43600 ) ;
#20212=CARTESIAN_POINT ( 'NONE',  ( 9.457646018065525792E-16, -4.062499998634408804, 5.148502694627439702 ) ) ;
#20213=CARTESIAN_POINT ( 'NONE',  ( 2.229367062500001939, 20.77083333469892779, 3.861377020970579999 ) ) ;
#20214=CARTESIAN_POINT ( 'NONE',  ( -4.458734124999999437, -42.64583333196773651, -2.574251347313719407 ) ) ;
#20220=CARTESIAN_POINT ( 'NONE',  ( -2.229367062499996610, -74.14583333196773651, 3.861377020970582219 ) ) ;
#20221=CARTESIAN_POINT ( 'NONE',  ( 2.500000000000002220, -107.5416666639354730, 4.330127018922192761 ) ) ;
#20223=EDGE_CURVE ( 'NONE', #23230, #8786, #19382, .T. ) ;
#20224=CARTESIAN_POINT ( 'NONE',  ( -1.339745962155585168, 9.794658198738519062, -5.000000000000015987 ) ) ;
#20225=LINE ( 'NONE', #5109, #35771 ) ;
#20227=CARTESIAN_POINT ( 'NONE',  ( 5.000000000000000000, -57.49999999999999289, -6.123233995736766282E-16 ) ) ;
#20228=CARTESIAN_POINT ( 'NONE',  ( -6.972266317189433020E-16, -32.12499999726880873, -5.000000000000000000 ) ) ;
#20231=DIRECTION ( 'NONE',  ( -0.000000000000000000, 1.000000000000000000, -0.000000000000000000 ) ) ;
#20238=ORIENTED_EDGE ( 'NONE', *, *, #26111, .T. ) ;
#20239=CARTESIAN_POINT ( 'NONE',  ( 5.000000000000000000, 5.500000000000001776, -6.123233995736766282E-16 ) ) ;
#20242=ORIENTED_EDGE ( 'NONE', *, *, #21391, .T. ) ;
#20246=CARTESIAN_POINT ( 'NONE',  ( -2.229367062500000163, -46.72916666530106511, -3.861377020970580443 ) ) ;
#20247=CARTESIAN_POINT ( 'NONE',  ( 0.000000000000000000, -120.0000000000000000, 5.000000000000000000 ) ) ;
#20259=CARTESIAN_POINT ( 'NONE',  ( -4.458734124999999437, -87.56249999863439371, 0.000000000000000000 ) ) ;
#20260=CARTESIAN_POINT ( 'NONE',  ( -6.972266317189433020E-16, -3.250000000000001332, -5.000000000000000000 ) ) ;
#20261=ORIENTED_EDGE ( 'NONE', *, *, #59361, .F. ) ;
#20266=CARTESIAN_POINT ( 'NONE',  ( -2.229367062500000163, 5.520833334698927786, -3.861377020970580443 ) ) ;
#20267=CARTESIAN_POINT ( 'NONE',  ( 5.000000000000000888, -106.5833333333333286, 2.886751345948126879 ) ) ;
#20268=CARTESIAN_POINT ( 'NONE',  ( 2.229367062499998831, -14.89583333196773474, -3.861377020970580887 ) ) ;
#20273=CARTESIAN_POINT ( 'NONE',  ( 2.229367062499998831, 20.10416666803225993, -3.861377020970580887 ) ) ;
#20275=CARTESIAN_POINT ( 'NONE',  ( -4.458734124999997661, -97.22916666530105090, 2.574251347313722516 ) ) ;
#20276=DIRECTION ( 'NONE',  ( -0.000000000000000000, 1.000000000000000000, -0.000000000000000000 ) ) ;
#20277=CARTESIAN_POINT ( 'NONE',  ( 5.000000000000000000, -57.29166666393548013, -2.886751345948130876 ) ) ;
#20278=CARTESIAN_POINT ( 'NONE',  ( -2.229367062500000163, -12.47916666530107044, -3.861377020970580443 ) ) ;
#20282=CARTESIAN_POINT ( 'NONE',  ( 5.000000000000000000, -43.29166666393548724, -2.886751345948129988 ) ) ;
#20284=CARTESIAN_POINT ( 'NONE',  ( -2.229367062499996610, 11.85416666803225993, 3.861377020970582219 ) ) ;
#20285=CARTESIAN_POINT ( 'NONE',  ( 5.000000000000000888, -35.58333333333332860, 2.886751345948126879 ) ) ;
#20286=CARTESIAN_POINT ( 'NONE',  ( -6.972266317189433020E-16, -48.12499999726880873, -5.000000000000000000 ) ) ;
#20288=CARTESIAN_POINT ( 'NONE',  ( 4.458734124999999437, -59.81249999863440081, -5.460374474430324690E-16 ) ) ;
#20291=CARTESIAN_POINT ( 'NONE',  ( 5.000000000000000000, 4.500000000000000888, -6.123233995736766282E-16 ) ) ;
#20294=CARTESIAN_POINT ( 'NONE',  ( -4.458734124999999437, -55.31249999863440081, 0.000000000000000000 ) ) ;
#20295=CARTESIAN_POINT ( 'NONE',  ( 1.060575238724906964E-15, -88.62499999726880162, 5.773502691896257311 ) ) ;
#20296=AXIS2_PLACEMENT_3D ( 'NONE', #32093, #51729, #7669 ) ;
#20297=CARTESIAN_POINT ( 'NONE',  ( -2.229367062499996610, -34.14583333196772941, 3.861377020970582219 ) ) ;
#20299=CARTESIAN_POINT ( 'NONE',  ( -4.999999999999998224, 20.20833333606451987, 2.886751345948131764 ) ) ;
#20300=CARTESIAN_POINT ( 'NONE',  ( -1.230605004983934782E-13, -26.62499999726881583, 5.000000000000000000 ) ) ;
#20303=( BOUNDED_CURVE ( )  B_SPLINE_CURVE ( 2, ( #24018, #42370, #57814, #62328, #28836, #62649, #57508, #8293, #13112 ),
 .UNSPECIFIED., .F., .F. ) 
 B_SPLINE_CURVE_WITH_KNOTS ( ( 3, 2, 2, 2, 3 ),
 ( 0.1625000000000000056, 0.1630952380952380987, 0.1642857142857142849, 0.1654761904761904712, 0.1660714285714285643 ),
 .UNSPECIFIED. ) 
 CURVE ( )  GEOMETRIC_REPRESENTATION_ITEM ( )  RATIONAL_B_SPLINE_CURVE ( ( 0.9330127018922194093, 0.9330127018922194093, 1.000000000000000000, 0.8660254037844387076, 1.000000000000000000, 0.8660254037844387076, 1.000000000000000000, 0.9330127018922194093, 0.9330127018922194093 ) ) 
 REPRESENTATION_ITEM ( '' )  );
#20304=CARTESIAN_POINT ( 'NONE',  ( -2.500000000000000444, -43.16666666666665719, -4.330127018922193649 ) ) ;
#20305=CARTESIAN_POINT ( 'NONE',  ( -5.000000000000000000, -19.95833333060214798, -2.886751345948128211 ) ) ;
#20306=CYLINDRICAL_SURFACE ( 'NONE', #24273, 5.000000000000000000 ) ;
#20307=EDGE_LOOP ( 'NONE', ( #59006, #21941, #52073, #33861 ) ) ;
#20308=CARTESIAN_POINT ( 'NONE',  ( -2.229367062499996610, -101.1458333319677365, 3.861377020970582219 ) ) ;
#20309=CARTESIAN_POINT ( 'NONE',  ( 4.458734124999998549, 4.020833334698926009, -2.574251347313721627 ) ) ;
#20310=CARTESIAN_POINT ( 'NONE',  ( -6.972266317189433020E-16, -59.25000000000000000, -5.000000000000000000 ) ) ;
#20316=CARTESIAN_POINT ( 'NONE',  ( 1.975475456537005874E-15, -81.74999999999998579, 5.000000000000000000 ) ) ;
#20317=DIRECTION ( 'NONE',  ( -0.000000000000000000, 1.000000000000000000, -0.000000000000000000 ) ) ;
#20319=CARTESIAN_POINT ( 'NONE',  ( 1.975475456537005874E-15, -48.62499999726880162, 5.000000000000000000 ) ) ;
#20321=CARTESIAN_POINT ( 'NONE',  ( 4.330127018922258486, 30.00000000000000000, 7.499999999999910294 ) ) ;
#20322=CARTESIAN_POINT ( 'NONE',  ( 4.458734125000001214, -23.14583333196773651, 2.574251347313718519 ) ) ;
#20331=ORIENTED_EDGE ( 'NONE', *, *, #23213, .T. ) ;
#20332=DIRECTION ( 'NONE',  ( -0.5000000000000009992, 0.000000000000000000, -0.8660254037844380415 ) ) ;
#20334=CARTESIAN_POINT ( 'NONE',  ( 4.458734125000001214, -73.14583333196773651, 2.574251347313718519 ) ) ;
#20337=VERTEX_POINT ( 'NONE', #42773 ) ;
#20339=VECTOR ( 'NONE', #14312, 1000.000000000000000 ) ;
#20342=CARTESIAN_POINT ( 'NONE',  ( 2.229367062499998831, -3.895833331967739177, -3.861377020970580887 ) ) ;
#20343=ORIENTED_EDGE ( 'NONE', *, *, #35745, .T. ) ;
#20345=CYLINDRICAL_SURFACE ( 'NONE', #56209, 5.000000000000000000 ) ;
#20350=( BOUNDED_CURVE ( )  B_SPLINE_CURVE ( 2, ( #11083, #40025, #5631, #54190, #10128, #50330, #59343, #44214, #29735 ),
 .UNSPECIFIED., .F., .F. ) 
 B_SPLINE_CURVE_WITH_KNOTS ( ( 3, 2, 2, 2, 3 ),
 ( 0.1160714285714285754, 0.1166666666666666685, 0.1178571428571428548, 0.1190476190476190410, 0.1196428571428571480 ),
 .UNSPECIFIED. ) 
 CURVE ( )  GEOMETRIC_REPRESENTATION_ITEM ( )  RATIONAL_B_SPLINE_CURVE ( ( 0.9330127018922194093, 0.9330127018922194093, 1.000000000000000000, 0.8660254037844387076, 1.000000000000000000, 0.8660254037844387076, 1.000000000000000000, 0.9330127018922185211, 0.9330127018922192983 ) ) 
 REPRESENTATION_ITEM ( '' )  );
#20352=ORIENTED_EDGE ( 'NONE', *, *, #58619, .F. ) ;
#20353=CARTESIAN_POINT ( 'NONE',  ( 4.458734125000000326, -78.89583333196775072, 2.574251347313718519 ) ) ;
#20355=CARTESIAN_POINT ( 'NONE',  ( -4.458734124999999437, 3.604166668032260379, -2.574251347313719407 ) ) ;
#20358=CARTESIAN_POINT ( 'NONE',  ( -2.500000000000000444, -87.16666666666667140, -4.330127018922193649 ) ) ;
#20360=CARTESIAN_POINT ( 'NONE',  ( -4.458734124999998549, -67.47916666530106511, 2.574251347313722516 ) ) ;
#20361=CARTESIAN_POINT ( 'NONE',  ( 2.500000000000002220, -23.54166666393548368, 4.330127018922192761 ) ) ;
#20362=CARTESIAN_POINT ( 'NONE',  ( 1.975475456537005874E-15, -14.74999999999999822, 5.000000000000000000 ) ) ;
#20363=CARTESIAN_POINT ( 'NONE',  ( 9.457646018065525792E-16, 28.93750000136558853, 5.148502694627439702 ) ) ;
#20364=CARTESIAN_POINT ( 'NONE',  ( -6.972266317189433020E-16, -38.12499999726880873, -5.000000000000000000 ) ) ;
#20365=CARTESIAN_POINT ( 'NONE',  ( 1.339745962155615144, -43.58034179853029144, 4.999999999999999112 ) ) ;
#20366=CARTESIAN_POINT ( 'NONE',  ( 2.229367062499998831, -46.64583333196774362, -3.861377020970580887 ) ) ;
#20367=CARTESIAN_POINT ( 'NONE',  ( -4.458734124999999437, -33.64583333196772941, -2.574251347313719407 ) ) ;
#20370=CARTESIAN_POINT ( 'NONE',  ( -5.000000000000000000, 18.00000000000000000, 0.000000000000000000 ) ) ;
#20373=CARTESIAN_POINT ( 'NONE',  ( -4.458734124999999437, -38.39583333196773651, -2.574251347313719407 ) ) ;
#20374=CARTESIAN_POINT ( 'NONE',  ( -4.999999999999999112, -73.79166666393547303, 2.886751345948131764 ) ) ;
#20377=CARTESIAN_POINT ( 'NONE',  ( -6.972266317189433020E-16, -15.12499999726881050, -5.000000000000000000 ) ) ;
#20378=CARTESIAN_POINT ( 'NONE',  ( 9.457646018065525792E-16, -81.31249999863440792, 5.148502694627439702 ) ) ;
#20381=CYLINDRICAL_SURFACE ( 'NONE', #50272, 5.000000000000000000 ) ;
#20382=CARTESIAN_POINT ( 'NONE',  ( 5.000000000000000000, -27.49999999999999645, -6.123233995736766282E-16 ) ) ;
#20386=ORIENTED_EDGE ( 'NONE', *, *, #34178, .F. ) ;
#20388=CARTESIAN_POINT ( 'NONE',  ( -2.500000000000000444, 23.95833333606451987, -4.330127018922193649 ) ) ;
#20391=VECTOR ( 'NONE', #16056, 1000.000000000000000 ) ;
#20394=CARTESIAN_POINT ( 'NONE',  ( -1.339745962155640457, 4.205341801261477386, 4.999999999999984901 ) ) ;
#20396=CARTESIAN_POINT ( 'NONE',  ( 6.123233995736766282E-16, 30.00000000000000000, -5.000000000000000000 ) ) ;
#20400=CARTESIAN_POINT ( 'NONE',  ( 4.458734125000001214, -19.89583333196773651, 2.574251347313718519 ) ) ;
#20404=EDGE_CURVE ( 'NONE', #57091, #29555, #36697, .T. ) ;
#20406=ORIENTED_EDGE ( 'NONE', *, *, #48721, .T. ) ;
#20409=EDGE_LOOP ( 'NONE', ( #56510, #17005, #2513, #60104 ) ) ;
#20414=ADVANCED_FACE ( 'NONE', ( #61784 ), #13522, .T. ) ;
#20417=CARTESIAN_POINT ( 'NONE',  ( 1.975475456537005874E-15, 15.25000000000000000, 5.000000000000000000 ) ) ;
#20419=VERTEX_POINT ( 'NONE', #22864 ) ;
#20420=LINE ( 'NONE', #19773, #2913 ) ;
#20421=EDGE_CURVE ( 'NONE', #26096, #19049, #56332, .T. ) ;
#20422=CARTESIAN_POINT ( 'NONE',  ( -3.152548672688508926E-16, 14.43750000136559386, -5.148502694627439702 ) ) ;
#20426=LINE ( 'NONE', #59993, #33611 ) ;
#20427=AXIS2_PLACEMENT_3D ( 'NONE', #46428, #38038, #37104 ) ;
#20429=CARTESIAN_POINT ( 'NONE',  ( -4.458734124999997661, -67.22916666530106511, 2.574251347313722516 ) ) ;
#20431=CARTESIAN_POINT ( 'NONE',  ( -4.458734124999999437, 17.60416666803225993, -2.574251347313719407 ) ) ;
#20434=CARTESIAN_POINT ( 'NONE',  ( 3.044556291839386294E-14, 17.75000000000000355, -5.000000000000000000 ) ) ;
#20436=CARTESIAN_POINT ( 'NONE',  ( 4.458734125000001214, -51.14583333196772941, 2.574251347313718519 ) ) ;
#20437=CARTESIAN_POINT ( 'NONE',  ( 5.000000000000000000, -10.29166666393547835, -2.886751345948129988 ) ) ;
#20438=CARTESIAN_POINT ( 'NONE',  ( -4.999999999999998224, -65.79166666393547303, 2.886751345948131764 ) ) ;
#20441=CARTESIAN_POINT ( 'NONE',  ( 4.458734124999998549, -13.97916666530107221, -2.574251347313721627 ) ) ;
#20442=ORIENTED_EDGE ( 'NONE', *, *, #47502, .T. ) ;
#20443=CARTESIAN_POINT ( 'NONE',  ( 1.339745962155612702, 23.70534180126148271, -5.000000000000000000 ) ) ;
#20444=CARTESIAN_POINT ( 'NONE',  ( -4.458734124999999437, -102.3124999986344079, 0.000000000000000000 ) ) ;
#20446=ORIENTED_EDGE ( 'NONE', *, *, #45342, .T. ) ;
#20447=CARTESIAN_POINT ( 'NONE',  ( 2.229367062500001939, -96.22916666530105090, 3.861377020970579999 ) ) ;
#20449=CARTESIAN_POINT ( 'NONE',  ( -2.500000000000000444, -58.04166666393548013, -4.330127018922193649 ) ) ;
#20453=EDGE_CURVE ( 'NONE', #19054, #1919, #41178, .T. ) ;
#20454=CARTESIAN_POINT ( 'NONE',  ( -4.458734124999999437, -16.39583333196773651, -2.574251347313719407 ) ) ;
#20455=CARTESIAN_POINT ( 'NONE',  ( -2.229367062500000163, 5.270833334698927786, -3.861377020970580443 ) ) ;
#20456=CARTESIAN_POINT ( 'NONE',  ( 2.229367062499998831, -64.89583333196773651, -3.861377020970580887 ) ) ;
#20458=LINE ( 'NONE', #40057, #54330 ) ;
#20460=CARTESIAN_POINT ( 'NONE',  ( -5.000000000000000000, -11.99999999999999645, 0.000000000000000000 ) ) ;
#20468=CARTESIAN_POINT ( 'NONE',  ( 2.499999999999998668, -93.33333333333332860, -4.330127018922193649 ) ) ;
#20472=CARTESIAN_POINT ( 'NONE',  ( 2.500000000000002220, -75.66666666666665719, 4.330127018922192761 ) ) ;
#20476=ORIENTED_EDGE ( 'NONE', *, *, #10323, .F. ) ;
#20477=VECTOR ( 'NONE', #46974, 1000.000000000000000 ) ;
#20478=DIRECTION ( 'NONE',  ( -0.000000000000000000, 1.000000000000000000, -0.000000000000000000 ) ) ;
#20480=VECTOR ( 'NONE', #47328, 1000.000000000000000 ) ;
#20483=EDGE_CURVE ( 'NONE', #34023, #19443, #61424, .T. ) ;
#20484=VERTEX_POINT ( 'NONE', #57281 ) ;
#20491=CARTESIAN_POINT ( 'NONE',  ( 9.457646018065525792E-16, -60.31249999863440792, 5.148502694627439702 ) ) ;
#20494=ORIENTED_EDGE ( 'NONE', *, *, #39203, .F. ) ;
#20498=ORIENTED_EDGE ( 'NONE', *, *, #47180, .F. ) ;
#20502=CARTESIAN_POINT ( 'NONE',  ( -4.458734124999999437, -108.6458333319677365, -2.574251347313719407 ) ) ;
#20504=ORIENTED_EDGE ( 'NONE', *, *, #62976, .F. ) ;
#20508=CARTESIAN_POINT ( 'NONE',  ( -2.229367062499996610, -43.14583333196773651, 3.861377020970582219 ) ) ;
#20513=CARTESIAN_POINT ( 'NONE',  ( -4.458734124999999437, -50.31249999863440792, 0.000000000000000000 ) ) ;
#20514=CARTESIAN_POINT ( 'NONE',  ( 2.499999999999998668, 29.66666666666666430, -4.330127018922193649 ) ) ;
#20515=CARTESIAN_POINT ( 'NONE',  ( 9.457646018065525792E-16, -16.06249999863440436, 5.148502694627439702 ) ) ;
#20516=CARTESIAN_POINT ( 'NONE',  ( -5.000000000000000000, -99.08333333333332860, -2.886751345948128211 ) ) ;
#20518=CARTESIAN_POINT ( 'NONE',  ( 2.229367062499998831, -32.89583333196773651, -3.861377020970580887 ) ) ;
#20519=CARTESIAN_POINT ( 'NONE',  ( -4.999999999999999112, 8.208333336064518093, 2.886751345948131764 ) ) ;
#20520=CARTESIAN_POINT ( 'NONE',  ( 5.000000000000000888, -50.58333333333332860, 2.886751345948126879 ) ) ;
#20524=LINE ( 'NONE', #34996, #15142 ) ;
#20525=FACE_OUTER_BOUND ( 'NONE', #32611, .T. ) ;
#20527=CARTESIAN_POINT ( 'NONE',  ( -3.152548672688508926E-16, -0.8124999986344056957, -5.148502694627439702 ) ) ;
#20528=ORIENTED_EDGE ( 'NONE', *, *, #8234, .T. ) ;
#20531=CARTESIAN_POINT ( 'NONE',  ( 4.458734124999999437, -88.81249999863439371, -5.460374474430324690E-16 ) ) ;
#20532=CARTESIAN_POINT ( 'NONE',  ( 9.457646018065525792E-16, -37.06249999863440792, 5.148502694627439702 ) ) ;
#20533=CARTESIAN_POINT ( 'NONE',  ( -6.972266317189433020E-16, -9.250000000000000000, -5.000000000000000000 ) ) ;
#20534=CARTESIAN_POINT ( 'NONE',  ( 4.458734124999998549, -78.97916666530106511, -2.574251347313721627 ) ) ;
#20539=CARTESIAN_POINT ( 'NONE',  ( 2.229367062500001939, 0.02083333469892964529, 3.861377020970579999 ) ) ;
#20540=CARTESIAN_POINT ( 'NONE',  ( -4.458734124999999437, 23.43750000136559564, 0.000000000000000000 ) ) ;
#20541=CARTESIAN_POINT ( 'NONE',  ( -4.458734124999999437, -48.56249999863440792, 0.000000000000000000 ) ) ;
#20548=CARTESIAN_POINT ( 'NONE',  ( -4.458734124999999437, -74.39583333196775072, -2.574251347313719407 ) ) ;
#20549=CARTESIAN_POINT ( 'NONE',  ( -2.500000000000000444, -110.0416666639354730, -4.330127018922193649 ) ) ;
#20553=CARTESIAN_POINT ( 'NONE',  ( -3.535250795749689387E-16, -60.25000000000000000, -5.773502691896257311 ) ) ;
#20554=CARTESIAN_POINT ( 'NONE',  ( -1.339745962155613812, -75.20534180126148271, -5.000000000000000000 ) ) ;
#20557=CYLINDRICAL_SURFACE ( 'NONE', #56119, 5.000000000000000000 ) ;
#20558=CARTESIAN_POINT ( 'NONE',  ( -5.000000000000000000, -99.08333333333332860, -2.886751345948128211 ) ) ;
#20567=ORIENTED_EDGE ( 'NONE', *, *, #47530, .F. ) ;
#20568=DIRECTION ( 'NONE',  ( 0.000000000000000000, 0.000000000000000000, 1.000000000000000000 ) ) ;
#20575=CARTESIAN_POINT ( 'NONE',  ( 4.458734124999999437, -45.06249999863440081, -5.460374474430324690E-16 ) ) ;
#20576=CARTESIAN_POINT ( 'NONE',  ( 1.975475456537005874E-15, -15.62499999726881406, 5.000000000000000000 ) ) ;
#20578=FACE_OUTER_BOUND ( 'NONE', #32518, .T. ) ;
#20579=AXIS2_PLACEMENT_3D ( 'NONE', #33816, #57960, #62787 ) ;
#20583=DIRECTION ( 'NONE',  ( -0.000000000000000000, 1.000000000000000000, -0.000000000000000000 ) ) ;
#20585=CARTESIAN_POINT ( 'NONE',  ( 4.458734124999998549, -94.97916666530106511, -2.574251347313721627 ) ) ;
#20595=CARTESIAN_POINT ( 'NONE',  ( 4.458734125000001214, 4.104166668032260823, 2.574251347313718519 ) ) ;
#20596=EDGE_CURVE ( 'NONE', #33989, #29077, #52285, .T. ) ;
#20598=CARTESIAN_POINT ( 'NONE',  ( -2.229367062500000163, -15.72916666530107399, -3.861377020970580443 ) ) ;
#20599=CARTESIAN_POINT ( 'NONE',  ( -5.000000000000000000, -101.0000000000000000, 0.000000000000000000 ) ) ;
#20603=CARTESIAN_POINT ( 'NONE',  ( 9.457646018065525792E-16, 14.68750000136559564, 5.148502694627439702 ) ) ;
#20605=DIRECTION ( 'NONE',  ( -0.000000000000000000, 1.000000000000000000, -0.000000000000000000 ) ) ;
#20606=LINE ( 'NONE', #40210, #29812 ) ;
#20607=CARTESIAN_POINT ( 'NONE',  ( 2.229367062499998831, -21.64583333196774007, -3.861377020970580887 ) ) ;
#20611=CARTESIAN_POINT ( 'NONE',  ( -5.000000000000000000, -47.95833333060214443, -2.886751345948128211 ) ) ;
#20613=CARTESIAN_POINT ( 'NONE',  ( 9.457646018065525792E-16, 14.93750000136559386, 5.148502694627439702 ) ) ;
#20616=CARTESIAN_POINT ( 'NONE',  ( -2.229367062500000163, -68.47916666530107932, -3.861377020970580443 ) ) ;
#20620=CARTESIAN_POINT ( 'NONE',  ( -3.535250795749689387E-16, 2.749999999999999112, -5.773502691896257311 ) ) ;
#20624=CARTESIAN_POINT ( 'NONE',  ( 2.229367062499998831, -56.64583333196773651, -3.861377020970580887 ) ) ;
#20625=CARTESIAN_POINT ( 'NONE',  ( -3.535250795749689387E-16, -91.12499999726878741, -5.773502691896257311 ) ) ;
#20626=CARTESIAN_POINT ( 'NONE',  ( -3.152548672688508926E-16, -34.56249999863440792, -5.148502694627439702 ) ) ;
#20627=CARTESIAN_POINT ( 'NONE',  ( 0.000000000000000000, -120.0000000000000000, 0.000000000000000000 ) ) ;
#20628=CYLINDRICAL_SURFACE ( 'NONE', #4954, 5.000000000000000000 ) ;
#20630=CARTESIAN_POINT ( 'NONE',  ( 5.000000000000000000, 1.500000000000001332, -6.123233995736766282E-16 ) ) ;
#20632=CARTESIAN_POINT ( 'NONE',  ( -2.500000000000000444, -45.16666666666665719, -4.330127018922193649 ) ) ;
#20634=CARTESIAN_POINT ( 'NONE',  ( 5.000000000000000888, -86.45833333060213022, 2.886751345948126879 ) ) ;
#20635=EDGE_LOOP ( 'NONE', ( #35273, #46789, #54960, #20386 ) ) ;
#20636=CARTESIAN_POINT ( 'NONE',  ( -4.458734124999998549, -107.2291666653010509, 2.574251347313722516 ) ) ;
#20637=CARTESIAN_POINT ( 'NONE',  ( -3.152548672688508926E-16, 3.187500001365594748, -5.148502694627439702 ) ) ;
#20638=CARTESIAN_POINT ( 'NONE',  ( 1.975475456537005874E-15, -96.62499999726880162, 5.000000000000000000 ) ) ;
#20647=CARTESIAN_POINT ( 'NONE',  ( -6.972266317189433020E-16, -5.249999999999998224, -5.000000000000000000 ) ) ;
#20648=CARTESIAN_POINT ( 'NONE',  ( 5.000000000000000000, -6.416666666666667851, -2.886751345948130876 ) ) ;
#20649=ORIENTED_EDGE ( 'NONE', *, *, #53861, .F. ) ;
#20650=LINE ( 'NONE', #45721, #27859 ) ;
#20653=CARTESIAN_POINT ( 'NONE',  ( -4.458734124999998549, -31.47916666530107221, 2.574251347313722516 ) ) ;
#20654=DIRECTION ( 'NONE',  ( 0.000000000000000000, 0.000000000000000000, 1.000000000000000000 ) ) ;
#20660=VERTEX_POINT ( 'NONE', #30010 ) ;
#20663=CARTESIAN_POINT ( 'NONE',  ( 4.458734125000001214, -78.14583333196775072, 2.574251347313718519 ) ) ;
#20665=EDGE_LOOP ( 'NONE', ( #17645, #24358, #60274, #42497 ) ) ;
#20666=CARTESIAN_POINT ( 'NONE',  ( 0.000000000000000000, -120.0000000000000000, 5.000000000000000000 ) ) ;
#20670=CARTESIAN_POINT ( 'NONE',  ( 9.457646018065525792E-16, -3.312499998634407472, 5.148502694627439702 ) ) ;
#20673=DIRECTION ( 'NONE',  ( -0.000000000000000000, 1.000000000000000000, -0.000000000000000000 ) ) ;
#20676=CARTESIAN_POINT ( 'NONE',  ( 5.000000000000000000, -47.29166666393547303, -2.886751345948130876 ) ) ;
#20678=CARTESIAN_POINT ( 'NONE',  ( 0.000000000000000000, -120.0000000000000000, 0.000000000000000000 ) ) ;
#20679=ORIENTED_EDGE ( 'NONE', *, *, #54526, .F. ) ;
#20680=CARTESIAN_POINT ( 'NONE',  ( 4.458734124999999437, -81.81249999863440792, -5.460374474430324690E-16 ) ) ;
#20681=DIRECTION ( 'NONE',  ( 0.000000000000000000, 0.000000000000000000, 1.000000000000000000 ) ) ;
#20682=CARTESIAN_POINT ( 'NONE',  ( 4.458734125000001214, -1.895833331967737623, 2.574251347313718519 ) ) ;
#20685=CARTESIAN_POINT ( 'NONE',  ( 4.458734124999998549, -68.97916666530106511, -2.574251347313721627 ) ) ;
#20686=CARTESIAN_POINT ( 'NONE',  ( -2.500000000000000444, -28.04166666393548013, -4.330127018922193649 ) ) ;
#20689=CARTESIAN_POINT ( 'NONE',  ( -1.339745962155610925, -3.794658198738523058, 5.000000000000000000 ) ) ;
#20692=CARTESIAN_POINT ( 'NONE',  ( 4.458734124999998549, -43.72916666530106511, -2.574251347313721627 ) ) ;
#20693=CARTESIAN_POINT ( 'NONE',  ( -2.229367062500000163, -30.72916666530107221, -3.861377020970580443 ) ) ;
#20696=CARTESIAN_POINT ( 'NONE',  ( 1.060575238724906964E-15, 18.24999999999999645, 5.773502691896257311 ) ) ;
#20699=EDGE_CURVE ( 'NONE', #33480, #55181, #59946, .T. ) ;
#20700=CARTESIAN_POINT ( 'NONE',  ( -4.458734124999999437, -42.31249999863440081, 0.000000000000000000 ) ) ;
#20701=CARTESIAN_POINT ( 'NONE',  ( 5.000000000000000888, -74.45833333060214443, 2.886751345948126879 ) ) ;
#20705=CARTESIAN_POINT ( 'NONE',  ( -4.458734124999999437, -79.56249999863440792, 0.000000000000000000 ) ) ;
#20709=CARTESIAN_POINT ( 'NONE',  ( 5.000000000000000000, -26.41666666666666430, -2.886751345948129988 ) ) ;
#20715=CARTESIAN_POINT ( 'NONE',  ( 5.000000000000000888, 21.54166666939785202, 2.886751345948126879 ) ) ;
#20720=CARTESIAN_POINT ( 'NONE',  ( 1.975475456537005874E-15, -6.749999999999999112, 5.000000000000000000 ) ) ;
#20721=CARTESIAN_POINT ( 'NONE',  ( 2.500000000000002220, 15.45833333606451987, 4.330127018922192761 ) ) ;
#20722=CARTESIAN_POINT ( 'NONE',  ( -1.339745962155613812, -62.20534180126146850, -5.000000000000000000 ) ) ;
#20724=CARTESIAN_POINT ( 'NONE',  ( -3.152548672688508926E-16, -15.81249999863440436, -5.148502694627439702 ) ) ;
#20729=ORIENTED_EDGE ( 'NONE', *, *, #19746, .T. ) ;
#20730=DIRECTION ( 'NONE',  ( -0.000000000000000000, 1.000000000000000000, -0.000000000000000000 ) ) ;
#20732=ORIENTED_EDGE ( 'NONE', *, *, #61016, .F. ) ;
#20733=CARTESIAN_POINT ( 'NONE',  ( -2.500000000000000444, -86.16666666666667140, -4.330127018922193649 ) ) ;
#20735=ORIENTED_EDGE ( 'NONE', *, *, #61016, .T. ) ;
#20736=( BOUNDED_CURVE ( )  B_SPLINE_CURVE ( 2, ( #8644, #57553, #46947, #37921, #3515, #38241, #13156, #8960, #53019 ),
 .UNSPECIFIED., .F., .F. ) 
 B_SPLINE_CURVE_WITH_KNOTS ( ( 3, 2, 2, 2, 3 ),
 ( 0.4553571428571428492, 0.4559523809523809423, 0.4571428571428571286, 0.4583333333333333148, 0.4589285714285714080 ),
 .UNSPECIFIED. ) 
 CURVE ( )  GEOMETRIC_REPRESENTATION_ITEM ( )  RATIONAL_B_SPLINE_CURVE ( ( 0.9330127018922194093, 0.9330127018922194093, 1.000000000000000000, 0.8660254037844387076, 1.000000000000000000, 0.8660254037844387076, 1.000000000000000000, 0.9330127018922194093, 0.9330127018922194093 ) ) 
 REPRESENTATION_ITEM ( '' )  );
#20742=CARTESIAN_POINT ( 'NONE',  ( -6.972266317189433020E-16, -87.12499999726880162, -5.000000000000000000 ) ) ;
#20743=CARTESIAN_POINT ( 'NONE',  ( -4.458734124999999437, 15.60416666803225993, -2.574251347313719407 ) ) ;
#20747=LINE ( 'NONE', #26523, #36701 ) ;
#20748=CARTESIAN_POINT ( 'NONE',  ( 4.458734124999999437, -66.81249999863440792, -5.460374474430324690E-16 ) ) ;
#20750=CARTESIAN_POINT ( 'NONE',  ( 4.458734125000001214, 17.10416666803225993, 2.574251347313718519 ) ) ;
#20752=CYLINDRICAL_SURFACE ( 'NONE', #1862, 5.000000000000000000 ) ;
#20753=CARTESIAN_POINT ( 'NONE',  ( 2.229367062499998831, -52.89583333196773651, -3.861377020970580887 ) ) ;
#20754=CARTESIAN_POINT ( 'NONE',  ( -3.535250795749689387E-16, -11.12499999726881761, -5.773502691896257311 ) ) ;
#20756=LINE ( 'NONE', #40362, #18337 ) ;
#20759=CARTESIAN_POINT ( 'NONE',  ( -2.229367062499996610, -14.39583333196774184, 3.861377020970582219 ) ) ;
#20762=CARTESIAN_POINT ( 'NONE',  ( 4.458734125000001214, -103.8958333319677365, 2.574251347313718519 ) ) ;
#20764=VERTEX_POINT ( 'NONE', #50277 ) ;
#20765=CARTESIAN_POINT ( 'NONE',  ( -4.458734124999999437, -96.64583333196773651, -2.574251347313719407 ) ) ;
#20768=CARTESIAN_POINT ( 'NONE',  ( -5.000000000000000000, -56.87499999726880162, 0.000000000000000000 ) ) ;
#20772=CARTESIAN_POINT ( 'NONE',  ( 4.458734125000000326, -22.89583333196773651, 2.574251347313718519 ) ) ;
#20773=CARTESIAN_POINT ( 'NONE',  ( 2.229367062499998831, 6.104166668032262599, -3.861377020970580887 ) ) ;
#20774=CARTESIAN_POINT ( 'NONE',  ( -3.152548672688508926E-16, -62.81249999863440792, -5.148502694627439702 ) ) ;
#20775=CARTESIAN_POINT ( 'NONE',  ( 2.499999999999998668, -94.20833333060213022, -4.330127018922193649 ) ) ;
#20777=FACE_OUTER_BOUND ( 'NONE', #52687, .T. ) ;
#20779=CARTESIAN_POINT ( 'NONE',  ( -2.499999999999996447, -13.83333333333333570, 4.330127018922195425 ) ) ;
#20781=EDGE_LOOP ( 'NONE', ( #45047, #53086, #33997, #2462 ) ) ;
#20783=CARTESIAN_POINT ( 'NONE',  ( -1.339745962155613812, -38.20534180126147561, -5.000000000000000000 ) ) ;
#20784=CARTESIAN_POINT ( 'NONE',  ( 1.339745962155612702, -38.16965819600732601, -5.000000000000000000 ) ) ;
#20787=EDGE_CURVE ( 'NONE', #14134, #35143, #23536, .T. ) ;
#20788=DIRECTION ( 'NONE',  ( -0.000000000000000000, 1.000000000000000000, -0.000000000000000000 ) ) ;
#20791=CARTESIAN_POINT ( 'NONE',  ( 1.975475456537005874E-15, 20.37500000273118417, 5.000000000000000000 ) ) ;
#20793=CARTESIAN_POINT ( 'NONE',  ( -5.000000000000000000, -75.00000000000000000, 0.000000000000000000 ) ) ;
#20796=CARTESIAN_POINT ( 'NONE',  ( -1.339745962155610925, -97.79465819873851729, 5.000000000000000000 ) ) ;
#20798=CARTESIAN_POINT ( 'NONE',  ( -5.000000000000000000, -53.95833333060214443, -2.886751345948128211 ) ) ;
#20804=ORIENTED_EDGE ( 'NONE', *, *, #57825, .F. ) ;
#20808=CARTESIAN_POINT ( 'NONE',  ( 5.000000000000000000, -55.41666666666667140, -2.886751345948130876 ) ) ;
#20812=DIRECTION ( 'NONE',  ( -0.000000000000000000, 1.000000000000000000, -0.000000000000000000 ) ) ;
#20817=EDGE_CURVE ( 'NONE', #33932, #38122, #16816, .T. ) ;
#20818=CARTESIAN_POINT ( 'NONE',  ( 4.458734124999998549, -77.72916666530106511, -2.574251347313721627 ) ) ;
#20819=CARTESIAN_POINT ( 'NONE',  ( -4.458734124999999437, 29.68750000136559208, 0.000000000000000000 ) ) ;
#20825=CARTESIAN_POINT ( 'NONE',  ( 2.229367062500001939, -42.97916666530107932, 3.861377020970579999 ) ) ;
#20828=CARTESIAN_POINT ( 'NONE',  ( -2.229367062500000163, -47.47916666530106511, -3.861377020970580443 ) ) ;
#20830=CARTESIAN_POINT ( 'NONE',  ( -6.031010364368858512E-14, 2.375000002731183280, 5.000000000000000000 ) ) ;
#20831=CARTESIAN_POINT ( 'NONE',  ( 2.229367062499998831, -17.64583333196773651, -3.861377020970580887 ) ) ;
#20832=CARTESIAN_POINT ( 'NONE',  ( -2.499999999999996447, -101.8333333333333286, 4.330127018922195425 ) ) ;
#20835=CARTESIAN_POINT ( 'NONE',  ( -3.152548672688508926E-16, -35.81249999863440792, -5.148502694627439702 ) ) ;
#20836=CARTESIAN_POINT ( 'NONE',  ( -5.000000000000000000, 4.041666669397852019, -2.886751345948128211 ) ) ;
#20841=CARTESIAN_POINT ( 'NONE',  ( -2.229367062499996610, -0.3958333319677397322, 3.861377020970582219 ) ) ;
#20842=ORIENTED_EDGE ( 'NONE', *, *, #35105, .F. ) ;
#20845=CARTESIAN_POINT ( 'NONE',  ( -2.229367062499996610, -86.14583333196773651, 3.861377020970582219 ) ) ;
#20846=CARTESIAN_POINT ( 'NONE',  ( 4.458734124999998549, -34.72916666530107221, -2.574251347313721627 ) ) ;
#20848=CARTESIAN_POINT ( 'NONE',  ( 9.457646018065525792E-16, -81.31249999863440792, 5.148502694627439702 ) ) ;
#20855=CARTESIAN_POINT ( 'NONE',  ( -3.152548672688508926E-16, -8.562499998634406140, -5.148502694627439702 ) ) ;
#20856=CARTESIAN_POINT ( 'NONE',  ( -4.458734124999999437, 21.43750000136559208, 0.000000000000000000 ) ) ;
#20857=CARTESIAN_POINT ( 'NONE',  ( 2.229367062499998831, -48.89583333196772941, -3.861377020970580887 ) ) ;
#20858=CARTESIAN_POINT ( 'NONE',  ( 5.000000000000000000, -11.41666666666666607, -2.886751345948130876 ) ) ;
#20861=VERTEX_POINT ( 'NONE', #17137 ) ;
#20864=CARTESIAN_POINT ( 'NONE',  ( -4.458734124999999437, -77.31249999863440792, 0.000000000000000000 ) ) ;
#20865=CARTESIAN_POINT ( 'NONE',  ( 5.000000000000000000, -109.3749999972688016, -6.123233995736766282E-16 ) ) ;
#20871=CARTESIAN_POINT ( 'NONE',  ( -2.499999999999996447, -57.83333333333333570, 4.330127018922195425 ) ) ;
#20876=CARTESIAN_POINT ( 'NONE',  ( 1.975475456537005874E-15, -71.75000000000000000, 5.000000000000000000 ) ) ;
#20882=ORIENTED_EDGE ( 'NONE', *, *, #19667, .F. ) ;
#20884=CARTESIAN_POINT ( 'NONE',  ( 1.975475456537005874E-15, -59.62499999726880873, 5.000000000000000000 ) ) ;
#20890=CARTESIAN_POINT ( 'NONE',  ( -2.229367062499996610, -48.39583333196772941, 3.861377020970582219 ) ) ;
#20891=CARTESIAN_POINT ( 'NONE',  ( -5.000000000000000000, -15.87499999726881406, 0.000000000000000000 ) ) ;
#20892=( BOUNDED_CURVE ( )  B_SPLINE_CURVE ( 2, ( #12300, #62468, #22915, #7479, #2654, #62145, #31916, #51543, #27092 ),
 .UNSPECIFIED., .F., .F. ) 
 B_SPLINE_CURVE_WITH_KNOTS ( ( 3, 2, 2, 2, 3 ),
 ( 0.2660714285714285698, 0.2666666666666666630, 0.2678571428571428492, 0.2690476190476190355, 0.2696428571428571286 ),
 .UNSPECIFIED. ) 
 CURVE ( )  GEOMETRIC_REPRESENTATION_ITEM ( )  RATIONAL_B_SPLINE_CURVE ( ( 0.9330127018922194093, 0.9330127018922194093, 1.000000000000000000, 0.8660254037844387076, 1.000000000000000000, 0.8660254037844387076, 1.000000000000000000, 0.9330127018922194093, 0.9330127018922194093 ) ) 
 REPRESENTATION_ITEM ( '' )  );
#20894=CARTESIAN_POINT ( 'NONE',  ( -5.000000000000000000, -56.87499999726880162, 0.000000000000000000 ) ) ;
#20898=CYLINDRICAL_SURFACE ( 'NONE', #10876, 5.000000000000000000 ) ;
#20900=CARTESIAN_POINT ( 'NONE',  ( -4.458734124999998549, -92.47916666530106511, 2.574251347313722516 ) ) ;
#20901=LINE ( 'NONE', #25076, #49210 ) ;
#20902=EDGE_LOOP ( 'NONE', ( #59211, #41996, #47233, #41675 ) ) ;
#20903=CARTESIAN_POINT ( 'NONE',  ( 0.000000000000000000, -120.0000000000000000, 0.000000000000000000 ) ) ;
#20907=EDGE_LOOP ( 'NONE', ( #7145, #25939, #45988, #56561 ) ) ;
#20908=CARTESIAN_POINT ( 'NONE',  ( -2.229367062500000163, -4.479166665301070438, -3.861377020970580443 ) ) ;
#20909=CARTESIAN_POINT ( 'NONE',  ( 5.000000000000000888, -1.458333330602148870, 2.886751345948126879 ) ) ;
#20910=CARTESIAN_POINT ( 'NONE',  ( 4.458734124999999437, -16.06249999863440436, -5.460374474430324690E-16 ) ) ;
#20911=CARTESIAN_POINT ( 'NONE',  ( 1.975475456537005874E-15, -100.6249999972688016, 5.000000000000000000 ) ) ;
#20915=( BOUNDED_CURVE ( )  B_SPLINE_CURVE ( 2, ( #20316, #39917, #3077, #3392, #42293, #37794, #52275, #37475, #17550 ),
 .UNSPECIFIED., .F., .F. ) 
 B_SPLINE_CURVE_WITH_KNOTS ( ( 3, 2, 2, 2, 3 ),
 ( 0.7982142857142857650, 0.7988095238095238582, 0.8000000000000000444, 0.8011904761904762307, 0.8017857142857143238 ),
 .UNSPECIFIED. ) 
 CURVE ( )  GEOMETRIC_REPRESENTATION_ITEM ( )  RATIONAL_B_SPLINE_CURVE ( ( 0.9330127018922194093, 0.9330127018922194093, 1.000000000000000000, 0.8660254037844387076, 1.000000000000000000, 0.8660254037844387076, 1.000000000000000000, 0.9330127018922194093, 0.9330127018922194093 ) ) 
 REPRESENTATION_ITEM ( '' )  );
#20916=CARTESIAN_POINT ( 'NONE',  ( -4.458734124999999437, 16.43750000136559564, 0.000000000000000000 ) ) ;
#20917=VERTEX_POINT ( 'NONE', #41245 ) ;
#20919=CARTESIAN_POINT ( 'NONE',  ( -6.972266317189433020E-16, -71.12499999726878741, -5.000000000000000000 ) ) ;
#20920=CARTESIAN_POINT ( 'NONE',  ( -2.229367062500000163, -17.47916666530106866, -3.861377020970580443 ) ) ;
#20921=CARTESIAN_POINT ( 'NONE',  ( 1.975475456537005874E-15, -80.74999999999998579, 5.000000000000000000 ) ) ;
#20925=CARTESIAN_POINT ( 'NONE',  ( -2.500000000000000444, -49.04166666393547303, -4.330127018922193649 ) ) ;
#20926=CARTESIAN_POINT ( 'NONE',  ( -5.000000000000000000, 21.04166666939784847, -2.886751345948128211 ) ) ;
#20927=CARTESIAN_POINT ( 'NONE',  ( -2.229367062500000163, 15.52083333469892779, -3.861377020970580443 ) ) ;
#20928=CARTESIAN_POINT ( 'NONE',  ( 5.000000000000000000, -35.41666666666666430, -2.886751345948130876 ) ) ;
#20931=CARTESIAN_POINT ( 'NONE',  ( 2.229367062500001939, -65.97916666530106511, 3.861377020970579999 ) ) ;
#20934=CARTESIAN_POINT ( 'NONE',  ( -2.499999999999996447, 4.166666666666666075, 4.330127018922195425 ) ) ;
#20936=CARTESIAN_POINT ( 'NONE',  ( -2.500000000000000444, 21.83333333333333215, -4.330127018922193649 ) ) ;
#20937=CARTESIAN_POINT ( 'NONE',  ( 4.458734124999998549, -56.72916666530107932, -2.574251347313721627 ) ) ;
#20938=CARTESIAN_POINT ( 'NONE',  ( -5.000000000000000000, -95.87499999726881583, 0.000000000000000000 ) ) ;
#20939=CARTESIAN_POINT ( 'NONE',  ( 4.458734124999998549, -32.72916666530106511, -2.574251347313721627 ) ) ;
#20941=EDGE_CURVE ( 'NONE', #60646, #41255, #8329, .T. ) ;
#20942=CARTESIAN_POINT ( 'NONE',  ( -2.500000000000000444, -42.04166666393548013, -4.330127018922193649 ) ) ;
#20946=CARTESIAN_POINT ( 'NONE',  ( -4.999999999999998224, -48.91666666666666430, 2.886751345948131764 ) ) ;
#20948=CARTESIAN_POINT ( 'NONE',  ( -5.000000000000000000, -40.99999999999999289, 0.000000000000000000 ) ) ;
#20949=CARTESIAN_POINT ( 'NONE',  ( 1.975475456537005874E-15, -53.74999999999999289, 5.000000000000000000 ) ) ;
#20952=CARTESIAN_POINT ( 'NONE',  ( -2.229367062499996610, -107.1458333319677365, 3.861377020970582219 ) ) ;
#20953=CARTESIAN_POINT ( 'NONE',  ( 9.457646018065525792E-16, -2.312499998634407028, 5.148502694627439702 ) ) ;
#20954=CARTESIAN_POINT ( 'NONE',  ( -6.972266317189433020E-16, -97.12499999726880162, -5.000000000000000000 ) ) ;
#20955=ADVANCED_FACE ( 'NONE', ( #53436 ), #47975, .T. ) ;
#20959=EDGE_CURVE ( 'NONE', #32214, #54588, #45321, .T. ) ;
#20964=DIRECTION ( 'NONE',  ( -0.000000000000000000, 1.000000000000000000, -0.000000000000000000 ) ) ;
#20969=CARTESIAN_POINT ( 'NONE',  ( 4.458734124999998549, -32.97916666530106511, -2.574251347313721627 ) ) ;
#20975=VERTEX_POINT ( 'NONE', #58584 ) ;
#20976=CARTESIAN_POINT ( 'NONE',  ( -2.500000000000000444, -83.04166666393547303, -4.330127018922193649 ) ) ;
#20977=ORIENTED_EDGE ( 'NONE', *, *, #19667, .T. ) ;
#20978=CARTESIAN_POINT ( 'NONE',  ( 4.458734124999998549, -76.97916666530106511, -2.574251347313721627 ) ) ;
#20981=CARTESIAN_POINT ( 'NONE',  ( 2.500000000000002220, -16.66666666666666430, 4.330127018922192761 ) ) ;
#20982=CARTESIAN_POINT ( 'NONE',  ( 0.000000000000000000, -120.0000000000000000, 0.000000000000000000 ) ) ;
#20984=CARTESIAN_POINT ( 'NONE',  ( -4.458734124999999437, -4.562499998634401699, 0.000000000000000000 ) ) ;
#20985=ORIENTED_EDGE ( 'NONE', *, *, #20421, .T. ) ;
#20987=CARTESIAN_POINT ( 'NONE',  ( -6.972266317189433020E-16, -27.24999999999999645, -5.000000000000000000 ) ) ;
#20991=DIRECTION ( 'NONE',  ( 0.000000000000000000, 0.000000000000000000, 1.000000000000000000 ) ) ;
#20992=ORIENTED_EDGE ( 'NONE', *, *, #18947, .T. ) ;
#20993=CARTESIAN_POINT ( 'NONE',  ( -2.229367062499996610, -82.14583333196773651, 3.861377020970582219 ) ) ;
#20995=CARTESIAN_POINT ( 'NONE',  ( -4.458734124999999437, -4.395833331967740065, -2.574251347313719407 ) ) ;
#20998=CARTESIAN_POINT ( 'NONE',  ( 4.458734124999998549, -70.97916666530107932, -2.574251347313721627 ) ) ;
#20999=CARTESIAN_POINT ( 'NONE',  ( -3.535250795749689387E-16, -30.12499999726881228, -5.773502691896257311 ) ) ;
#21000=CARTESIAN_POINT ( 'NONE',  ( -6.972266317189433020E-16, -15.25000000000000000, -5.000000000000000000 ) ) ;
#21002=CARTESIAN_POINT ( 'NONE',  ( -5.000000000000000000, -56.08333333333332860, -2.886751345948128211 ) ) ;
#21004=CARTESIAN_POINT ( 'NONE',  ( -4.458734124999998549, -53.22916666530107932, 2.574251347313722516 ) ) ;
#21006=CARTESIAN_POINT ( 'NONE',  ( -2.229367062500000163, -31.72916666530107577, -3.861377020970580443 ) ) ;
#21008=CARTESIAN_POINT ( 'NONE',  ( 2.500000000000002220, 19.33333333333333570, 4.330127018922192761 ) ) ;
#21010=DIRECTION ( 'NONE',  ( -0.000000000000000000, 1.000000000000000000, -0.000000000000000000 ) ) ;
#21011=CARTESIAN_POINT ( 'NONE',  ( 2.229367062499998831, -42.64583333196773651, -3.861377020970580887 ) ) ;
#21012=CARTESIAN_POINT ( 'NONE',  ( -4.999999999999999112, -79.79166666393545881, 2.886751345948131764 ) ) ;
#21016=CARTESIAN_POINT ( 'NONE',  ( -6.972266317189433020E-16, -59.12499999726880873, -5.000000000000000000 ) ) ;
#21017=CARTESIAN_POINT ( 'NONE',  ( 2.229367062499998831, -79.89583333196773651, -3.861377020970580887 ) ) ;
#21019=CARTESIAN_POINT ( 'NONE',  ( 1.464175926609780648E-14, 21.87500000273118062, -5.000000000000000000 ) ) ;
#21020=CARTESIAN_POINT ( 'NONE',  ( -2.499999999999996447, -26.83333333333333570, 4.330127018922195425 ) ) ;
#21026=CARTESIAN_POINT ( 'NONE',  ( 5.000000000000000888, 23.54166666939785202, 2.886751345948126879 ) ) ;
#21027=CARTESIAN_POINT ( 'NONE',  ( -6.972266317189433020E-16, -61.12499999726880162, -5.000000000000000000 ) ) ;
#21032=AXIS2_PLACEMENT_3D ( 'NONE', #40846, #26065, #21881 ) ;
#21033=ADVANCED_FACE ( 'NONE', ( #3929 ), #23547, .T. ) ;
#21035=DIRECTION ( 'NONE',  ( 0.000000000000000000, 0.000000000000000000, 1.000000000000000000 ) ) ;
#21036=CARTESIAN_POINT ( 'NONE',  ( 1.339745962155612702, -11.16965819600733667, -5.000000000000000000 ) ) ;
#21038=DIRECTION ( 'NONE',  ( -0.000000000000000000, 1.000000000000000000, -0.000000000000000000 ) ) ;
#21040=CARTESIAN_POINT ( 'NONE',  ( 2.229367062500001939, -14.22916666530107221, 3.861377020970579999 ) ) ;
#21045=AXIS2_PLACEMENT_3D ( 'NONE', #36871, #12424, #36546 ) ;
#21049=ORIENTED_EDGE ( 'NONE', *, *, #54696, .T. ) ;
#21050=CARTESIAN_POINT ( 'NONE',  ( 2.499999999999998668, -58.33333333333333570, -4.330127018922193649 ) ) ;
#21053=CARTESIAN_POINT ( 'NONE',  ( -2.500000000000000444, -10.16666666666666430, -4.330127018922193649 ) ) ;
#21058=CARTESIAN_POINT ( 'NONE',  ( 5.000000000000000000, 11.50000000000000000, -6.123233995736766282E-16 ) ) ;
#21059=CARTESIAN_POINT ( 'NONE',  ( -2.229367062499996610, 15.85416666803226171, 3.861377020970582219 ) ) ;
#21060=( BOUNDED_CURVE ( )  B_SPLINE_CURVE ( 2, ( #43967, #8328, #63294, #28556, #62360, #19533, #38829, #39147, #13766 ),
 .UNSPECIFIED., .F., .F. ) 
 B_SPLINE_CURVE_WITH_KNOTS ( ( 3, 2, 2, 2, 3 ),
 ( 0.6982142857142856762, 0.6988095238095237693, 0.6999999999999999556, 0.7011904761904761418, 0.7017857142857142350 ),
 .UNSPECIFIED. ) 
 CURVE ( )  GEOMETRIC_REPRESENTATION_ITEM ( )  RATIONAL_B_SPLINE_CURVE ( ( 0.9330127018922194093, 0.9330127018922194093, 1.000000000000000000, 0.8660254037844387076, 1.000000000000000000, 0.8660254037844387076, 1.000000000000000000, 0.9330127018922194093, 0.9330127018922194093 ) ) 
 REPRESENTATION_ITEM ( '' )  );
#21063=DIRECTION ( 'NONE',  ( -0.000000000000000000, 1.000000000000000000, -0.000000000000000000 ) ) ;
#21064=DIRECTION ( 'NONE',  ( -0.000000000000000000, 1.000000000000000000, -0.000000000000000000 ) ) ;
#21065=ORIENTED_EDGE ( 'NONE', *, *, #32650, .F. ) ;
#21066=CARTESIAN_POINT ( 'NONE',  ( -2.229367062500000163, -63.47916666530106511, -3.861377020970580443 ) ) ;
#21068=CARTESIAN_POINT ( 'NONE',  ( 4.458734124999998549, 12.27083333469892423, -2.574251347313721627 ) ) ;
#21069=CARTESIAN_POINT ( 'NONE',  ( 1.339745962155612702, -60.16965819600731891, -5.000000000000000000 ) ) ;
#21071=CARTESIAN_POINT ( 'NONE',  ( -2.229367062500000163, -56.72916666530107221, -3.861377020970580443 ) ) ;
#21072=CARTESIAN_POINT ( 'NONE',  ( 5.000000000000000000, -16.29166666393548368, -2.886751345948129988 ) ) ;
#21075=CARTESIAN_POINT ( 'NONE',  ( -6.972266317189433020E-16, -10.24999999999999822, -5.000000000000000000 ) ) ;
#21077=CARTESIAN_POINT ( 'NONE',  ( -4.458734124999999437, -15.64583333196773829, -2.574251347313719407 ) ) ;
#21080=CARTESIAN_POINT ( 'NONE',  ( 4.458734125000001214, -104.8958333319677365, 2.574251347313718519 ) ) ;
#21082=ORIENTED_EDGE ( 'NONE', *, *, #33847, .T. ) ;
#21083=CARTESIAN_POINT ( 'NONE',  ( -2.229367062499996610, -101.3958333319677365, 3.861377020970582219 ) ) ;
#21084=CARTESIAN_POINT ( 'NONE',  ( -4.458734124999999437, -26.39583333196773651, -2.574251347313719407 ) ) ;
#21085=CARTESIAN_POINT ( 'NONE',  ( 2.499999999999998668, -57.20833333060214443, -4.330127018922193649 ) ) ;
#21089=CARTESIAN_POINT ( 'NONE',  ( -4.458734124999999437, -22.31249999863440436, 0.000000000000000000 ) ) ;
#21090=CARTESIAN_POINT ( 'NONE',  ( -4.458734124999999437, -63.64583333196773651, -2.574251347313719407 ) ) ;
#21091=CARTESIAN_POINT ( 'NONE',  ( 1.339745962155615144, 8.294658198738519062, 4.999999999999999112 ) ) ;
#21095=CARTESIAN_POINT ( 'NONE',  ( -2.499999999999996447, -12.83333333333333570, 4.330127018922195425 ) ) ;
#21099=CARTESIAN_POINT ( 'NONE',  ( -2.500000000000000444, -38.16666666666667140, -4.330127018922193649 ) ) ;
#21104=DIRECTION ( 'NONE',  ( 0.000000000000000000, 0.000000000000000000, 1.000000000000000000 ) ) ;
#21106=CARTESIAN_POINT ( 'NONE',  ( 5.000000000000000000, -79.41666666666665719, -2.886751345948129988 ) ) ;
#21109=CARTESIAN_POINT ( 'NONE',  ( 1.975475456537005874E-15, -97.74999999999998579, 5.000000000000000000 ) ) ;
#21112=CARTESIAN_POINT ( 'NONE',  ( -4.999999999999998224, -53.79166666393548013, 2.886751345948131764 ) ) ;
#21129=VECTOR ( 'NONE', #4752, 1000.000000000000000 ) ;
#21130=CARTESIAN_POINT ( 'NONE',  ( -4.458734124999999437, -79.39583333196773651, -2.574251347313719407 ) ) ;
#21131=CARTESIAN_POINT ( 'NONE',  ( 2.229367062499998831, -107.8958333319677365, -3.861377020970580887 ) ) ;
#21132=CARTESIAN_POINT ( 'NONE',  ( 1.975475456537005874E-15, 20.24999999999999289, 5.000000000000000000 ) ) ;
#21133=ORIENTED_EDGE ( 'NONE', *, *, #62637, .T. ) ;
#21138=CARTESIAN_POINT ( 'NONE',  ( -4.458734124999997661, -44.22916666530106511, 2.574251347313722516 ) ) ;
#21141=CARTESIAN_POINT ( 'NONE',  ( -3.152548672688508926E-16, -47.56249999863442213, -5.148502694627439702 ) ) ;
#21144=CARTESIAN_POINT ( 'NONE',  ( 4.458734125000001214, -15.89583333196773651, 2.574251347313718519 ) ) ;
#21145=CARTESIAN_POINT ( 'NONE',  ( 5.000000000000000000, -99.41666666666664298, -2.886751345948129988 ) ) ;
#21146=EDGE_CURVE ( 'NONE', #969, #15028, #1765, .T. ) ;
#21148=CARTESIAN_POINT ( 'NONE',  ( -4.458734124999999437, -40.56249999863440081, 0.000000000000000000 ) ) ;
#21149=CARTESIAN_POINT ( 'NONE',  ( 5.000000000000000000, 1.625000002731184834, -6.123233995736766282E-16 ) ) ;
#21150=CARTESIAN_POINT ( 'NONE',  ( -2.499999999999996447, -6.708333330602149758, 4.330127018922195425 ) ) ;
#21154=CARTESIAN_POINT ( 'NONE',  ( -4.458734124999997661, 0.5208333346989266754, 2.574251347313722516 ) ) ;
#21156=CARTESIAN_POINT ( 'NONE',  ( -6.972266317189433020E-16, -48.24999999999999289, -5.000000000000000000 ) ) ;
#21157=CARTESIAN_POINT ( 'NONE',  ( 5.000000000000000000, -57.49999999999999289, -6.123233995736766282E-16 ) ) ;
#21158=CARTESIAN_POINT ( 'NONE',  ( -2.229367062500000163, -89.47916666530106511, -3.861377020970580443 ) ) ;
#21159=CARTESIAN_POINT ( 'NONE',  ( -4.458734124999999437, -33.39583333196772941, -2.574251347313719407 ) ) ;
#21161=CARTESIAN_POINT ( 'NONE',  ( 9.457646018065525792E-16, -84.31249999863437949, 5.148502694627439702 ) ) ;
#21163=DIRECTION ( 'NONE',  ( -0.000000000000000000, 1.000000000000000000, -0.000000000000000000 ) ) ;
#21165=CARTESIAN_POINT ( 'NONE',  ( 4.458734124999999437, -7.812499998634405252, -5.460374474430324690E-16 ) ) ;
#21166=CARTESIAN_POINT ( 'NONE',  ( 2.229367062500001939, 23.77083333469892779, 3.861377020970579999 ) ) ;
#21167=CARTESIAN_POINT ( 'NONE',  ( -4.458734124999999437, -46.64583333196774362, -2.574251347313719407 ) ) ;
#21174=CARTESIAN_POINT ( 'NONE',  ( 4.458734124999998549, -72.72916666530106511, -2.574251347313721627 ) ) ;
#21175=CARTESIAN_POINT ( 'NONE',  ( 5.000000000000000000, -110.2916666639354588, -2.886751345948129988 ) ) ;
#21177=VECTOR ( 'NONE', #45994, 1000.000000000000000 ) ;
#21181=CARTESIAN_POINT ( 'NONE',  ( -5.000000000000000000, -67.00000000000000000, 0.000000000000000000 ) ) ;
#21187=CARTESIAN_POINT ( 'NONE',  ( 6.123233995736766282E-16, -120.0000000000000000, -5.000000000000000000 ) ) ;
#21194=VERTEX_POINT ( 'NONE', #43459 ) ;
#21195=CARTESIAN_POINT ( 'NONE',  ( 1.339745962155615144, -35.58034179853028434, 4.999999999999999112 ) ) ;
#21198=ORIENTED_EDGE ( 'NONE', *, *, #46687, .F. ) ;
#21201=CARTESIAN_POINT ( 'NONE',  ( 4.458734125000001214, -47.14583333196774362, 2.574251347313718519 ) ) ;
#21204=CARTESIAN_POINT ( 'NONE',  ( -6.972266317189433020E-16, -22.12499999726881228, -5.000000000000000000 ) ) ;
#21210=CARTESIAN_POINT ( 'NONE',  ( 1.975475456537005874E-15, -58.62499999726879452, 5.000000000000000000 ) ) ;
#21212=CARTESIAN_POINT ( 'NONE',  ( 9.457646018065525792E-16, -93.31249999863439371, 5.148502694627439702 ) ) ;
#21218=ADVANCED_FACE ( 'NONE', ( #39264 ), #19016, .T. ) ;
#21220=ORIENTED_EDGE ( 'NONE', *, *, #43993, .F. ) ;
#21221=AXIS2_PLACEMENT_3D ( 'NONE', #24417, #5432, #4791 ) ;
#21222=CARTESIAN_POINT ( 'NONE',  ( -4.458734124999998549, -4.229166665301070438, 2.574251347313722516 ) ) ;
#21223=AXIS2_PLACEMENT_3D ( 'NONE', #10867, #47496, #26946 ) ;
#21224=CARTESIAN_POINT ( 'NONE',  ( 4.458734124999999437, -23.06249999863440436, -5.460374474430324690E-16 ) ) ;
#21230=CARTESIAN_POINT ( 'NONE',  ( 9.457646018065525792E-16, 13.68750000136559386, 5.148502694627439702 ) ) ;
#21234=CARTESIAN_POINT ( 'NONE',  ( 2.229367062500001939, -16.97916666530106866, 3.861377020970579999 ) ) ;
#21238=CARTESIAN_POINT ( 'NONE',  ( 5.000000000000000000, -44.37499999726880873, -6.123233995736766282E-16 ) ) ;
#21240=CARTESIAN_POINT ( 'NONE',  ( 9.457646018065525792E-16, 6.937500001365595637, 5.148502694627439702 ) ) ;
#21241=CARTESIAN_POINT ( 'NONE',  ( 1.975475456537005874E-15, -8.624999997268812280, 5.000000000000000000 ) ) ;
#21242=ORIENTED_EDGE ( 'NONE', *, *, #50256, .F. ) ;
#21244=CARTESIAN_POINT ( 'NONE',  ( 4.458734124999999437, -68.81249999863439371, -5.460374474430324690E-16 ) ) ;
#21246=CARTESIAN_POINT ( 'NONE',  ( -5.000000000000000000, -1.000000000000000888, 0.000000000000000000 ) ) ;
#21248=CARTESIAN_POINT ( 'NONE',  ( -5.000000000000000000, 26.12500000273118417, 0.000000000000000000 ) ) ;
#21249=CARTESIAN_POINT ( 'NONE',  ( 2.229367062499998831, -58.64583333196773651, -3.861377020970580887 ) ) ;
#21250=CARTESIAN_POINT ( 'NONE',  ( -2.500000000000000444, -94.04166666393547303, -4.330127018922193649 ) ) ;
#21252=CARTESIAN_POINT ( 'NONE',  ( -2.499999999999996447, 20.29166666939784847, 4.330127018922195425 ) ) ;
#21256=CARTESIAN_POINT ( 'NONE',  ( 5.000000000000000000, -45.50000000000000000, -6.123233995736766282E-16 ) ) ;
#21257=LINE ( 'NONE', #30582, #43868 ) ;
#21259=EDGE_LOOP ( 'NONE', ( #14017, #33991, #40412, #873 ) ) ;
#21260=CARTESIAN_POINT ( 'NONE',  ( -4.458734124999998549, -108.2291666653010651, 2.574251347313722516 ) ) ;
#21261=CARTESIAN_POINT ( 'NONE',  ( -4.458734124999999437, -1.645833331967737401, -2.574251347313719407 ) ) ;
#21263=VECTOR ( 'NONE', #50570, 1000.000000000000114 ) ;
#21264=CARTESIAN_POINT ( 'NONE',  ( 1.339745962155612702, -73.16965819600734733, -5.000000000000000000 ) ) ;
#21267=VECTOR ( 'NONE', #17360, 1000.000000000000000 ) ;
#21274=EDGE_LOOP ( 'NONE', ( #60968, #24267, #49835, #22655 ) ) ;
#21275=CARTESIAN_POINT ( 'NONE',  ( 5.000000000000000000, -101.5000000000000000, -6.123233995736766282E-16 ) ) ;
#21277=CARTESIAN_POINT ( 'NONE',  ( -4.458734124999999437, -28.56249999863440081, 0.000000000000000000 ) ) ;
#21285=EDGE_CURVE ( 'NONE', #248, #20337, #37072, .T. ) ;
#21286=CARTESIAN_POINT ( 'NONE',  ( -2.500000000000000444, -94.04166666393547303, -4.330127018922193649 ) ) ;
#21288=CARTESIAN_POINT ( 'NONE',  ( -2.229367062500000163, -80.72916666530106511, -3.861377020970580443 ) ) ;
#21289=DIRECTION ( 'NONE',  ( 0.000000000000000000, 0.000000000000000000, 1.000000000000000000 ) ) ;
#21296=CARTESIAN_POINT ( 'NONE',  ( -2.229367062499996610, -3.395833331967738733, 3.861377020970582219 ) ) ;
#21298=ADVANCED_FACE ( 'NONE', ( #15479 ), #49560, .T. ) ;
#21301=CARTESIAN_POINT ( 'NONE',  ( 1.975475456537005874E-15, -44.74999999999999289, 5.000000000000000000 ) ) ;
#21302=ADVANCED_FACE ( 'NONE', ( #39899 ), #35098, .T. ) ;
#21303=ADVANCED_FACE ( 'NONE', ( #40233 ), #54716, .T. ) ;
#21306=AXIS2_PLACEMENT_3D ( 'NONE', #30379, #50002, #24608 ) ;
#21307=DIRECTION ( 'NONE',  ( -0.000000000000000000, 1.000000000000000000, -0.000000000000000000 ) ) ;
#21308=ORIENTED_EDGE ( 'NONE', *, *, #56294, .T. ) ;
#21309=CARTESIAN_POINT ( 'NONE',  ( -3.152548672688508926E-16, -84.56249999863439371, -5.148502694627439702 ) ) ;
#21310=EDGE_CURVE ( 'NONE', #9578, #15905, #1341, .T. ) ;
#21311=FACE_OUTER_BOUND ( 'NONE', #61296, .T. ) ;
#21312=CARTESIAN_POINT ( 'NONE',  ( 2.229367062499998831, -4.645833331967740065, -3.861377020970580887 ) ) ;
#21315=VECTOR ( 'NONE', #29677, 1000.000000000000000 ) ;
#21317=CARTESIAN_POINT ( 'NONE',  ( 1.060575238724906964E-15, -29.62499999726881228, 5.773502691896257311 ) ) ;
#21319=CARTESIAN_POINT ( 'NONE',  ( 4.458734124999998549, 25.27083333469892779, -2.574251347313721627 ) ) ;
#21322=CARTESIAN_POINT ( 'NONE',  ( 9.457646018065525792E-16, -53.06249999863441502, 5.148502694627439702 ) ) ;
#21323=CARTESIAN_POINT ( 'NONE',  ( 4.458734124999999437, -36.06249999863440792, -5.460374474430324690E-16 ) ) ;
#21326=CARTESIAN_POINT ( 'NONE',  ( -2.500000000000000444, 20.83333333333333215, -4.330127018922193649 ) ) ;
#21329=CARTESIAN_POINT ( 'NONE',  ( 9.457646018065525792E-16, -44.06249999863439371, 5.148502694627439702 ) ) ;
#21330=CARTESIAN_POINT ( 'NONE',  ( -2.500000000000000444, -78.04166666393547303, -4.330127018922193649 ) ) ;
#21334=CARTESIAN_POINT ( 'NONE',  ( -2.229367062499996610, -82.39583333196773651, 3.861377020970582219 ) ) ;
#21336=CARTESIAN_POINT ( 'NONE',  ( 0.000000000000000000, -120.0000000000000000, 0.000000000000000000 ) ) ;
#21337=CARTESIAN_POINT ( 'NONE',  ( 5.000000000000000000, -26.49999999999999645, -6.123233995736766282E-16 ) ) ;
#21341=ORIENTED_EDGE ( 'NONE', *, *, #54601, .T. ) ;
#21342=CARTESIAN_POINT ( 'NONE',  ( -4.458734124999998549, -88.22916666530107932, 2.574251347313722516 ) ) ;
#21343=CARTESIAN_POINT ( 'NONE',  ( 9.457646018065525792E-16, 12.68750000136559208, 5.148502694627439702 ) ) ;
#21344=CARTESIAN_POINT ( 'NONE',  ( -5.000000000000000000, 16.04166666939785202, -2.886751345948128211 ) ) ;
#21350=CARTESIAN_POINT ( 'NONE',  ( -6.972266317189433020E-16, 15.87500000273118417, -5.000000000000000000 ) ) ;
#21352=CARTESIAN_POINT ( 'NONE',  ( -2.499999999999996447, -61.83333333333333570, 4.330127018922195425 ) ) ;
#21354=LINE ( 'NONE', #10742, #46934 ) ;
#21356=CARTESIAN_POINT ( 'NONE',  ( -4.458734124999998549, -16.47916666530107577, 2.574251347313722516 ) ) ;
#21362=VECTOR ( 'NONE', #40860, 1000.000000000000000 ) ;
#21366=CARTESIAN_POINT ( 'NONE',  ( 0.000000000000000000, -120.0000000000000000, 0.000000000000000000 ) ) ;
#21367=VERTEX_POINT ( 'NONE', #5819 ) ;
#21369=CARTESIAN_POINT ( 'NONE',  ( 6.123233995736766282E-16, -120.0000000000000000, -5.000000000000000000 ) ) ;
#21372=CARTESIAN_POINT ( 'NONE',  ( -6.972266317189433020E-16, -10.24999999999999822, -5.000000000000000000 ) ) ;
#21374=CARTESIAN_POINT ( 'NONE',  ( 5.000000000000000888, -86.58333333333332860, 2.886751345948126879 ) ) ;
#21376=ORIENTED_EDGE ( 'NONE', *, *, #23713, .F. ) ;
#21377=CARTESIAN_POINT ( 'NONE',  ( -6.972266317189433020E-16, 11.74999999999999645, -5.000000000000000000 ) ) ;
#21378=CARTESIAN_POINT ( 'NONE',  ( 4.458734124999999437, 13.18750000136559208, -5.460374474430324690E-16 ) ) ;
#21379=EDGE_CURVE ( 'NONE', #32387, #47937, #35114, .T. ) ;
#21385=EDGE_CURVE ( 'NONE', #45889, #51535, #55359, .T. ) ;
#21386=CARTESIAN_POINT ( 'NONE',  ( 2.229367062500001939, -63.97916666530106511, 3.861377020970579999 ) ) ;
#21388=CARTESIAN_POINT ( 'NONE',  ( 4.458734125000001214, 12.10416666803226171, 2.574251347313718519 ) ) ;
#21391=EDGE_CURVE ( 'NONE', #59111, #62654, #54338, .T. ) ;
#21393=CARTESIAN_POINT ( 'NONE',  ( -2.229367062499996610, -55.39583333196773651, 3.861377020970582219 ) ) ;
#21394=CARTESIAN_POINT ( 'NONE',  ( -4.999999999999999112, -16.79166666393548368, 2.886751345948131764 ) ) ;
#21395=CARTESIAN_POINT ( 'NONE',  ( 5.000000000000000000, -48.50000000000000000, -6.123233995736766282E-16 ) ) ;
#21396=DIRECTION ( 'NONE',  ( -1.000000000000000000, -0.000000000000000000, -3.614007241618347908E-17 ) ) ;
#21398=CARTESIAN_POINT ( 'NONE',  ( 2.229367062500001939, -14.22916666530107221, 3.861377020970579999 ) ) ;
#21400=VECTOR ( 'NONE', #13926, 1000.000000000000000 ) ;
#21401=PLANE ( 'NONE',  #44 ) ;
#21402=CARTESIAN_POINT ( 'NONE',  ( 4.458734124999999437, -101.8124999986344079, -5.460374474430324690E-16 ) ) ;
#21405=CARTESIAN_POINT ( 'NONE',  ( 2.229367062499998831, -103.8958333319677365, -3.861377020970580887 ) ) ;
#21407=CARTESIAN_POINT ( 'NONE',  ( -4.458734124999998549, -29.22916666530107221, 2.574251347313722516 ) ) ;
#21408=CARTESIAN_POINT ( 'NONE',  ( -5.000000000000000000, -63.87499999726880873, 0.000000000000000000 ) ) ;
#21411=CARTESIAN_POINT ( 'NONE',  ( -4.458734124999999437, -22.39583333196773651, -2.574251347313719407 ) ) ;
#21412=CARTESIAN_POINT ( 'NONE',  ( 2.229367062499998831, -65.89583333196773651, -3.861377020970580887 ) ) ;
#21413=CARTESIAN_POINT ( 'NONE',  ( 6.158835246850667461E-14, 8.749999999999998224, -4.999999999999999112 ) ) ;
#21417=CARTESIAN_POINT ( 'NONE',  ( -5.000000000000000000, -11.00000000000000355, 0.000000000000000000 ) ) ;
#21421=DIRECTION ( 'NONE',  ( -0.000000000000000000, 1.000000000000000000, -0.000000000000000000 ) ) ;
#21426=CARTESIAN_POINT ( 'NONE',  ( 1.339745962155499015, -95.58034179853029855, 5.000000000000065725 ) ) ;
#21430=EDGE_LOOP ( 'NONE', ( #23129, #36220, #9228, #22829 ) ) ;
#21433=CARTESIAN_POINT ( 'NONE',  ( 2.499999999999998668, 26.66666666666666430, -4.330127018922193649 ) ) ;
#21441=( BOUNDED_CURVE ( )  B_SPLINE_CURVE ( 2, ( #13679, #38131, #55631, #47769, #1923, #37817, #55940, #57756, #26982 ),
 .UNSPECIFIED., .F., .F. ) 
 B_SPLINE_CURVE_WITH_KNOTS ( ( 3, 2, 2, 2, 3 ),
 ( 0.8982142857142857428, 0.8988095238095238360, 0.9000000000000000222, 0.9011904761904762085, 0.9017857142857143016 ),
 .UNSPECIFIED. ) 
 CURVE ( )  GEOMETRIC_REPRESENTATION_ITEM ( )  RATIONAL_B_SPLINE_CURVE ( ( 0.9330127018922194093, 0.9330127018922194093, 1.000000000000000000, 0.8660254037844387076, 1.000000000000000000, 0.8660254037844387076, 1.000000000000000000, 0.9330127018922194093, 0.9330127018922194093 ) ) 
 REPRESENTATION_ITEM ( '' )  );
#21442=CYLINDRICAL_SURFACE ( 'NONE', #32692, 5.000000000000000000 ) ;
#21445=AXIS2_PLACEMENT_3D ( 'NONE', #47518, #32411, #33051 ) ;
#21448=ORIENTED_EDGE ( 'NONE', *, *, #59503, .F. ) ;
#21454=CARTESIAN_POINT ( 'NONE',  ( 4.458734124999999437, -79.81249999863440792, -5.460374474430324690E-16 ) ) ;
#21455=CARTESIAN_POINT ( 'NONE',  ( 4.458734124999998549, 29.27083333469892423, -2.574251347313721627 ) ) ;
#21458=DIRECTION ( 'NONE',  ( -0.000000000000000000, 1.000000000000000000, -0.000000000000000000 ) ) ;
#21462=CARTESIAN_POINT ( 'NONE',  ( 1.339745962155612702, 0.8303418039926664385, -5.000000000000000000 ) ) ;
#21465=CARTESIAN_POINT ( 'NONE',  ( -3.152548672688508926E-16, -49.56249999863441502, -5.148502694627439702 ) ) ;
#21467=CARTESIAN_POINT ( 'NONE',  ( 2.229367062500001939, 29.02083333469892779, 3.861377020970579999 ) ) ;
#21468=CARTESIAN_POINT ( 'NONE',  ( 5.000000000000000000, -108.4166666666666572, -2.886751345948129988 ) ) ;
#21470=CARTESIAN_POINT ( 'NONE',  ( 4.458734125000001214, -38.14583333196773651, 2.574251347313718519 ) ) ;
#21471=CARTESIAN_POINT ( 'NONE',  ( 2.499999999999998668, 3.791666669397852019, -4.330127018922193649 ) ) ;
#21472=CARTESIAN_POINT ( 'NONE',  ( 5.000000000000000000, -50.50000000000000000, -6.123233995736766282E-16 ) ) ;
#21477=CARTESIAN_POINT ( 'NONE',  ( 9.457646018065525792E-16, -95.06249999863440792, 5.148502694627439702 ) ) ;
#21479=CARTESIAN_POINT ( 'NONE',  ( -4.458734124999999437, -0.6458333319677399542, -2.574251347313719407 ) ) ;
#21480=ORIENTED_EDGE ( 'NONE', *, *, #38543, .T. ) ;
#21483=CARTESIAN_POINT ( 'NONE',  ( -4.458734124999999437, -89.31249999863440792, 0.000000000000000000 ) ) ;
#21485=CARTESIAN_POINT ( 'NONE',  ( -2.229367062500000163, -86.72916666530107932, -3.861377020970580443 ) ) ;
#21489=CARTESIAN_POINT ( 'NONE',  ( 4.458734125000000326, -4.895833331967740065, 2.574251347313718519 ) ) ;
#21490=CARTESIAN_POINT ( 'NONE',  ( -4.458734124999999437, 18.43750000136559564, 0.000000000000000000 ) ) ;
#21491=CARTESIAN_POINT ( 'NONE',  ( -4.458734124999997661, -50.47916666530107221, 2.574251347313722516 ) ) ;
#21492=CARTESIAN_POINT ( 'NONE',  ( 1.975475456537005874E-15, -7.624999997268812280, 5.000000000000000000 ) ) ;
#21495=CARTESIAN_POINT ( 'NONE',  ( 1.975475456537005874E-15, -43.62499999726880873, 5.000000000000000000 ) ) ;
#21496=VERTEX_POINT ( 'NONE', #62005 ) ;
#21499=( BOUNDED_CURVE ( )  B_SPLINE_CURVE ( 2, ( #9675, #10319, #63413, #10631, #38625, #38944, #58580, #45051, #26714 ),
 .UNSPECIFIED., .F., .F. ) 
 B_SPLINE_CURVE_WITH_KNOTS ( ( 3, 2, 2, 2, 3 ),
 ( 0.9124999999999999778, 0.9130952380952380709, 0.9142857142857142572, 0.9154761904761904434, 0.9160714285714285365 ),
 .UNSPECIFIED. ) 
 CURVE ( )  GEOMETRIC_REPRESENTATION_ITEM ( )  RATIONAL_B_SPLINE_CURVE ( ( 0.9330127018922194093, 0.9330127018922194093, 1.000000000000000000, 0.8660254037844387076, 1.000000000000000000, 0.8660254037844387076, 1.000000000000000000, 0.9330127018922194093, 0.9330127018922194093 ) ) 
 REPRESENTATION_ITEM ( '' )  );
#21501=CARTESIAN_POINT ( 'NONE',  ( -2.229367062500000163, -76.47916666530106511, -3.861377020970580443 ) ) ;
#21502=CARTESIAN_POINT ( 'NONE',  ( 4.458734124999998549, 29.02083333469893134, -2.574251347313721627 ) ) ;
#21503=ADVANCED_FACE ( 'NONE', ( #52033 ), #52967, .T. ) ;
#21508=CARTESIAN_POINT ( 'NONE',  ( 5.000000000000000000, -64.41666666666667140, -2.886751345948129988 ) ) ;
#21509=CARTESIAN_POINT ( 'NONE',  ( 5.000000000000000888, -36.45833333060213732, 2.886751345948126879 ) ) ;
#21512=DIRECTION ( 'NONE',  ( -0.000000000000000000, 1.000000000000000000, -0.000000000000000000 ) ) ;
#21513=CARTESIAN_POINT ( 'NONE',  ( -2.499999999999996447, 9.166666666666666075, 4.330127018922195425 ) ) ;
#21520=ORIENTED_EDGE ( 'NONE', *, *, #3507, .T. ) ;
#21522=CARTESIAN_POINT ( 'NONE',  ( -1.975475456537005874E-15, 27.37500000273118417, 5.000000000000000000 ) ) ;
#21527=CARTESIAN_POINT ( 'NONE',  ( -4.458734124999998549, -47.47916666530106511, 2.574251347313722516 ) ) ;
#21528=CARTESIAN_POINT ( 'NONE',  ( 5.000000000000000000, -34.41666666666666430, -2.886751345948130876 ) ) ;
#21531=CARTESIAN_POINT ( 'NONE',  ( -4.999999999999998224, -21.79166666393548368, 2.886751345948131764 ) ) ;
#21538=CARTESIAN_POINT ( 'NONE',  ( -4.458734124999999437, -92.64583333196773651, -2.574251347313719407 ) ) ;
#21539=FACE_OUTER_BOUND ( 'NONE', #32704, .T. ) ;
#21540=ORIENTED_EDGE ( 'NONE', *, *, #58971, .F. ) ;
#21544=FACE_OUTER_BOUND ( 'NONE', #43116, .T. ) ;
#21545=VECTOR ( 'NONE', #55438, 1000.000000000000000 ) ;
#21546=CARTESIAN_POINT ( 'NONE',  ( 4.458734124999999437, -2.812499998634407472, -5.460374474430324690E-16 ) ) ;
#21548=CARTESIAN_POINT ( 'NONE',  ( 9.457646018065525792E-16, -23.31249999863440436, 5.148502694627439702 ) ) ;
#21554=CARTESIAN_POINT ( 'NONE',  ( -2.229367062500000163, 13.27083333469892779, -3.861377020970580443 ) ) ;
#21555=VERTEX_POINT ( 'NONE', #42049 ) ;
#21557=DIRECTION ( 'NONE',  ( -0.000000000000000000, 1.000000000000000000, -0.000000000000000000 ) ) ;
#21558=CARTESIAN_POINT ( 'NONE',  ( 2.499999999999998668, -84.33333333333332860, -4.330127018922193649 ) ) ;
#21559=CARTESIAN_POINT ( 'NONE',  ( 2.229367062500001939, -17.97916666530106866, 3.861377020970579999 ) ) ;
#21560=CARTESIAN_POINT ( 'NONE',  ( 6.123233995736766282E-16, -120.0000000000000000, -5.000000000000000000 ) ) ;
#21563=CARTESIAN_POINT ( 'NONE',  ( 2.499999999999998668, -44.20833333060214443, -4.330127018922193649 ) ) ;
#21564=CARTESIAN_POINT ( 'NONE',  ( 2.500000000000002220, -24.66666666666666430, 4.330127018922192761 ) ) ;
#21565=CARTESIAN_POINT ( 'NONE',  ( -2.229367062499996610, 9.854166668032261711, 3.861377020970582219 ) ) ;
#21566=CARTESIAN_POINT ( 'NONE',  ( -2.500000000000000444, -63.04166666393547303, -4.330127018922193649 ) ) ;
#21569=CARTESIAN_POINT ( 'NONE',  ( -2.229367062499996610, -66.14583333196773651, 3.861377020970582219 ) ) ;
#21571=CARTESIAN_POINT ( 'NONE',  ( 5.000000000000000888, -0.5833333333333350357, 2.886751345948126879 ) ) ;
#21573=CARTESIAN_POINT ( 'NONE',  ( 2.229367062500001939, -56.97916666530107932, 3.861377020970579999 ) ) ;
#21574=CARTESIAN_POINT ( 'NONE',  ( 2.499999999999998668, -97.20833333060213022, -4.330127018922193649 ) ) ;
#21581=CARTESIAN_POINT ( 'NONE',  ( -4.999999999999999112, -49.91666666666666430, 2.886751345948131764 ) ) ;
#21583=CARTESIAN_POINT ( 'NONE',  ( 2.499999999999998668, -17.20833333060214443, -4.330127018922193649 ) ) ;
#21585=CARTESIAN_POINT ( 'NONE',  ( -4.458734124999999437, -107.3958333319677365, -2.574251347313719407 ) ) ;
#21586=CARTESIAN_POINT ( 'NONE',  ( -3.152548672688508926E-16, -0.8124999986344055847, -5.148502694627439702 ) ) ;
#21591=( BOUNDED_CURVE ( )  B_SPLINE_CURVE ( 2, ( #27119, #16829, #2678, #17476, #21980, #27424, #42850, #28059, #7507 ),
 .UNSPECIFIED., .F., .F. ) 
 B_SPLINE_CURVE_WITH_KNOTS ( ( 3, 2, 2, 2, 3 ),
 ( 0.4553571428571428492, 0.4559523809523809423, 0.4571428571428571286, 0.4583333333333333148, 0.4589285714285714080 ),
 .UNSPECIFIED. ) 
 CURVE ( )  GEOMETRIC_REPRESENTATION_ITEM ( )  RATIONAL_B_SPLINE_CURVE ( ( 0.9330127018922194093, 0.9330127018922194093, 1.000000000000000000, 0.8660254037844387076, 1.000000000000000000, 0.8660254037844387076, 1.000000000000000000, 0.9330127018922194093, 0.9330127018922194093 ) ) 
 REPRESENTATION_ITEM ( '' )  );
#21593=EDGE_CURVE ( 'NONE', #14094, #38980, #41665, .T. ) ;
#21597=CARTESIAN_POINT ( 'NONE',  ( -5.000000000000000000, 28.04166666939785202, -2.886751345948128211 ) ) ;
#21598=ADVANCED_FACE ( 'NONE', ( #27266 ), #3462, .T. ) ;
#21601=CARTESIAN_POINT ( 'NONE',  ( -4.999999999999998224, -55.79166666393548013, 2.886751345948131764 ) ) ;
#21603=CARTESIAN_POINT ( 'NONE',  ( -3.152548672688508926E-16, -30.81249999863440436, -5.148502694627439702 ) ) ;
#21604=CARTESIAN_POINT ( 'NONE',  ( 1.975475456537005874E-15, -86.75000000000001421, 5.000000000000000000 ) ) ;
#21612=ORIENTED_EDGE ( 'NONE', *, *, #27440, .F. ) ;
#21613=CARTESIAN_POINT ( 'NONE',  ( -2.229367062500000163, -79.72916666530106511, -3.861377020970580443 ) ) ;
#21615=ORIENTED_EDGE ( 'NONE', *, *, #22761, .T. ) ;
#21619=CARTESIAN_POINT ( 'NONE',  ( -4.458734124999999437, -11.56249999863440792, 0.000000000000000000 ) ) ;
#21620=ORIENTED_EDGE ( 'NONE', *, *, #22183, .T. ) ;
#21622=DIRECTION ( 'NONE',  ( -0.000000000000000000, 1.000000000000000000, -0.000000000000000000 ) ) ;
#21624=EDGE_CURVE ( 'NONE', #49905, #45912, #60932, .T. ) ;
#21625=CARTESIAN_POINT ( 'NONE',  ( 2.229367062499998831, -7.895833331967735624, -3.861377020970580887 ) ) ;
#21627=AXIS2_PLACEMENT_3D ( 'NONE', #10615, #21557, #60483 ) ;
#21628=CARTESIAN_POINT ( 'NONE',  ( -6.972266317189433020E-16, -60.12499999726880162, -5.000000000000000000 ) ) ;
#21631=ORIENTED_EDGE ( 'NONE', *, *, #48877, .T. ) ;
#21632=CARTESIAN_POINT ( 'NONE',  ( 9.457646018065525792E-16, -87.06249999863439371, 5.148502694627439702 ) ) ;
#21634=CARTESIAN_POINT ( 'NONE',  ( 4.458734125000001214, -2.895833331967738289, 2.574251347313718519 ) ) ;
#21636=CARTESIAN_POINT ( 'NONE',  ( -5.000000000000000000, -31.87499999726880873, 0.000000000000000000 ) ) ;
#21638=CARTESIAN_POINT ( 'NONE',  ( -4.458734124999999437, 24.60416666803225993, -2.574251347313719407 ) ) ;
#21639=CARTESIAN_POINT ( 'NONE',  ( -6.972266317189433020E-16, -56.25000000000000000, -5.000000000000000000 ) ) ;
#21641=CARTESIAN_POINT ( 'NONE',  ( -3.152548672688508926E-16, -53.56249999863439371, -5.148502694627439702 ) ) ;
#21642=CARTESIAN_POINT ( 'NONE',  ( 4.458734125000000326, -38.14583333196773651, 2.574251347313718519 ) ) ;
#21646=CARTESIAN_POINT ( 'NONE',  ( -2.499999999999996447, 13.16666666666666607, 4.330127018922195425 ) ) ;
#21649=CARTESIAN_POINT ( 'NONE',  ( 4.458734124999998549, -40.72916666530107221, -2.574251347313721627 ) ) ;
#21650=CARTESIAN_POINT ( 'NONE',  ( -3.535250795749689387E-16, -78.12499999726880162, -5.773502691896257311 ) ) ;
#21651=EDGE_CURVE ( 'NONE', #50712, #21367, #50202, .T. ) ;
#21654=EDGE_CURVE ( 'NONE', #37904, #62207, #3814, .T. ) ;
#21655=LINE ( 'NONE', #60582, #23384 ) ;
#21657=CARTESIAN_POINT ( 'NONE',  ( 4.458734125000000326, -86.14583333196775072, 2.574251347313718519 ) ) ;
#21660=CARTESIAN_POINT ( 'NONE',  ( 5.000000000000000000, -30.41666666666666785, -2.886751345948129988 ) ) ;
#21662=ORIENTED_EDGE ( 'NONE', *, *, #33067, .F. ) ;
#21664=ORIENTED_EDGE ( 'NONE', *, *, #38995, .T. ) ;
#21665=CARTESIAN_POINT ( 'NONE',  ( -2.229367062499996610, -91.14583333196773651, 3.861377020970582219 ) ) ;
#21666=CARTESIAN_POINT ( 'NONE',  ( 2.229367062500001939, 11.77083333469892601, 3.861377020970579999 ) ) ;
#21667=CARTESIAN_POINT ( 'NONE',  ( -5.000000000000000000, 16.12500000273118417, 0.000000000000000000 ) ) ;
#21668=CARTESIAN_POINT ( 'NONE',  ( 1.975475456537005874E-15, -89.74999999999998579, 5.000000000000000000 ) ) ;
#21670=ADVANCED_FACE ( 'NONE', ( #18859 ), #38789, .T. ) ;
#21674=CARTESIAN_POINT ( 'NONE',  ( -4.999999999999998224, -109.9166666666666572, 2.886751345948131764 ) ) ;
#21675=CARTESIAN_POINT ( 'NONE',  ( 5.000000000000000000, -1.500000000000001332, -6.123233995736766282E-16 ) ) ;
#21676=EDGE_CURVE ( 'NONE', #6165, #18131, #4292, .T. ) ;
#21677=CARTESIAN_POINT ( 'NONE',  ( -1.339745962155613812, -75.08034179853029855, -5.000000000000000000 ) ) ;
#21679=AXIS2_PLACEMENT_3D ( 'NONE', #57332, #38012, #57644 ) ;
#21680=( BOUNDED_CURVE ( )  B_SPLINE_CURVE ( 2, ( #36092, #11633, #2327, #11952, #16788, #7149, #59917, #30298, #41216 ),
 .UNSPECIFIED., .F., .F. ) 
 B_SPLINE_CURVE_WITH_KNOTS ( ( 3, 2, 2, 2, 3 ),
 ( 0.8696428571428571619, 0.8702380952380952550, 0.8714285714285714413, 0.8726190476190476275, 0.8732142857142857206 ),
 .UNSPECIFIED. ) 
 CURVE ( )  GEOMETRIC_REPRESENTATION_ITEM ( )  RATIONAL_B_SPLINE_CURVE ( ( 0.9330127018922194093, 0.9330127018922194093, 1.000000000000000000, 0.8660254037844387076, 1.000000000000000000, 0.8660254037844387076, 1.000000000000000000, 0.9330127018922194093, 0.9330127018922194093 ) ) 
 REPRESENTATION_ITEM ( '' )  );
#21681=CARTESIAN_POINT ( 'NONE',  ( 1.975475456537005874E-15, -42.75000000000000000, 5.000000000000000000 ) ) ;
#21682=CARTESIAN_POINT ( 'NONE',  ( -2.229367062500000163, -14.72916666530107221, -3.861377020970580443 ) ) ;
#21691=CARTESIAN_POINT ( 'NONE',  ( 5.000000000000000000, -85.29166666393547303, -2.886751345948130876 ) ) ;
#21693=CARTESIAN_POINT ( 'NONE',  ( 4.458734125000001214, -61.14583333196773651, 2.574251347313718519 ) ) ;
#21695=CARTESIAN_POINT ( 'NONE',  ( 5.000000000000000000, -58.41666666666665719, -2.886751345948130876 ) ) ;
#21697=VERTEX_POINT ( 'NONE', #48454 ) ;
#21702=ORIENTED_EDGE ( 'NONE', *, *, #14576, .F. ) ;
#21703=CARTESIAN_POINT ( 'NONE',  ( 1.339745962155615144, 11.29465819873851906, 4.999999999999999112 ) ) ;
#21704=CARTESIAN_POINT ( 'NONE',  ( 4.458734125000001214, 8.104166668032261711, 2.574251347313718519 ) ) ;
#21707=CARTESIAN_POINT ( 'NONE',  ( -2.480964764533239819E-13, -108.6249999972688016, 5.000000000000000000 ) ) ;
#21709=EDGE_LOOP ( 'NONE', ( #8520, #4909, #13557, #2159, #59036, #20261, #43393, #40659, #36100, #48118, #12565, #34887, #61947, #19594, #43564, #13459, #53851, #4651, #58351, #43024, #57437, #35984, #33794, #33295, #39719, #48173, #25048, #20679, #37584, #56712, #49649, #16849, #27151, #60040, #41624, #18945, #50708, #50631, #59907, #34396, #22332, #32326, #16933, #30114, #21856, #60467, #25225, #37329, #21740, #57523, #53682, #12291, #25158, #21612, #25092, #479, #32846, #61563, #9543, #31155, #48524, #3057, #45566, #63610, #24913, #46032, #54364, #61245, #27224, #8448, #51740, #15455, #48074, #27738, #18738, #18676, #38987, #39301, #4749, #10034, #16037, #60425, #26512, #58254, #57849, #32566, #40734, #14677, #34793, #25478, #21065, #56187, #50074, #15562, #42314, #40316, #3787, #29971, #26798, #57207, #36382, #43056, #17883, #32113, #4037, #43153, #44939, #32459, #54910, #36340, #61321, #18407, #25705, #56877, #27596, #41600, #20649, #2961, #7459, #45594, #21376, #44850, #45615, #28549, #38911, #25623, #44601, #36369, #56980, #40082, #17921, #18149, #49364, #42903, #17802, #33448, #48450, #37427, #45873, #8282, #28165, #5685, #10903, #54010, #59377, #8532, #21220, #51801, #7150, #35679, #16538, #57615, #53487, #37485, #14697, #10020, #22343, #16008, #6683, #26130, #51016, #45493, #358, #57990, #52713, #37444, #15830, #13686, #49680, #59905, #53869, #40687, #3737, #40009, #32436, #28927, #40076, #40126, #15800, #16888, #50206, #48342, #63183, #31243, #52549, #22157, #15407, #49281, #15193, #47188, #30368, #26351, #50391, #14679, #1358, #4336, #49001, #55085, #53053, #18802, #35572, #20060, #43713, #32986, #555, #17236, #62895, #28021, #12809, #62134, #15140, #48162, #39540, #6620, #11609, #28473, #29472, #3391, #46768, #40339, #33083, #18840, #34260, #27305, #30360, #2927, #29327, #41191, #6509, #21448, #1686, #54502, #35908, #12911, #44551, #29891, #60328, #38512, #16511, #32498, #6325, #44264, #6084, #956, #28130, #38606, #40102, #35350, #19992, #42385, #32306, #28469, #3411, #44383, #30780, #20882, #22232, #12347, #58228, #47327, #28363, #48321, #25358, #35284, #47872, #42713, #6757, #18743, #18254, #28012, #45941, #21662, #24721, #49671, #35709, #43009, #27007, #51288, #16765, #25639, #1161, #50065, #13976, #16305 ) ) ;
#21710=CARTESIAN_POINT ( 'NONE',  ( 9.457646018065525792E-16, -70.06249999863439371, 5.148502694627439702 ) ) ;
#21712=CARTESIAN_POINT ( 'NONE',  ( 4.458734124999999437, 10.18750000136559386, -5.460374474430324690E-16 ) ) ;
#21713=CARTESIAN_POINT ( 'NONE',  ( -5.000000000000000000, -69.87499999726880162, 0.000000000000000000 ) ) ;
#21714=FACE_OUTER_BOUND ( 'NONE', #9097, .T. ) ;
#21715=CARTESIAN_POINT ( 'NONE',  ( 9.457646018065525792E-16, -54.31249999863440081, 5.148502694627439702 ) ) ;
#21716=CARTESIAN_POINT ( 'NONE',  ( 2.499999999999998668, -12.20833333060214798, -4.330127018922193649 ) ) ;
#21718=DIRECTION ( 'NONE',  ( -0.000000000000000000, 1.000000000000000000, -0.000000000000000000 ) ) ;
#21719=CARTESIAN_POINT ( 'NONE',  ( 5.000000000000000888, -65.58333333333332860, 2.886751345948126879 ) ) ;
#21720=CARTESIAN_POINT ( 'NONE',  ( 4.458734124999998549, -21.97916666530107221, -2.574251347313721627 ) ) ;
#21722=CARTESIAN_POINT ( 'NONE',  ( -1.339745962155613812, -102.2053418012614827, -5.000000000000000000 ) ) ;
#21723=CARTESIAN_POINT ( 'NONE',  ( -4.458734124999999437, -107.3958333319677365, -2.574251347313719407 ) ) ;
#21725=EDGE_LOOP ( 'NONE', ( #43230, #48061, #33703, #49347 ) ) ;
#21726=CARTESIAN_POINT ( 'NONE',  ( 4.458734124999999437, -101.0624999986344079, -5.460374474430324690E-16 ) ) ;
#21727=CARTESIAN_POINT ( 'NONE',  ( -3.152548672688508926E-16, -27.56249999863440081, -5.148502694627439702 ) ) ;
#21728=CARTESIAN_POINT ( 'NONE',  ( 2.500000000000002220, -64.54166666393547303, 4.330127018922192761 ) ) ;
#21732=CARTESIAN_POINT ( 'NONE',  ( -4.458734124999999437, -21.39583333196774007, -2.574251347313719407 ) ) ;
#21733=CARTESIAN_POINT ( 'NONE',  ( 4.458734124999998549, -67.97916666530106511, -2.574251347313721627 ) ) ;
#21734=FACE_OUTER_BOUND ( 'NONE', #45672, .T. ) ;
#21738=CARTESIAN_POINT ( 'NONE',  ( -4.999999999999999112, -12.91666666666666785, 2.886751345948131764 ) ) ;
#21740=ORIENTED_EDGE ( 'NONE', *, *, #57459, .F. ) ;
#21742=EDGE_CURVE ( 'NONE', #38436, #62035, #30082, .T. ) ;
#21746=EDGE_CURVE ( 'NONE', #24993, #53062, #48245, .T. ) ;
#21747=CARTESIAN_POINT ( 'NONE',  ( 1.339745962155608039, 25.29465819873851729, 5.000000000000003553 ) ) ;
#21756=LINE ( 'NONE', #18794, #56170 ) ;
#21758=CARTESIAN_POINT ( 'NONE',  ( 0.000000000000000000, -120.0000000000000000, 0.000000000000000000 ) ) ;
#21760=EDGE_CURVE ( 'NONE', #34735, #37487, #36522, .T. ) ;
#21762=EDGE_CURVE ( 'NONE', #41671, #5841, #19004, .T. ) ;
#21764=EDGE_LOOP ( 'NONE', ( #5380, #29460, #7282, #33203 ) ) ;
#21770=VERTEX_POINT ( 'NONE', #31699 ) ;
#21775=( BOUNDED_CURVE ( )  B_SPLINE_CURVE ( 2, ( #59188, #35376, #40830, #26361, #6441, #20909, #336, #50812, #5789 ),
 .UNSPECIFIED., .F., .F. ) 
 B_SPLINE_CURVE_WITH_KNOTS ( ( 3, 2, 2, 2, 3 ),
 ( 0.2160714285714285809, 0.2166666666666666741, 0.2178571428571428603, 0.2190476190476190466, 0.2196428571428571397 ),
 .UNSPECIFIED. ) 
 CURVE ( )  GEOMETRIC_REPRESENTATION_ITEM ( )  RATIONAL_B_SPLINE_CURVE ( ( 0.9330127018922194093, 0.9330127018922194093, 1.000000000000000000, 0.8660254037844387076, 1.000000000000000000, 0.8660254037844387076, 1.000000000000000000, 0.9330127018922194093, 0.9330127018922194093 ) ) 
 REPRESENTATION_ITEM ( '' )  );
#21776=CARTESIAN_POINT ( 'NONE',  ( 4.458734125000001214, -77.89583333196773651, 2.574251347313718519 ) ) ;
#21777=CARTESIAN_POINT ( 'NONE',  ( -4.458734124999999437, 26.60416666803225993, -2.574251347313719407 ) ) ;
#21778=CARTESIAN_POINT ( 'NONE',  ( 2.500000000000002220, -18.66666666666666430, 4.330127018922192761 ) ) ;
#21780=DIRECTION ( 'NONE',  ( -0.000000000000000000, 1.000000000000000000, -0.000000000000000000 ) ) ;
#21786=CARTESIAN_POINT ( 'NONE',  ( 2.229367062500001939, -56.97916666530107932, 3.861377020970579999 ) ) ;
#21788=CARTESIAN_POINT ( 'NONE',  ( 4.458734125000001214, 27.10416666803225993, 2.574251347313718519 ) ) ;
#21789=CARTESIAN_POINT ( 'NONE',  ( 2.500000000000002220, -108.6666666666666572, 4.330127018922192761 ) ) ;
#21791=CARTESIAN_POINT ( 'NONE',  ( -4.458734124999999437, -37.56249999863440792, 0.000000000000000000 ) ) ;
#21792=CARTESIAN_POINT ( 'NONE',  ( 1.060575238724906964E-15, 1.375000002731184834, 5.773502691896257311 ) ) ;
#21796=CARTESIAN_POINT ( 'NONE',  ( 1.339745962155619807, 24.70534180126147916, -4.999999999999996447 ) ) ;
#21797=CARTESIAN_POINT ( 'NONE',  ( 2.229367062500001939, -96.97916666530105090, 3.861377020970579999 ) ) ;
#21798=CARTESIAN_POINT ( 'NONE',  ( -4.458734124999999437, -3.645833331967739177, -2.574251347313719407 ) ) ;
#21799=ORIENTED_EDGE ( 'NONE', *, *, #5255, .T. ) ;
#21801=CYLINDRICAL_SURFACE ( 'NONE', #60666, 5.000000000000000000 ) ;
#21802=CARTESIAN_POINT ( 'NONE',  ( 4.458734124999998549, -89.72916666530106511, -2.574251347313721627 ) ) ;
#21804=CARTESIAN_POINT ( 'NONE',  ( 4.458734124999999437, -89.06249999863439371, -5.460374474430324690E-16 ) ) ;
#21808=CARTESIAN_POINT ( 'NONE',  ( 4.458734125000000326, -8.895833331967736513, 2.574251347313718519 ) ) ;
#21809=CARTESIAN_POINT ( 'NONE',  ( -2.229367062500000163, 19.27083333469892779, -3.861377020970580443 ) ) ;
#21810=CARTESIAN_POINT ( 'NONE',  ( 2.229367062499998831, -50.89583333196772941, -3.861377020970580887 ) ) ;
#21811=CARTESIAN_POINT ( 'NONE',  ( 1.975475456537005874E-15, -11.74999999999999645, 5.000000000000000000 ) ) ;
#21817=CARTESIAN_POINT ( 'NONE',  ( 2.229367062500001939, -78.97916666530106511, 3.861377020970579999 ) ) ;
#21818=CARTESIAN_POINT ( 'NONE',  ( 5.000000000000000000, -108.2916666639354730, -2.886751345948129988 ) ) ;
#21820=CARTESIAN_POINT ( 'NONE',  ( -2.500000000000000444, -58.04166666393548013, -4.330127018922193649 ) ) ;
#21823=CARTESIAN_POINT ( 'NONE',  ( -3.535250795749689387E-16, -67.25000000000000000, -5.773502691896257311 ) ) ;
#21827=ORIENTED_EDGE ( 'NONE', *, *, #45248, .T. ) ;
#21830=CARTESIAN_POINT ( 'NONE',  ( -2.500000000000000444, 8.833333333333332149, -4.330127018922193649 ) ) ;
#21831=CARTESIAN_POINT ( 'NONE',  ( -1.339745962155610925, -106.6696581960073189, 5.000000000000000000 ) ) ;
#21839=CARTESIAN_POINT ( 'NONE',  ( 5.000000000000000000, -28.41666666666666430, -2.886751345948130876 ) ) ;
#21844=CARTESIAN_POINT ( 'NONE',  ( -4.458734124999999437, -53.56249999863439371, 0.000000000000000000 ) ) ;
#21845=CARTESIAN_POINT ( 'NONE',  ( 2.500000000000002220, -34.66666666666666430, 4.330127018922192761 ) ) ;
#21847=CYLINDRICAL_SURFACE ( 'NONE', #1542, 5.000000000000000000 ) ;
#21854=CARTESIAN_POINT ( 'NONE',  ( -2.229367062499996610, -96.39583333196773651, 3.861377020970582219 ) ) ;
#21856=ORIENTED_EDGE ( 'NONE', *, *, #8596, .F. ) ;
#21861=CARTESIAN_POINT ( 'NONE',  ( -2.229367062499996610, -1.145833331967736957, 3.861377020970582219 ) ) ;
#21862=CARTESIAN_POINT ( 'NONE',  ( -2.229367062500000163, -94.72916666530106511, -3.861377020970580443 ) ) ;
#21864=CARTESIAN_POINT ( 'NONE',  ( -4.458734124999998549, -21.47916666530107221, 2.574251347313722516 ) ) ;
#21871=CARTESIAN_POINT ( 'NONE',  ( -3.152548672688508926E-16, 12.18750000136559564, -5.148502694627439702 ) ) ;
#21873=CARTESIAN_POINT ( 'NONE',  ( -2.500000000000000444, -53.04166666393548013, -4.330127018922193649 ) ) ;
#21875=CARTESIAN_POINT ( 'NONE',  ( 5.000000000000000000, -84.49999999999998579, -6.123233995736766282E-16 ) ) ;
#21876=CARTESIAN_POINT ( 'NONE',  ( -2.229367062499996610, -19.14583333196774007, 3.861377020970582219 ) ) ;
#21880=CARTESIAN_POINT ( 'NONE',  ( 1.060575238724906964E-15, -44.62499999726881583, 5.773502691896257311 ) ) ;
#21881=DIRECTION ( 'NONE',  ( 0.000000000000000000, 0.000000000000000000, 1.000000000000000000 ) ) ;
#21882=CARTESIAN_POINT ( 'NONE',  ( -2.229367062500000163, 8.520833334698926009, -3.861377020970580443 ) ) ;
#21886=CARTESIAN_POINT ( 'NONE',  ( -2.229367062499996610, -65.14583333196773651, 3.861377020970582219 ) ) ;
#21888=CARTESIAN_POINT ( 'NONE',  ( -4.999999999999999112, 0.08333333333333457771, 2.886751345948131764 ) ) ;
#21890=DIRECTION ( 'NONE',  ( -0.000000000000000000, 1.000000000000000000, -0.000000000000000000 ) ) ;
#21891=CARTESIAN_POINT ( 'NONE',  ( -4.458734124999999437, -59.31249999863440081, 0.000000000000000000 ) ) ;
#21892=CARTESIAN_POINT ( 'NONE',  ( -3.535250795749689387E-16, -94.12499999726881583, -5.773502691896257311 ) ) ;
#21893=CARTESIAN_POINT ( 'NONE',  ( 0.000000000000000000, -120.0000000000000000, 5.000000000000000000 ) ) ;
#21896=CARTESIAN_POINT ( 'NONE',  ( 5.000000000000000888, -49.58333333333332860, 2.886751345948126879 ) ) ;
#21900=CARTESIAN_POINT ( 'NONE',  ( -3.152548672688508926E-16, -105.5624999986344079, -5.148502694627439702 ) ) ;
#21901=CARTESIAN_POINT ( 'NONE',  ( -4.458734124999999437, -0.6458333319677399542, -2.574251347313719407 ) ) ;
#21909=CARTESIAN_POINT ( 'NONE',  ( -6.972266317189433020E-16, -81.24999999999998579, -5.000000000000000000 ) ) ;
#21915=CARTESIAN_POINT ( 'NONE',  ( -4.458734124999999437, -30.56249999863440436, 0.000000000000000000 ) ) ;
#21923=CARTESIAN_POINT ( 'NONE',  ( 5.000000000000000000, -70.37499999726880162, -6.123233995736766282E-16 ) ) ;
#21924=CARTESIAN_POINT ( 'NONE',  ( -4.458734124999999437, -77.64583333196773651, -2.574251347313719407 ) ) ;
#21925=CARTESIAN_POINT ( 'NONE',  ( 6.123233995736766282E-16, -120.0000000000000000, -5.000000000000000000 ) ) ;
#21927=DIRECTION ( 'NONE',  ( -0.000000000000000000, 1.000000000000000000, -0.000000000000000000 ) ) ;
#21931=CARTESIAN_POINT ( 'NONE',  ( -3.152548672688508926E-16, -9.812499998634406140, -5.148502694627439702 ) ) ;
#21933=CARTESIAN_POINT ( 'NONE',  ( -6.972266317189433020E-16, -38.25000000000000000, -5.000000000000000000 ) ) ;
#21934=CARTESIAN_POINT ( 'NONE',  ( 1.339745962155627135, 17.70534180126147916, -4.999999999999991118 ) ) ;
#21935=CARTESIAN_POINT ( 'NONE',  ( -2.229367062500000163, -8.729166665301073991, -3.861377020970580443 ) ) ;
#21936=CARTESIAN_POINT ( 'NONE',  ( 0.000000000000000000, -120.0000000000000000, 0.000000000000000000 ) ) ;
#21941=ORIENTED_EDGE ( 'NONE', *, *, #7587, .F. ) ;
#21942=CARTESIAN_POINT ( 'NONE',  ( -2.229367062499996610, -84.14583333196773651, 3.861377020970582219 ) ) ;
#21943=CARTESIAN_POINT ( 'NONE',  ( -1.339745962155610925, -67.79465819873851729, 5.000000000000000000 ) ) ;
#21944=CARTESIAN_POINT ( 'NONE',  ( 9.457646018065525792E-16, -3.062499998634407472, 5.148502694627439702 ) ) ;
#21945=FACE_OUTER_BOUND ( 'NONE', #27446, .T. ) ;
#21948=CARTESIAN_POINT ( 'NONE',  ( -5.000000000000000000, -29.87499999726881228, 0.000000000000000000 ) ) ;
#21951=CARTESIAN_POINT ( 'NONE',  ( -4.458734124999999437, 22.60416666803225993, -2.574251347313719407 ) ) ;
#21954=CARTESIAN_POINT ( 'NONE',  ( -2.229367062499996610, -49.14583333196772941, 3.861377020970582219 ) ) ;
#21955=CARTESIAN_POINT ( 'NONE',  ( 4.458734124999999437, -35.06249999863440792, -5.460374474430324690E-16 ) ) ;
#21958=CARTESIAN_POINT ( 'NONE',  ( 2.500000000000002220, 14.33333333333333393, 4.330127018922192761 ) ) ;
#21961=CARTESIAN_POINT ( 'NONE',  ( -2.229367062499996610, -41.14583333196773651, 3.861377020970582219 ) ) ;
#21962=CARTESIAN_POINT ( 'NONE',  ( 5.000000000000000888, -76.45833333060215864, 2.886751345948126879 ) ) ;
#21963=ADVANCED_FACE ( 'NONE', ( #41977 ), #17222, .T. ) ;
#21967=( BOUNDED_CURVE ( )  B_SPLINE_CURVE ( 2, ( #13593, #32576, #8764, #28372, #7511, #47059, #46736, #2682, #22625 ),
 .UNSPECIFIED., .F., .F. ) 
 B_SPLINE_CURVE_WITH_KNOTS ( ( 3, 2, 2, 2, 3 ),
 ( 0.09821428571428571230, 0.09880952380952380543, 0.1000000000000000056, 0.1011904761904761918, 0.1017857142857142849 ),
 .UNSPECIFIED. ) 
 CURVE ( )  GEOMETRIC_REPRESENTATION_ITEM ( )  RATIONAL_B_SPLINE_CURVE ( ( 0.9330127018922194093, 0.9330127018922194093, 1.000000000000000000, 0.8660254037844387076, 1.000000000000000000, 0.8660254037844387076, 1.000000000000000000, 0.9330127018922194093, 0.9330127018922194093 ) ) 
 REPRESENTATION_ITEM ( '' )  );
#21968=CARTESIAN_POINT ( 'NONE',  ( -6.972266317189433020E-16, -64.12499999726880162, -5.000000000000000000 ) ) ;
#21969=CARTESIAN_POINT ( 'NONE',  ( -2.229367062499996610, -84.39583333196773651, 3.861377020970582219 ) ) ;
#21971=CARTESIAN_POINT ( 'NONE',  ( 1.975475456537005874E-15, -63.74999999999998579, 5.000000000000000000 ) ) ;
#21972=CARTESIAN_POINT ( 'NONE',  ( 5.000000000000000888, -34.58333333333332860, 2.886751345948126879 ) ) ;
#21977=CARTESIAN_POINT ( 'NONE',  ( -2.229367062499996610, -93.14583333196773651, 3.861377020970582219 ) ) ;
#21978=CARTESIAN_POINT ( 'NONE',  ( -3.152548672688508926E-16, 11.18750000136559564, -5.148502694627439702 ) ) ;
#21979=CARTESIAN_POINT ( 'NONE',  ( -5.000000000000000000, 14.12500000273118594, 0.000000000000000000 ) ) ;
#21980=CARTESIAN_POINT ( 'NONE',  ( -5.000000000000000000, -34.87499999726881583, 0.000000000000000000 ) ) ;
#21984=EDGE_CURVE ( 'NONE', #24823, #54905, #37799, .T. ) ;
#21990=CARTESIAN_POINT ( 'NONE',  ( 5.000000000000000888, -96.58333333333332860, 2.886751345948126879 ) ) ;
#21992=CARTESIAN_POINT ( 'NONE',  ( 2.229367062499998831, -14.89583333196773474, -3.861377020970580887 ) ) ;
#22000=ORIENTED_EDGE ( 'NONE', *, *, #52040, .F. ) ;
#22002=VERTEX_POINT ( 'NONE', #61619 ) ;
#22003=CARTESIAN_POINT ( 'NONE',  ( 9.457646018065525792E-16, -62.31249999863440792, 5.148502694627439702 ) ) ;
#22009=DIRECTION ( 'NONE',  ( 0.000000000000000000, 0.000000000000000000, 1.000000000000000000 ) ) ;
#22012=ORIENTED_EDGE ( 'NONE', *, *, #27238, .T. ) ;
#22014=CARTESIAN_POINT ( 'NONE',  ( -3.152548672688508926E-16, 10.43750000136559386, -5.148502694627439702 ) ) ;
#22020=ORIENTED_EDGE ( 'NONE', *, *, #37785, .T. ) ;
#22021=CARTESIAN_POINT ( 'NONE',  ( 4.458734124999998549, -70.72916666530107932, -2.574251347313721627 ) ) ;
#22023=CARTESIAN_POINT ( 'NONE',  ( 2.229367062500001939, 13.02083333469892779, 3.861377020970579999 ) ) ;
#22024=CARTESIAN_POINT ( 'NONE',  ( 5.000000000000000000, -60.37499999726880873, -6.123233995736766282E-16 ) ) ;
#22025=LINE ( 'NONE', #61905, #36741 ) ;
#22026=CARTESIAN_POINT ( 'NONE',  ( 4.458734125000001214, -55.14583333196772941, 2.574251347313718519 ) ) ;
#22027=CARTESIAN_POINT ( 'NONE',  ( 5.000000000000000888, -15.45833333060214265, 2.886751345948126879 ) ) ;
#22028=EDGE_CURVE ( 'NONE', #2572, #3938, #39100, .T. ) ;
#22029=CARTESIAN_POINT ( 'NONE',  ( 0.000000000000000000, -120.0000000000000000, 0.000000000000000000 ) ) ;
#22031=CARTESIAN_POINT ( 'NONE',  ( -1.339745962155613812, -84.08034179853027013, -5.000000000000000000 ) ) ;
#22032=CARTESIAN_POINT ( 'NONE',  ( 2.229367062499998831, -20.89583333196774007, -3.861377020970580887 ) ) ;
#22034=CARTESIAN_POINT ( 'NONE',  ( -5.000000000000000000, -102.0833333333333286, -2.886751345948128211 ) ) ;
#22035=CARTESIAN_POINT ( 'NONE',  ( 1.060575238724906964E-15, 29.25000000000000000, 5.773502691896257311 ) ) ;
#22037=VERTEX_POINT ( 'NONE', #2757 ) ;
#22038=CARTESIAN_POINT ( 'NONE',  ( -2.229367062500000163, -102.7291666653010651, -3.861377020970580443 ) ) ;
#22039=CARTESIAN_POINT ( 'NONE',  ( -4.458734124999999437, -24.31249999863440436, 0.000000000000000000 ) ) ;
#22040=CARTESIAN_POINT ( 'NONE',  ( 5.000000000000000000, -65.29166666393548724, -2.886751345948129988 ) ) ;
#22043=CARTESIAN_POINT ( 'NONE',  ( -2.229367062499996610, -25.14583333196773651, 3.861377020970582219 ) ) ;
#22044=CARTESIAN_POINT ( 'NONE',  ( 2.229367062500001939, -68.22916666530106511, 3.861377020970579999 ) ) ;
#22045=CARTESIAN_POINT ( 'NONE',  ( 5.000000000000000888, 8.416666666666666075, 2.886751345948126879 ) ) ;
#22047=DIRECTION ( 'NONE',  ( -0.000000000000000000, -1.000000000000000000, -0.000000000000000000 ) ) ;
#22049=CARTESIAN_POINT ( 'NONE',  ( -4.999999999999999112, -17.91666666666666430, 2.886751345948131764 ) ) ;
#22051=ORIENTED_EDGE ( 'NONE', *, *, #47579, .T. ) ;
#22052=CARTESIAN_POINT ( 'NONE',  ( -4.458734124999999437, 29.68750000136559208, 0.000000000000000000 ) ) ;
#22058=EDGE_CURVE ( 'NONE', #42260, #40791, #61308, .T. ) ;
#22059=CARTESIAN_POINT ( 'NONE',  ( 8.660254037844342889, 30.00000000000000000, 0.000000000000000000 ) ) ;
#22060=AXIS2_PLACEMENT_3D ( 'NONE', #21366, #37120, #51903 ) ;
#22063=CARTESIAN_POINT ( 'NONE',  ( -6.972266317189433020E-16, -87.12499999726880162, -5.000000000000000000 ) ) ;
#22066=ORIENTED_EDGE ( 'NONE', *, *, #9960, .T. ) ;
#22067=CARTESIAN_POINT ( 'NONE',  ( -2.499999999999996447, -29.70833333060215153, 4.330127018922195425 ) ) ;
#22068=ORIENTED_EDGE ( 'NONE', *, *, #57897, .F. ) ;
#22073=VERTEX_POINT ( 'NONE', #51649 ) ;
#22081=CARTESIAN_POINT ( 'NONE',  ( -5.000000000000000000, 20.99999999999999645, 0.000000000000000000 ) ) ;
#22083=ADVANCED_FACE ( 'NONE', ( #37173 ), #57736, .T. ) ;
#22085=CARTESIAN_POINT ( 'NONE',  ( 2.229367062500001939, -78.97916666530106511, 3.861377020970579999 ) ) ;
#22086=CARTESIAN_POINT ( 'NONE',  ( -2.229367062500000163, 23.52083333469892779, -3.861377020970580443 ) ) ;
#22087=ADVANCED_FACE ( 'NONE', ( #47444 ), #23012, .T. ) ;
#22093=CARTESIAN_POINT ( 'NONE',  ( 2.499999999999998668, 0.7916666693978530178, -4.330127018922193649 ) ) ;
#22094=CARTESIAN_POINT ( 'NONE',  ( -5.000000000000000000, -82.99999999999998579, 0.000000000000000000 ) ) ;
#22096=CARTESIAN_POINT ( 'NONE',  ( 0.000000000000000000, -120.0000000000000000, 0.000000000000000000 ) ) ;
#22097=CARTESIAN_POINT ( 'NONE',  ( -4.458734124999997661, -53.22916666530107932, 2.574251347313722516 ) ) ;
#22099=CARTESIAN_POINT ( 'NONE',  ( 2.229367062500001939, 27.02083333469892423, 3.861377020970579999 ) ) ;
#22101=EDGE_CURVE ( 'NONE', #34069, #7844, #38724, .T. ) ;
#22102=CARTESIAN_POINT ( 'NONE',  ( -5.000000000000000000, -108.0833333333333428, -2.886751345948128211 ) ) ;
#22105=CARTESIAN_POINT ( 'NONE',  ( 2.229367062499998831, -38.89583333196773651, -3.861377020970580887 ) ) ;
#22106=CARTESIAN_POINT ( 'NONE',  ( -5.000000000000000000, -0.8749999972688139449, 0.000000000000000000 ) ) ;
#22111=EDGE_CURVE ( 'NONE', #27444, #44174, #43856, .T. ) ;
#22112=CARTESIAN_POINT ( 'NONE',  ( -2.229367062500000163, -103.4791666653010651, -3.861377020970580443 ) ) ;
#22113=CARTESIAN_POINT ( 'NONE',  ( 4.458734124999998549, -3.979166665301070438, -2.574251347313721627 ) ) ;
#22114=ORIENTED_EDGE ( 'NONE', *, *, #55706, .T. ) ;
#22116=CARTESIAN_POINT ( 'NONE',  ( 4.458734124999998549, -91.72916666530106511, -2.574251347313721627 ) ) ;
#22119=CARTESIAN_POINT ( 'NONE',  ( -4.458734124999998549, -89.47916666530106511, 2.574251347313722516 ) ) ;
#22121=CARTESIAN_POINT ( 'NONE',  ( 0.000000000000000000, -120.0000000000000000, 5.000000000000000000 ) ) ;
#22123=CARTESIAN_POINT ( 'NONE',  ( -2.229367062499996610, -7.145833331967735624, 3.861377020970582219 ) ) ;
#22124=CARTESIAN_POINT ( 'NONE',  ( 4.458734124999998549, 14.02083333469892779, -2.574251347313721627 ) ) ;
#22125=CARTESIAN_POINT ( 'NONE',  ( 9.457646018065525792E-16, -51.31249999863440792, 5.148502694627439702 ) ) ;
#22132=CARTESIAN_POINT ( 'NONE',  ( -2.229367062500000163, -82.47916666530106511, -3.861377020970580443 ) ) ;
#22133=CARTESIAN_POINT ( 'NONE',  ( -4.458734124999998549, 26.52083333469892779, 2.574251347313722516 ) ) ;
#22140=CARTESIAN_POINT ( 'NONE',  ( -5.000000000000000000, -66.08333333333332860, -2.886751345948128211 ) ) ;
#22141=CARTESIAN_POINT ( 'NONE',  ( -1.339745962155613368, 29.79465819873851729, -5.000000000000000000 ) ) ;
#22143=ORIENTED_EDGE ( 'NONE', *, *, #60217, .T. ) ;
#22144=CARTESIAN_POINT ( 'NONE',  ( 1.975475456537005874E-15, -61.62499999726880873, 5.000000000000000000 ) ) ;
#22145=CARTESIAN_POINT ( 'NONE',  ( 5.000000000000000888, 7.416666666666665186, 2.886751345948126879 ) ) ;
#22146=CARTESIAN_POINT ( 'NONE',  ( 2.500000000000002220, -40.66666666666667140, 4.330127018922192761 ) ) ;
#22150=VECTOR ( 'NONE', #41869, 1000.000000000000000 ) ;
#22151=( BOUNDED_CURVE ( )  B_SPLINE_CURVE ( 2, ( #42893, #18461, #13939, #63160, #57708, #9426, #33253, #13634, #19394 ),
 .UNSPECIFIED., .F., .F. ) 
 B_SPLINE_CURVE_WITH_KNOTS ( ( 3, 2, 2, 2, 3 ),
 ( 0.8946428571428571841, 0.8952380952380952772, 0.8964285714285714635, 0.8976190476190476497, 0.8982142857142857428 ),
 .UNSPECIFIED. ) 
 CURVE ( )  GEOMETRIC_REPRESENTATION_ITEM ( )  RATIONAL_B_SPLINE_CURVE ( ( 0.9330127018922194093, 0.9330127018922194093, 1.000000000000000000, 0.8660254037844387076, 1.000000000000000000, 0.8660254037844387076, 1.000000000000000000, 0.9330127018922194093, 0.9330127018922194093 ) ) 
 REPRESENTATION_ITEM ( '' )  );
#22157=ORIENTED_EDGE ( 'NONE', *, *, #7863, .F. ) ;
#22160=CARTESIAN_POINT ( 'NONE',  ( -4.458734124999999437, -50.64583333196773651, -2.574251347313719407 ) ) ;
#22162=CARTESIAN_POINT ( 'NONE',  ( -2.499999999999996447, -21.70833333060214798, 4.330127018922195425 ) ) ;
#22163=EDGE_LOOP ( 'NONE', ( #54205, #58051, #54412, #3175 ) ) ;
#22167=CARTESIAN_POINT ( 'NONE',  ( -2.499999999999996447, -58.70833333060214443, 4.330127018922195425 ) ) ;
#22169=CARTESIAN_POINT ( 'NONE',  ( 4.458734125000001214, -101.1458333319677365, 2.574251347313718519 ) ) ;
#22171=ORIENTED_EDGE ( 'NONE', *, *, #6331, .T. ) ;
#22175=CARTESIAN_POINT ( 'NONE',  ( 9.457646018065525792E-16, -5.062499998634401699, 5.148502694627439702 ) ) ;
#22176=CARTESIAN_POINT ( 'NONE',  ( -4.458734124999999437, -97.64583333196773651, -2.574251347313719407 ) ) ;
#22178=CARTESIAN_POINT ( 'NONE',  ( -2.229367062499996610, -23.39583333196773651, 3.861377020970582219 ) ) ;
#22179=CARTESIAN_POINT ( 'NONE',  ( 1.975475456537005874E-15, -74.62499999726880162, 5.000000000000000000 ) ) ;
#22183=EDGE_CURVE ( 'NONE', #62586, #36804, #56804, .T. ) ;
#22184=CARTESIAN_POINT ( 'NONE',  ( 5.000000000000000000, -72.41666666666665719, -2.886751345948130876 ) ) ;
#22187=CARTESIAN_POINT ( 'NONE',  ( 2.229367062500001939, 10.77083333469892956, 3.861377020970579999 ) ) ;
#22189=CARTESIAN_POINT ( 'NONE',  ( -2.500000000000000444, -5.166666666666666963, -4.330127018922193649 ) ) ;
#22190=CARTESIAN_POINT ( 'NONE',  ( 5.000000000000000000, -61.41666666666665719, -2.886751345948130876 ) ) ;
#22191=CARTESIAN_POINT ( 'NONE',  ( -5.000000000000000000, -90.00000000000000000, 0.000000000000000000 ) ) ;
#22192=CARTESIAN_POINT ( 'NONE',  ( -3.152548672688508926E-16, -25.56249999863440436, -5.148502694627439702 ) ) ;
#22194=CARTESIAN_POINT ( 'NONE',  ( 9.457646018065525792E-16, -70.31249999863439371, 5.148502694627439702 ) ) ;
#22195=CARTESIAN_POINT ( 'NONE',  ( 1.975475456537005874E-15, 16.37500000273118417, 5.000000000000000000 ) ) ;
#22200=CARTESIAN_POINT ( 'NONE',  ( 5.000000000000000000, -52.29166666393548013, -2.886751345948129988 ) ) ;
#22202=CARTESIAN_POINT ( 'NONE',  ( -2.229367062499996610, 6.854166668032259935, 3.861377020970582219 ) ) ;
#22203=CYLINDRICAL_SURFACE ( 'NONE', #60263, 5.000000000000000000 ) ;
#22206=CARTESIAN_POINT ( 'NONE',  ( -2.229367062499996610, -71.14583333196773651, 3.861377020970582219 ) ) ;
#22208=( BOUNDED_CURVE ( )  B_SPLINE_CURVE ( 2, ( #27883, #62634, #57800, #12465, #47505, #41719, #33346, #32076, #17291 ),
 .UNSPECIFIED., .F., .F. ) 
 B_SPLINE_CURVE_WITH_KNOTS ( ( 3, 2, 2, 2, 3 ),
 ( 0.4767857142857143127, 0.4773809523809524058, 0.4785714285714285920, 0.4797619047619047783, 0.4803571428571428714 ),
 .UNSPECIFIED. ) 
 CURVE ( )  GEOMETRIC_REPRESENTATION_ITEM ( )  RATIONAL_B_SPLINE_CURVE ( ( 0.9330127018922194093, 0.9330127018922225179, 1.000000000000000000, 0.8660254037844387076, 1.000000000000000000, 0.8660254037844387076, 1.000000000000000000, 0.9330127018922194093, 0.9330127018922194093 ) ) 
 REPRESENTATION_ITEM ( '' )  );
#22209=CARTESIAN_POINT ( 'NONE',  ( -4.999999999999999112, -0.9166666666666664076, 2.886751345948131764 ) ) ;
#22212=CARTESIAN_POINT ( 'NONE',  ( -2.229367062500000163, -65.47916666530106511, -3.861377020970580443 ) ) ;
#22213=CARTESIAN_POINT ( 'NONE',  ( 5.000000000000000000, -94.37499999726881583, -6.123233995736766282E-16 ) ) ;
#22214=CARTESIAN_POINT ( 'NONE',  ( 1.339745962155612702, 5.830341803992665106, -5.000000000000000000 ) ) ;
#22218=CARTESIAN_POINT ( 'NONE',  ( -4.999999999999999112, -46.91666666666665719, 2.886751345948131764 ) ) ;
#22222=CARTESIAN_POINT ( 'NONE',  ( -4.458734124999999437, -110.3124999986343937, 0.000000000000000000 ) ) ;
#22229=ORIENTED_EDGE ( 'NONE', *, *, #38648, .F. ) ;
#22230=CARTESIAN_POINT ( 'NONE',  ( 1.975475456537005874E-15, -100.6249999972688016, 5.000000000000000000 ) ) ;
#22232=ORIENTED_EDGE ( 'NONE', *, *, #62203, .F. ) ;
#22236=CARTESIAN_POINT ( 'NONE',  ( 4.458734124999999437, -35.06249999863440792, -5.460374474430324690E-16 ) ) ;
#22248=CARTESIAN_POINT ( 'NONE',  ( -3.152548672688508926E-16, -83.81249999863439371, -5.148502694627439702 ) ) ;
#22249=VERTEX_POINT ( 'NONE', #53835 ) ;
#22250=CARTESIAN_POINT ( 'NONE',  ( 6.123233995736766282E-16, -120.0000000000000000, -5.000000000000000000 ) ) ;
#22254=CARTESIAN_POINT ( 'NONE',  ( 4.458734124999999437, -10.06249999863440614, -5.460374474430324690E-16 ) ) ;
#22256=CARTESIAN_POINT ( 'NONE',  ( 1.975475456537005874E-15, -84.74999999999998579, 5.000000000000000000 ) ) ;
#22257=DIRECTION ( 'NONE',  ( -0.000000000000000000, 1.000000000000000000, -0.000000000000000000 ) ) ;
#22258=CARTESIAN_POINT ( 'NONE',  ( 2.229367062500001939, -9.229166665301075767, 3.861377020970579999 ) ) ;
#22259=CARTESIAN_POINT ( 'NONE',  ( 6.158835246850666199E-14, 8.875000002731182391, -4.999999999999999112 ) ) ;
#22263=CARTESIAN_POINT ( 'NONE',  ( 2.229367062499998831, 26.10416666803225993, -3.861377020970580887 ) ) ;
#22264=ORIENTED_EDGE ( 'NONE', *, *, #5596, .T. ) ;
#22265=CARTESIAN_POINT ( 'NONE',  ( 4.458734125000000326, -84.89583333196773651, 2.574251347313718519 ) ) ;
#22267=CARTESIAN_POINT ( 'NONE',  ( 4.458734124999999437, -9.812499998634406140, -5.460374474430324690E-16 ) ) ;
#22268=DIRECTION ( 'NONE',  ( 0.000000000000000000, 0.000000000000000000, 1.000000000000000000 ) ) ;
#22269=CYLINDRICAL_SURFACE ( 'NONE', #44844, 5.000000000000000000 ) ;
#22270=CARTESIAN_POINT ( 'NONE',  ( -5.000000000000000000, -36.95833333060213732, -2.886751345948128211 ) ) ;
#22272=CARTESIAN_POINT ( 'NONE',  ( 4.458734124999998549, 24.27083333469892779, -2.574251347313721627 ) ) ;
#22273=CARTESIAN_POINT ( 'NONE',  ( -5.000000000000000000, -20.87499999726881228, 0.000000000000000000 ) ) ;
#22275=CARTESIAN_POINT ( 'NONE',  ( -2.229367062499996610, -52.14583333196773651, 3.861377020970582219 ) ) ;
#22279=CARTESIAN_POINT ( 'NONE',  ( -3.535250795749689387E-16, 16.75000000000000355, -5.773502691896257311 ) ) ;
#22282=CARTESIAN_POINT ( 'NONE',  ( -4.458734124999998549, -46.22916666530106511, 2.574251347313722516 ) ) ;
#22283=CARTESIAN_POINT ( 'NONE',  ( 2.499999999999998668, -81.20833333060213022, -4.330127018922193649 ) ) ;
#22289=CARTESIAN_POINT ( 'NONE',  ( -4.458734124999999437, -86.56249999863439371, 0.000000000000000000 ) ) ;
#22291=CARTESIAN_POINT ( 'NONE',  ( -2.500000000000000444, -32.16666666666666430, -4.330127018922193649 ) ) ;
#22292=CARTESIAN_POINT ( 'NONE',  ( -2.500000000000000444, 23.83333333333333215, -4.330127018922193649 ) ) ;
#22293=VERTEX_POINT ( 'NONE', #4019 ) ;
#22295=ORIENTED_EDGE ( 'NONE', *, *, #59480, .F. ) ;
#22296=CARTESIAN_POINT ( 'NONE',  ( -4.458734124999999437, -90.31249999863440792, 0.000000000000000000 ) ) ;
#22297=CARTESIAN_POINT ( 'NONE',  ( -2.229367062499996610, 14.60416666803226171, 3.861377020970582219 ) ) ;
#22298=CARTESIAN_POINT ( 'NONE',  ( 2.499999999999998668, 15.79166666939785202, -4.330127018922193649 ) ) ;
#22300=EDGE_CURVE ( 'NONE', #12016, #15518, #25974, .T. ) ;
#22303=CARTESIAN_POINT ( 'NONE',  ( 5.000000000000000000, -80.50000000000000000, -6.123233995736766282E-16 ) ) ;
#22310=CARTESIAN_POINT ( 'NONE',  ( -2.499999999999996447, -42.83333333333333570, 4.330127018922195425 ) ) ;
#22311=CARTESIAN_POINT ( 'NONE',  ( 2.229367062500001939, -20.22916666530107221, 3.861377020970579999 ) ) ;
#22320=CARTESIAN_POINT ( 'NONE',  ( -6.972266317189433020E-16, -85.12499999726880162, -5.000000000000000000 ) ) ;
#22321=ORIENTED_EDGE ( 'NONE', *, *, #18546, .F. ) ;
#22322=CARTESIAN_POINT ( 'NONE',  ( -4.458734124999998549, -62.47916666530106511, 2.574251347313722516 ) ) ;
#22328=CARTESIAN_POINT ( 'NONE',  ( -5.000000000000000000, 27.04166666939785202, -2.886751345948128211 ) ) ;
#22332=ORIENTED_EDGE ( 'NONE', *, *, #56313, .F. ) ;
#22338=CARTESIAN_POINT ( 'NONE',  ( -4.458734124999999437, 8.687500001365595637, 0.000000000000000000 ) ) ;
#22341=CARTESIAN_POINT ( 'NONE',  ( 1.975475456537005874E-15, -23.62499999726880873, 5.000000000000000000 ) ) ;
#22343=ORIENTED_EDGE ( 'NONE', *, *, #15502, .F. ) ;
#22344=CARTESIAN_POINT ( 'NONE',  ( -2.229367062500000163, -69.47916666530107932, -3.861377020970580443 ) ) ;
#22345=CARTESIAN_POINT ( 'NONE',  ( 1.975475456537005874E-15, -10.62499999726881228, 5.000000000000000000 ) ) ;
#22346=CARTESIAN_POINT ( 'NONE',  ( 4.458734125000001214, 11.10416666803225993, 2.574251347313718519 ) ) ;
#22348=CARTESIAN_POINT ( 'NONE',  ( -4.458734124999998549, -60.47916666530105800, 2.574251347313722516 ) ) ;
#22349=CARTESIAN_POINT ( 'NONE',  ( -2.499999999999996447, -16.70833333060214443, 4.330127018922195425 ) ) ;
#22350=CARTESIAN_POINT ( 'NONE',  ( 1.975475456537005874E-15, -32.62499999726880873, 5.000000000000000000 ) ) ;
#22353=CARTESIAN_POINT ( 'NONE',  ( 2.229367062499998831, -34.64583333196772941, -3.861377020970580887 ) ) ;
#22354=CARTESIAN_POINT ( 'NONE',  ( 4.458734124999998549, -20.97916666530107221, -2.574251347313721627 ) ) ;
#22357=CARTESIAN_POINT ( 'NONE',  ( -4.458734124999999437, -110.3124999986343937, 0.000000000000000000 ) ) ;
#22360=CARTESIAN_POINT ( 'NONE',  ( 4.458734124999999437, -104.0624999986344079, -5.460374474430324690E-16 ) ) ;
#22361=CARTESIAN_POINT ( 'NONE',  ( -4.458734124999999437, -32.39583333196773651, -2.574251347313719407 ) ) ;
#22362=CARTESIAN_POINT ( 'NONE',  ( -3.535250795749689387E-16, -64.12499999726881583, -5.773502691896257311 ) ) ;
#22365=CARTESIAN_POINT ( 'NONE',  ( -4.458734124999997661, -31.22916666530106866, 2.574251347313722516 ) ) ;
#22366=CARTESIAN_POINT ( 'NONE',  ( 9.457646018065525792E-16, -68.31249999863440792, 5.148502694627439702 ) ) ;
#22367=LINE ( 'NONE', #55517, #56221 ) ;
#22369=CARTESIAN_POINT ( 'NONE',  ( 1.975475456537005874E-15, -32.62499999726880873, 5.000000000000000000 ) ) ;
#22371=CARTESIAN_POINT ( 'NONE',  ( 2.500000000000002220, -15.66666666666666963, 4.330127018922192761 ) ) ;
#22373=EDGE_LOOP ( 'NONE', ( #26585, #57752, #5361, #55627 ) ) ;
#22376=VECTOR ( 'NONE', #57240, 1000.000000000000000 ) ;
#22378=CARTESIAN_POINT ( 'NONE',  ( -5.000000000000000000, -1.083333333333331927, -2.886751345948128211 ) ) ;
#22380=EDGE_CURVE ( 'NONE', #41, #25378, #19741, .T. ) ;
#22388=EDGE_LOOP ( 'NONE', ( #61387, #17173, #12323, #20004 ) ) ;
#22399=ORIENTED_EDGE ( 'NONE', *, *, #28102, .T. ) ;
#22403=CARTESIAN_POINT ( 'NONE',  ( 1.975475456537005874E-15, -42.74999999999999289, 5.000000000000000000 ) ) ;
#22407=ORIENTED_EDGE ( 'NONE', *, *, #3927, .T. ) ;
#22408=CARTESIAN_POINT ( 'NONE',  ( -3.152548672688508926E-16, -80.56249999863440792, -5.148502694627439702 ) ) ;
#22409=CARTESIAN_POINT ( 'NONE',  ( -2.229367062499996610, 21.85416666803226349, 3.861377020970582219 ) ) ;
#22411=EDGE_LOOP ( 'NONE', ( #19658, #18192, #46371, #35893 ) ) ;
#22416=CARTESIAN_POINT ( 'NONE',  ( 0.000000000000000000, -120.0000000000000000, 0.000000000000000000 ) ) ;
#22418=VECTOR ( 'NONE', #37451, 1000.000000000000000 ) ;
#22419=CARTESIAN_POINT ( 'NONE',  ( -6.972266317189433020E-16, -20.24999999999999645, -5.000000000000000000 ) ) ;
#22420=CARTESIAN_POINT ( 'NONE',  ( 4.458734125000000326, -53.89583333196773651, 2.574251347313718519 ) ) ;
#22422=CARTESIAN_POINT ( 'NONE',  ( -4.458734124999998549, 27.77083333469892423, 2.574251347313722516 ) ) ;
#22423=AXIS2_PLACEMENT_3D ( 'NONE', #16431, #55994, #6471 ) ;
#22424=CARTESIAN_POINT ( 'NONE',  ( 5.000000000000000000, -104.4166666666666572, -2.886751345948129988 ) ) ;
#22426=CARTESIAN_POINT ( 'NONE',  ( -2.229367062500000163, -38.72916666530107221, -3.861377020970580443 ) ) ;
#22428=CARTESIAN_POINT ( 'NONE',  ( 2.499999999999998668, 1.791666669397853795, -4.330127018922193649 ) ) ;
#22432=CARTESIAN_POINT ( 'NONE',  ( -4.458734124999999437, -101.3124999986344079, 0.000000000000000000 ) ) ;
#22434=CARTESIAN_POINT ( 'NONE',  ( -2.229367062499996610, -3.395833331967738733, 3.861377020970582219 ) ) ;
#22435=VERTEX_POINT ( 'NONE', #21668 ) ;
#22437=CARTESIAN_POINT ( 'NONE',  ( -2.229367062499996610, -91.14583333196773651, 3.861377020970582219 ) ) ;
#22439=CARTESIAN_POINT ( 'NONE',  ( 2.229367062499998831, -88.89583333196773651, -3.861377020970580887 ) ) ;
#22441=CARTESIAN_POINT ( 'NONE',  ( 1.339745962155641346, -2.169658196007335338, -4.999999999999983125 ) ) ;
#22443=CARTESIAN_POINT ( 'NONE',  ( -2.229367062500000163, -12.47916666530107044, -3.861377020970580443 ) ) ;
#22444=CARTESIAN_POINT ( 'NONE',  ( -3.152548672688508926E-16, 19.18750000136559208, -5.148502694627439702 ) ) ;
#22445=CARTESIAN_POINT ( 'NONE',  ( -3.152548672688508926E-16, -52.81249999863440792, -5.148502694627439702 ) ) ;
#22448=CARTESIAN_POINT ( 'NONE',  ( 5.000000000000000000, -84.49999999999998579, -6.123233995736766282E-16 ) ) ;
#22452=CARTESIAN_POINT ( 'NONE',  ( 5.000000000000000000, 26.62500000273118772, -6.123233995736766282E-16 ) ) ;
#22453=CARTESIAN_POINT ( 'NONE',  ( -2.229367062500000163, -78.47916666530106511, -3.861377020970580443 ) ) ;
#22454=CARTESIAN_POINT ( 'NONE',  ( 9.457646018065525792E-16, 26.68750000136559564, 5.148502694627439702 ) ) ;
#22458=EDGE_CURVE ( 'NONE', #58717, #20660, #56427, .T. ) ;
#22462=CARTESIAN_POINT ( 'NONE',  ( 5.000000000000000000, -64.50000000000000000, -6.123233995736766282E-16 ) ) ;
#22463=DIRECTION ( 'NONE',  ( -0.000000000000000000, 1.000000000000000000, -0.000000000000000000 ) ) ;
#22466=CARTESIAN_POINT ( 'NONE',  ( -2.480964764533239819E-13, -94.75000000000000000, 5.000000000000000000 ) ) ;
#22468=CARTESIAN_POINT ( 'NONE',  ( -2.500000000000000444, 27.83333333333333215, -4.330127018922193649 ) ) ;
#22469=CARTESIAN_POINT ( 'NONE',  ( -1.339745962155613812, -109.0803417985302843, -5.000000000000000000 ) ) ;
#22483=CARTESIAN_POINT ( 'NONE',  ( 9.457646018065525792E-16, -49.31249999863441502, 5.148502694627439702 ) ) ;
#22492=CARTESIAN_POINT ( 'NONE',  ( -2.229367062500000163, -100.7291666653010651, -3.861377020970580443 ) ) ;
#22493=CARTESIAN_POINT ( 'NONE',  ( -6.972266317189433020E-16, 10.75000000000000000, -5.000000000000000000 ) ) ;
#22497=CARTESIAN_POINT ( 'NONE',  ( 2.500000000000002220, -60.66666666666665719, 4.330127018922192761 ) ) ;
#22498=CARTESIAN_POINT ( 'NONE',  ( -2.229367062500000163, -8.479166665301073991, -3.861377020970580443 ) ) ;
#22499=CARTESIAN_POINT ( 'NONE',  ( 4.458734124999999437, -95.06249999863440792, -5.460374474430324690E-16 ) ) ;
#22501=CARTESIAN_POINT ( 'NONE',  ( 2.229367062500001939, -22.22916666530107221, 3.861377020970579999 ) ) ;
#22509=CARTESIAN_POINT ( 'NONE',  ( -2.229367062499996610, 9.604166668032261711, 3.861377020970582219 ) ) ;
#22511=CARTESIAN_POINT ( 'NONE',  ( -4.999999999999998224, -80.91666666666667140, 2.886751345948131764 ) ) ;
#22512=CARTESIAN_POINT ( 'NONE',  ( -6.972266317189433020E-16, -61.25000000000000000, -5.000000000000000000 ) ) ;
#22513=CARTESIAN_POINT ( 'NONE',  ( -5.000000000000000000, -93.08333333333331439, -2.886751345948128211 ) ) ;
#22514=CARTESIAN_POINT ( 'NONE',  ( -3.152548672688508926E-16, -23.56249999863440436, -5.148502694627439702 ) ) ;
#22516=CARTESIAN_POINT ( 'NONE',  ( 2.229367062500001939, -70.22916666530107932, 3.861377020970579999 ) ) ;
#22519=LINE ( 'NONE', #46958, #42744 ) ;
#22520=( BOUNDED_CURVE ( )  B_SPLINE_CURVE ( 2, ( #48743, #4686, #38776, #4379, #29430, #28505, #58414, #63562, #38172 ),
 .UNSPECIFIED., .F., .F. ) 
 B_SPLINE_CURVE_WITH_KNOTS ( ( 3, 2, 2, 2, 3 ),
 ( 0.4696428571428571397, 0.4702380952380952328, 0.4714285714285714191, 0.4726190476190476053, 0.4732142857142856984 ),
 .UNSPECIFIED. ) 
 CURVE ( )  GEOMETRIC_REPRESENTATION_ITEM ( )  RATIONAL_B_SPLINE_CURVE ( ( 0.9330127018922194093, 0.9330127018922194093, 1.000000000000000000, 0.8660254037844387076, 1.000000000000000000, 0.8660254037844387076, 1.000000000000000000, 0.9330127018922194093, 0.9330127018922194093 ) ) 
 REPRESENTATION_ITEM ( '' )  );
#22522=CARTESIAN_POINT ( 'NONE',  ( 2.229367062500001939, 6.020833334698927786, 3.861377020970579999 ) ) ;
#22523=CARTESIAN_POINT ( 'NONE',  ( -5.000000000000000000, -62.87499999726880873, 0.000000000000000000 ) ) ;
#22526=CARTESIAN_POINT ( 'NONE',  ( 4.458734124999999437, -70.81249999863439371, -5.460374474430324690E-16 ) ) ;
#22528=CARTESIAN_POINT ( 'NONE',  ( 1.060575238724906964E-15, 0.2500000000000002220, 5.773502691896257311 ) ) ;
#22531=CARTESIAN_POINT ( 'NONE',  ( -2.229367062500000163, -66.47916666530106511, -3.861377020970580443 ) ) ;
#22532=CARTESIAN_POINT ( 'NONE',  ( 5.000000000000000000, -102.3749999972688158, -6.123233995736766282E-16 ) ) ;
#22533=( BOUNDED_CURVE ( )  B_SPLINE_CURVE ( 2, ( #55973, #31193, #49539, #20277, #55659, #29912, #25095, #59523, #1956 ),
 .UNSPECIFIED., .F., .F. ) 
 B_SPLINE_CURVE_WITH_KNOTS ( ( 3, 2, 2, 2, 3 ),
 ( 0.6160714285714286031, 0.6166666666666666963, 0.6178571428571428825, 0.6190476190476190688, 0.6196428571428571619 ),
 .UNSPECIFIED. ) 
 CURVE ( )  GEOMETRIC_REPRESENTATION_ITEM ( )  RATIONAL_B_SPLINE_CURVE ( ( 0.9330127018922194093, 0.9330127018922194093, 1.000000000000000000, 0.8660254037844387076, 1.000000000000000000, 0.8660254037844387076, 1.000000000000000000, 0.9330127018922194093, 0.9330127018922194093 ) ) 
 REPRESENTATION_ITEM ( '' )  );
#22534=CARTESIAN_POINT ( 'NONE',  ( -6.972266317189433020E-16, -41.24999999999998579, -5.000000000000000000 ) ) ;
#22537=CARTESIAN_POINT ( 'NONE',  ( 2.229367062500001939, -104.2291666653010651, 3.861377020970579999 ) ) ;
#22539=CARTESIAN_POINT ( 'NONE',  ( -2.499999999999996447, -47.83333333333332149, 4.330127018922195425 ) ) ;
#22540=CARTESIAN_POINT ( 'NONE',  ( -5.000000000000000000, -23.08333333333333215, -2.886751345948128211 ) ) ;
#22542=ORIENTED_EDGE ( 'NONE', *, *, #6070, .F. ) ;
#22546=CARTESIAN_POINT ( 'NONE',  ( -5.000000000000000000, -6.083333333333336590, -2.886751345948128211 ) ) ;
#22549=ORIENTED_EDGE ( 'NONE', *, *, #45248, .F. ) ;
#22557=CARTESIAN_POINT ( 'NONE',  ( 4.458734125000001214, -37.14583333196773651, 2.574251347313718519 ) ) ;
#22559=CARTESIAN_POINT ( 'NONE',  ( 1.975475456537005874E-15, -82.74999999999998579, 5.000000000000000000 ) ) ;
#22564=VECTOR ( 'NONE', #14431, 1000.000000000000000 ) ;
#22569=CARTESIAN_POINT ( 'NONE',  ( -5.000000000000000000, -93.95833333060213022, -2.886751345948128211 ) ) ;
#22570=CARTESIAN_POINT ( 'NONE',  ( -4.458734124999999437, -81.64583333196773651, -2.574251347313719407 ) ) ;
#22572=ORIENTED_EDGE ( 'NONE', *, *, #59503, .T. ) ;
#22574=DIRECTION ( 'NONE',  ( 0.000000000000000000, 0.000000000000000000, 1.000000000000000000 ) ) ;
#22576=CARTESIAN_POINT ( 'NONE',  ( 4.458734124999998549, -40.72916666530107221, -2.574251347313721627 ) ) ;
#22577=CARTESIAN_POINT ( 'NONE',  ( -4.458734124999999437, -9.562499998634406140, 0.000000000000000000 ) ) ;
#22580=CARTESIAN_POINT ( 'NONE',  ( -2.499999999999996447, -1.833333333333332593, 4.330127018922195425 ) ) ;
#22581=CARTESIAN_POINT ( 'NONE',  ( 2.229367062500001939, -5.229166665301071326, 3.861377020970579999 ) ) ;
#22587=CARTESIAN_POINT ( 'NONE',  ( 9.457646018065525792E-16, 26.68750000136559564, 5.148502694627439702 ) ) ;
#22588=VERTEX_POINT ( 'NONE', #41574 ) ;
#22589=CARTESIAN_POINT ( 'NONE',  ( -2.229367062500000163, -88.47916666530106511, -3.861377020970580443 ) ) ;
#22590=CARTESIAN_POINT ( 'NONE',  ( -6.972266317189433020E-16, -78.24999999999998579, -5.000000000000000000 ) ) ;
#22591=CARTESIAN_POINT ( 'NONE',  ( -3.152548672688508926E-16, -9.562499998634406140, -5.148502694627439702 ) ) ;
#22592=CARTESIAN_POINT ( 'NONE',  ( -1.339745962155613812, 19.79465819873851729, -5.000000000000000000 ) ) ;
#22595=CARTESIAN_POINT ( 'NONE',  ( -5.000000000000000000, -35.95833333060213732, -2.886751345948128211 ) ) ;
#22597=CARTESIAN_POINT ( 'NONE',  ( 4.458734125000000326, 27.10416666803225993, 2.574251347313718519 ) ) ;
#22598=CARTESIAN_POINT ( 'NONE',  ( -5.000000000000000000, -97.87499999726881583, 0.000000000000000000 ) ) ;
#22600=CARTESIAN_POINT ( 'NONE',  ( 9.457646018065525792E-16, -57.06249999863440081, 5.148502694627439702 ) ) ;
#22603=CARTESIAN_POINT ( 'NONE',  ( -3.535250795749689387E-16, 14.75000000000000000, -5.773502691896257311 ) ) ;
#22607=CARTESIAN_POINT ( 'NONE',  ( 4.458734125000001214, -49.89583333196772941, 2.574251347313718519 ) ) ;
#22608=CARTESIAN_POINT ( 'NONE',  ( -4.999999999999999112, -84.79166666393547303, 2.886751345948131764 ) ) ;
#22610=CARTESIAN_POINT ( 'NONE',  ( 5.000000000000000888, -37.45833333060213732, 2.886751345948126879 ) ) ;
#22611=CARTESIAN_POINT ( 'NONE',  ( -5.000000000000000000, -63.95833333060213732, -2.886751345948128211 ) ) ;
#22612=CARTESIAN_POINT ( 'NONE',  ( -2.229367062500000163, -86.72916666530107932, -3.861377020970580443 ) ) ;
#22614=CARTESIAN_POINT ( 'NONE',  ( 5.000000000000000000, -34.41666666666666430, -2.886751345948129988 ) ) ;
#22615=CARTESIAN_POINT ( 'NONE',  ( 2.500000000000002220, 8.458333336064518093, 4.330127018922192761 ) ) ;
#22619=CARTESIAN_POINT ( 'NONE',  ( -2.229367062500000163, -95.47916666530107932, -3.861377020970580443 ) ) ;
#22620=CARTESIAN_POINT ( 'NONE',  ( 4.458734125000001214, 14.85416666803225993, 2.574251347313718519 ) ) ;
#22621=CARTESIAN_POINT ( 'NONE',  ( -3.535250795749689387E-16, 17.87500000273118417, -5.773502691896257311 ) ) ;
#22625=CARTESIAN_POINT ( 'NONE',  ( -6.972266317189433020E-16, 14.87500000273118594, -5.000000000000000000 ) ) ;
#22626=CARTESIAN_POINT ( 'NONE',  ( -2.500000000000000444, -82.16666666666667140, -4.330127018922193649 ) ) ;
#22632=CARTESIAN_POINT ( 'NONE',  ( -5.000000000000000000, -43.08333333333333570, -2.886751345948128211 ) ) ;
#22633=CARTESIAN_POINT ( 'NONE',  ( -4.458734124999999437, -21.56249999863440436, 0.000000000000000000 ) ) ;
#22645=CARTESIAN_POINT ( 'NONE',  ( -4.458734124999998549, -68.47916666530106511, 2.574251347313722516 ) ) ;
#22647=CARTESIAN_POINT ( 'NONE',  ( -4.769696007084728073, -120.0000000000000000, 1.499999999999999556 ) ) ;
#22649=VECTOR ( 'NONE', #63316, 1000.000000000000000 ) ;
#22655=ORIENTED_EDGE ( 'NONE', *, *, #56976, .T. ) ;
#22656=CARTESIAN_POINT ( 'NONE',  ( -5.000000000000000000, 2.041666669397854239, -2.886751345948128211 ) ) ;
#22657=CARTESIAN_POINT ( 'NONE',  ( 4.458734124999998549, 10.27083333469892779, -2.574251347313721627 ) ) ;
#22660=CARTESIAN_POINT ( 'NONE',  ( -6.972266317189433020E-16, -1.124999997268814278, -5.000000000000000000 ) ) ;
#22663=CARTESIAN_POINT ( 'NONE',  ( -2.229367062500000163, -71.47916666530107932, -3.861377020970580443 ) ) ;
#22665=CARTESIAN_POINT ( 'NONE',  ( -4.458734124999998549, 6.770833334698928674, 2.574251347313722516 ) ) ;
#22666=CARTESIAN_POINT ( 'NONE',  ( -4.999999999999998224, -41.91666666666667140, 2.886751345948131764 ) ) ;
#22667=CARTESIAN_POINT ( 'NONE',  ( -4.458734124999999437, -60.56249999863440081, 0.000000000000000000 ) ) ;
#22668=CARTESIAN_POINT ( 'NONE',  ( -5.000000000000000000, -20.87499999726881228, 0.000000000000000000 ) ) ;
#22669=CARTESIAN_POINT ( 'NONE',  ( -1.339745962155610925, -18.79465819873852084, 5.000000000000000000 ) ) ;
#22670=DIRECTION ( 'NONE',  ( -0.000000000000000000, 1.000000000000000000, -0.000000000000000000 ) ) ;
#22672=LINE ( 'NONE', #12690, #12114 ) ;
#22673=CARTESIAN_POINT ( 'NONE',  ( 2.229367062500001939, -41.97916666530107932, 3.861377020970579999 ) ) ;
#22674=CARTESIAN_POINT ( 'NONE',  ( 9.457646018065525792E-16, -20.31249999863439726, 5.148502694627439702 ) ) ;
#22675=ORIENTED_EDGE ( 'NONE', *, *, #63400, .T. ) ;
#22677=CARTESIAN_POINT ( 'NONE',  ( -4.458734124999998549, -110.2291666653010651, 2.574251347313722516 ) ) ;
#22679=ORIENTED_EDGE ( 'NONE', *, *, #47661, .T. ) ;
#22680=CARTESIAN_POINT ( 'NONE',  ( 4.458734124999998549, -108.9791666653010651, -2.574251347313721627 ) ) ;
#22681=CARTESIAN_POINT ( 'NONE',  ( -4.458734124999999437, -30.39583333196773651, -2.574251347313719407 ) ) ;
#22682=CARTESIAN_POINT ( 'NONE',  ( -4.999999999999999112, -60.79166666393547303, 2.886751345948131764 ) ) ;
#22685=CARTESIAN_POINT ( 'NONE',  ( 2.229367062500001939, -30.97916666530107221, 3.861377020970579999 ) ) ;
#22686=CARTESIAN_POINT ( 'NONE',  ( 4.458734124999999437, -68.06249999863440792, -5.460374474430324690E-16 ) ) ;
#22691=CARTESIAN_POINT ( 'NONE',  ( -5.000000000000000000, -19.08333333333333570, -2.886751345948128211 ) ) ;
#22694=AXIS2_PLACEMENT_3D ( 'NONE', #62941, #14350, #33972 ) ;
#22698=CARTESIAN_POINT ( 'NONE',  ( -6.972266317189433020E-16, -87.12499999726880162, -5.000000000000000000 ) ) ;
#22704=CARTESIAN_POINT ( 'NONE',  ( 5.000000000000000000, 28.58333333333333215, -2.886751345948130876 ) ) ;
#22705=DIRECTION ( 'NONE',  ( -0.000000000000000000, 1.000000000000000000, -0.000000000000000000 ) ) ;
#22715=VERTEX_POINT ( 'NONE', #56077 ) ;
#22720=CARTESIAN_POINT ( 'NONE',  ( -6.972266317189433020E-16, -72.12499999726878741, -5.000000000000000000 ) ) ;
#22723=CARTESIAN_POINT ( 'NONE',  ( 1.975475456537005874E-15, 23.37500000273118417, 5.000000000000000000 ) ) ;
#22725=CARTESIAN_POINT ( 'NONE',  ( -4.458734124999999437, -82.31249999863440792, 0.000000000000000000 ) ) ;
#22726=CARTESIAN_POINT ( 'NONE',  ( 2.229367062500001939, 26.02083333469892779, 3.861377020970579999 ) ) ;
#22733=CYLINDRICAL_SURFACE ( 'NONE', #16115, 5.000000000000000000 ) ;
#22736=CARTESIAN_POINT ( 'NONE',  ( 4.458734124999998549, -52.72916666530107221, -2.574251347313721627 ) ) ;
#22739=CARTESIAN_POINT ( 'NONE',  ( 9.457646018065525792E-16, 20.93750000136558853, 5.148502694627439702 ) ) ;
#22740=EDGE_CURVE ( 'NONE', #32214, #10009, #51881, .T. ) ;
#22741=CARTESIAN_POINT ( 'NONE',  ( 5.000000000000000888, -104.5833333333333286, 2.886751345948126879 ) ) ;
#22743=CARTESIAN_POINT ( 'NONE',  ( 4.458734124999999437, -46.06249999863440081, -5.460374474430324690E-16 ) ) ;
#22744=CARTESIAN_POINT ( 'NONE',  ( -5.000000000000000000, -3.874999997268816720, 0.000000000000000000 ) ) ;
#22748=CARTESIAN_POINT ( 'NONE',  ( 2.229367062500001939, -102.9791666653010651, 3.861377020970579999 ) ) ;
#22749=CARTESIAN_POINT ( 'NONE',  ( 4.458734125000000326, -6.145833331967740953, 2.574251347313718519 ) ) ;
#22751=CARTESIAN_POINT ( 'NONE',  ( 1.975475456537005874E-15, -51.75000000000000711, 5.000000000000000000 ) ) ;
#22752=CARTESIAN_POINT ( 'NONE',  ( 4.458734124999999437, -95.81249999863440792, -5.460374474430324690E-16 ) ) ;
#22754=CARTESIAN_POINT ( 'NONE',  ( -2.229367062499996610, -90.39583333196773651, 3.861377020970582219 ) ) ;
#22758=EDGE_CURVE ( 'NONE', #16611, #55752, #42533, .T. ) ;
#22759=CARTESIAN_POINT ( 'NONE',  ( -2.229367062500000163, -14.47916666530107221, -3.861377020970580443 ) ) ;
#22760=CARTESIAN_POINT ( 'NONE',  ( -4.458734124999999437, 15.43750000136559386, 0.000000000000000000 ) ) ;
#22761=EDGE_CURVE ( 'NONE', #29335, #19698, #21591, .T. ) ;
#22762=CARTESIAN_POINT ( 'NONE',  ( 2.229367062500001939, -53.22916666530107221, 3.861377020970579999 ) ) ;
#22764=CARTESIAN_POINT ( 'NONE',  ( -2.500000000000000444, -69.16666666666667140, -4.330127018922193649 ) ) ;
#22771=CARTESIAN_POINT ( 'NONE',  ( 4.458734124999998549, -77.72916666530106511, -2.574251347313721627 ) ) ;
#22772=CARTESIAN_POINT ( 'NONE',  ( 2.229367062500001939, 22.77083333469892423, 3.861377020970579999 ) ) ;
#22773=EDGE_CURVE ( 'NONE', #32181, #49141, #56541, .T. ) ;
#22778=CARTESIAN_POINT ( 'NONE',  ( -5.000000000000000000, -67.99999999999998579, 0.000000000000000000 ) ) ;
#22781=ORIENTED_EDGE ( 'NONE', *, *, #58534, .F. ) ;
#22782=CARTESIAN_POINT ( 'NONE',  ( 1.339745962155612702, -18.16965819600733312, -5.000000000000000000 ) ) ;
#22784=CARTESIAN_POINT ( 'NONE',  ( 1.975475456537005874E-15, -40.74999999999999289, 5.000000000000000000 ) ) ;
#22787=VECTOR ( 'NONE', #50335, 1000.000000000000000 ) ;
#22788=CARTESIAN_POINT ( 'NONE',  ( -6.972266317189433020E-16, -107.1249999972687874, -5.000000000000000000 ) ) ;
#22790=EDGE_CURVE ( 'NONE', #11153, #37277, #6383, .T. ) ;
#22798=CARTESIAN_POINT ( 'NONE',  ( 2.229367062499998831, -49.89583333196772941, -3.861377020970580887 ) ) ;
#22800=CARTESIAN_POINT ( 'NONE',  ( -4.999999999999998224, 10.20833333606451987, 2.886751345948131764 ) ) ;
#22805=ORIENTED_EDGE ( 'NONE', *, *, #18185, .T. ) ;
#22808=CARTESIAN_POINT ( 'NONE',  ( -4.458734124999999437, -98.64583333196773651, -2.574251347313719407 ) ) ;
#22810=VERTEX_POINT ( 'NONE', #7194 ) ;
#22815=EDGE_CURVE ( 'NONE', #28751, #62202, #43729, .T. ) ;
#22816=CARTESIAN_POINT ( 'NONE',  ( 4.458734125000001214, -4.895833331967740065, 2.574251347313718519 ) ) ;
#22817=CARTESIAN_POINT ( 'NONE',  ( -4.458734124999999437, -93.56249999863440792, 0.000000000000000000 ) ) ;
#22818=EDGE_CURVE ( 'NONE', #45276, #44207, #19112, .T. ) ;
#22821=CARTESIAN_POINT ( 'NONE',  ( 4.458734124999999437, -27.06249999863440081, -5.460374474430324690E-16 ) ) ;
#22825=CARTESIAN_POINT ( 'NONE',  ( -1.339745962155613812, -91.20534180126146850, -5.000000000000000000 ) ) ;
#22828=CARTESIAN_POINT ( 'NONE',  ( -3.152548672688508926E-16, 11.18750000136559386, -5.148502694627439702 ) ) ;
#22829=ORIENTED_EDGE ( 'NONE', *, *, #33502, .F. ) ;
#22830=CARTESIAN_POINT ( 'NONE',  ( -6.972266317189433020E-16, -53.12499999726880162, -5.000000000000000000 ) ) ;
#22832=CARTESIAN_POINT ( 'NONE',  ( -4.999999999999999112, -91.91666666666667140, 2.886751345948131764 ) ) ;
#22833=CARTESIAN_POINT ( 'NONE',  ( -4.458734124999998549, -27.22916666530107221, 2.574251347313722516 ) ) ;
#22834=CARTESIAN_POINT ( 'NONE',  ( 2.499999999999998668, -73.33333333333332860, -4.330127018922193649 ) ) ;
#22835=CARTESIAN_POINT ( 'NONE',  ( -2.229367062499996610, -69.39583333196773651, 3.861377020970582219 ) ) ;
#22839=CARTESIAN_POINT ( 'NONE',  ( -2.229367062500000163, 3.520833334698929118, -3.861377020970580443 ) ) ;
#22844=CARTESIAN_POINT ( 'NONE',  ( 2.229367062500001939, -71.97916666530107932, 3.861377020970579999 ) ) ;
#22846=CARTESIAN_POINT ( 'NONE',  ( -2.499999999999996447, -3.833333333333334370, 4.330127018922195425 ) ) ;
#22849=CARTESIAN_POINT ( 'NONE',  ( 2.229367062500001939, -62.97916666530106511, 3.861377020970579999 ) ) ;
#22850=CARTESIAN_POINT ( 'NONE',  ( -4.999999999999999112, -98.79166666393547303, 2.886751345948131764 ) ) ;
#22853=CARTESIAN_POINT ( 'NONE',  ( 4.458734124999999437, -107.0624999986343937, -5.460374474430324690E-16 ) ) ;
#22855=CARTESIAN_POINT ( 'NONE',  ( -3.535250795749689387E-16, -48.25000000000000000, -5.773502691896257311 ) ) ;
#22856=CARTESIAN_POINT ( 'NONE',  ( -2.499999999999996447, -22.83333333333333215, 4.330127018922195425 ) ) ;
#22857=CARTESIAN_POINT ( 'NONE',  ( -4.330127018922205195, 45.00000000000000000, -7.499999999999943157 ) ) ;
#22860=CARTESIAN_POINT ( 'NONE',  ( 1.975475456537005874E-15, -99.62499999726880162, 5.000000000000000000 ) ) ;
#22864=CARTESIAN_POINT ( 'NONE',  ( 1.975475456537005874E-15, 12.24999999999999822, 5.000000000000000000 ) ) ;
#22869=ORIENTED_EDGE ( 'NONE', *, *, #57115, .T. ) ;
#22870=CARTESIAN_POINT ( 'NONE',  ( 2.493747252781420335E-13, -90.25000000000000000, -5.000000000000000000 ) ) ;
#22873=CARTESIAN_POINT ( 'NONE',  ( 2.229367062499998831, -35.89583333196773651, -3.861377020970580887 ) ) ;
#22882=CARTESIAN_POINT ( 'NONE',  ( 2.229367062500001939, -84.22916666530107932, 3.861377020970579999 ) ) ;
#22888=CARTESIAN_POINT ( 'NONE',  ( 4.458734125000001214, -9.145833331967736513, 2.574251347313718519 ) ) ;
#22895=CARTESIAN_POINT ( 'NONE',  ( 9.457646018065525792E-16, -5.312499998634402587, 5.148502694627439702 ) ) ;
#22901=CARTESIAN_POINT ( 'NONE',  ( -3.152548672688508926E-16, 25.18750000136558853, -5.148502694627439702 ) ) ;
#22902=EDGE_LOOP ( 'NONE', ( #36308, #3194, #12492, #63405 ) ) ;
#22903=CARTESIAN_POINT ( 'NONE',  ( 4.458734125000000326, -92.89583333196773651, 2.574251347313718519 ) ) ;
#22904=CARTESIAN_POINT ( 'NONE',  ( -6.972266317189433020E-16, -31.24999999999999645, -5.000000000000000000 ) ) ;
#22905=CARTESIAN_POINT ( 'NONE',  ( -2.229367062499996610, -7.145833331967735624, 3.861377020970582219 ) ) ;
#22909=CARTESIAN_POINT ( 'NONE',  ( 5.000000000000000888, -48.58333333333333570, 2.886751345948126879 ) ) ;
#22910=( BOUNDED_CURVE ( )  B_SPLINE_CURVE ( 2, ( #43674, #8965, #14726, #28262, #28576, #38852, #9901, #276, #9274 ),
 .UNSPECIFIED., .F., .F. ) 
 B_SPLINE_CURVE_WITH_KNOTS ( ( 3, 2, 2, 2, 3 ),
 ( 0.1446428571428571563, 0.1452380952380952495, 0.1464285714285714357, 0.1476190476190476220, 0.1482142857142857151 ),
 .UNSPECIFIED. ) 
 CURVE ( )  GEOMETRIC_REPRESENTATION_ITEM ( )  RATIONAL_B_SPLINE_CURVE ( ( 0.9330127018922194093, 0.9330127018922209636, 1.000000000000000000, 0.8660254037844387076, 1.000000000000000000, 0.8660254037844387076, 1.000000000000000000, 0.9330127018922194093, 0.9330127018922194093 ) ) 
 REPRESENTATION_ITEM ( '' )  );
#22911=CARTESIAN_POINT ( 'NONE',  ( -2.499999999999996447, 15.16666666666666607, 4.330127018922195425 ) ) ;
#22912=CARTESIAN_POINT ( 'NONE',  ( 5.000000000000000888, -34.45833333060213732, 2.886751345948126879 ) ) ;
#22913=DIRECTION ( 'NONE',  ( -0.000000000000000000, 1.000000000000000000, -0.000000000000000000 ) ) ;
#22914=CARTESIAN_POINT ( 'NONE',  ( -3.152548672688508926E-16, 18.43750000136559564, -5.148502694627439702 ) ) ;
#22915=CARTESIAN_POINT ( 'NONE',  ( 2.499999999999998668, -7.333333333333330373, -4.330127018922193649 ) ) ;
#22918=CARTESIAN_POINT ( 'NONE',  ( -4.458734124999999437, -54.39583333196773651, -2.574251347313719407 ) ) ;
#22921=CARTESIAN_POINT ( 'NONE',  ( 5.000000000000000000, 15.50000000000000000, -6.123233995736766282E-16 ) ) ;
#22925=CARTESIAN_POINT ( 'NONE',  ( 2.229367062499998831, -47.64583333196774362, -3.861377020970580887 ) ) ;
#22926=CARTESIAN_POINT ( 'NONE',  ( -2.499999999999996447, -85.70833333060214443, 4.330127018922195425 ) ) ;
#22929=CARTESIAN_POINT ( 'NONE',  ( 4.458734124999998549, -86.97916666530107932, -2.574251347313721627 ) ) ;
#22931=CARTESIAN_POINT ( 'NONE',  ( -2.500000000000000444, -35.16666666666666430, -4.330127018922193649 ) ) ;
#22936=CARTESIAN_POINT ( 'NONE',  ( -2.229367062500000163, -98.47916666530105090, -3.861377020970580443 ) ) ;
#22937=CARTESIAN_POINT ( 'NONE',  ( 4.458734124999998549, 7.020833334698929562, -2.574251347313721627 ) ) ;
#22938=CARTESIAN_POINT ( 'NONE',  ( 2.499999999999998668, 10.79166666939785202, -4.330127018922193649 ) ) ;
#22943=CARTESIAN_POINT ( 'NONE',  ( -5.000000000000000000, -81.00000000000000000, 0.000000000000000000 ) ) ;
#22948=DIRECTION ( 'NONE',  ( -0.000000000000000000, 1.000000000000000000, -0.000000000000000000 ) ) ;
#22949=CARTESIAN_POINT ( 'NONE',  ( 4.458734124999998549, -19.97916666530106866, -2.574251347313721627 ) ) ;
#22950=CARTESIAN_POINT ( 'NONE',  ( 5.000000000000000000, -107.3749999972687874, -6.123233995736766282E-16 ) ) ;
#22957=ORIENTED_EDGE ( 'NONE', *, *, #38515, .T. ) ;
#22958=FACE_OUTER_BOUND ( 'NONE', #45720, .T. ) ;
#22959=VERTEX_POINT ( 'NONE', #45709 ) ;
#22960=CARTESIAN_POINT ( 'NONE',  ( 2.229367062500001939, -68.22916666530106511, 3.861377020970579999 ) ) ;
#22961=CARTESIAN_POINT ( 'NONE',  ( -6.972266317189433020E-16, 10.87500000273118417, -5.000000000000000000 ) ) ;
#22963=( BOUNDED_CURVE ( )  B_SPLINE_CURVE ( 2, ( #38025, #47670, #27417, #38337, #37392, #2998, #22615, #3622, #13583 ),
 .UNSPECIFIED., .F., .F. ) 
 B_SPLINE_CURVE_WITH_KNOTS ( ( 3, 2, 2, 2, 3 ),
 ( 0.1446428571428571563, 0.1452380952380952495, 0.1464285714285714357, 0.1476190476190476220, 0.1482142857142857151 ),
 .UNSPECIFIED. ) 
 CURVE ( )  GEOMETRIC_REPRESENTATION_ITEM ( )  RATIONAL_B_SPLINE_CURVE ( ( 0.9330127018922194093, 0.9330127018922209636, 1.000000000000000000, 0.8660254037844387076, 1.000000000000000000, 0.8660254037844387076, 1.000000000000000000, 0.9330127018922194093, 0.9330127018922194093 ) ) 
 REPRESENTATION_ITEM ( '' )  );
#22967=ORIENTED_EDGE ( 'NONE', *, *, #26905, .T. ) ;
#22968=DIRECTION ( 'NONE',  ( -0.000000000000000000, 1.000000000000000000, -0.000000000000000000 ) ) ;
#22969=CARTESIAN_POINT ( 'NONE',  ( 9.457646018065525792E-16, 6.937500001365594748, 5.148502694627439702 ) ) ;
#22972=CARTESIAN_POINT ( 'NONE',  ( -5.000000000000000000, 6.041666669397852019, -2.886751345948128211 ) ) ;
#22973=DIRECTION ( 'NONE',  ( -0.000000000000000000, 1.000000000000000000, -0.000000000000000000 ) ) ;
#22974=ORIENTED_EDGE ( 'NONE', *, *, #38515, .F. ) ;
#22975=CARTESIAN_POINT ( 'NONE',  ( -2.229367062500000163, -72.47916666530107932, -3.861377020970580443 ) ) ;
#22976=CARTESIAN_POINT ( 'NONE',  ( 1.975475456537005874E-15, 14.37500000273118417, 5.000000000000000000 ) ) ;
#22977=CARTESIAN_POINT ( 'NONE',  ( -4.458734124999998549, 9.770833334698927786, 2.574251347313722516 ) ) ;
#22979=CARTESIAN_POINT ( 'NONE',  ( -2.229367062500000163, -58.72916666530106511, -3.861377020970580443 ) ) ;
#22980=CARTESIAN_POINT ( 'NONE',  ( -4.999999999999999112, -19.79166666393547658, 2.886751345948131764 ) ) ;
#22981=CARTESIAN_POINT ( 'NONE',  ( -4.999999999999998224, -99.91666666666665719, 2.886751345948131764 ) ) ;
#22982=CARTESIAN_POINT ( 'NONE',  ( -6.972266317189433020E-16, -45.12499999726880162, -5.000000000000000000 ) ) ;
#22984=CARTESIAN_POINT ( 'NONE',  ( 1.975475456537005874E-15, -83.62499999726878741, 5.000000000000000000 ) ) ;
#22986=CARTESIAN_POINT ( 'NONE',  ( 4.458734124999999437, -38.81249999863440081, -5.460374474430324690E-16 ) ) ;
#22988=CARTESIAN_POINT ( 'NONE',  ( -2.229367062500000163, -26.72916666530106866, -3.861377020970580443 ) ) ;
#22989=ORIENTED_EDGE ( 'NONE', *, *, #9420, .T. ) ;
#22991=CARTESIAN_POINT ( 'NONE',  ( 9.457646018065525792E-16, -107.0624999986343937, 5.148502694627439702 ) ) ;
#22994=CARTESIAN_POINT ( 'NONE',  ( -3.152548672688508926E-16, -109.8124999986343795, -5.148502694627439702 ) ) ;
#22995=CARTESIAN_POINT ( 'NONE',  ( 4.458734124999999437, -33.81249999863440792, -5.460374474430324690E-16 ) ) ;
#22996=CARTESIAN_POINT ( 'NONE',  ( 1.060575238724906964E-15, -69.62499999726880162, 5.773502691896257311 ) ) ;
#22999=EDGE_CURVE ( 'NONE', #9589, #32181, #54063, .T. ) ;
#23000=CARTESIAN_POINT ( 'NONE',  ( -2.229367062499996610, -29.14583333196774007, 3.861377020970582219 ) ) ;
#23001=CARTESIAN_POINT ( 'NONE',  ( 4.458734125000000326, -70.14583333196773651, 2.574251347313718519 ) ) ;
#23004=CARTESIAN_POINT ( 'NONE',  ( 2.500000000000002220, -32.66666666666666430, 4.330127018922192761 ) ) ;
#23005=CARTESIAN_POINT ( 'NONE',  ( 1.339745962155612702, 22.83034180399266333, -5.000000000000000000 ) ) ;
#23006=CARTESIAN_POINT ( 'NONE',  ( 2.499999999999998668, -16.33333333333333215, -4.330127018922193649 ) ) ;
#23008=ORIENTED_EDGE ( 'NONE', *, *, #9494, .T. ) ;
#23011=CARTESIAN_POINT ( 'NONE',  ( 1.060575238724906964E-15, 27.37500000273118062, 5.773502691896257311 ) ) ;
#23012=CYLINDRICAL_SURFACE ( 'NONE', #59689, 5.000000000000000000 ) ;
#23018=EDGE_LOOP ( 'NONE', ( #60784, #6892, #29659, #30931 ) ) ;
#23025=ORIENTED_EDGE ( 'NONE', *, *, #27958, .F. ) ;
#23036=CARTESIAN_POINT ( 'NONE',  ( -4.458734124999998549, -81.22916666530106511, 2.574251347313722516 ) ) ;
#23037=CARTESIAN_POINT ( 'NONE',  ( -4.458734124999998549, 26.77083333469893134, 2.574251347313722516 ) ) ;
#23040=CARTESIAN_POINT ( 'NONE',  ( 5.000000000000000888, -69.45833333060214443, 2.886751345948126879 ) ) ;
#23046=CARTESIAN_POINT ( 'NONE',  ( -4.458734124999999437, -53.39583333196773651, -2.574251347313719407 ) ) ;
#23047=CARTESIAN_POINT ( 'NONE',  ( 5.000000000000000000, 10.49999999999999822, -6.123233995736766282E-16 ) ) ;
#23048=CARTESIAN_POINT ( 'NONE',  ( 9.457646018065525792E-16, 25.93750000136559564, 5.148502694627439702 ) ) ;
#23049=CARTESIAN_POINT ( 'NONE',  ( 5.000000000000000000, -109.4166666666666572, -2.886751345948129988 ) ) ;
#23051=CARTESIAN_POINT ( 'NONE',  ( 4.458734124999998549, -42.97916666530107221, -2.574251347313721627 ) ) ;
#23052=CARTESIAN_POINT ( 'NONE',  ( 1.060575238724906964E-15, -3.624999997268816276, 5.773502691896257311 ) ) ;
#23056=CARTESIAN_POINT ( 'NONE',  ( 2.229367062500001939, -101.9791666653010651, 3.861377020970579999 ) ) ;
#23057=CARTESIAN_POINT ( 'NONE',  ( 2.229367062500001939, -3.229166665301069550, 3.861377020970579999 ) ) ;
#23060=CARTESIAN_POINT ( 'NONE',  ( 2.229367062499998831, -91.64583333196773651, -3.861377020970580887 ) ) ;
#23062=CARTESIAN_POINT ( 'NONE',  ( 4.458734124999999437, -94.06249999863440792, -5.460374474430324690E-16 ) ) ;
#23065=CARTESIAN_POINT ( 'NONE',  ( -4.458734124999997661, -14.22916666530107221, 2.574251347313722516 ) ) ;
#23066=CARTESIAN_POINT ( 'NONE',  ( 4.458734124999998549, 13.02083333469892779, -2.574251347313721627 ) ) ;
#23067=CARTESIAN_POINT ( 'NONE',  ( 4.458734125000000326, -51.14583333196772941, 2.574251347313718519 ) ) ;
#23076=CARTESIAN_POINT ( 'NONE',  ( -2.500000000000000444, -70.16666666666667140, -4.330127018922193649 ) ) ;
#23077=CARTESIAN_POINT ( 'NONE',  ( 4.458734124999998549, -81.72916666530106511, -2.574251347313721627 ) ) ;
#23078=CARTESIAN_POINT ( 'NONE',  ( 2.229367062499998831, 25.10416666803225993, -3.861377020970580887 ) ) ;
#23084=CARTESIAN_POINT ( 'NONE',  ( 2.500000000000002220, -70.66666666666667140, 4.330127018922192761 ) ) ;
#23086=ORIENTED_EDGE ( 'NONE', *, *, #909, .F. ) ;
#23088=DIRECTION ( 'NONE',  ( -0.000000000000000000, 1.000000000000000000, -0.000000000000000000 ) ) ;
#23092=ADVANCED_FACE ( 'NONE', ( #6480 ), #19982, .T. ) ;
#23093=CARTESIAN_POINT ( 'NONE',  ( 0.000000000000000000, -120.0000000000000000, 0.000000000000000000 ) ) ;
#23097=CARTESIAN_POINT ( 'NONE',  ( 2.500000000000002220, -28.66666666666666785, 4.330127018922192761 ) ) ;
#23099=VERTEX_POINT ( 'NONE', #25124 ) ;
#23102=CARTESIAN_POINT ( 'NONE',  ( -4.458734124999999437, -51.64583333196773651, -2.574251347313719407 ) ) ;
#23104=CARTESIAN_POINT ( 'NONE',  ( -6.972266317189433020E-16, -55.12499999726880873, -5.000000000000000000 ) ) ;
#23112=CARTESIAN_POINT ( 'NONE',  ( 2.229367062499998831, -99.89583333196773651, -3.861377020970580887 ) ) ;
#23113=CARTESIAN_POINT ( 'NONE',  ( -4.999999999999998224, -26.79166666393547658, 2.886751345948131764 ) ) ;
#23117=CYLINDRICAL_SURFACE ( 'NONE', #34236, 5.000000000000000000 ) ;
#23118=CARTESIAN_POINT ( 'NONE',  ( 4.458734125000001214, -5.895833331967740953, 2.574251347313718519 ) ) ;
#23119=CARTESIAN_POINT ( 'NONE',  ( 2.229367062500001939, -97.22916666530105090, 3.861377020970579999 ) ) ;
#23121=CARTESIAN_POINT ( 'NONE',  ( -2.229367062499996610, -26.39583333196774007, 3.861377020970582219 ) ) ;
#23122=CARTESIAN_POINT ( 'NONE',  ( 1.975475456537005874E-15, -74.75000000000000000, 5.000000000000000000 ) ) ;
#23126=CARTESIAN_POINT ( 'NONE',  ( -4.999999999999998224, 17.08333333333333215, 2.886751345948131764 ) ) ;
#23128=CARTESIAN_POINT ( 'NONE',  ( -4.458734124999999437, 8.354166668032261711, -2.574251347313719407 ) ) ;
#23129=ORIENTED_EDGE ( 'NONE', *, *, #27955, .F. ) ;
#23130=DIRECTION ( 'NONE',  ( -0.000000000000000000, 1.000000000000000000, -0.000000000000000000 ) ) ;
#23131=CARTESIAN_POINT ( 'NONE',  ( -2.499999999999996447, -89.83333333333332860, 4.330127018922195425 ) ) ;
#23132=CARTESIAN_POINT ( 'NONE',  ( -4.458734124999998549, -22.22916666530107221, 2.574251347313722516 ) ) ;
#23134=CARTESIAN_POINT ( 'NONE',  ( -2.229367062500000163, -78.72916666530106511, -3.861377020970580443 ) ) ;
#23138=CARTESIAN_POINT ( 'NONE',  ( 4.458734124999998549, 4.270833334698926897, -2.574251347313721627 ) ) ;
#23139=CARTESIAN_POINT ( 'NONE',  ( -3.152548672688508926E-16, 26.18750000136559564, -5.148502694627439702 ) ) ;
#23140=CARTESIAN_POINT ( 'NONE',  ( -2.229367062500000163, -38.72916666530107221, -3.861377020970580443 ) ) ;
#23141=CARTESIAN_POINT ( 'NONE',  ( -4.999999999999998224, -3.791666663935478798, 2.886751345948131764 ) ) ;
#23143=CARTESIAN_POINT ( 'NONE',  ( 2.229367062499998831, -70.64583333196773651, -3.861377020970580887 ) ) ;
#23145=CARTESIAN_POINT ( 'NONE',  ( -5.000000000000000000, -8.083333333333330373, -2.886751345948128211 ) ) ;
#23148=CARTESIAN_POINT ( 'NONE',  ( -4.458734124999999437, -65.31249999863440792, 0.000000000000000000 ) ) ;
#23149=CARTESIAN_POINT ( 'NONE',  ( -3.535250795749689387E-16, -101.1249999972688158, -5.773502691896257311 ) ) ;
#23153=CARTESIAN_POINT ( 'NONE',  ( -3.152548672688508926E-16, -108.8124999986343937, -5.148502694627439702 ) ) ;
#23155=CARTESIAN_POINT ( 'NONE',  ( -3.535250795749689387E-16, -56.25000000000000000, -5.773502691896257311 ) ) ;
#23156=CARTESIAN_POINT ( 'NONE',  ( -5.000000000000000000, 27.00000000000000000, 0.000000000000000000 ) ) ;
#23158=ORIENTED_EDGE ( 'NONE', *, *, #54678, .T. ) ;
#23159=CARTESIAN_POINT ( 'NONE',  ( 6.123233995736766282E-16, -120.0000000000000000, -5.000000000000000000 ) ) ;
#23163=EDGE_CURVE ( 'NONE', #17975, #26112, #59556, .T. ) ;
#23165=CARTESIAN_POINT ( 'NONE',  ( -6.972266317189433020E-16, -31.12499999726880873, -5.000000000000000000 ) ) ;
#23169=CARTESIAN_POINT ( 'NONE',  ( 5.000000000000000000, -81.41666666666667140, -2.886751345948130876 ) ) ;
#23174=CARTESIAN_POINT ( 'NONE',  ( 2.229367062499998831, -36.89583333196773651, -3.861377020970580887 ) ) ;
#23185=CARTESIAN_POINT ( 'NONE',  ( -3.152548672688508926E-16, -85.81249999863440792, -5.148502694627439702 ) ) ;
#23187=EDGE_LOOP ( 'NONE', ( #51600, #33626, #35064, #61017 ) ) ;
#23189=CARTESIAN_POINT ( 'NONE',  ( -6.972266317189433020E-16, -43.25000000000000000, -5.000000000000000000 ) ) ;
#23193=CARTESIAN_POINT ( 'NONE',  ( -4.999999999999998224, -1.916666666666663854, 2.886751345948131764 ) ) ;
#23194=CARTESIAN_POINT ( 'NONE',  ( 4.458734124999999437, -11.06249999863440792, -5.460374474430324690E-16 ) ) ;
#23197=CARTESIAN_POINT ( 'NONE',  ( 2.499999999999998668, -77.20833333060214443, -4.330127018922193649 ) ) ;
#23199=CARTESIAN_POINT ( 'NONE',  ( -4.458734124999997661, 24.52083333469892779, 2.574251347313722516 ) ) ;
#23201=CARTESIAN_POINT ( 'NONE',  ( 9.457646018065525792E-16, -93.06249999863440792, 5.148502694627439702 ) ) ;
#23202=CARTESIAN_POINT ( 'NONE',  ( -4.999999999999998224, -30.91666666666667140, 2.886751345948131764 ) ) ;
#23204=CARTESIAN_POINT ( 'NONE',  ( 9.457646018065525792E-16, -7.062499998634404363, 5.148502694627439702 ) ) ;
#23209=CARTESIAN_POINT ( 'NONE',  ( 2.500000000000002220, -36.54166666393547303, 4.330127018922192761 ) ) ;
#23211=CARTESIAN_POINT ( 'NONE',  ( -4.458734124999999437, 18.60416666803225993, -2.574251347313719407 ) ) ;
#23213=EDGE_CURVE ( 'NONE', #4881, #23583, #34333, .T. ) ;
#23215=CARTESIAN_POINT ( 'NONE',  ( 2.229367062500001939, -57.97916666530107932, 3.861377020970579999 ) ) ;
#23217=CARTESIAN_POINT ( 'NONE',  ( 1.975475456537005874E-15, -105.6249999972688016, 5.000000000000000000 ) ) ;
#23218=CARTESIAN_POINT ( 'NONE',  ( 5.000000000000000000, 7.500000000000000000, -6.123233995736766282E-16 ) ) ;
#23221=CARTESIAN_POINT ( 'NONE',  ( -2.229367062500000163, -48.47916666530106511, -3.861377020970580443 ) ) ;
#23222=CARTESIAN_POINT ( 'NONE',  ( 2.499999999999998668, -86.20833333060214443, -4.330127018922193649 ) ) ;
#23224=CARTESIAN_POINT ( 'NONE',  ( -1.230605004983934782E-13, -37.62499999726881583, 5.000000000000000000 ) ) ;
#23226=CARTESIAN_POINT ( 'NONE',  ( -2.229367062499996610, -90.39583333196773651, 3.861377020970582219 ) ) ;
#23228=CARTESIAN_POINT ( 'NONE',  ( -5.000000000000000000, -37.99999999999999289, 0.000000000000000000 ) ) ;
#23230=VERTEX_POINT ( 'NONE', #16116 ) ;
#23233=CARTESIAN_POINT ( 'NONE',  ( -4.458734124999999437, -96.31249999863440792, 0.000000000000000000 ) ) ;
#23234=CARTESIAN_POINT ( 'NONE',  ( 4.458734124999999437, 9.937500001365593860, -5.460374474430324690E-16 ) ) ;
#23235=CARTESIAN_POINT ( 'NONE',  ( 5.000000000000000000, 9.708333336064519870, -2.886751345948129988 ) ) ;
#23241=CARTESIAN_POINT ( 'NONE',  ( 5.000000000000000000, -61.37499999726880873, -6.123233995736766282E-16 ) ) ;
#23243=EDGE_CURVE ( 'NONE', #56096, #44174, #47863, .T. ) ;
#23245=CYLINDRICAL_SURFACE ( 'NONE', #20427, 5.000000000000000000 ) ;
#23248=CARTESIAN_POINT ( 'NONE',  ( 0.000000000000000000, -120.0000000000000000, 0.000000000000000000 ) ) ;
#23250=LINE ( 'NONE', #58831, #18135 ) ;
#23252=CARTESIAN_POINT ( 'NONE',  ( -4.458734124999999437, -18.64583333196774007, -2.574251347313719407 ) ) ;
#23259=EDGE_CURVE ( 'NONE', #63455, #58748, #30896, .T. ) ;
#23267=CARTESIAN_POINT ( 'NONE',  ( -4.458734124999999437, -65.56249999863440792, 0.000000000000000000 ) ) ;
#23269=LINE ( 'NONE', #38057, #39968 ) ;
#23270=VERTEX_POINT ( 'NONE', #56643 ) ;
#23271=EDGE_CURVE ( 'NONE', #454, #24668, #17077, .T. ) ;
#23274=CARTESIAN_POINT ( 'NONE',  ( 2.229367062499998831, 1.104166668032261711, -3.861377020970580887 ) ) ;
#23277=DIRECTION ( 'NONE',  ( -0.000000000000000000, 1.000000000000000000, -0.000000000000000000 ) ) ;
#23278=CARTESIAN_POINT ( 'NONE',  ( 9.457646018065525792E-16, 4.937500001365596525, 5.148502694627439702 ) ) ;
#23283=VECTOR ( 'NONE', #13240, 1000.000000000000000 ) ;
#23285=CARTESIAN_POINT ( 'NONE',  ( -3.152548672688508926E-16, -73.56249999863439371, -5.148502694627439702 ) ) ;
#23287=CARTESIAN_POINT ( 'NONE',  ( -4.458734124999999437, 4.687500001365595637, 0.000000000000000000 ) ) ;
#23291=CARTESIAN_POINT ( 'NONE',  ( -4.458734124999999437, -60.64583333196774362, -2.574251347313719407 ) ) ;
#23292=CARTESIAN_POINT ( 'NONE',  ( 2.500000000000002220, -18.54166666393547658, 4.330127018922192761 ) ) ;
#23294=CARTESIAN_POINT ( 'NONE',  ( 5.000000000000000888, -42.45833333060214443, 2.886751345948126879 ) ) ;
#23298=CARTESIAN_POINT ( 'NONE',  ( 4.458734125000001214, -38.89583333196773651, 2.574251347313718519 ) ) ;
#23299=CARTESIAN_POINT ( 'NONE',  ( 4.458734124999999437, -25.06249999863440792, -5.460374474430324690E-16 ) ) ;
#23301=CARTESIAN_POINT ( 'NONE',  ( -4.999999999999999112, 28.08333333333333570, 2.886751345948131764 ) ) ;
#23303=VERTEX_POINT ( 'NONE', #17074 ) ;
#23304=CARTESIAN_POINT ( 'NONE',  ( -4.458734124999999437, -110.5624999986343937, 0.000000000000000000 ) ) ;
#23305=CARTESIAN_POINT ( 'NONE',  ( -2.229367062499996610, -33.14583333196772941, 3.861377020970582219 ) ) ;
#23306=CARTESIAN_POINT ( 'NONE',  ( 5.000000000000000000, -70.37499999726880162, -6.123233995736766282E-16 ) ) ;
#23309=ADVANCED_BREP_SHAPE_REPRESENTATION ( '', ( #50626, #43054 ), #29681 ) ;
#23310=CARTESIAN_POINT ( 'NONE',  ( 4.458734125000000326, -27.89583333196774007, 2.574251347313718519 ) ) ;
#23311=CARTESIAN_POINT ( 'NONE',  ( -3.152548672688508926E-16, -74.81249999863439371, -5.148502694627439702 ) ) ;
#23312=CARTESIAN_POINT ( 'NONE',  ( 1.464175926609780648E-14, 22.74999999999999645, -5.000000000000000000 ) ) ;
#23316=CARTESIAN_POINT ( 'NONE',  ( 2.500000000000002220, -5.541666663935480130, 4.330127018922192761 ) ) ;
#23317=CARTESIAN_POINT ( 'NONE',  ( 2.499999999999998668, -19.33333333333333570, -4.330127018922193649 ) ) ;
#23322=CARTESIAN_POINT ( 'NONE',  ( -4.999999999999999112, 25.20833333606451987, 2.886751345948131764 ) ) ;
#23323=CARTESIAN_POINT ( 'NONE',  ( 1.975475456537005874E-15, -110.6249999972688158, 5.000000000000000000 ) ) ;
#23325=CYLINDRICAL_SURFACE ( 'NONE', #35588, 5.000000000000000000 ) ;
#23327=CARTESIAN_POINT ( 'NONE',  ( -1.339745962155613812, -52.08034179853028434, -5.000000000000000000 ) ) ;
#23329=CARTESIAN_POINT ( 'NONE',  ( -1.339745962155610925, -80.66965819600734733, 5.000000000000000000 ) ) ;
#23331=CARTESIAN_POINT ( 'NONE',  ( 2.499999999999998668, -12.33333333333333570, -4.330127018922193649 ) ) ;
#23332=ORIENTED_EDGE ( 'NONE', *, *, #30448, .T. ) ;
#23333=( BOUNDED_CURVE ( )  B_SPLINE_CURVE ( 2, ( #42858, #44028, #49186, #63358, #20239, #45168, #19595, #4802, #19274 ),
 .UNSPECIFIED., .F., .F. ) 
 B_SPLINE_CURVE_WITH_KNOTS ( ( 3, 2, 2, 2, 3 ),
 ( 0.1732142857142857095, 0.1738095238095238027, 0.1749999999999999889, 0.1761904761904762029, 0.1767857142857142960 ),
 .UNSPECIFIED. ) 
 CURVE ( )  GEOMETRIC_REPRESENTATION_ITEM ( )  RATIONAL_B_SPLINE_CURVE ( ( 0.9330127018922194093, 0.9330127018922194093, 1.000000000000000000, 0.8660254037844387076, 1.000000000000000000, 0.8660254037844387076, 1.000000000000000000, 0.9330127018922194093, 0.9330127018922194093 ) ) 
 REPRESENTATION_ITEM ( '' )  );
#23339=AXIS2_PLACEMENT_3D ( 'NONE', #61119, #23130, #2898 ) ;
#23344=ORIENTED_EDGE ( 'NONE', *, *, #50061, .F. ) ;
#23345=CARTESIAN_POINT ( 'NONE',  ( 1.339745962155615144, -34.70534180126148271, 4.999999999999999112 ) ) ;
#23346=CARTESIAN_POINT ( 'NONE',  ( 1.975475456537005874E-15, -53.74999999999999289, 5.000000000000000000 ) ) ;
#23353=EDGE_LOOP ( 'NONE', ( #8474, #24793, #36540, #48080 ) ) ;
#23354=ADVANCED_FACE ( 'NONE', ( #61780 ), #41499, .T. ) ;
#23355=CARTESIAN_POINT ( 'NONE',  ( 2.229367062499998831, -81.64583333196773651, -3.861377020970580887 ) ) ;
#23356=CARTESIAN_POINT ( 'NONE',  ( -4.458734124999999437, 20.60416666803225993, -2.574251347313719407 ) ) ;
#23358=ORIENTED_EDGE ( 'NONE', *, *, #10968, .T. ) ;
#23366=CARTESIAN_POINT ( 'NONE',  ( -2.229367062499996610, -58.14583333196773651, 3.861377020970582219 ) ) ;
#23368=CARTESIAN_POINT ( 'NONE',  ( -4.458734124999999437, 25.60416666803225993, -2.574251347313719407 ) ) ;
#23371=CARTESIAN_POINT ( 'NONE',  ( 4.458734124999999437, -43.06249999863440081, -5.460374474430324690E-16 ) ) ;
#23372=CARTESIAN_POINT ( 'NONE',  ( -5.000000000000000000, -3.958333330602147537, -2.886751345948128211 ) ) ;
#23373=CARTESIAN_POINT ( 'NONE',  ( 1.975475456537005874E-15, -31.75000000000000000, 5.000000000000000000 ) ) ;
#23376=CARTESIAN_POINT ( 'NONE',  ( 2.229367062500001939, -104.9791666653010651, 3.861377020970579999 ) ) ;
#23377=CARTESIAN_POINT ( 'NONE',  ( -2.229367062500000163, -10.72916666530106866, -3.861377020970580443 ) ) ;
#23379=AXIS2_PLACEMENT_3D ( 'NONE', #10224, #58482, #39799 ) ;
#23380=CARTESIAN_POINT ( 'NONE',  ( -6.972266317189433020E-16, -52.25000000000000711, -5.000000000000000000 ) ) ;
#23381=CARTESIAN_POINT ( 'NONE',  ( 2.229367062500001939, -92.97916666530106511, 3.861377020970579999 ) ) ;
#23383=CARTESIAN_POINT ( 'NONE',  ( 2.229367062500001939, -90.22916666530106511, 3.861377020970579999 ) ) ;
#23384=VECTOR ( 'NONE', #41246, 1000.000000000000000 ) ;
#23385=CARTESIAN_POINT ( 'NONE',  ( -2.500000000000000444, -51.04166666393547303, -4.330127018922193649 ) ) ;
#23388=CARTESIAN_POINT ( 'NONE',  ( 4.458734124999999437, -11.81249999863440081, -5.460374474430324690E-16 ) ) ;
#23389=CARTESIAN_POINT ( 'NONE',  ( 9.457646018065525792E-16, 11.68750000136559564, 5.148502694627439702 ) ) ;
#23390=CARTESIAN_POINT ( 'NONE',  ( 4.458734124999999437, -53.06249999863440792, -5.460374474430324690E-16 ) ) ;
#23391=DIRECTION ( 'NONE',  ( 0.000000000000000000, 0.000000000000000000, 1.000000000000000000 ) ) ;
#23394=CARTESIAN_POINT ( 'NONE',  ( 5.000000000000000000, -8.291666663935481907, -2.886751345948130876 ) ) ;
#23398=CARTESIAN_POINT ( 'NONE',  ( 1.339745962155612702, -68.29465819873851729, -5.000000000000000000 ) ) ;
#23399=CARTESIAN_POINT ( 'NONE',  ( -2.500000000000000444, -67.04166666393547303, -4.330127018922193649 ) ) ;
#23400=CARTESIAN_POINT ( 'NONE',  ( -4.458734124999998549, -86.22916666530106511, 2.574251347313722516 ) ) ;
#23401=CARTESIAN_POINT ( 'NONE',  ( -4.458734124999998549, 23.52083333469892779, 2.574251347313722516 ) ) ;
#23404=DIRECTION ( 'NONE',  ( -0.000000000000000000, 1.000000000000000000, -0.000000000000000000 ) ) ;
#23405=FACE_OUTER_BOUND ( 'NONE', #50963, .T. ) ;
#23407=CARTESIAN_POINT ( 'NONE',  ( -5.000000000000000000, -71.00000000000000000, 0.000000000000000000 ) ) ;
#23410=CARTESIAN_POINT ( 'NONE',  ( 5.000000000000000888, -18.45833333060214798, 2.886751345948126879 ) ) ;
#23411=CARTESIAN_POINT ( 'NONE',  ( -5.000000000000000000, -79.95833333060213022, -2.886751345948128211 ) ) ;
#23415=CARTESIAN_POINT ( 'NONE',  ( 3.044556291839386294E-14, 18.75000000000000355, -5.000000000000000000 ) ) ;
#23424=CARTESIAN_POINT ( 'NONE',  ( -2.229367062500000163, -57.72916666530107932, -3.861377020970580443 ) ) ;
#23436=CARTESIAN_POINT ( 'NONE',  ( 9.457646018065525792E-16, -97.31249999863440792, 5.148502694627439702 ) ) ;
#23441=CARTESIAN_POINT ( 'NONE',  ( 2.499999999999998668, -83.33333333333332860, -4.330127018922193649 ) ) ;
#23442=CARTESIAN_POINT ( 'NONE',  ( 2.229367062500001939, -9.979166665301068662, 3.861377020970579999 ) ) ;
#23443=CARTESIAN_POINT ( 'NONE',  ( -4.458734124999997661, -100.4791666653010651, 2.574251347313722516 ) ) ;
#23445=CARTESIAN_POINT ( 'NONE',  ( -2.229367062500000163, -25.72916666530106866, -3.861377020970580443 ) ) ;
#23448=CARTESIAN_POINT ( 'NONE',  ( 0.000000000000000000, -120.0000000000000000, 5.000000000000000000 ) ) ;
#23450=CARTESIAN_POINT ( 'NONE',  ( -2.229367062499996610, 7.604166668032260823, 3.861377020970582219 ) ) ;
#23451=EDGE_LOOP ( 'NONE', ( #26323, #59894, #39840, #6092 ) ) ;
#23454=CARTESIAN_POINT ( 'NONE',  ( -2.499999999999996447, -91.83333333333334281, 4.330127018922195425 ) ) ;
#23455=CARTESIAN_POINT ( 'NONE',  ( 2.229367062499998831, -25.64583333196773651, -3.861377020970580887 ) ) ;
#23456=CARTESIAN_POINT ( 'NONE',  ( -6.972266317189433020E-16, 6.875000002731185944, -5.000000000000000000 ) ) ;
#23457=CARTESIAN_POINT ( 'NONE',  ( -2.229367062499996610, -76.39583333196773651, 3.861377020970582219 ) ) ;
#23458=EDGE_CURVE ( 'NONE', #7844, #43959, #63350, .T. ) ;
#23460=LINE ( 'NONE', #57251, #47883 ) ;
#23461=( BOUNDED_CURVE ( )  B_SPLINE_CURVE ( 2, ( #13215, #38587, #23814, #37658, #53081, #57299, #32838, #13839, #4201 ),
 .UNSPECIFIED., .F., .F. ) 
 B_SPLINE_CURVE_WITH_KNOTS ( ( 3, 2, 2, 2, 3 ),
 ( 0.4017857142857143016, 0.4023809523809523947, 0.4035714285714285809, 0.4047619047619047672, 0.4053571428571428603 ),
 .UNSPECIFIED. ) 
 CURVE ( )  GEOMETRIC_REPRESENTATION_ITEM ( )  RATIONAL_B_SPLINE_CURVE ( ( 0.9330127018922194093, 0.9330127018922194093, 1.000000000000000000, 0.8660254037844387076, 1.000000000000000000, 0.8660254037844387076, 1.000000000000000000, 0.9330127018922194093, 0.9330127018922194093 ) ) 
 REPRESENTATION_ITEM ( '' )  );
#23463=CARTESIAN_POINT ( 'NONE',  ( 4.458734124999999437, 3.187500001365594304, -5.460374474430324690E-16 ) ) ;
#23464=CARTESIAN_POINT ( 'NONE',  ( -4.458734124999998549, 27.52083333469892779, 2.574251347313722516 ) ) ;
#23465=CARTESIAN_POINT ( 'NONE',  ( 4.458734124999998549, -39.97916666530107221, -2.574251347313721627 ) ) ;
#23466=CARTESIAN_POINT ( 'NONE',  ( 0.000000000000000000, -120.0000000000000000, 0.000000000000000000 ) ) ;
#23470=CARTESIAN_POINT ( 'NONE',  ( 2.229367062499998831, -68.64583333196773651, -3.861377020970580887 ) ) ;
#23471=CARTESIAN_POINT ( 'NONE',  ( -2.499999999999996447, -99.70833333060214443, 4.330127018922195425 ) ) ;
#23474=CARTESIAN_POINT ( 'NONE',  ( 5.000000000000000000, 9.708333336064519870, -2.886751345948130876 ) ) ;
#23475=CARTESIAN_POINT ( 'NONE',  ( -2.229367062499996610, -104.3958333319677365, 3.861377020970582219 ) ) ;
#23477=CARTESIAN_POINT ( 'NONE',  ( -4.999999999999999112, -55.91666666666667140, 2.886751345948131764 ) ) ;
#23486=AXIS2_PLACEMENT_3D ( 'NONE', #22029, #41621, #4925 ) ;
#23497=CARTESIAN_POINT ( 'NONE',  ( -4.458734124999998549, -35.47916666530107221, 2.574251347313722516 ) ) ;
#23498=CYLINDRICAL_SURFACE ( 'NONE', #58397, 5.000000000000000000 ) ;
#23506=CARTESIAN_POINT ( 'NONE',  ( -4.458734124999998549, -81.47916666530106511, 2.574251347313722516 ) ) ;
#23508=ORIENTED_EDGE ( 'NONE', *, *, #49168, .T. ) ;
#23512=CARTESIAN_POINT ( 'NONE',  ( -6.972266317189433020E-16, -105.2500000000000000, -5.000000000000000000 ) ) ;
#23516=ORIENTED_EDGE ( 'NONE', *, *, #4795, .T. ) ;
#23517=CARTESIAN_POINT ( 'NONE',  ( 5.000000000000000000, -78.50000000000000000, -6.123233995736766282E-16 ) ) ;
#23518=CARTESIAN_POINT ( 'NONE',  ( -4.458734124999999437, -11.64583333196773829, -2.574251347313719407 ) ) ;
#23520=CARTESIAN_POINT ( 'NONE',  ( 5.000000000000000000, -77.37499999726881583, -6.123233995736766282E-16 ) ) ;
#23522=CARTESIAN_POINT ( 'NONE',  ( 4.458734124999998549, 25.02083333469892779, -2.574251347313721627 ) ) ;
#23523=VERTEX_POINT ( 'NONE', #4178 ) ;
#23524=CARTESIAN_POINT ( 'NONE',  ( -4.458734124999999437, -93.31249999863440792, 0.000000000000000000 ) ) ;
#23527=CARTESIAN_POINT ( 'NONE',  ( 4.458734124999998549, -7.729166665301073103, -2.574251347313721627 ) ) ;
#23531=CARTESIAN_POINT ( 'NONE',  ( -2.499999999999996447, -87.83333333333332860, 4.330127018922195425 ) ) ;
#23532=CARTESIAN_POINT ( 'NONE',  ( -5.000000000000000000, -36.87499999726881583, 0.000000000000000000 ) ) ;
#23534=CARTESIAN_POINT ( 'NONE',  ( 4.458734124999998549, 19.27083333469893134, -2.574251347313721627 ) ) ;
#23535=CARTESIAN_POINT ( 'NONE',  ( 5.000000000000000000, -51.37499999726881583, -6.123233995736766282E-16 ) ) ;
#23536=( BOUNDED_CURVE ( )  B_SPLINE_CURVE ( 2, ( #11983, #7181, #26789, #57020, #46408, #51556, #41560, #2357, #57339 ),
 .UNSPECIFIED., .F., .F. ) 
 B_SPLINE_CURVE_WITH_KNOTS ( ( 3, 2, 2, 2, 3 ),
 ( 0.6732142857142857650, 0.6738095238095238582, 0.6750000000000000444, 0.6761904761904762307, 0.6767857142857143238 ),
 .UNSPECIFIED. ) 
 CURVE ( )  GEOMETRIC_REPRESENTATION_ITEM ( )  RATIONAL_B_SPLINE_CURVE ( ( 0.9330127018922194093, 0.9330127018922194093, 1.000000000000000000, 0.8660254037844387076, 1.000000000000000000, 0.8660254037844387076, 1.000000000000000000, 0.9330127018922194093, 0.9330127018922194093 ) ) 
 REPRESENTATION_ITEM ( '' )  );
#23538=CARTESIAN_POINT ( 'NONE',  ( -2.229367062499996610, -58.14583333196773651, 3.861377020970582219 ) ) ;
#23541=CARTESIAN_POINT ( 'NONE',  ( 2.499999999999998668, 7.666666666666665186, -4.330127018922193649 ) ) ;
#23544=CARTESIAN_POINT ( 'NONE',  ( 4.458734124999998549, -46.72916666530106511, -2.574251347313721627 ) ) ;
#23545=CARTESIAN_POINT ( 'NONE',  ( 1.060575238724906964E-15, -82.62499999726880162, 5.773502691896257311 ) ) ;
#23547=CYLINDRICAL_SURFACE ( 'NONE', #20579, 5.000000000000000000 ) ;
#23550=EDGE_CURVE ( 'NONE', #19195, #24536, #37186, .T. ) ;
#23551=CARTESIAN_POINT ( 'NONE',  ( -4.458734124999999437, -89.64583333196773651, -2.574251347313719407 ) ) ;
#23553=CARTESIAN_POINT ( 'NONE',  ( 5.000000000000000888, -37.58333333333332860, 2.886751345948126879 ) ) ;
#23554=CARTESIAN_POINT ( 'NONE',  ( -6.972266317189433020E-16, 23.75000000000000000, -5.000000000000000000 ) ) ;
#23555=EDGE_LOOP ( 'NONE', ( #38226, #55398, #20729, #53644 ) ) ;
#23557=ORIENTED_EDGE ( 'NONE', *, *, #20005, .F. ) ;
#23558=CARTESIAN_POINT ( 'NONE',  ( -3.152548672688508926E-16, -95.56249999863442213, -5.148502694627439702 ) ) ;
#23559=CARTESIAN_POINT ( 'NONE',  ( 2.229367062500001939, 5.770833334698927786, 3.861377020970579999 ) ) ;
#23560=COLOUR_RGB ( '',0.8941176470588234615, 0.8941176470588234615, 0.8941176470588234615 ) ;
#23561=CARTESIAN_POINT ( 'NONE',  ( 2.500000000000002220, 9.458333336064519870, 4.330127018922192761 ) ) ;
#23565=VECTOR ( 'NONE', #55285, 1000.000000000000000 ) ;
#23576=CARTESIAN_POINT ( 'NONE',  ( -4.458734124999999437, -20.56249999863440081, 0.000000000000000000 ) ) ;
#23583=VERTEX_POINT ( 'NONE', #62724 ) ;
#23584=EDGE_CURVE ( 'NONE', #53594, #46354, #63105, .T. ) ;
#23585=CARTESIAN_POINT ( 'NONE',  ( 0.000000000000000000, -120.0000000000000000, 0.000000000000000000 ) ) ;
#23587=CARTESIAN_POINT ( 'NONE',  ( 9.457646018065525792E-16, -70.31249999863439371, 5.148502694627439702 ) ) ;
#23588=DIRECTION ( 'NONE',  ( -0.000000000000000000, 1.000000000000000000, -0.000000000000000000 ) ) ;
#23589=CARTESIAN_POINT ( 'NONE',  ( -2.500000000000000444, -6.041666663935481019, -4.330127018922193649 ) ) ;
#23593=CARTESIAN_POINT ( 'NONE',  ( 4.458734124999999437, 2.937500001365594304, -5.460374474430324690E-16 ) ) ;
#23595=CARTESIAN_POINT ( 'NONE',  ( -2.499999999999996447, -54.83333333333332860, 4.330127018922195425 ) ) ;
#23600=ORIENTED_EDGE ( 'NONE', *, *, #37869, .T. ) ;
#23601=CARTESIAN_POINT ( 'NONE',  ( 9.457646018065525792E-16, -74.06249999863440792, 5.148502694627439702 ) ) ;
#23603=CARTESIAN_POINT ( 'NONE',  ( -4.458734124999999437, 8.604166668032261711, -2.574251347313719407 ) ) ;
#23608=EDGE_CURVE ( 'NONE', #53065, #20011, #41294, .T. ) ;
#23609=CARTESIAN_POINT ( 'NONE',  ( -4.458734124999999437, -59.64583333196773651, -2.574251347313719407 ) ) ;
#23610=CARTESIAN_POINT ( 'NONE',  ( 5.000000000000000888, -18.45833333060214798, 2.886751345948126879 ) ) ;
#23611=CARTESIAN_POINT ( 'NONE',  ( 1.975475456537005874E-15, -40.74999999999999289, 5.000000000000000000 ) ) ;
#23615=CARTESIAN_POINT ( 'NONE',  ( -3.152548672688508926E-16, -39.56249999863440081, -5.148502694627439702 ) ) ;
#23616=CARTESIAN_POINT ( 'NONE',  ( 2.229367062499998831, -25.89583333196773651, -3.861377020970580887 ) ) ;
#23618=CARTESIAN_POINT ( 'NONE',  ( -4.999999999999999112, 24.08333333333333215, 2.886751345948131764 ) ) ;
#23621=CARTESIAN_POINT ( 'NONE',  ( 9.457646018065525792E-16, -110.3124999986343937, 5.148502694627439702 ) ) ;
#23622=CARTESIAN_POINT ( 'NONE',  ( -4.458734124999999437, -30.31249999863440436, 0.000000000000000000 ) ) ;
#23623=CARTESIAN_POINT ( 'NONE',  ( -3.535250795749689387E-16, -69.12499999726880162, -5.773502691896257311 ) ) ;
#23628=CARTESIAN_POINT ( 'NONE',  ( -4.458734124999999437, -72.64583333196773651, -2.574251347313719407 ) ) ;
#23633=CARTESIAN_POINT ( 'NONE',  ( 2.500000000000002220, -19.66666666666666430, 4.330127018922192761 ) ) ;
#23636=CARTESIAN_POINT ( 'NONE',  ( -1.339745962155613812, -79.08034179853028434, -5.000000000000000000 ) ) ;
#23638=CARTESIAN_POINT ( 'NONE',  ( 5.000000000000000000, 24.70833333606451987, -2.886751345948129988 ) ) ;
#23639=CARTESIAN_POINT ( 'NONE',  ( 5.000000000000000000, 4.708333336064518093, -2.886751345948130876 ) ) ;
#23643=CARTESIAN_POINT ( 'NONE',  ( 5.000000000000000000, 28.49999999999999645, -6.123233995736766282E-16 ) ) ;
#23644=CARTESIAN_POINT ( 'NONE',  ( -1.339745962155610925, -40.66965819600732601, 5.000000000000000000 ) ) ;
#23647=VERTEX_POINT ( 'NONE', #622 ) ;
#23651=VECTOR ( 'NONE', #23404, 1000.000000000000000 ) ;
#23657=CARTESIAN_POINT ( 'NONE',  ( 1.975475456537005874E-15, -69.62499999726880162, 5.000000000000000000 ) ) ;
#23662=CARTESIAN_POINT ( 'NONE',  ( 0.000000000000000000, -120.0000000000000000, 0.000000000000000000 ) ) ;
#23664=AXIS2_PLACEMENT_3D ( 'NONE', #20, #34402, #43741 ) ;
#23666=CARTESIAN_POINT ( 'NONE',  ( -4.458734124999999437, -81.31249999863440792, 0.000000000000000000 ) ) ;
#23667=CARTESIAN_POINT ( 'NONE',  ( 4.458734125000001214, 17.10416666803225993, 2.574251347313718519 ) ) ;
#23673=CARTESIAN_POINT ( 'NONE',  ( 1.975475456537005874E-15, 11.37500000273118239, 5.000000000000000000 ) ) ;
#23675=CARTESIAN_POINT ( 'NONE',  ( 5.000000000000000000, 4.500000000000000888, -6.123233995736766282E-16 ) ) ;
#23676=CARTESIAN_POINT ( 'NONE',  ( 9.457646018065525792E-16, -62.06249999863440792, 5.148502694627439702 ) ) ;
#23678=CARTESIAN_POINT ( 'NONE',  ( -4.458734124999999437, 24.68750000136559208, 0.000000000000000000 ) ) ;
#23679=CARTESIAN_POINT ( 'NONE',  ( 1.060575238724906964E-15, -109.7499999999999858, 5.773502691896257311 ) ) ;
#23682=CARTESIAN_POINT ( 'NONE',  ( 4.458734124999998549, -44.97916666530107221, -2.574251347313721627 ) ) ;
#23683=CARTESIAN_POINT ( 'NONE',  ( 5.000000000000000000, -6.374999997268812280, -6.123233995736766282E-16 ) ) ;
#23684=CARTESIAN_POINT ( 'NONE',  ( -6.972266317189433020E-16, -93.24999999999998579, -5.000000000000000000 ) ) ;
#23687=CARTESIAN_POINT ( 'NONE',  ( -4.458734124999999437, -110.3124999986343937, 0.000000000000000000 ) ) ;
#23688=CARTESIAN_POINT ( 'NONE',  ( -4.458734124999997661, -12.47916666530107044, 2.574251347313722516 ) ) ;
#23690=VERTEX_POINT ( 'NONE', #16365 ) ;
#23691=CARTESIAN_POINT ( 'NONE',  ( 2.500000000000002220, -52.66666666666666430, 4.330127018922192761 ) ) ;
#23692=CARTESIAN_POINT ( 'NONE',  ( 4.458734125000001214, -95.89583333196773651, 2.574251347313718519 ) ) ;
#23694=CARTESIAN_POINT ( 'NONE',  ( 2.229367062499998831, -91.89583333196773651, -3.861377020970580887 ) ) ;
#23696=CARTESIAN_POINT ( 'NONE',  ( -4.999999999999999112, -52.79166666393547303, 2.886751345948131764 ) ) ;
#23702=CARTESIAN_POINT ( 'NONE',  ( -4.458734124999999437, -13.31249999863440259, 0.000000000000000000 ) ) ;
#23703=CARTESIAN_POINT ( 'NONE',  ( 4.458734124999999437, 8.937500001365592084, -5.460374474430324690E-16 ) ) ;
#23704=CARTESIAN_POINT ( 'NONE',  ( 2.229367062499998831, -59.89583333196774362, -3.861377020970580887 ) ) ;
#23705=CARTESIAN_POINT ( 'NONE',  ( -6.972266317189433020E-16, -14.12499999726881228, -5.000000000000000000 ) ) ;
#23706=CARTESIAN_POINT ( 'NONE',  ( 2.500000000000002220, -15.54166666393548191, 4.330127018922192761 ) ) ;
#23709=EDGE_CURVE ( 'NONE', #26645, #8886, #56911, .T. ) ;
#23710=ORIENTED_EDGE ( 'NONE', *, *, #46042, .T. ) ;
#23713=EDGE_CURVE ( 'NONE', #43496, #32964, #36420, .T. ) ;
#23714=CARTESIAN_POINT ( 'NONE',  ( 1.975475456537005874E-15, -24.74999999999999645, 5.000000000000000000 ) ) ;
#23715=CARTESIAN_POINT ( 'NONE',  ( -4.458734124999999437, -87.39583333196773651, -2.574251347313719407 ) ) ;
#23716=CARTESIAN_POINT ( 'NONE',  ( -4.458734124999998549, 18.52083333469892779, 2.574251347313722516 ) ) ;
#23722=CARTESIAN_POINT ( 'NONE',  ( -2.499999999999996447, -70.83333333333332860, 4.330127018922195425 ) ) ;
#23724=ORIENTED_EDGE ( 'NONE', *, *, #11031, .F. ) ;
#23725=CARTESIAN_POINT ( 'NONE',  ( 1.339745962155615144, -79.70534180126146850, 4.999999999999999112 ) ) ;
#23727=CARTESIAN_POINT ( 'NONE',  ( -5.000000000000000000, -104.0000000000000142, 0.000000000000000000 ) ) ;
#23732=EDGE_LOOP ( 'NONE', ( #41182, #11384, #25555, #22020 ) ) ;
#23738=CARTESIAN_POINT ( 'NONE',  ( 4.458734124999999437, -58.06249999863440081, -5.460374474430324690E-16 ) ) ;
#23751=CARTESIAN_POINT ( 'NONE',  ( 4.458734125000001214, -106.1458333319677365, 2.574251347313718519 ) ) ;
#23755=CARTESIAN_POINT ( 'NONE',  ( -4.458734124999997661, -39.22916666530107221, 2.574251347313722516 ) ) ;
#23757=CARTESIAN_POINT ( 'NONE',  ( 4.458734124999998549, -14.72916666530107399, -2.574251347313721627 ) ) ;
#23758=CARTESIAN_POINT ( 'NONE',  ( -3.152548672688508926E-16, -99.81249999863440792, -5.148502694627439702 ) ) ;
#23760=CARTESIAN_POINT ( 'NONE',  ( -2.229367062500000163, -26.72916666530106866, -3.861377020970580443 ) ) ;
#23765=CARTESIAN_POINT ( 'NONE',  ( -2.229367062499996610, 3.604166668032260379, 3.861377020970582219 ) ) ;
#23768=CARTESIAN_POINT ( 'NONE',  ( -2.500000000000000444, 15.95833333606451809, -4.330127018922193649 ) ) ;
#23769=CARTESIAN_POINT ( 'NONE',  ( 5.000000000000000888, -96.58333333333332860, 2.886751345948126879 ) ) ;
#23770=CARTESIAN_POINT ( 'NONE',  ( -3.152548672688508926E-16, -28.56249999863440436, -5.148502694627439702 ) ) ;
#23771=CARTESIAN_POINT ( 'NONE',  ( 4.458734124999999437, -74.06249999863440792, -5.460374474430324690E-16 ) ) ;
#23773=CARTESIAN_POINT ( 'NONE',  ( -6.972266317189433020E-16, -102.1249999972688158, -5.000000000000000000 ) ) ;
#23775=CARTESIAN_POINT ( 'NONE',  ( -4.458734124999999437, 3.604166668032260379, -2.574251347313719407 ) ) ;
#23776=CARTESIAN_POINT ( 'NONE',  ( -4.458734124999999437, 29.43750000136559208, 0.000000000000000000 ) ) ;
#23777=CARTESIAN_POINT ( 'NONE',  ( 4.458734124999998549, -40.97916666530106511, -2.574251347313721627 ) ) ;
#23782=CARTESIAN_POINT ( 'NONE',  ( -4.458734124999999437, -68.31249999863439371, 0.000000000000000000 ) ) ;
#23783=CARTESIAN_POINT ( 'NONE',  ( -4.999999999999999112, -101.7916666639354446, 2.886751345948131764 ) ) ;
#23785=DIRECTION ( 'NONE',  ( -0.000000000000000000, 1.000000000000000000, -0.000000000000000000 ) ) ;
#23786=CARTESIAN_POINT ( 'NONE',  ( -3.152548672688508926E-16, -107.8124999986343937, -5.148502694627439702 ) ) ;
#23788=CARTESIAN_POINT ( 'NONE',  ( 2.500000000000002220, -56.66666666666667140, 4.330127018922192761 ) ) ;
#23789=CARTESIAN_POINT ( 'NONE',  ( -5.000000000000000000, -22.00000000000000000, 0.000000000000000000 ) ) ;
#23791=ORIENTED_EDGE ( 'NONE', *, *, #30578, .T. ) ;
#23792=CARTESIAN_POINT ( 'NONE',  ( -1.339745962155610925, -26.79465819873852084, 5.000000000000000000 ) ) ;
#23793=CARTESIAN_POINT ( 'NONE',  ( -4.999999999999998224, 13.08333333333333215, 2.886751345948131764 ) ) ;
#23800=VERTEX_POINT ( 'NONE', #3164 ) ;
#23807=CARTESIAN_POINT ( 'NONE',  ( -4.458734124999999437, -42.56249999863440081, 0.000000000000000000 ) ) ;
#23814=CARTESIAN_POINT ( 'NONE',  ( 2.499999999999998668, -26.33333333333333215, -4.330127018922193649 ) ) ;
#23816=CARTESIAN_POINT ( 'NONE',  ( -4.458734124999999437, -90.64583333196773651, -2.574251347313719407 ) ) ;
#23818=VERTEX_POINT ( 'NONE', #61389 ) ;
#23819=DIRECTION ( 'NONE',  ( -0.000000000000000000, 1.000000000000000000, -0.000000000000000000 ) ) ;
#23821=CARTESIAN_POINT ( 'NONE',  ( -4.999999999999998224, -104.9166666666666572, 2.886751345948131764 ) ) ;
#23824=( BOUNDED_CURVE ( )  B_SPLINE_CURVE ( 2, ( #7575, #27810, #16899, #2750, #3387, #60978, #36515, #27187, #22369 ),
 .UNSPECIFIED., .F., .F. ) 
 B_SPLINE_CURVE_WITH_KNOTS ( ( 3, 2, 2, 2, 3 ),
 ( 0.4375000000000000000, 0.4380952380952380931, 0.4392857142857142794, 0.4404761904761904656, 0.4410714285714285587 ),
 .UNSPECIFIED. ) 
 CURVE ( )  GEOMETRIC_REPRESENTATION_ITEM ( )  RATIONAL_B_SPLINE_CURVE ( ( 0.9330127018922194093, 0.9330127018922194093, 1.000000000000000000, 0.8660254037844387076, 1.000000000000000000, 0.8660254037844387076, 1.000000000000000000, 0.9330127018922194093, 0.9330127018922194093 ) ) 
 REPRESENTATION_ITEM ( '' )  );
#23826=CARTESIAN_POINT ( 'NONE',  ( 2.229367062500001939, -12.22916666530107044, 3.861377020970579999 ) ) ;
#23830=VECTOR ( 'NONE', #25149, 1000.000000000000000 ) ;
#23833=CARTESIAN_POINT ( 'NONE',  ( 9.457646018065525792E-16, 22.68750000136559564, 5.148502694627439702 ) ) ;
#23835=CARTESIAN_POINT ( 'NONE',  ( 4.458734124999998549, -89.72916666530106511, -2.574251347313721627 ) ) ;
#23836=FACE_OUTER_BOUND ( 'NONE', #60798, .T. ) ;
#23838=CARTESIAN_POINT ( 'NONE',  ( -3.152548672688508926E-16, -15.56249999863440614, -5.148502694627439702 ) ) ;
#23839=CARTESIAN_POINT ( 'NONE',  ( -4.999999999999998224, -84.79166666393547303, 2.886751345948131764 ) ) ;
#23842=CARTESIAN_POINT ( 'NONE',  ( 2.499999999999998668, -39.20833333060214443, -4.330127018922193649 ) ) ;
#23844=CARTESIAN_POINT ( 'NONE',  ( 4.458734124999998549, 17.27083333469892779, -2.574251347313721627 ) ) ;
#23845=CARTESIAN_POINT ( 'NONE',  ( 2.500000000000002220, -46.54166666393547303, 4.330127018922192761 ) ) ;
#23847=CARTESIAN_POINT ( 'NONE',  ( -4.458734124999999437, -58.31249999863440081, 0.000000000000000000 ) ) ;
#23849=LINE ( 'NONE', #14183, #8316 ) ;
#23850=CARTESIAN_POINT ( 'NONE',  ( -3.535250795749689387E-16, 8.750000000000000000, -5.773502691896257311 ) ) ;
#23853=CARTESIAN_POINT ( 'NONE',  ( 9.457646018065525792E-16, -52.06249999863440792, 5.148502694627439702 ) ) ;
#23854=CARTESIAN_POINT ( 'NONE',  ( -2.499999999999996447, -81.70833333060213022, 4.330127018922195425 ) ) ;
#23856=CARTESIAN_POINT ( 'NONE',  ( 1.975475456537005874E-15, -14.62499999726881228, 5.000000000000000000 ) ) ;
#23858=CARTESIAN_POINT ( 'NONE',  ( -2.229367062500000163, -91.72916666530106511, -3.861377020970580443 ) ) ;
#23860=CARTESIAN_POINT ( 'NONE',  ( -3.535250795749689387E-16, -39.24999999999999289, -5.773502691896257311 ) ) ;
#23862=CARTESIAN_POINT ( 'NONE',  ( 1.975475456537005874E-15, -85.62499999726880162, 5.000000000000000000 ) ) ;
#23864=CARTESIAN_POINT ( 'NONE',  ( 9.457646018065525792E-16, -94.06249999863439371, 5.148502694627439702 ) ) ;
#23865=CARTESIAN_POINT ( 'NONE',  ( -4.458734124999998549, 9.520833334698927786, 2.574251347313722516 ) ) ;
#23866=CARTESIAN_POINT ( 'NONE',  ( -5.000000000000000000, 13.04166666939785379, -2.886751345948128211 ) ) ;
#23870=CARTESIAN_POINT ( 'NONE',  ( -4.999999999999998224, 3.083333333333333925, 2.886751345948131764 ) ) ;
#23874=CARTESIAN_POINT ( 'NONE',  ( 5.000000000000000000, 19.50000000000000000, -6.123233995736766282E-16 ) ) ;
#23880=CARTESIAN_POINT ( 'NONE',  ( -4.458734124999999437, -26.64583333196773651, -2.574251347313719407 ) ) ;
#23881=CARTESIAN_POINT ( 'NONE',  ( -4.999999999999998224, 22.20833333606451987, 2.886751345948131764 ) ) ;
#23885=EDGE_CURVE ( 'NONE', #19213, #24693, #50323, .T. ) ;
#23889=EDGE_LOOP ( 'NONE', ( #31290, #20735, #47851, #20804 ) ) ;
#23892=CARTESIAN_POINT ( 'NONE',  ( -4.458734124999999437, -69.64583333196773651, -2.574251347313719407 ) ) ;
#23894=EDGE_LOOP ( 'NONE', ( #4414, #53612, #58979, #48488 ) ) ;
#23895=LINE ( 'NONE', #38060, #11661 ) ;
#23897=CARTESIAN_POINT ( 'NONE',  ( 2.229367062499998831, -0.8958333319677401763, -3.861377020970580887 ) ) ;
#23898=ORIENTED_EDGE ( 'NONE', *, *, #50417, .F. ) ;
#23900=CARTESIAN_POINT ( 'NONE',  ( -1.339745962155610925, -19.79465819873851729, 5.000000000000000000 ) ) ;
#23901=EDGE_CURVE ( 'NONE', #7254, #3563, #54453, .T. ) ;
#23907=CARTESIAN_POINT ( 'NONE',  ( 4.458734124999999437, -75.81249999863440792, -5.460374474430324690E-16 ) ) ;
#23909=CARTESIAN_POINT ( 'NONE',  ( -2.229367062500000163, 3.520833334698929118, -3.861377020970580443 ) ) ;
#23910=DIRECTION ( 'NONE',  ( -0.000000000000000000, 1.000000000000000000, -0.000000000000000000 ) ) ;
#23911=CARTESIAN_POINT ( 'NONE',  ( 2.229367062500001939, -65.22916666530106511, 3.861377020970579999 ) ) ;
#23912=CARTESIAN_POINT ( 'NONE',  ( 1.060575238724906964E-15, -17.62499999726881583, 5.773502691896257311 ) ) ;
#23914=CARTESIAN_POINT ( 'NONE',  ( 0.000000000000000000, -120.0000000000000000, 0.000000000000000000 ) ) ;
#23916=CARTESIAN_POINT ( 'NONE',  ( -5.000000000000000000, -105.8749999972688158, 0.000000000000000000 ) ) ;
#23917=DIRECTION ( 'NONE',  ( -0.000000000000000000, 1.000000000000000000, -0.000000000000000000 ) ) ;
#23918=CARTESIAN_POINT ( 'NONE',  ( -3.152548672688508926E-16, -40.56249999863440081, -5.148502694627439702 ) ) ;
#23919=CARTESIAN_POINT ( 'NONE',  ( -4.458734124999999437, -29.64583333196773651, -2.574251347313719407 ) ) ;
#23922=LINE ( 'NONE', #28430, #58624 ) ;
#23923=CARTESIAN_POINT ( 'NONE',  ( -2.499999999999996447, 26.16666666666666430, 4.330127018922195425 ) ) ;
#23925=CARTESIAN_POINT ( 'NONE',  ( 4.458734124999998549, -107.9791666653010651, -2.574251347313721627 ) ) ;
#23926=CARTESIAN_POINT ( 'NONE',  ( 9.457646018065525792E-16, -37.06249999863440792, 5.148502694627439702 ) ) ;
#23927=CARTESIAN_POINT ( 'NONE',  ( 5.000000000000000000, -69.29166666393548724, -2.886751345948129988 ) ) ;
#23931=CARTESIAN_POINT ( 'NONE',  ( -2.229367062499996610, -73.39583333196773651, 3.861377020970582219 ) ) ;
#23934=CARTESIAN_POINT ( 'NONE',  ( -1.339745962155613812, -28.08034179853028789, -5.000000000000000000 ) ) ;
#23936=CARTESIAN_POINT ( 'NONE',  ( 5.000000000000000000, -20.49999999999999645, -6.123233995736766282E-16 ) ) ;
#23940=CARTESIAN_POINT ( 'NONE',  ( -2.499999999999996447, -78.70833333060214443, 4.330127018922195425 ) ) ;
#23942=CARTESIAN_POINT ( 'NONE',  ( -2.500000000000000444, 27.95833333606451987, -4.330127018922193649 ) ) ;
#23945=DIRECTION ( 'NONE',  ( -0.000000000000000000, 1.000000000000000000, -0.000000000000000000 ) ) ;
#23949=CARTESIAN_POINT ( 'NONE',  ( 5.000000000000000888, -12.58333333333333570, 2.886751345948126879 ) ) ;
#23952=EDGE_CURVE ( 'NONE', #60902, #20484, #61054, .T. ) ;
#23957=CYLINDRICAL_SURFACE ( 'NONE', #13223, 5.000000000000000000 ) ;
#23958=CARTESIAN_POINT ( 'NONE',  ( -2.500000000000000444, -12.16666666666666607, -4.330127018922193649 ) ) ;
#23964=CARTESIAN_POINT ( 'NONE',  ( 2.499999999999998668, -53.20833333060213732, -4.330127018922193649 ) ) ;
#23969=EDGE_CURVE ( 'NONE', #22435, #24993, #3930, .T. ) ;
#23970=CARTESIAN_POINT ( 'NONE',  ( 4.458734125000001214, 18.10416666803225638, 2.574251347313718519 ) ) ;
#23977=CARTESIAN_POINT ( 'NONE',  ( 1.975475456537005874E-15, -102.7499999999999858, 5.000000000000000000 ) ) ;
#23978=CARTESIAN_POINT ( 'NONE',  ( 4.458734124999999437, -58.81249999863440081, -5.460374474430324690E-16 ) ) ;
#23979=CARTESIAN_POINT ( 'NONE',  ( 1.975475456537005874E-15, -11.62499999726881406, 5.000000000000000000 ) ) ;
#23980=CARTESIAN_POINT ( 'NONE',  ( 4.458734124999999437, 22.18750000136559564, -5.460374474430324690E-16 ) ) ;
#23981=CARTESIAN_POINT ( 'NONE',  ( 5.000000000000000000, -102.2916666639354588, -2.886751345948130876 ) ) ;
#23983=CARTESIAN_POINT ( 'NONE',  ( -4.458734124999999437, -46.64583333196774362, -2.574251347313719407 ) ) ;
#23984=CARTESIAN_POINT ( 'NONE',  ( 1.060575238724906964E-15, -1.624999997268814500, 5.773502691896257311 ) ) ;
#23986=DIRECTION ( 'NONE',  ( -0.000000000000000000, 1.000000000000000000, -0.000000000000000000 ) ) ;
#23988=CARTESIAN_POINT ( 'NONE',  ( 2.229367062500001939, -109.9791666653010651, 3.861377020970579999 ) ) ;
#23989=CARTESIAN_POINT ( 'NONE',  ( 4.458734124999999437, -13.06249999863440259, -5.460374474430324690E-16 ) ) ;
#23990=ORIENTED_EDGE ( 'NONE', *, *, #91, .T. ) ;
#23992=CARTESIAN_POINT ( 'NONE',  ( 4.458734124999999437, -97.81249999863440792, -5.460374474430324690E-16 ) ) ;
#23994=CARTESIAN_POINT ( 'NONE',  ( 9.457646018065525792E-16, -92.31249999863439371, 5.148502694627439702 ) ) ;
#23995=EDGE_CURVE ( 'NONE', #39107, #58623, #49561, .T. ) ;
#23996=CARTESIAN_POINT ( 'NONE',  ( 5.000000000000000000, -53.37499999726881583, -6.123233995736766282E-16 ) ) ;
#23997=DIRECTION ( 'NONE',  ( -0.000000000000000000, 1.000000000000000000, -0.000000000000000000 ) ) ;
#24001=CARTESIAN_POINT ( 'NONE',  ( 4.458734124999999437, -15.81249999863440436, -5.460374474430324690E-16 ) ) ;
#24002=CARTESIAN_POINT ( 'NONE',  ( 4.458734124999999437, 13.93750000136559386, -5.460374474430324690E-16 ) ) ;
#24003=CARTESIAN_POINT ( 'NONE',  ( -4.458734124999999437, -57.64583333196773651, -2.574251347313719407 ) ) ;
#24004=CARTESIAN_POINT ( 'NONE',  ( -2.499999999999996447, -68.83333333333332860, 4.330127018922195425 ) ) ;
#24011=CARTESIAN_POINT ( 'NONE',  ( 1.975475456537005874E-15, -66.74999999999998579, 5.000000000000000000 ) ) ;
#24013=CARTESIAN_POINT ( 'NONE',  ( -4.458734124999998549, -87.22916666530107932, 2.574251347313722516 ) ) ;
#24014=CARTESIAN_POINT ( 'NONE',  ( -2.229367062499996610, 16.60416666803225638, 3.861377020970582219 ) ) ;
#24018=CARTESIAN_POINT ( 'NONE',  ( 1.975475456537005874E-15, 7.249999999999998224, 5.000000000000000000 ) ) ;
#24020=CARTESIAN_POINT ( 'NONE',  ( -2.499999999999996447, -69.83333333333332860, 4.330127018922195425 ) ) ;
#24023=CARTESIAN_POINT ( 'NONE',  ( 5.000000000000000888, -102.5833333333333286, 2.886751345948126879 ) ) ;
#24025=EDGE_LOOP ( 'NONE', ( #53832, #35031, #420, #9310 ) ) ;
#24026=CARTESIAN_POINT ( 'NONE',  ( -5.000000000000000000, -79.87499999726881583, 0.000000000000000000 ) ) ;
#24039=EDGE_CURVE ( 'NONE', #37137, #30949, #28845, .T. ) ;
#24042=CARTESIAN_POINT ( 'NONE',  ( -4.458734124999998549, -59.47916666530106511, 2.574251347313722516 ) ) ;
#24044=CARTESIAN_POINT ( 'NONE',  ( -6.031010364368858512E-14, 3.375000002731183280, 5.000000000000000000 ) ) ;
#24045=ORIENTED_EDGE ( 'NONE', *, *, #55494, .T. ) ;
#24047=ADVANCED_FACE ( 'NONE', ( #8302 ), #47524, .T. ) ;
#24049=EDGE_CURVE ( 'NONE', #31719, #48295, #1501, .T. ) ;
#24051=VERTEX_POINT ( 'NONE', #60605 ) ;
#24054=CARTESIAN_POINT ( 'NONE',  ( 4.458734124999998549, -104.9791666653010651, -2.574251347313721627 ) ) ;
#24057=EDGE_CURVE ( 'NONE', #44922, #45518, #39221, .T. ) ;
#24060=CARTESIAN_POINT ( 'NONE',  ( 4.458734125000000326, -37.89583333196773651, 2.574251347313718519 ) ) ;
#24061=EDGE_CURVE ( 'NONE', #33389, #40505, #5609, .T. ) ;
#24062=EDGE_CURVE ( 'NONE', #4593, #25319, #8068, .T. ) ;
#24064=CARTESIAN_POINT ( 'NONE',  ( 2.229367062500001939, -12.97916666530107221, 3.861377020970579999 ) ) ;
#24065=CARTESIAN_POINT ( 'NONE',  ( 4.458734124999998549, -99.97916666530106511, -2.574251347313721627 ) ) ;
#24068=CARTESIAN_POINT ( 'NONE',  ( -4.458734124999999437, -25.56249999863440792, 0.000000000000000000 ) ) ;
#24075=CARTESIAN_POINT ( 'NONE',  ( 4.458734125000000326, 2.854166668032259491, 2.574251347313718519 ) ) ;
#24076=( BOUNDED_CURVE ( )  B_SPLINE_CURVE ( 2, ( #38548, #3532, #8977, #23141, #58179, #14424, #42749, #53039, #62392 ),
 .UNSPECIFIED., .F., .F. ) 
 B_SPLINE_CURVE_WITH_KNOTS ( ( 3, 2, 2, 2, 3 ),
 ( 0.2339285714285714302, 0.2345238095238095233, 0.2357142857142857095, 0.2369047619047618958, 0.2374999999999999889 ),
 .UNSPECIFIED. ) 
 CURVE ( )  GEOMETRIC_REPRESENTATION_ITEM ( )  RATIONAL_B_SPLINE_CURVE ( ( 0.9330127018922194093, 0.9330127018922194093, 1.000000000000000000, 0.8660254037844387076, 1.000000000000000000, 0.8660254037844387076, 1.000000000000000000, 0.9330127018922194093, 0.9330127018922194093 ) ) 
 REPRESENTATION_ITEM ( '' )  );
#24078=CARTESIAN_POINT ( 'NONE',  ( -4.999999999999998224, 2.083333333333333037, 2.886751345948131764 ) ) ;
#24079=CARTESIAN_POINT ( 'NONE',  ( 1.975475456537005874E-15, 16.37500000273118417, 5.000000000000000000 ) ) ;
#24080=CARTESIAN_POINT ( 'NONE',  ( -4.999999999999999112, -97.91666666666664298, 2.886751345948131764 ) ) ;
#24081=CARTESIAN_POINT ( 'NONE',  ( -4.458734124999998549, -29.22916666530107221, 2.574251347313722516 ) ) ;
#24082=CARTESIAN_POINT ( 'NONE',  ( 5.000000000000000888, -73.58333333333332860, 2.886751345948126879 ) ) ;
#24083=CARTESIAN_POINT ( 'NONE',  ( -3.152548672688508926E-16, -74.81249999863439371, -5.148502694627439702 ) ) ;
#24085=CARTESIAN_POINT ( 'NONE',  ( -2.500000000000000444, -102.0416666639354588, -4.330127018922193649 ) ) ;
#24087=CARTESIAN_POINT ( 'NONE',  ( -2.229367062500000163, 2.520833334698928230, -3.861377020970580443 ) ) ;
#24088=CARTESIAN_POINT ( 'NONE',  ( -3.152548672688508926E-16, 29.18750000136559208, -5.148502694627439702 ) ) ;
#24089=CARTESIAN_POINT ( 'NONE',  ( 2.229367062500001939, -45.22916666530106511, 3.861377020970579999 ) ) ;
#24090=CARTESIAN_POINT ( 'NONE',  ( 1.975475456537005874E-15, -55.74999999999999289, 5.000000000000000000 ) ) ;
#24092=ORIENTED_EDGE ( 'NONE', *, *, #33834, .T. ) ;
#24095=CARTESIAN_POINT ( 'NONE',  ( -4.458734124999999437, -71.39583333196773651, -2.574251347313719407 ) ) ;
#24096=CARTESIAN_POINT ( 'NONE',  ( -4.999999999999999112, -105.7916666639354588, 2.886751345948131764 ) ) ;
#24099=CARTESIAN_POINT ( 'NONE',  ( 9.457646018065525792E-16, -110.3124999986343937, 5.148502694627439702 ) ) ;
#24101=CARTESIAN_POINT ( 'NONE',  ( 5.000000000000000000, -54.41666666666666430, -2.886751345948129988 ) ) ;
#24102=CARTESIAN_POINT ( 'NONE',  ( -2.500000000000000444, -22.16666666666666785, -4.330127018922193649 ) ) ;
#24104=ORIENTED_EDGE ( 'NONE', *, *, #35780, .F. ) ;
#24106=( BOUNDED_CURVE ( )  B_SPLINE_CURVE ( 2, ( #906, #63620, #20514, #35620, #39155, #45264, #49127, #15361, #35298 ),
 .UNSPECIFIED., .F., .F. ) 
 B_SPLINE_CURVE_WITH_KNOTS ( ( 3, 2, 2, 2, 3 ),
 ( 0.001785714285714286092, 0.002380952380952381167, 0.003571428571428571317, 0.004761904761904762334, 0.005357142857142858060 ),
 .UNSPECIFIED. ) 
 CURVE ( )  GEOMETRIC_REPRESENTATION_ITEM ( )  RATIONAL_B_SPLINE_CURVE ( ( 0.9330127018922194093, 0.9330127018922194093, 1.000000000000000000, 0.8660254037844387076, 1.000000000000000000, 0.8660254037844387076, 1.000000000000000000, 0.9330127018922191873, 0.9330127018922192983 ) ) 
 REPRESENTATION_ITEM ( '' )  );
#24117=EDGE_LOOP ( 'NONE', ( #22542, #30415, #58304, #31811 ) ) ;
#24121=CARTESIAN_POINT ( 'NONE',  ( -2.229367062500000163, -42.72916666530107932, -3.861377020970580443 ) ) ;
#24130=CARTESIAN_POINT ( 'NONE',  ( -4.458734124999998549, -87.47916666530107932, 2.574251347313722516 ) ) ;
#24139=CARTESIAN_POINT ( 'NONE',  ( 9.457646018065525792E-16, -13.31249999863440259, 5.148502694627439702 ) ) ;
#24140=CARTESIAN_POINT ( 'NONE',  ( -1.339745962155610925, -34.79465819873851729, 5.000000000000000000 ) ) ;
#24142=CARTESIAN_POINT ( 'NONE',  ( -2.499999999999996447, 4.291666669397852907, 4.330127018922195425 ) ) ;
#24144=CARTESIAN_POINT ( 'NONE',  ( 2.229367062500001939, 21.77083333469892779, 3.861377020970579999 ) ) ;
#24145=ORIENTED_EDGE ( 'NONE', *, *, #13935, .T. ) ;
#24146=CARTESIAN_POINT ( 'NONE',  ( 4.458734124999998549, -91.72916666530106511, -2.574251347313721627 ) ) ;
#24147=CARTESIAN_POINT ( 'NONE',  ( -6.972266317189433020E-16, -34.12499999726881583, -5.000000000000000000 ) ) ;
#24149=CARTESIAN_POINT ( 'NONE',  ( 4.458734124999999437, -11.81249999863440081, -5.460374474430324690E-16 ) ) ;
#24151=CARTESIAN_POINT ( 'NONE',  ( -6.972266317189433020E-16, -73.25000000000000000, -5.000000000000000000 ) ) ;
#24153=CARTESIAN_POINT ( 'NONE',  ( -2.499999999999996447, -40.70833333060214443, 4.330127018922195425 ) ) ;
#24154=DIRECTION ( 'NONE',  ( -0.000000000000000000, 1.000000000000000000, -0.000000000000000000 ) ) ;
#24155=CARTESIAN_POINT ( 'NONE',  ( -4.458734124999997661, 16.77083333469892779, 2.574251347313722516 ) ) ;
#24156=CARTESIAN_POINT ( 'NONE',  ( 1.339745962155615144, -46.58034179853028434, 4.999999999999999112 ) ) ;
#24159=CARTESIAN_POINT ( 'NONE',  ( 9.457646018065525792E-16, -61.06249999863440081, 5.148502694627439702 ) ) ;
#24162=CARTESIAN_POINT ( 'NONE',  ( 5.000000000000000000, 12.50000000000000000, -6.123233995736766282E-16 ) ) ;
#24165=CARTESIAN_POINT ( 'NONE',  ( 2.229367062499998831, -54.64583333196773651, -3.861377020970580887 ) ) ;
#24166=CARTESIAN_POINT ( 'NONE',  ( -5.000000000000000000, -89.95833333060214443, -2.886751345948128211 ) ) ;
#24168=CARTESIAN_POINT ( 'NONE',  ( -1.339745962155610925, -104.6696581960073331, 5.000000000000000000 ) ) ;
#24169=CARTESIAN_POINT ( 'NONE',  ( -4.458734124999999437, -90.56249999863440792, 0.000000000000000000 ) ) ;
#24171=CARTESIAN_POINT ( 'NONE',  ( 2.499999999999998668, -38.33333333333332860, -4.330127018922193649 ) ) ;
#24172=DIRECTION ( 'NONE',  ( 0.000000000000000000, 0.000000000000000000, 1.000000000000000000 ) ) ;
#24173=CARTESIAN_POINT ( 'NONE',  ( 5.000000000000000000, -22.50000000000000000, -6.123233995736766282E-16 ) ) ;
#24175=CARTESIAN_POINT ( 'NONE',  ( 2.229367062500001939, -103.9791666653010651, 3.861377020970579999 ) ) ;
#24176=CARTESIAN_POINT ( 'NONE',  ( 9.457646018065525792E-16, 9.687500001365593860, 5.148502694627439702 ) ) ;
#24179=EDGE_CURVE ( 'NONE', #14365, #22959, #14609, .T. ) ;
#24183=EDGE_LOOP ( 'NONE', ( #49074, #20494, #31078, #36876 ) ) ;
#24184=DIRECTION ( 'NONE',  ( 0.000000000000000000, 0.000000000000000000, 1.000000000000000000 ) ) ;
#24188=CARTESIAN_POINT ( 'NONE',  ( 2.229367062500001939, -27.22916666530106866, 3.861377020970579999 ) ) ;
#24189=LINE ( 'NONE', #14215, #16302 ) ;
#24194=AXIS2_PLACEMENT_3D ( 'NONE', #29269, #53416, #47956 ) ;
#24199=CARTESIAN_POINT ( 'NONE',  ( 1.339745962155615144, -93.58034179853028434, 4.999999999999999112 ) ) ;
#24201=CARTESIAN_POINT ( 'NONE',  ( -3.152548672688508926E-16, -74.81249999863439371, -5.148502694627439702 ) ) ;
#24202=CARTESIAN_POINT ( 'NONE',  ( -6.972266317189433020E-16, -43.25000000000000000, -5.000000000000000000 ) ) ;
#24203=( NAMED_UNIT ( * ) SI_UNIT ( $, .STERADIAN. ) SOLID_ANGLE_UNIT ( ) );
#24204=EDGE_LOOP ( 'NONE', ( #54006, #58617, #2233 ) ) ;
#24208=CARTESIAN_POINT ( 'NONE',  ( -3.152548672688508926E-16, -0.8124999986344055847, -5.148502694627439702 ) ) ;
#24210=DIRECTION ( 'NONE',  ( 0.000000000000000000, 0.000000000000000000, 1.000000000000000000 ) ) ;
#24214=CARTESIAN_POINT ( 'NONE',  ( -1.339745962155610925, 6.330341803992665106, 5.000000000000000000 ) ) ;
#24216=VERTEX_POINT ( 'NONE', #47685 ) ;
#24217=CARTESIAN_POINT ( 'NONE',  ( 4.458734124999998549, -74.72916666530106511, -2.574251347313721627 ) ) ;
#24218=CARTESIAN_POINT ( 'NONE',  ( -6.972266317189433020E-16, -0.1249999972688142363, -5.000000000000000000 ) ) ;
#24219=CARTESIAN_POINT ( 'NONE',  ( 4.458734124999998549, 3.270833334698929118, -2.574251347313721627 ) ) ;
#24220=CARTESIAN_POINT ( 'NONE',  ( -5.000000000000000000, -42.87499999726880873, 0.000000000000000000 ) ) ;
#24221=CARTESIAN_POINT ( 'NONE',  ( -4.458734124999999437, -64.56249999863440792, 0.000000000000000000 ) ) ;
#24222=CARTESIAN_POINT ( 'NONE',  ( 5.000000000000000000, -27.29166666393547658, -2.886751345948129988 ) ) ;
#24224=CYLINDRICAL_SURFACE ( 'NONE', #34698, 5.000000000000000000 ) ;
#24226=LINE ( 'NONE', #9740, #21315 ) ;
#24227=CARTESIAN_POINT ( 'NONE',  ( 9.457646018065525792E-16, -45.06249999863440792, 5.148502694627439702 ) ) ;
#24228=CARTESIAN_POINT ( 'NONE',  ( 2.229367062500001939, -25.22916666530106866, 3.861377020970579999 ) ) ;
#24231=CARTESIAN_POINT ( 'NONE',  ( 5.000000000000000000, 27.58333333333332860, -2.886751345948129988 ) ) ;
#24233=CARTESIAN_POINT ( 'NONE',  ( 2.499999999999998668, -54.20833333060213732, -4.330127018922193649 ) ) ;
#24234=EDGE_CURVE ( 'NONE', #50232, #45912, #46431, .T. ) ;
#24235=CARTESIAN_POINT ( 'NONE',  ( -3.152548672688508926E-16, -38.56249999863439371, -5.148502694627439702 ) ) ;
#24236=CARTESIAN_POINT ( 'NONE',  ( 5.000000000000000000, -73.37499999726880162, -6.123233995736766282E-16 ) ) ;
#24240=CARTESIAN_POINT ( 'NONE',  ( -4.458734124999999437, -77.56249999863440792, 0.000000000000000000 ) ) ;
#24243=CARTESIAN_POINT ( 'NONE',  ( 0.000000000000000000, -120.0000000000000000, 5.000000000000000000 ) ) ;
#24244=DIRECTION ( 'NONE',  ( 0.000000000000000000, 0.000000000000000000, 1.000000000000000000 ) ) ;
#24245=CARTESIAN_POINT ( 'NONE',  ( -2.499999999999996447, -22.83333333333333215, 4.330127018922195425 ) ) ;
#24249=CARTESIAN_POINT ( 'NONE',  ( -1.339745962155610925, -48.79465819873850307, 5.000000000000000000 ) ) ;
#24253=CARTESIAN_POINT ( 'NONE',  ( 1.339745962155612702, -48.16965819600734022, -5.000000000000000000 ) ) ;
#24255=CARTESIAN_POINT ( 'NONE',  ( -5.000000000000000000, 8.041666669397852019, -2.886751345948128211 ) ) ;
#24257=CARTESIAN_POINT ( 'NONE',  ( 1.975475456537005874E-15, 15.25000000000000000, 5.000000000000000000 ) ) ;
#24258=CARTESIAN_POINT ( 'NONE',  ( 0.000000000000000000, -120.0000000000000000, 5.000000000000000000 ) ) ;
#24259=CARTESIAN_POINT ( 'NONE',  ( 5.000000000000000000, -89.37499999726880162, -6.123233995736766282E-16 ) ) ;
#24261=CARTESIAN_POINT ( 'NONE',  ( -2.229367062499996610, -23.14583333196773651, 3.861377020970582219 ) ) ;
#24265=EDGE_LOOP ( 'NONE', ( #15231, #24377, #3315, #38490 ) ) ;
#24267=ORIENTED_EDGE ( 'NONE', *, *, #14116, .F. ) ;
#24268=CARTESIAN_POINT ( 'NONE',  ( 5.000000000000000000, -4.499999999999997335, -6.123233995736766282E-16 ) ) ;
#24269=CARTESIAN_POINT ( 'NONE',  ( 0.000000000000000000, -120.0000000000000000, 0.000000000000000000 ) ) ;
#24271=EDGE_LOOP ( 'NONE', ( #34450, #54187, #5541, #21615 ) ) ;
#24273=AXIS2_PLACEMENT_3D ( 'NONE', #16751, #6476, #1659 ) ;
#24279=ORIENTED_EDGE ( 'NONE', *, *, #44760, .F. ) ;
#24280=AXIS2_PLACEMENT_3D ( 'NONE', #14173, #53417, #43754 ) ;
#24282=CARTESIAN_POINT ( 'NONE',  ( 2.229367062499998831, 21.35416666803226349, -3.861377020970580887 ) ) ;
#24286=CARTESIAN_POINT ( 'NONE',  ( -6.972266317189433020E-16, -88.25000000000000000, -5.000000000000000000 ) ) ;
#24287=CARTESIAN_POINT ( 'NONE',  ( 1.339745962155612702, -100.2946581987385315, -5.000000000000000000 ) ) ;
#24290=CARTESIAN_POINT ( 'NONE',  ( 4.458734124999998549, -58.72916666530106511, -2.574251347313721627 ) ) ;
#24292=CARTESIAN_POINT ( 'NONE',  ( 2.229367062500001939, 17.02083333469892779, 3.861377020970579999 ) ) ;
#24294=CARTESIAN_POINT ( 'NONE',  ( 2.229367062500001939, -50.22916666530107221, 3.861377020970579999 ) ) ;
#24295=CARTESIAN_POINT ( 'NONE',  ( 2.500000000000002220, -11.54166666393547835, 4.330127018922192761 ) ) ;
#24299=CARTESIAN_POINT ( 'NONE',  ( 4.458734124999999437, -105.8124999986344221, -5.460374474430324690E-16 ) ) ;
#24300=CARTESIAN_POINT ( 'NONE',  ( -4.458734124999999437, -13.64583333196774184, -2.574251347313719407 ) ) ;
#24303=CARTESIAN_POINT ( 'NONE',  ( 9.457646018065525792E-16, -101.0624999986344079, 5.148502694627439702 ) ) ;
#24305=CARTESIAN_POINT ( 'NONE',  ( 2.229367062499998831, -94.89583333196773651, -3.861377020970580887 ) ) ;
#24306=EDGE_CURVE ( 'NONE', #54724, #29833, #30203, .T. ) ;
#24308=CARTESIAN_POINT ( 'NONE',  ( -3.535250795749689387E-16, -51.12499999726880873, -5.773502691896257311 ) ) ;
#24311=CARTESIAN_POINT ( 'NONE',  ( -3.152548672688508926E-16, -20.56249999863440081, -5.148502694627439702 ) ) ;
#24312=CARTESIAN_POINT ( 'NONE',  ( 9.457646018065525792E-16, 9.687500001365593860, 5.148502694627439702 ) ) ;
#24313=CARTESIAN_POINT ( 'NONE',  ( 4.458734124999999437, -60.06249999863440081, -5.460374474430324690E-16 ) ) ;
#24318=CARTESIAN_POINT ( 'NONE',  ( 2.499999999999998668, -6.333333333333336590, -4.330127018922193649 ) ) ;
#24319=ORIENTED_EDGE ( 'NONE', *, *, #4109, .F. ) ;
#24323=CARTESIAN_POINT ( 'NONE',  ( -1.339745962155613812, -9.205341801261479162, -5.000000000000000000 ) ) ;
#24324=ADVANCED_FACE ( 'NONE', ( #33217 ), #32902, .T. ) ;
#24325=CARTESIAN_POINT ( 'NONE',  ( 1.975475456537005874E-15, -102.7499999999999858, 5.000000000000000000 ) ) ;
#24326=CARTESIAN_POINT ( 'NONE',  ( -2.229367062500000163, -87.47916666530107932, -3.861377020970580443 ) ) ;
#24327=CARTESIAN_POINT ( 'NONE',  ( 4.458734125000001214, 16.85416666803225638, 2.574251347313718519 ) ) ;
#24329=VECTOR ( 'NONE', #17611, 1000.000000000000000 ) ;
#24334=CARTESIAN_POINT ( 'NONE',  ( -6.972266317189433020E-16, -7.249999999999998224, -5.000000000000000000 ) ) ;
#24337=CARTESIAN_POINT ( 'NONE',  ( 2.499999999999998668, -76.33333333333334281, -4.330127018922193649 ) ) ;
#24348=ORIENTED_EDGE ( 'NONE', *, *, #28064, .F. ) ;
#24355=CARTESIAN_POINT ( 'NONE',  ( 4.458734124999999437, -55.06249999863440081, -5.460374474430324690E-16 ) ) ;
#24357=CARTESIAN_POINT ( 'NONE',  ( 2.499999999999998668, 3.791666669397852019, -4.330127018922193649 ) ) ;
#24358=ORIENTED_EDGE ( 'NONE', *, *, #9884, .F. ) ;
#24364=CARTESIAN_POINT ( 'NONE',  ( -4.458734124999998549, -107.4791666653010651, 2.574251347313722516 ) ) ;
#24369=CARTESIAN_POINT ( 'NONE',  ( 9.457646018065525792E-16, -38.06249999863440792, 5.148502694627439702 ) ) ;
#24373=CARTESIAN_POINT ( 'NONE',  ( -4.458734124999999437, -11.39583333196774007, -2.574251347313719407 ) ) ;
#24375=( BOUNDED_CURVE ( )  B_SPLINE_CURVE ( 2, ( #2884, #45978, #55958, #2560, #41140, #1943, #22497, #50495, #56275 ),
 .UNSPECIFIED., .F., .F. ) 
 B_SPLINE_CURVE_WITH_KNOTS ( ( 3, 2, 2, 2, 3 ),
 ( 0.6446428571428571841, 0.6452380952380952772, 0.6464285714285714635, 0.6476190476190476497, 0.6482142857142857428 ),
 .UNSPECIFIED. ) 
 CURVE ( )  GEOMETRIC_REPRESENTATION_ITEM ( )  RATIONAL_B_SPLINE_CURVE ( ( 0.9330127018922194093, 0.9330127018922194093, 1.000000000000000000, 0.8660254037844387076, 1.000000000000000000, 0.8660254037844387076, 1.000000000000000000, 0.9330127018922194093, 0.9330127018922194093 ) ) 
 REPRESENTATION_ITEM ( '' )  );
#24376=CARTESIAN_POINT ( 'NONE',  ( -4.458734124999997661, -98.47916666530105090, 2.574251347313722516 ) ) ;
#24377=ORIENTED_EDGE ( 'NONE', *, *, #11828, .F. ) ;
#24379=CARTESIAN_POINT ( 'NONE',  ( -4.458734124999999437, -31.64583333196773651, -2.574251347313719407 ) ) ;
#24380=AXIS2_PLACEMENT_3D ( 'NONE', #61998, #52960, #17918 ) ;
#24386=CARTESIAN_POINT ( 'NONE',  ( -2.229367062500000163, 6.270833334698928674, -3.861377020970580443 ) ) ;
#24389=CARTESIAN_POINT ( 'NONE',  ( 1.060575238724906964E-15, -95.75000000000000000, 5.773502691896257311 ) ) ;
#24390=CARTESIAN_POINT ( 'NONE',  ( -3.152548672688508926E-16, -27.56249999863440081, -5.148502694627439702 ) ) ;
#24392=CARTESIAN_POINT ( 'NONE',  ( 2.229367062500001939, -78.22916666530106511, 3.861377020970579999 ) ) ;
#24398=CARTESIAN_POINT ( 'NONE',  ( 4.458734124999999437, -4.812499998634402587, -5.460374474430324690E-16 ) ) ;
#24399=CARTESIAN_POINT ( 'NONE',  ( 9.457646018065525792E-16, 28.68750000136559208, 5.148502694627439702 ) ) ;
#24400=CARTESIAN_POINT ( 'NONE',  ( 2.229367062499998831, -43.89583333196774362, -3.861377020970580887 ) ) ;
#24405=CARTESIAN_POINT ( 'NONE',  ( 2.229367062500001939, -67.97916666530106511, 3.861377020970579999 ) ) ;
#24406=CARTESIAN_POINT ( 'NONE',  ( -2.499999999999996447, -103.7083333306021444, 4.330127018922195425 ) ) ;
#24409=CARTESIAN_POINT ( 'NONE',  ( -1.339745962155610925, 10.20534180126147739, 5.000000000000000000 ) ) ;
#24411=CARTESIAN_POINT ( 'NONE',  ( -4.458734124999999437, -109.5624999986343937, 0.000000000000000000 ) ) ;
#24413=CARTESIAN_POINT ( 'NONE',  ( 5.000000000000000888, -54.58333333333332860, 2.886751345948126879 ) ) ;
#24414=DIRECTION ( 'NONE',  ( -1.061635649774262822E-14, 0.000000000000000000, -1.000000000000000000 ) ) ;
#24417=CARTESIAN_POINT ( 'NONE',  ( 0.000000000000000000, -120.0000000000000000, 0.000000000000000000 ) ) ;
#24425=ORIENTED_EDGE ( 'NONE', *, *, #62998, .T. ) ;
#24426=CARTESIAN_POINT ( 'NONE',  ( -1.339745962155613812, -24.20534180126147206, -5.000000000000000000 ) ) ;
#24433=CARTESIAN_POINT ( 'NONE',  ( 2.229367062500001939, -39.22916666530107221, 3.861377020970579999 ) ) ;
#24439=CARTESIAN_POINT ( 'NONE',  ( 1.339745962155612702, -89.29465819873851729, -5.000000000000000000 ) ) ;
#24441=CARTESIAN_POINT ( 'NONE',  ( 2.229367062500001939, -90.22916666530106511, 3.861377020970579999 ) ) ;
#24442=CARTESIAN_POINT ( 'NONE',  ( 5.000000000000000888, -108.5833333333333144, 2.886751345948126879 ) ) ;
#24444=CARTESIAN_POINT ( 'NONE',  ( -5.000000000000000000, 14.04166666939785202, -2.886751345948128211 ) ) ;
#24449=CARTESIAN_POINT ( 'NONE',  ( 4.458734125000001214, 5.104166668032261711, 2.574251347313718519 ) ) ;
#24450=CARTESIAN_POINT ( 'NONE',  ( -4.999999999999998224, -70.79166666393547303, 2.886751345948131764 ) ) ;
#24451=CARTESIAN_POINT ( 'NONE',  ( -4.458734124999998549, -14.47916666530107221, 2.574251347313722516 ) ) ;
#24454=CARTESIAN_POINT ( 'NONE',  ( -4.999999999999998224, 4.208333336064518093, 2.886751345948131764 ) ) ;
#24457=CARTESIAN_POINT ( 'NONE',  ( -4.458734124999999437, 18.43750000136559564, 0.000000000000000000 ) ) ;
#24459=CARTESIAN_POINT ( 'NONE',  ( -4.458734124999999437, -96.39583333196773651, -2.574251347313719407 ) ) ;
#24462=CARTESIAN_POINT ( 'NONE',  ( -2.229367062499996610, -12.14583333196774007, 3.861377020970582219 ) ) ;
#24465=CARTESIAN_POINT ( 'NONE',  ( -6.972266317189433020E-16, -88.25000000000000000, -5.000000000000000000 ) ) ;
#24466=EDGE_CURVE ( 'NONE', #37025, #50637, #3557, .T. ) ;
#24467=CARTESIAN_POINT ( 'NONE',  ( -5.000000000000000000, -42.95833333060214443, -2.886751345948128211 ) ) ;
#24468=CARTESIAN_POINT ( 'NONE',  ( 0.000000000000000000, -120.0000000000000000, 0.000000000000000000 ) ) ;
#24469=CARTESIAN_POINT ( 'NONE',  ( 9.457646018065525792E-16, 12.93750000136559208, 5.148502694627439702 ) ) ;
#24470=CARTESIAN_POINT ( 'NONE',  ( 2.500000000000002220, -51.54166666393547303, 4.330127018922192761 ) ) ;
#24473=CARTESIAN_POINT ( 'NONE',  ( -2.229367062500000163, -60.47916666530106511, -3.861377020970580443 ) ) ;
#24475=( BOUNDED_CURVE ( )  B_SPLINE_CURVE ( 2, ( #27579, #49410, #53288, #866, #9224, #19503, #53914, #49086, #24334 ),
 .UNSPECIFIED., .F., .F. ) 
 B_SPLINE_CURVE_WITH_KNOTS ( ( 3, 2, 2, 2, 3 ),
 ( 0.2625000000000000111, 0.2630952380952381042, 0.2642857142857142905, 0.2654761904761904767, 0.2660714285714285698 ),
 .UNSPECIFIED. ) 
 CURVE ( )  GEOMETRIC_REPRESENTATION_ITEM ( )  RATIONAL_B_SPLINE_CURVE ( ( 0.9330127018922194093, 0.9330127018922194093, 1.000000000000000000, 0.8660254037844387076, 1.000000000000000000, 0.8660254037844387076, 1.000000000000000000, 0.9330127018922194093, 0.9330127018922194093 ) ) 
 REPRESENTATION_ITEM ( '' )  );
#24476=CARTESIAN_POINT ( 'NONE',  ( 2.499999999999998668, -109.2083333306021444, -4.330127018922193649 ) ) ;
#24477=CARTESIAN_POINT ( 'NONE',  ( 2.499999999999998668, 9.666666666666667851, -4.330127018922193649 ) ) ;
#24480=CARTESIAN_POINT ( 'NONE',  ( -2.229367062499996610, -51.14583333196772941, 3.861377020970582219 ) ) ;
#24481=CARTESIAN_POINT ( 'NONE',  ( 5.000000000000000888, -91.45833333060214443, 2.886751345948126879 ) ) ;
#24482=CARTESIAN_POINT ( 'NONE',  ( 4.458734124999999437, -27.81249999863440081, -5.460374474430324690E-16 ) ) ;
#24484=CARTESIAN_POINT ( 'NONE',  ( 1.339745962155612702, -14.16965819600733312, -5.000000000000000000 ) ) ;
#24488=CARTESIAN_POINT ( 'NONE',  ( 5.000000000000000000, -36.50000000000000711, -6.123233995736766282E-16 ) ) ;
#24493=CARTESIAN_POINT ( 'NONE',  ( 9.457646018065525792E-16, -103.0624999986344221, 5.148502694627439702 ) ) ;
#24494=CARTESIAN_POINT ( 'NONE',  ( -2.229367062499996610, 1.604166668032262155, 3.861377020970582219 ) ) ;
#24495=CARTESIAN_POINT ( 'NONE',  ( 5.000000000000000888, -80.58333333333332860, 2.886751345948126879 ) ) ;
#24503=VERTEX_POINT ( 'NONE', #14840 ) ;
#24505=CYLINDRICAL_SURFACE ( 'NONE', #48702, 5.000000000000000000 ) ;
#24509=CARTESIAN_POINT ( 'NONE',  ( -4.458734124999998549, -26.47916666530107221, 2.574251347313722516 ) ) ;
#24510=VECTOR ( 'NONE', #13275, 1000.000000000000000 ) ;
#24515=VECTOR ( 'NONE', #20478, 1000.000000000000000 ) ;
#24520=LINE ( 'NONE', #45408, #40271 ) ;
#24521=ORIENTED_EDGE ( 'NONE', *, *, #58600, .T. ) ;
#24522=CARTESIAN_POINT ( 'NONE',  ( 4.458734124999998549, -72.97916666530107932, -2.574251347313721627 ) ) ;
#24528=CARTESIAN_POINT ( 'NONE',  ( -3.152548672688508926E-16, 1.187500001365596081, -5.148502694627439702 ) ) ;
#24531=CARTESIAN_POINT ( 'NONE',  ( 2.500000000000002220, -69.54166666393547303, 4.330127018922192761 ) ) ;
#24536=VERTEX_POINT ( 'NONE', #34794 ) ;
#24537=CARTESIAN_POINT ( 'NONE',  ( 2.229367062499998831, -75.64583333196773651, -3.861377020970580887 ) ) ;
#24539=CARTESIAN_POINT ( 'NONE',  ( 4.458734124999998549, 1.270833334698927342, -2.574251347313721627 ) ) ;
#24540=CARTESIAN_POINT ( 'NONE',  ( -2.499999999999996447, -82.83333333333332860, 4.330127018922195425 ) ) ;
#24542=CARTESIAN_POINT ( 'NONE',  ( -2.229367062499996610, -64.39583333196773651, 3.861377020970582219 ) ) ;
#24543=CARTESIAN_POINT ( 'NONE',  ( -4.999999999999999112, -24.79166666393548368, 2.886751345948131764 ) ) ;
#24545=CARTESIAN_POINT ( 'NONE',  ( -2.229367062500000163, 28.52083333469892779, -3.861377020970580443 ) ) ;
#24546=CARTESIAN_POINT ( 'NONE',  ( -2.499999999999996447, -64.70833333060213022, 4.330127018922195425 ) ) ;
#24547=CARTESIAN_POINT ( 'NONE',  ( 9.457646018065525792E-16, -48.06249999863440081, 5.148502694627439702 ) ) ;
#24549=CARTESIAN_POINT ( 'NONE',  ( 2.229367062500001939, -30.22916666530107221, 3.861377020970579999 ) ) ;
#24551=STYLED_ITEM ( 'NONE', ( #4578 ), #23309 ) ;
#24553=CARTESIAN_POINT ( 'NONE',  ( -5.000000000000000000, 24.99999999999999645, 0.000000000000000000 ) ) ;
#24555=CARTESIAN_POINT ( 'NONE',  ( -1.339745962155613812, -50.20534180126148271, -5.000000000000000000 ) ) ;
#24556=AXIS2_PLACEMENT_3D ( 'NONE', #49834, #19926, #15751 ) ;
#24557=CARTESIAN_POINT ( 'NONE',  ( 4.458734124999998549, -39.72916666530107932, -2.574251347313721627 ) ) ;
#24558=CARTESIAN_POINT ( 'NONE',  ( -5.000000000000000000, -72.87499999726880162, 0.000000000000000000 ) ) ;
#24562=CARTESIAN_POINT ( 'NONE',  ( -4.458734124999999437, -76.56249999863440792, 0.000000000000000000 ) ) ;
#24567=CARTESIAN_POINT ( 'NONE',  ( -3.535250795749689387E-16, -24.24999999999999645, -5.773502691896257311 ) ) ;
#24573=CARTESIAN_POINT ( 'NONE',  ( 2.500000000000002220, 20.45833333606451987, 4.330127018922192761 ) ) ;
#24574=CARTESIAN_POINT ( 'NONE',  ( 5.000000000000000888, 4.541666669397852019, 2.886751345948126879 ) ) ;
#24579=CARTESIAN_POINT ( 'NONE',  ( -5.000000000000000000, 4.000000000000000000, 0.000000000000000000 ) ) ;
#24581=CARTESIAN_POINT ( 'NONE',  ( 1.339745962155612702, -89.16965819600733312, -5.000000000000000000 ) ) ;
#24582=CARTESIAN_POINT ( 'NONE',  ( 0.000000000000000000, -120.0000000000000000, 5.000000000000000000 ) ) ;
#24583=CARTESIAN_POINT ( 'NONE',  ( 1.975475456537005874E-15, -62.74999999999998579, 5.000000000000000000 ) ) ;
#24584=CARTESIAN_POINT ( 'NONE',  ( 4.458734125000001214, -21.89583333196773296, 2.574251347313718519 ) ) ;
#24585=CARTESIAN_POINT ( 'NONE',  ( 5.000000000000000000, -97.37499999726881583, -6.123233995736766282E-16 ) ) ;
#24589=ORIENTED_EDGE ( 'NONE', *, *, #55412, .F. ) ;
#24592=CARTESIAN_POINT ( 'NONE',  ( 0.000000000000000000, -120.0000000000000000, 0.000000000000000000 ) ) ;
#24593=CARTESIAN_POINT ( 'NONE',  ( -4.999999999999998224, -28.91666666666666430, 2.886751345948131764 ) ) ;
#24597=DIRECTION ( 'NONE',  ( -0.000000000000000000, 1.000000000000000000, -0.000000000000000000 ) ) ;
#24599=CARTESIAN_POINT ( 'NONE',  ( 5.000000000000000000, -53.29166666393548013, -2.886751345948130876 ) ) ;
#24602=CARTESIAN_POINT ( 'NONE',  ( 1.339745962155615144, -103.5803417985302701, 4.999999999999999112 ) ) ;
#24603=CARTESIAN_POINT ( 'NONE',  ( -2.229367062499996610, 20.85416666803226349, 3.861377020970582219 ) ) ;
#24608=DIRECTION ( 'NONE',  ( 0.000000000000000000, 0.000000000000000000, 1.000000000000000000 ) ) ;
#24609=CARTESIAN_POINT ( 'NONE',  ( 1.339745962155615144, -100.7053418012614827, 4.999999999999999112 ) ) ;
#24611=CARTESIAN_POINT ( 'NONE',  ( -4.458734124999999437, -59.39583333196773651, -2.574251347313719407 ) ) ;
#24613=CARTESIAN_POINT ( 'NONE',  ( 4.458734124999998549, 16.27083333469892779, -2.574251347313721627 ) ) ;
#24615=CARTESIAN_POINT ( 'NONE',  ( -3.152548672688508926E-16, -51.81249999863440792, -5.148502694627439702 ) ) ;
#24616=CARTESIAN_POINT ( 'NONE',  ( 5.000000000000000000, -9.291666663935483683, -2.886751345948129988 ) ) ;
#24618=CARTESIAN_POINT ( 'NONE',  ( 0.000000000000000000, -120.0000000000000000, 0.000000000000000000 ) ) ;
#24620=CARTESIAN_POINT ( 'NONE',  ( 2.229367062499998831, -108.6458333319677365, -3.861377020970580887 ) ) ;
#24621=CARTESIAN_POINT ( 'NONE',  ( -4.458734124999999437, -12.56249999863440259, 0.000000000000000000 ) ) ;
#24622=( BOUNDED_CURVE ( )  B_SPLINE_CURVE ( 2, ( #51066, #40451, #36275, #61359, #7010, #2199, #50437, #41082, #60091 ),
 .UNSPECIFIED., .F., .F. ) 
 B_SPLINE_CURVE_WITH_KNOTS ( ( 3, 2, 2, 2, 3 ),
 ( 0.01607142857142857331, 0.01666666666666666644, 0.01785714285714285615, 0.01904761904761904934, 0.01964285714285714593 ),
 .UNSPECIFIED. ) 
 CURVE ( )  GEOMETRIC_REPRESENTATION_ITEM ( )  RATIONAL_B_SPLINE_CURVE ( ( 0.9330127018922194093, 0.9330127018922195203, 1.000000000000000000, 0.8660254037844387076, 1.000000000000000000, 0.8660254037844387076, 1.000000000000000000, 0.9330127018922191873, 0.9330127018922194093 ) ) 
 REPRESENTATION_ITEM ( '' )  );
#24623=VERTEX_POINT ( 'NONE', #10023 ) ;
#24625=CARTESIAN_POINT ( 'NONE',  ( -4.458734124999999437, -97.31249999863440792, 0.000000000000000000 ) ) ;
#24627=CARTESIAN_POINT ( 'NONE',  ( 2.229367062499998831, -99.89583333196773651, -3.861377020970580887 ) ) ;
#24629=CARTESIAN_POINT ( 'NONE',  ( 2.500000000000002220, -57.54166666393548013, 4.330127018922192761 ) ) ;
#24633=CARTESIAN_POINT ( 'NONE',  ( -3.152548672688508926E-16, -19.56249999863440081, -5.148502694627439702 ) ) ;
#24634=CARTESIAN_POINT ( 'NONE',  ( -4.458734124999999437, 4.354166668032260823, -2.574251347313719407 ) ) ;
#24635=CARTESIAN_POINT ( 'NONE',  ( 2.229367062500001939, -60.22916666530106511, 3.861377020970579999 ) ) ;
#24638=CARTESIAN_POINT ( 'NONE',  ( 5.000000000000000000, -8.374999997268814056, -6.123233995736766282E-16 ) ) ;
#24640=CARTESIAN_POINT ( 'NONE',  ( -3.535250795749689387E-16, -6.249999999999998224, -5.773502691896257311 ) ) ;
#24646=CARTESIAN_POINT ( 'NONE',  ( 4.458734124999999437, -83.81249999863439371, -5.460374474430324690E-16 ) ) ;
#24647=CARTESIAN_POINT ( 'NONE',  ( 2.229367062500001939, 20.77083333469892779, 3.861377020970579999 ) ) ;
#24650=CARTESIAN_POINT ( 'NONE',  ( 1.975475456537005874E-15, -88.62499999726880162, 5.000000000000000000 ) ) ;
#24652=CARTESIAN_POINT ( 'NONE',  ( 2.499999999999998668, 20.79166666939784847, -4.330127018922193649 ) ) ;
#24654=CARTESIAN_POINT ( 'NONE',  ( -5.000000000000000000, -78.00000000000000000, 0.000000000000000000 ) ) ;
#24657=CARTESIAN_POINT ( 'NONE',  ( 0.000000000000000000, -120.0000000000000000, 0.000000000000000000 ) ) ;
#24659=CARTESIAN_POINT ( 'NONE',  ( -2.499999999999996447, -103.8333333333333286, 4.330127018922195425 ) ) ;
#24668=VERTEX_POINT ( 'NONE', #29635 ) ;
#24671=CARTESIAN_POINT ( 'NONE',  ( -4.458734124999998549, -55.47916666530107221, 2.574251347313722516 ) ) ;
#24677=EDGE_CURVE ( 'NONE', #34132, #45305, #12936, .T. ) ;
#24681=CARTESIAN_POINT ( 'NONE',  ( -2.229367062499996610, -106.3958333319677365, 3.861377020970582219 ) ) ;
#24686=CARTESIAN_POINT ( 'NONE',  ( -2.229367062499996610, -41.14583333196773651, 3.861377020970582219 ) ) ;
#24688=DIRECTION ( 'NONE',  ( -0.000000000000000000, 1.000000000000000000, -0.000000000000000000 ) ) ;
#24689=AXIS2_PLACEMENT_3D ( 'NONE', #32405, #7975, #57186 ) ;
#24690=CARTESIAN_POINT ( 'NONE',  ( 1.975475456537005874E-15, 9.375000002731185944, 5.000000000000000000 ) ) ;
#24691=CARTESIAN_POINT ( 'NONE',  ( -2.229367062500000163, -10.47916666530106866, -3.861377020970580443 ) ) ;
#24692=CARTESIAN_POINT ( 'NONE',  ( 4.458734124999998549, -102.9791666653010651, -2.574251347313721627 ) ) ;
#24693=VERTEX_POINT ( 'NONE', #33530 ) ;
#24694=EDGE_CURVE ( 'NONE', #22715, #2538, #40917, .T. ) ;
#24696=CARTESIAN_POINT ( 'NONE',  ( 9.457646018065525792E-16, -34.31249999863440792, 5.148502694627439702 ) ) ;
#24697=EDGE_CURVE ( 'NONE', #6026, #22810, #27775, .T. ) ;
#24698=CARTESIAN_POINT ( 'NONE',  ( 5.000000000000000000, 7.625000002731186832, -6.123233995736766282E-16 ) ) ;
#24699=CARTESIAN_POINT ( 'NONE',  ( -6.000000000000000000, -114.9999999999999858, -1.500000000000000000 ) ) ;
#24705=CARTESIAN_POINT ( 'NONE',  ( 2.229367062499998831, 6.104166668032262599, -3.861377020970580887 ) ) ;
#24707=CARTESIAN_POINT ( 'NONE',  ( 0.000000000000000000, -120.0000000000000000, 5.000000000000000000 ) ) ;
#24708=CARTESIAN_POINT ( 'NONE',  ( 5.000000000000000888, 2.416666666666667851, 2.886751345948126879 ) ) ;
#24709=CARTESIAN_POINT ( 'NONE',  ( 1.060575238724906964E-15, -94.75000000000000000, 5.773502691896257311 ) ) ;
#24710=CARTESIAN_POINT ( 'NONE',  ( -4.458734124999998549, -31.22916666530107221, 2.574251347313722516 ) ) ;
#24711=CARTESIAN_POINT ( 'NONE',  ( -4.458734124999999437, -79.56249999863440792, 0.000000000000000000 ) ) ;
#24713=CYLINDRICAL_SURFACE ( 'NONE', #49997, 5.000000000000000000 ) ;
#24716=CARTESIAN_POINT ( 'NONE',  ( -2.229367062500000163, -0.4791666653010707710, -3.861377020970580443 ) ) ;
#24717=CARTESIAN_POINT ( 'NONE',  ( 4.458734124999999437, 21.93750000136559208, -5.460374474430324690E-16 ) ) ;
#24718=CARTESIAN_POINT ( 'NONE',  ( 2.229367062500001939, -41.22916666530107932, 3.861377020970579999 ) ) ;
#24719=CARTESIAN_POINT ( 'NONE',  ( -6.972266317189433020E-16, -46.12499999726880873, -5.000000000000000000 ) ) ;
#24721=ORIENTED_EDGE ( 'NONE', *, *, #57204, .F. ) ;
#24723=CARTESIAN_POINT ( 'NONE',  ( 2.229367062499998831, -70.64583333196773651, -3.861377020970580887 ) ) ;
#24724=CARTESIAN_POINT ( 'NONE',  ( 2.500000000000002220, -103.5416666639354730, 4.330127018922192761 ) ) ;
#24726=CARTESIAN_POINT ( 'NONE',  ( -5.000000000000000000, 9.916666666666667851, -2.886751345948128211 ) ) ;
#24727=EDGE_CURVE ( 'NONE', #36804, #29555, #10107, .T. ) ;
#24728=CARTESIAN_POINT ( 'NONE',  ( 4.458734125000000326, -110.1458333319677365, 2.574251347313718519 ) ) ;
#24730=CARTESIAN_POINT ( 'NONE',  ( -5.000000000000000000, -62.00000000000000000, 0.000000000000000000 ) ) ;
#24731=CARTESIAN_POINT ( 'NONE',  ( -4.999999999999998224, -21.91666666666666785, 2.886751345948131764 ) ) ;
#24738=VECTOR ( 'NONE', #10091, 1000.000000000000000 ) ;
#24743=ORIENTED_EDGE ( 'NONE', *, *, #61479, .T. ) ;
#24744=CARTESIAN_POINT ( 'NONE',  ( -5.000000000000000000, -75.87499999726880162, 0.000000000000000000 ) ) ;
#24749=CARTESIAN_POINT ( 'NONE',  ( -2.229367062500000163, -43.72916666530106511, -3.861377020970580443 ) ) ;
#24750=CARTESIAN_POINT ( 'NONE',  ( -2.499999999999996447, -15.70833333060214443, 4.330127018922195425 ) ) ;
#24752=CYLINDRICAL_SURFACE ( 'NONE', #8732, 5.000000000000000000 ) ;
#24754=EDGE_CURVE ( 'NONE', #62985, #58767, #10658, .T. ) ;
#24758=EDGE_CURVE ( 'NONE', #44925, #1202, #16704, .T. ) ;
#24761=CARTESIAN_POINT ( 'NONE',  ( -2.229367062500000163, -87.72916666530107932, -3.861377020970580443 ) ) ;
#24763=VERTEX_POINT ( 'NONE', #36383 ) ;
#24764=CARTESIAN_POINT ( 'NONE',  ( 7.204675194429079505E-15, 26.87500000273118417, -5.000000000000000000 ) ) ;
#24769=CARTESIAN_POINT ( 'NONE',  ( -4.458734124999998549, 1.770833334698927786, 2.574251347313722516 ) ) ;
#24771=CARTESIAN_POINT ( 'NONE',  ( -2.500000000000000444, -14.16666666666666785, -4.330127018922193649 ) ) ;
#24772=CARTESIAN_POINT ( 'NONE',  ( -4.458734124999998549, -15.47916666530107399, 2.574251347313722516 ) ) ;
#24773=EDGE_CURVE ( 'NONE', #24693, #57442, #20650, .T. ) ;
#24774=CARTESIAN_POINT ( 'NONE',  ( -4.999999999999998224, -100.9166666666666572, 2.886751345948131764 ) ) ;
#24776=CARTESIAN_POINT ( 'NONE',  ( -5.000000000000000000, 4.125000002731186832, 0.000000000000000000 ) ) ;
#24778=CARTESIAN_POINT ( 'NONE',  ( -4.458734124999999437, 22.35416666803225638, -2.574251347313719407 ) ) ;
#24780=CARTESIAN_POINT ( 'NONE',  ( -4.458734124999997661, -99.22916666530105090, 2.574251347313722516 ) ) ;
#24782=CARTESIAN_POINT ( 'NONE',  ( 9.457646018065525792E-16, -13.06249999863440259, 5.148502694627439702 ) ) ;
#24786=CARTESIAN_POINT ( 'NONE',  ( 2.499999999999998668, -43.20833333060214443, -4.330127018922193649 ) ) ;
#24787=CARTESIAN_POINT ( 'NONE',  ( 1.339745962155615144, -67.58034179853029855, 4.999999999999999112 ) ) ;
#24788=CARTESIAN_POINT ( 'NONE',  ( 2.229367062499998831, 13.35416666803226171, -3.861377020970580887 ) ) ;
#24792=CARTESIAN_POINT ( 'NONE',  ( -2.229367062500000163, -64.47916666530106511, -3.861377020970580443 ) ) ;
#24793=ORIENTED_EDGE ( 'NONE', *, *, #60942, .T. ) ;
#24797=CARTESIAN_POINT ( 'NONE',  ( -4.999999999999999112, 3.083333333333333925, 2.886751345948131764 ) ) ;
#24799=DIRECTION ( 'NONE',  ( 0.000000000000000000, 0.000000000000000000, 1.000000000000000000 ) ) ;
#24800=CARTESIAN_POINT ( 'NONE',  ( -4.458734124999998549, -54.22916666530107221, 2.574251347313722516 ) ) ;
#24801=CARTESIAN_POINT ( 'NONE',  ( 2.500000000000002220, -88.54166666393548724, 4.330127018922192761 ) ) ;
#24802=CARTESIAN_POINT ( 'NONE',  ( -2.229367062500000163, -35.47916666530107221, -3.861377020970580443 ) ) ;
#24804=CARTESIAN_POINT ( 'NONE',  ( 1.975475456537005874E-15, -98.62499999726880162, 5.000000000000000000 ) ) ;
#24807=( BOUNDED_CURVE ( )  B_SPLINE_CURVE ( 2, ( #61965, #28480, #52616, #62599, #42956, #18521, #58066, #48095, #4050 ),
 .UNSPECIFIED., .F., .F. ) 
 B_SPLINE_CURVE_WITH_KNOTS ( ( 3, 2, 2, 2, 3 ),
 ( 0.3339285714285714080, 0.3345238095238095011, 0.3357142857142856873, 0.3369047619047619291, 0.3375000000000000222 ),
 .UNSPECIFIED. ) 
 CURVE ( )  GEOMETRIC_REPRESENTATION_ITEM ( )  RATIONAL_B_SPLINE_CURVE ( ( 0.9330127018922194093, 0.9330127018922194093, 1.000000000000000000, 0.8660254037844387076, 1.000000000000000000, 0.8660254037844387076, 1.000000000000000000, 0.9330127018922194093, 0.9330127018922194093 ) ) 
 REPRESENTATION_ITEM ( '' )  );
#24808=CARTESIAN_POINT ( 'NONE',  ( -2.500000000000000444, -44.16666666666665719, -4.330127018922193649 ) ) ;
#24809=CARTESIAN_POINT ( 'NONE',  ( 2.500000000000002220, -98.54166666393545881, 4.330127018922192761 ) ) ;
#24812=CARTESIAN_POINT ( 'NONE',  ( 2.229367062499998831, -100.6458333319677365, -3.861377020970580887 ) ) ;
#24813=CARTESIAN_POINT ( 'NONE',  ( -3.152548672688508926E-16, 5.187500001365592972, -5.148502694627439702 ) ) ;
#24823=VERTEX_POINT ( 'NONE', #709 ) ;
#24827=CARTESIAN_POINT ( 'NONE',  ( -4.458734124999999437, -24.64583333196773651, -2.574251347313719407 ) ) ;
#24835=EDGE_CURVE ( 'NONE', #13829, #18331, #56156, .T. ) ;
#24839=ORIENTED_EDGE ( 'NONE', *, *, #25650, .F. ) ;
#24840=CARTESIAN_POINT ( 'NONE',  ( -2.229367062500000163, -72.72916666530107932, -3.861377020970580443 ) ) ;
#24843=ORIENTED_EDGE ( 'NONE', *, *, #47934, .F. ) ;
#24847=CARTESIAN_POINT ( 'NONE',  ( 4.458734124999998549, -3.979166665301070438, -2.574251347313721627 ) ) ;
#24848=ORIENTED_EDGE ( 'NONE', *, *, #10820, .T. ) ;
#24855=DIRECTION ( 'NONE',  ( -0.000000000000000000, 1.000000000000000000, -0.000000000000000000 ) ) ;
#24857=( BOUNDED_CURVE ( )  B_SPLINE_CURVE ( 2, ( #12678, #47094, #37442, #60633, #6911, #12037, #36177, #11715, #21707 ),
 .UNSPECIFIED., .F., .F. ) 
 B_SPLINE_CURVE_WITH_KNOTS ( ( 3, 2, 2, 2, 3 ),
 ( 0.9803571428571428159, 0.9809523809523809090, 0.9821428571428570953, 0.9833333333333332815, 0.9839285714285714857 ),
 .UNSPECIFIED. ) 
 CURVE ( )  GEOMETRIC_REPRESENTATION_ITEM ( )  RATIONAL_B_SPLINE_CURVE ( ( 0.9330127018922194093, 0.9330127018922194093, 1.000000000000000000, 0.8660254037844387076, 1.000000000000000000, 0.8660254037844387076, 1.000000000000000000, 0.9330127018922130810, 0.9330127018922194093 ) ) 
 REPRESENTATION_ITEM ( '' )  );
#24859=ADVANCED_FACE ( 'NONE', ( #11926 ), #61791, .T. ) ;
#24860=CARTESIAN_POINT ( 'NONE',  ( -3.152548672688508926E-16, -79.56249999863440792, -5.148502694627439702 ) ) ;
#24862=CARTESIAN_POINT ( 'NONE',  ( 2.500000000000002220, -0.5416666639354792423, 4.330127018922192761 ) ) ;
#24863=CARTESIAN_POINT ( 'NONE',  ( 9.457646018065525792E-16, 2.937500001365594304, 5.148502694627439702 ) ) ;
#24864=CARTESIAN_POINT ( 'NONE',  ( -3.535250795749689387E-16, -86.25000000000000000, -5.773502691896257311 ) ) ;
#24866=CARTESIAN_POINT ( 'NONE',  ( -4.458734124999998549, -63.47916666530106511, 2.574251347313722516 ) ) ;
#24867=CARTESIAN_POINT ( 'NONE',  ( 5.000000000000000888, -26.45833333060214443, 2.886751345948126879 ) ) ;
#24869=CARTESIAN_POINT ( 'NONE',  ( -6.972266317189433020E-16, -41.24999999999998579, -5.000000000000000000 ) ) ;
#24871=CARTESIAN_POINT ( 'NONE',  ( 2.499999999999998668, -3.208333330602147093, -4.330127018922193649 ) ) ;
#24872=CARTESIAN_POINT ( 'NONE',  ( -3.152548672688508926E-16, -48.56249999863440792, -5.148502694627439702 ) ) ;
#24873=CARTESIAN_POINT ( 'NONE',  ( 2.229367062500001939, -34.22916666530107221, 3.861377020970579999 ) ) ;
#24876=CARTESIAN_POINT ( 'NONE',  ( 5.000000000000000000, 22.50000000000000000, -6.123233995736766282E-16 ) ) ;
#24878=CARTESIAN_POINT ( 'NONE',  ( -2.500000000000000444, -50.16666666666666430, -4.330127018922193649 ) ) ;
#24879=CARTESIAN_POINT ( 'NONE',  ( -2.229367062499996610, -35.14583333196772941, 3.861377020970582219 ) ) ;
#24880=CARTESIAN_POINT ( 'NONE',  ( 5.000000000000000000, -71.37499999726880162, -6.123233995736766282E-16 ) ) ;
#24883=CARTESIAN_POINT ( 'NONE',  ( 2.499999999999998668, -37.33333333333332860, -4.330127018922193649 ) ) ;
#24884=CARTESIAN_POINT ( 'NONE',  ( 2.229367062500001939, -82.22916666530106511, 3.861377020970579999 ) ) ;
#24887=CARTESIAN_POINT ( 'NONE',  ( 1.975475456537005874E-15, -70.62499999726880162, 5.000000000000000000 ) ) ;
#24889=CARTESIAN_POINT ( 'NONE',  ( 5.000000000000000000, -24.50000000000000000, -6.123233995736766282E-16 ) ) ;
#24893=ORIENTED_EDGE ( 'NONE', *, *, #36239, .F. ) ;
#24895=CARTESIAN_POINT ( 'NONE',  ( 2.499999999999998668, 19.79166666939785202, -4.330127018922193649 ) ) ;
#24896=CARTESIAN_POINT ( 'NONE',  ( 2.500000000000002220, -48.54166666393547303, 4.330127018922192761 ) ) ;
#24901=CARTESIAN_POINT ( 'NONE',  ( 5.000000000000000000, -91.37499999726880162, -6.123233995736766282E-16 ) ) ;
#24904=CARTESIAN_POINT ( 'NONE',  ( -4.999999999999998224, -78.91666666666665719, 2.886751345948131764 ) ) ;
#24905=CARTESIAN_POINT ( 'NONE',  ( -2.229367062500000163, -19.47916666530106866, -3.861377020970580443 ) ) ;
#24906=CARTESIAN_POINT ( 'NONE',  ( 1.339745962155612702, 10.83034180399266511, -5.000000000000000000 ) ) ;
#24910=ORIENTED_EDGE ( 'NONE', *, *, #13894, .T. ) ;
#24913=ORIENTED_EDGE ( 'NONE', *, *, #5012, .F. ) ;
#24915=CARTESIAN_POINT ( 'NONE',  ( 1.339745962155627135, 11.83034180399266333, -4.999999999999991118 ) ) ;
#24917=ORIENTED_EDGE ( 'NONE', *, *, #59143, .T. ) ;
#24923=CARTESIAN_POINT ( 'NONE',  ( -6.972266317189433020E-16, -54.24999999999999289, -5.000000000000000000 ) ) ;
#24924=CARTESIAN_POINT ( 'NONE',  ( -2.229367062499996610, 11.85416666803225993, 3.861377020970582219 ) ) ;
#24925=CARTESIAN_POINT ( 'NONE',  ( -5.000000000000000000, -9.958333330602144429, -2.886751345948128211 ) ) ;
#24929=CYLINDRICAL_SURFACE ( 'NONE', #793, 5.000000000000000000 ) ;
#24932=CARTESIAN_POINT ( 'NONE',  ( 2.229367062499998831, -65.64583333196773651, -3.861377020970580887 ) ) ;
#24934=CARTESIAN_POINT ( 'NONE',  ( -2.229367062500000163, 19.52083333469893134, -3.861377020970580443 ) ) ;
#24938=CARTESIAN_POINT ( 'NONE',  ( -4.458734124999998549, -47.47916666530106511, 2.574251347313722516 ) ) ;
#24939=CARTESIAN_POINT ( 'NONE',  ( 5.000000000000000000, -11.29166666393547835, -2.886751345948129988 ) ) ;
#24940=CARTESIAN_POINT ( 'NONE',  ( 1.975475456537005874E-15, -25.62499999726881228, 5.000000000000000000 ) ) ;
#24941=CARTESIAN_POINT ( 'NONE',  ( -5.000000000000000000, -65.87499999726881583, 0.000000000000000000 ) ) ;
#24943=CARTESIAN_POINT ( 'NONE',  ( 4.458734125000000326, -108.8958333319677365, 2.574251347313718519 ) ) ;
#24944=CARTESIAN_POINT ( 'NONE',  ( 4.458734124999999437, -15.06249999863440436, -5.460374474430324690E-16 ) ) ;
#24947=CARTESIAN_POINT ( 'NONE',  ( 4.458734124999999437, -103.8124999986344079, -5.460374474430324690E-16 ) ) ;
#24949=CARTESIAN_POINT ( 'NONE',  ( -4.458734124999998549, -97.47916666530106511, 2.574251347313722516 ) ) ;
#24951=CARTESIAN_POINT ( 'NONE',  ( 5.000000000000000000, -57.29166666393548013, -2.886751345948129988 ) ) ;
#24956=CARTESIAN_POINT ( 'NONE',  ( 9.457646018065525792E-16, -20.06249999863440081, 5.148502694627439702 ) ) ;
#24957=CARTESIAN_POINT ( 'NONE',  ( -4.458734124999998549, 5.520833334698927786, 2.574251347313722516 ) ) ;
#24958=CARTESIAN_POINT ( 'NONE',  ( -3.152548672688508926E-16, -66.81249999863440792, -5.148502694627439702 ) ) ;
#24963=CARTESIAN_POINT ( 'NONE',  ( 5.000000000000000000, -6.416666666666666963, -2.886751345948129988 ) ) ;
#24964=ORIENTED_EDGE ( 'NONE', *, *, #12119, .F. ) ;
#24969=CARTESIAN_POINT ( 'NONE',  ( 9.457646018065525792E-16, -90.06249999863440792, 5.148502694627439702 ) ) ;
#24970=CARTESIAN_POINT ( 'NONE',  ( -4.458734124999999437, 16.35416666803225993, -2.574251347313719407 ) ) ;
#24972=CARTESIAN_POINT ( 'NONE',  ( 5.000000000000000000, -93.50000000000000000, -6.123233995736766282E-16 ) ) ;
#24974=DIRECTION ( 'NONE',  ( -0.000000000000000000, 1.000000000000000000, -0.000000000000000000 ) ) ;
#24976=CARTESIAN_POINT ( 'NONE',  ( -4.999999999999999112, -76.91666666666667140, 2.886751345948131764 ) ) ;
#24979=DIRECTION ( 'NONE',  ( 0.000000000000000000, 0.000000000000000000, 1.000000000000000000 ) ) ;
#24984=ORIENTED_EDGE ( 'NONE', *, *, #55822, .T. ) ;
#24988=ORIENTED_EDGE ( 'NONE', *, *, #43639, .T. ) ;
#24991=CARTESIAN_POINT ( 'NONE',  ( -2.229367062500000163, -61.72916666530106511, -3.861377020970580443 ) ) ;
#24993=VERTEX_POINT ( 'NONE', #22870 ) ;
#24999=CARTESIAN_POINT ( 'NONE',  ( 2.229367062500001939, -103.2291666653010651, 3.861377020970579999 ) ) ;
#25004=CARTESIAN_POINT ( 'NONE',  ( 4.458734124999999437, -44.81249999863440081, -5.460374474430324690E-16 ) ) ;
#25008=CARTESIAN_POINT ( 'NONE',  ( -2.229367062499996610, -47.14583333196774362, 3.861377020970582219 ) ) ;
#25010=CARTESIAN_POINT ( 'NONE',  ( -4.458734124999999437, -11.31249999863440792, 0.000000000000000000 ) ) ;
#25011=CARTESIAN_POINT ( 'NONE',  ( 5.000000000000000000, -103.4166666666666430, -2.886751345948129988 ) ) ;
#25013=CARTESIAN_POINT ( 'NONE',  ( -2.229367062499996610, -34.39583333196772941, 3.861377020970582219 ) ) ;
#25014=CARTESIAN_POINT ( 'NONE',  ( 5.000000000000000000, 4.708333336064518093, -2.886751345948129988 ) ) ;
#25015=CARTESIAN_POINT ( 'NONE',  ( -4.729367062499999719, 29.84375000068279604, 0.000000000000000000 ) ) ;
#25020=CARTESIAN_POINT ( 'NONE',  ( 1.339745962155612702, -30.16965819600732956, -5.000000000000000000 ) ) ;
#25021=CARTESIAN_POINT ( 'NONE',  ( 2.229367062500001939, 0.7708333346989268975, 3.861377020970579999 ) ) ;
#25024=CARTESIAN_POINT ( 'NONE',  ( -4.999999999999999112, -94.91666666666667140, 2.886751345948131764 ) ) ;
#25025=CARTESIAN_POINT ( 'NONE',  ( -3.152548672688508926E-16, -36.56249999863441502, -5.148502694627439702 ) ) ;
#25026=CARTESIAN_POINT ( 'NONE',  ( 2.499999999999998668, -95.33333333333332860, -4.330127018922193649 ) ) ;
#25027=CARTESIAN_POINT ( 'NONE',  ( 4.458734124999999437, -82.06249999863440792, -5.460374474430324690E-16 ) ) ;
#25029=CYLINDRICAL_SURFACE ( 'NONE', #53077, 5.000000000000000000 ) ;
#25032=CARTESIAN_POINT ( 'NONE',  ( -4.458734124999999437, -3.312499998634407916, 0.000000000000000000 ) ) ;
#25033=CARTESIAN_POINT ( 'NONE',  ( 4.458734124999998549, 23.02083333469892423, -2.574251347313721627 ) ) ;
#25034=CARTESIAN_POINT ( 'NONE',  ( -2.229367062499996610, -41.39583333196773651, 3.861377020970582219 ) ) ;
#25038=CARTESIAN_POINT ( 'NONE',  ( -4.458734124999999437, -75.31249999863440792, 0.000000000000000000 ) ) ;
#25039=CARTESIAN_POINT ( 'NONE',  ( -5.000000000000000000, -105.8749999972688158, 0.000000000000000000 ) ) ;
#25043=CARTESIAN_POINT ( 'NONE',  ( 4.458734124999998549, -109.9791666653010509, -2.574251347313721627 ) ) ;
#25045=CARTESIAN_POINT ( 'NONE',  ( 5.000000000000000888, -60.58333333333332860, 2.886751345948126879 ) ) ;
#25046=CARTESIAN_POINT ( 'NONE',  ( 1.339745962155615144, -36.58034179853029855, 4.999999999999999112 ) ) ;
#25048=ORIENTED_EDGE ( 'NONE', *, *, #62274, .F. ) ;
#25049=DIRECTION ( 'NONE',  ( -0.000000000000000000, 1.000000000000000000, -0.000000000000000000 ) ) ;
#25059=CARTESIAN_POINT ( 'NONE',  ( 2.500000000000002220, -35.54166666393547303, 4.330127018922192761 ) ) ;
#25066=CARTESIAN_POINT ( 'NONE',  ( -4.458734124999999437, -41.56249999863440081, 0.000000000000000000 ) ) ;
#25075=CARTESIAN_POINT ( 'NONE',  ( -4.458734124999999437, -88.56249999863439371, 0.000000000000000000 ) ) ;
#25076=CARTESIAN_POINT ( 'NONE',  ( 6.123233995736766282E-16, -120.0000000000000000, -5.000000000000000000 ) ) ;
#25082=CARTESIAN_POINT ( 'NONE',  ( 1.975475456537005874E-15, -65.74999999999998579, 5.000000000000000000 ) ) ;
#25084=CARTESIAN_POINT ( 'NONE',  ( 9.457646018065525792E-16, 2.937500001365594304, 5.148502694627439702 ) ) ;
#25085=CARTESIAN_POINT ( 'NONE',  ( 2.499999999999998668, 6.666666666666667851, -4.330127018922193649 ) ) ;
#25086=CARTESIAN_POINT ( 'NONE',  ( -2.229367062499996610, -19.39583333196774007, 3.861377020970582219 ) ) ;
#25087=CARTESIAN_POINT ( 'NONE',  ( 1.975475456537005874E-15, -100.7499999999999858, 5.000000000000000000 ) ) ;
#25091=CARTESIAN_POINT ( 'NONE',  ( 9.457646018065525792E-16, 19.68750000136559208, 5.148502694627439702 ) ) ;
#25092=ORIENTED_EDGE ( 'NONE', *, *, #38859, .F. ) ;
#25093=CARTESIAN_POINT ( 'NONE',  ( -2.229367062499996610, -97.14583333196773651, 3.861377020970582219 ) ) ;
#25094=CARTESIAN_POINT ( 'NONE',  ( -2.499999999999996447, -18.70833333060214798, 4.330127018922195425 ) ) ;
#25095=CARTESIAN_POINT ( 'NONE',  ( 2.500000000000002220, -57.54166666393548013, 4.330127018922192761 ) ) ;
#25096=CARTESIAN_POINT ( 'NONE',  ( 4.458734125000001214, -14.89583333196773474, 2.574251347313718519 ) ) ;
#25098=CARTESIAN_POINT ( 'NONE',  ( -2.480964764533239819E-13, -72.75000000000000000, 5.000000000000000000 ) ) ;
#25100=CARTESIAN_POINT ( 'NONE',  ( -4.999999999999999112, -41.79166666393548013, 2.886751345948131764 ) ) ;
#25101=CARTESIAN_POINT ( 'NONE',  ( -2.500000000000000444, 20.95833333606451987, -4.330127018922193649 ) ) ;
#25102=CARTESIAN_POINT ( 'NONE',  ( 9.457646018065525792E-16, 13.93750000136559564, 5.148502694627439702 ) ) ;
#25104=CARTESIAN_POINT ( 'NONE',  ( -1.339745962155610925, -47.66965819600734022, 5.000000000000000000 ) ) ;
#25106=CARTESIAN_POINT ( 'NONE',  ( -4.458734124999999437, -60.39583333196773651, -2.574251347313719407 ) ) ;
#25109=CARTESIAN_POINT ( 'NONE',  ( 1.060575238724906964E-15, 6.249999999999998224, 5.773502691896257311 ) ) ;
#25111=CARTESIAN_POINT ( 'NONE',  ( -3.152548672688508926E-16, -51.56249999863441502, -5.148502694627439702 ) ) ;
#25112=CARTESIAN_POINT ( 'NONE',  ( -4.999999999999999112, -91.79166666393547303, 2.886751345948131764 ) ) ;
#25114=CARTESIAN_POINT ( 'NONE',  ( 4.458734124999999437, -33.81249999863440792, -5.460374474430324690E-16 ) ) ;
#25115=DIRECTION ( 'NONE',  ( -0.000000000000000000, 1.000000000000000000, -0.000000000000000000 ) ) ;
#25116=CARTESIAN_POINT ( 'NONE',  ( 2.499999999999998668, 25.79166666939785202, -4.330127018922193649 ) ) ;
#25119=CARTESIAN_POINT ( 'NONE',  ( 5.000000000000000888, -42.58333333333334281, 2.886751345948126879 ) ) ;
#25120=CARTESIAN_POINT ( 'NONE',  ( 5.000000000000000000, -86.29166666393547303, -2.886751345948130876 ) ) ;
#25121=EDGE_LOOP ( 'NONE', ( #42081, #9782, #46831, #56822 ) ) ;
#25122=CARTESIAN_POINT ( 'NONE',  ( 2.229367062500001939, -98.97916666530105090, 3.861377020970579999 ) ) ;
#25123=CARTESIAN_POINT ( 'NONE',  ( 2.229367062499998831, 1.104166668032261711, -3.861377020970580887 ) ) ;
#25124=CARTESIAN_POINT ( 'NONE',  ( 1.975475456537005874E-15, -79.74999999999998579, 5.000000000000000000 ) ) ;
#25129=CARTESIAN_POINT ( 'NONE',  ( -1.339745962155613812, 2.794658198738520394, -5.000000000000000000 ) ) ;
#25137=DIRECTION ( 'NONE',  ( -0.000000000000000000, 1.000000000000000000, -0.000000000000000000 ) ) ;
#25140=CARTESIAN_POINT ( 'NONE',  ( -4.458734124999999437, -25.64583333196773651, -2.574251347313719407 ) ) ;
#25149=DIRECTION ( 'NONE',  ( -0.000000000000000000, -1.000000000000000000, -0.000000000000000000 ) ) ;
#25151=CARTESIAN_POINT ( 'NONE',  ( 4.458734124999999437, -74.06249999863440792, -5.460374474430324690E-16 ) ) ;
#25157=CARTESIAN_POINT ( 'NONE',  ( 4.458734125000001214, -6.145833331967741842, 2.574251347313718519 ) ) ;
#25158=ORIENTED_EDGE ( 'NONE', *, *, #52295, .F. ) ;
#25159=DIRECTION ( 'NONE',  ( 0.000000000000000000, 0.000000000000000000, 1.000000000000000000 ) ) ;
#25167=CARTESIAN_POINT ( 'NONE',  ( -4.458734124999997661, -80.22916666530107932, 2.574251347313722516 ) ) ;
#25169=CARTESIAN_POINT ( 'NONE',  ( -2.229367062499996610, -0.1458333319677394824, 3.861377020970582219 ) ) ;
#25171=CARTESIAN_POINT ( 'NONE',  ( -3.535250795749689387E-16, -85.24999999999998579, -5.773502691896257311 ) ) ;
#25173=CARTESIAN_POINT ( 'NONE',  ( 4.458734125000001214, -67.14583333196773651, 2.574251347313718519 ) ) ;
#25174=CARTESIAN_POINT ( 'NONE',  ( 5.000000000000000888, -25.45833333060214443, 2.886751345948126879 ) ) ;
#25176=CARTESIAN_POINT ( 'NONE',  ( -5.000000000000000000, -0.9583333306021485365, -2.886751345948128211 ) ) ;
#25177=CARTESIAN_POINT ( 'NONE',  ( -1.339745962155610925, -55.79465819873851729, 5.000000000000000000 ) ) ;
#25180=CARTESIAN_POINT ( 'NONE',  ( -3.152548672688508926E-16, -45.56249999863439371, -5.148502694627439702 ) ) ;
#25181=CARTESIAN_POINT ( 'NONE',  ( 4.458734125000000326, -33.14583333196774362, 2.574251347313718519 ) ) ;
#25184=CARTESIAN_POINT ( 'NONE',  ( 5.000000000000000888, 22.41666666666666785, 2.886751345948126879 ) ) ;
#25187=CARTESIAN_POINT ( 'NONE',  ( -2.229367062500000163, -36.47916666530107221, -3.861377020970580443 ) ) ;
#25188=CARTESIAN_POINT ( 'NONE',  ( 5.000000000000000888, -75.45833333060214443, 2.886751345948126879 ) ) ;
#25194=CARTESIAN_POINT ( 'NONE',  ( 4.458734124999998549, -82.97916666530106511, -2.574251347313721627 ) ) ;
#25198=CARTESIAN_POINT ( 'NONE',  ( 5.000000000000000888, 22.54166666939785202, 2.886751345948126879 ) ) ;
#25199=CARTESIAN_POINT ( 'NONE',  ( -2.499999999999996447, -29.83333333333332860, 4.330127018922195425 ) ) ;
#25201=VERTEX_POINT ( 'NONE', #34003 ) ;
#25203=VERTEX_POINT ( 'NONE', #53309 ) ;
#25205=CARTESIAN_POINT ( 'NONE',  ( -2.499999999999996447, 20.29166666939784847, 4.330127018922195425 ) ) ;
#25208=ADVANCED_FACE ( 'NONE', ( #37896 ), #19201, .T. ) ;
#25210=AXIS2_PLACEMENT_3D ( 'NONE', #20903, #54025, #29892 ) ;
#25215=EDGE_CURVE ( 'NONE', #34626, #12016, #58456, .T. ) ;
#25216=CARTESIAN_POINT ( 'NONE',  ( 6.123233995736766282E-16, -120.0000000000000000, -5.000000000000000000 ) ) ;
#25219=CARTESIAN_POINT ( 'NONE',  ( 4.458734124999998549, -23.72916666530107221, -2.574251347313721627 ) ) ;
#25220=CARTESIAN_POINT ( 'NONE',  ( 5.000000000000000000, 17.62500000273118417, -6.123233995736766282E-16 ) ) ;
#25225=ORIENTED_EDGE ( 'NONE', *, *, #39355, .F. ) ;
#25226=CARTESIAN_POINT ( 'NONE',  ( -1.339745962155614700, 25.33034180399266333, 4.999999999999999112 ) ) ;
#25228=ORIENTED_EDGE ( 'NONE', *, *, #20223, .T. ) ;
#25233=( BOUNDED_CURVE ( )  B_SPLINE_CURVE ( 2, ( #3978, #52554, #48339, #58318, #9414, #27780, #8796, #4286, #8486 ),
 .UNSPECIFIED., .F., .F. ) 
 B_SPLINE_CURVE_WITH_KNOTS ( ( 3, 2, 2, 2, 3 ),
 ( 0.09464285714285713969, 0.09523809523809523281, 0.09642857142857143293, 0.09761904761904761918, 0.09821428571428571230 ),
 .UNSPECIFIED. ) 
 CURVE ( )  GEOMETRIC_REPRESENTATION_ITEM ( )  RATIONAL_B_SPLINE_CURVE ( ( 0.9330127018922194093, 0.9330127018922194093, 1.000000000000000000, 0.8660254037844387076, 1.000000000000000000, 0.8660254037844387076, 1.000000000000000000, 0.9330127018922194093, 0.9330127018922194093 ) ) 
 REPRESENTATION_ITEM ( '' )  );
#25237=VERTEX_POINT ( 'NONE', #19522 ) ;
#25238=LINE ( 'NONE', #39067, #14165 ) ;
#25239=CARTESIAN_POINT ( 'NONE',  ( -4.458734124999999437, 13.60416666803226349, -2.574251347313719407 ) ) ;
#25243=DIRECTION ( 'NONE',  ( -0.000000000000000000, 1.000000000000000000, -0.000000000000000000 ) ) ;
#25245=CARTESIAN_POINT ( 'NONE',  ( -2.229367062500000163, -66.47916666530106511, -3.861377020970580443 ) ) ;
#25246=CARTESIAN_POINT ( 'NONE',  ( 0.000000000000000000, -120.0000000000000000, 0.000000000000000000 ) ) ;
#25247=CARTESIAN_POINT ( 'NONE',  ( 4.458734125000001214, 20.10416666803225993, 2.574251347313718519 ) ) ;
#25250=CARTESIAN_POINT ( 'NONE',  ( 2.229367062499998831, -50.89583333196772941, -3.861377020970580887 ) ) ;
#25251=CARTESIAN_POINT ( 'NONE',  ( -5.000000000000000000, -8.874999997268814056, 0.000000000000000000 ) ) ;
#25255=CARTESIAN_POINT ( 'NONE',  ( 2.493747252781420335E-13, -55.24999999999999289, -5.000000000000000000 ) ) ;
#25256=CARTESIAN_POINT ( 'NONE',  ( -4.458734124999999437, -14.64583333196773474, -2.574251347313719407 ) ) ;
#25258=CYLINDRICAL_SURFACE ( 'NONE', #17505, 5.000000000000000000 ) ;
#25259=CARTESIAN_POINT ( 'NONE',  ( -3.152548672688508926E-16, -103.5624999986344221, -5.148502694627439702 ) ) ;
#25261=VERTEX_POINT ( 'NONE', #58763 ) ;
#25262=CARTESIAN_POINT ( 'NONE',  ( 9.457646018065525792E-16, -98.31249999863440792, 5.148502694627439702 ) ) ;
#25264=CARTESIAN_POINT ( 'NONE',  ( -4.999999999999999112, -55.79166666393548013, 2.886751345948131764 ) ) ;
#25269=CARTESIAN_POINT ( 'NONE',  ( -2.229367062499996610, -19.14583333196774007, 3.861377020970582219 ) ) ;
#25270=CARTESIAN_POINT ( 'NONE',  ( 4.458734124999999437, 7.937500001365595637, -5.460374474430324690E-16 ) ) ;
#25271=CARTESIAN_POINT ( 'NONE',  ( 9.457646018065525792E-16, -62.31249999863440792, 5.148502694627439702 ) ) ;
#25272=CARTESIAN_POINT ( 'NONE',  ( 5.000000000000000000, -94.37499999726881583, -6.123233995736766282E-16 ) ) ;
#25274=LINE ( 'NONE', #55519, #56824 ) ;
#25276=CARTESIAN_POINT ( 'NONE',  ( -4.999999999999999112, -8.916666666666664298, 2.886751345948131764 ) ) ;
#25278=ORIENTED_EDGE ( 'NONE', *, *, #41458, .F. ) ;
#25284=LINE ( 'NONE', #33983, #42093 ) ;
#25285=CARTESIAN_POINT ( 'NONE',  ( 1.975475456537005874E-15, -64.74999999999998579, 5.000000000000000000 ) ) ;
#25286=DIRECTION ( 'NONE',  ( -0.000000000000000000, 1.000000000000000000, -0.000000000000000000 ) ) ;
#25288=CARTESIAN_POINT ( 'NONE',  ( -4.999999999999999112, -75.91666666666667140, 2.886751345948131764 ) ) ;
#25292=ORIENTED_EDGE ( 'NONE', *, *, #42145, .F. ) ;
#25294=CARTESIAN_POINT ( 'NONE',  ( -1.339745962155610925, -50.79465819873851018, 5.000000000000000000 ) ) ;
#25304=ORIENTED_EDGE ( 'NONE', *, *, #20141, .T. ) ;
#25307=CARTESIAN_POINT ( 'NONE',  ( -2.229367062500000163, -60.72916666530106511, -3.861377020970580443 ) ) ;
#25309=CARTESIAN_POINT ( 'NONE',  ( 1.339745962155612702, 3.830341803992665550, -5.000000000000000000 ) ) ;
#25313=CARTESIAN_POINT ( 'NONE',  ( -1.339745962155613812, -84.20534180126149693, -5.000000000000000000 ) ) ;
#25314=ORIENTED_EDGE ( 'NONE', *, *, #57883, .T. ) ;
#25315=( BOUNDED_CURVE ( )  B_SPLINE_CURVE ( 2, ( #33985, #48765, #24652, #44258, #19820, #5675, #45860, #6319, #20791 ),
 .UNSPECIFIED., .F., .F. ) 
 B_SPLINE_CURVE_WITH_KNOTS ( ( 3, 2, 2, 2, 3 ),
 ( 0.05892857142857142738, 0.05952380952380952051, 0.06071428571428571369, 0.06190476190476190688, 0.06250000000000000000 ),
 .UNSPECIFIED. ) 
 CURVE ( )  GEOMETRIC_REPRESENTATION_ITEM ( )  RATIONAL_B_SPLINE_CURVE ( ( 0.9330127018922194093, 0.9330127018922194093, 1.000000000000000000, 0.8660254037844387076, 1.000000000000000000, 0.8660254037844387076, 1.000000000000000000, 0.9330127018922194093, 0.9330127018922194093 ) ) 
 REPRESENTATION_ITEM ( '' )  );
#25317=CARTESIAN_POINT ( 'NONE',  ( 2.229367062500001939, 28.02083333469892779, 3.861377020970579999 ) ) ;
#25319=VERTEX_POINT ( 'NONE', #15041 ) ;
#25323=CARTESIAN_POINT ( 'NONE',  ( 2.229367062500001939, -41.97916666530107932, 3.861377020970579999 ) ) ;
#25326=CARTESIAN_POINT ( 'NONE',  ( -4.458734124999999437, -48.39583333196772941, -2.574251347313719407 ) ) ;
#25327=CARTESIAN_POINT ( 'NONE',  ( -4.458734124999998549, -16.22916666530107577, 2.574251347313722516 ) ) ;
#25328=CARTESIAN_POINT ( 'NONE',  ( 2.500000000000002220, -102.6666666666666572, 4.330127018922192761 ) ) ;
#25329=( BOUNDED_CURVE ( )  B_SPLINE_CURVE ( 2, ( #14326, #38760, #13074, #52630, #52325, #8259, #13391, #53569, #28491 ),
 .UNSPECIFIED., .F., .F. ) 
 B_SPLINE_CURVE_WITH_KNOTS ( ( 3, 2, 2, 2, 3 ),
 ( 0.5267857142857143016, 0.5273809523809523947, 0.5285714285714285809, 0.5297619047619047672, 0.5303571428571428603 ),
 .UNSPECIFIED. ) 
 CURVE ( )  GEOMETRIC_REPRESENTATION_ITEM ( )  RATIONAL_B_SPLINE_CURVE ( ( 0.9330127018922194093, 0.9330127018922194093, 1.000000000000000000, 0.8660254037844387076, 1.000000000000000000, 0.8660254037844387076, 1.000000000000000000, 0.9330127018922194093, 0.9330127018922194093 ) ) 
 REPRESENTATION_ITEM ( '' )  );
#25331=CARTESIAN_POINT ( 'NONE',  ( -2.229367062500000163, -32.72916666530106511, -3.861377020970580443 ) ) ;
#25332=CARTESIAN_POINT ( 'NONE',  ( 5.000000000000000888, 8.541666669397853795, 2.886751345948126879 ) ) ;
#25333=DIRECTION ( 'NONE',  ( -0.000000000000000000, 1.000000000000000000, -0.000000000000000000 ) ) ;
#25338=CARTESIAN_POINT ( 'NONE',  ( -4.458734124999999437, -2.562499998634407028, 0.000000000000000000 ) ) ;
#25342=CARTESIAN_POINT ( 'NONE',  ( 2.229367062499998831, -86.64583333196773651, -3.861377020970580887 ) ) ;
#25343=CARTESIAN_POINT ( 'NONE',  ( 4.458734124999998549, -33.72916666530106511, -2.574251347313721627 ) ) ;
#25344=CARTESIAN_POINT ( 'NONE',  ( 5.000000000000000000, -95.50000000000000000, -6.123233995736766282E-16 ) ) ;
#25345=CARTESIAN_POINT ( 'NONE',  ( 2.229367062499998831, -80.89583333196773651, -3.861377020970580887 ) ) ;
#25346=VECTOR ( 'NONE', #54858, 1000.000000000000000 ) ;
#25348=CYLINDRICAL_SURFACE ( 'NONE', #31490, 5.000000000000000000 ) ;
#25349=VECTOR ( 'NONE', #46146, 1000.000000000000000 ) ;
#25353=CARTESIAN_POINT ( 'NONE',  ( 4.458734125000000326, -2.895833331967738289, 2.574251347313718519 ) ) ;
#25354=CARTESIAN_POINT ( 'NONE',  ( -2.229367062500000163, 20.27083333469892779, -3.861377020970580443 ) ) ;
#25355=CARTESIAN_POINT ( 'NONE',  ( -4.458734124999997661, -48.47916666530106511, 2.574251347313722516 ) ) ;
#25356=CARTESIAN_POINT ( 'NONE',  ( 1.975475456537005874E-15, -15.75000000000000000, 5.000000000000000000 ) ) ;
#25358=ORIENTED_EDGE ( 'NONE', *, *, #29978, .F. ) ;
#25361=CARTESIAN_POINT ( 'NONE',  ( -3.152548672688508926E-16, -74.56249999863440792, -5.148502694627439702 ) ) ;
#25362=CARTESIAN_POINT ( 'NONE',  ( -3.535250795749689387E-16, -108.1249999972688016, -5.773502691896257311 ) ) ;
#25365=CARTESIAN_POINT ( 'NONE',  ( 4.458734125000000326, -109.1458333319677365, 2.574251347313718519 ) ) ;
#25367=CARTESIAN_POINT ( 'NONE',  ( 2.500000000000002220, -58.66666666666665719, 4.330127018922192761 ) ) ;
#25371=CARTESIAN_POINT ( 'NONE',  ( -5.000000000000000000, -72.95833333060214443, -2.886751345948128211 ) ) ;
#25372=CARTESIAN_POINT ( 'NONE',  ( -5.000000000000000000, -99.00000000000000000, 0.000000000000000000 ) ) ;
#25378=VERTEX_POINT ( 'NONE', #29823 ) ;
#25380=CARTESIAN_POINT ( 'NONE',  ( -2.500000000000000444, 10.95833333606451632, -4.330127018922193649 ) ) ;
#25386=CARTESIAN_POINT ( 'NONE',  ( 2.229367062499998831, -48.89583333196772941, -3.861377020970580887 ) ) ;
#25393=AXIS2_PLACEMENT_3D ( 'NONE', #2337, #55410, #16161 ) ;
#25398=CARTESIAN_POINT ( 'NONE',  ( -2.229367062499996610, -94.39583333196773651, 3.861377020970582219 ) ) ;
#25401=CARTESIAN_POINT ( 'NONE',  ( -1.230605004983934782E-13, -37.62499999726881583, 5.000000000000000000 ) ) ;
#25406=CARTESIAN_POINT ( 'NONE',  ( -4.458734124999998549, 5.770833334698927786, 2.574251347313722516 ) ) ;
#25407=CARTESIAN_POINT ( 'NONE',  ( 2.499999999999998668, -50.20833333060213732, -4.330127018922193649 ) ) ;
#25408=CARTESIAN_POINT ( 'NONE',  ( -4.458734124999998549, -18.47916666530106866, 2.574251347313722516 ) ) ;
#25410=CARTESIAN_POINT ( 'NONE',  ( 1.339745962155615144, -77.58034179853028434, 4.999999999999999112 ) ) ;
#25413=CARTESIAN_POINT ( 'NONE',  ( -2.229367062500000163, 18.27083333469892779, -3.861377020970580443 ) ) ;
#25416=CARTESIAN_POINT ( 'NONE',  ( 5.000000000000000888, -71.45833333060214443, 2.886751345948126879 ) ) ;
#25417=CARTESIAN_POINT ( 'NONE',  ( 9.457646018065525792E-16, -21.06249999863440436, 5.148502694627439702 ) ) ;
#25421=CARTESIAN_POINT ( 'NONE',  ( 2.500000000000002220, -45.54166666393547303, 4.330127018922192761 ) ) ;
#25422=CARTESIAN_POINT ( 'NONE',  ( 5.000000000000000000, -67.29166666393547303, -2.886751345948130876 ) ) ;
#25423=CARTESIAN_POINT ( 'NONE',  ( -2.229367062500000163, 14.52083333469892779, -3.861377020970580443 ) ) ;
#25424=CYLINDRICAL_SURFACE ( 'NONE', #36599, 5.000000000000000000 ) ;
#25425=ORIENTED_EDGE ( 'NONE', *, *, #9724, .T. ) ;
#25427=CARTESIAN_POINT ( 'NONE',  ( -4.458734124999999437, -62.31249999863440792, 0.000000000000000000 ) ) ;
#25428=ORIENTED_EDGE ( 'NONE', *, *, #19764, .F. ) ;
#25430=VECTOR ( 'NONE', #14949, 1000.000000000000000 ) ;
#25431=CARTESIAN_POINT ( 'NONE',  ( 2.500000000000002220, 5.333333333333332149, 4.330127018922192761 ) ) ;
#25433=CARTESIAN_POINT ( 'NONE',  ( -5.926426369611017623E-15, 26.37500000273118417, 5.000000000000000000 ) ) ;
#25434=CARTESIAN_POINT ( 'NONE',  ( 4.458734125000001214, -58.89583333196773651, 2.574251347313718519 ) ) ;
#25435=CARTESIAN_POINT ( 'NONE',  ( -3.535250795749689387E-16, -88.12499999726878741, -5.773502691896257311 ) ) ;
#25436=CARTESIAN_POINT ( 'NONE',  ( 4.458734124999998549, -33.72916666530107221, -2.574251347313721627 ) ) ;
#25437=CARTESIAN_POINT ( 'NONE',  ( 1.339745962155615144, -8.705341801261482715, 4.999999999999999112 ) ) ;
#25439=CARTESIAN_POINT ( 'NONE',  ( 2.499999999999998668, -16.20833333060214443, -4.330127018922193649 ) ) ;
#25441=CARTESIAN_POINT ( 'NONE',  ( 1.060575238724906964E-15, -43.75000000000000000, 5.773502691896257311 ) ) ;
#25442=DIRECTION ( 'NONE',  ( -0.000000000000000000, 1.000000000000000000, -0.000000000000000000 ) ) ;
#25443=CARTESIAN_POINT ( 'NONE',  ( 5.000000000000000000, -17.37499999726881583, -6.123233995736766282E-16 ) ) ;
#25444=ORIENTED_EDGE ( 'NONE', *, *, #19251, .T. ) ;
#25445=CARTESIAN_POINT ( 'NONE',  ( 2.229367062499998831, -106.6458333319677365, -3.861377020970580887 ) ) ;
#25446=CARTESIAN_POINT ( 'NONE',  ( -3.152548672688508926E-16, 4.187500001365595637, -5.148502694627439702 ) ) ;
#25455=CARTESIAN_POINT ( 'NONE',  ( 1.339745962155612702, -22.16965819600733312, -5.000000000000000000 ) ) ;
#25457=CARTESIAN_POINT ( 'NONE',  ( -4.999999999999998224, -48.79166666393547303, 2.886751345948131764 ) ) ;
#25459=CARTESIAN_POINT ( 'NONE',  ( -4.458734124999998549, -28.47916666530107221, 2.574251347313722516 ) ) ;
#25468=ORIENTED_EDGE ( 'NONE', *, *, #47134, .F. ) ;
#25469=CARTESIAN_POINT ( 'NONE',  ( -4.458734124999998549, -72.47916666530107932, 2.574251347313722516 ) ) ;
#25471=ORIENTED_EDGE ( 'NONE', *, *, #20421, .F. ) ;
#25476=VECTOR ( 'NONE', #60820, 1000.000000000000000 ) ;
#25477=CARTESIAN_POINT ( 'NONE',  ( -2.229367062499996610, -1.395833331967737179, 3.861377020970582219 ) ) ;
#25478=ORIENTED_EDGE ( 'NONE', *, *, #10882, .F. ) ;
#25479=CARTESIAN_POINT ( 'NONE',  ( 3.044556291839386294E-14, 17.75000000000000000, -5.000000000000000000 ) ) ;
#25485=CARTESIAN_POINT ( 'NONE',  ( 5.000000000000000000, -75.29166666393548724, -2.886751345948130876 ) ) ;
#25486=ORIENTED_EDGE ( 'NONE', *, *, #46381, .F. ) ;
#25487=CARTESIAN_POINT ( 'NONE',  ( -3.152548672688508926E-16, -81.56249999863440792, -5.148502694627439702 ) ) ;
#25488=CARTESIAN_POINT ( 'NONE',  ( 1.975475456537005874E-15, -75.74999999999998579, 5.000000000000000000 ) ) ;
#25489=CARTESIAN_POINT ( 'NONE',  ( 4.458734125000001214, -4.895833331967740065, 2.574251347313718519 ) ) ;
#25494=CARTESIAN_POINT ( 'NONE',  ( 2.229367062500001939, -71.22916666530107932, 3.861377020970579999 ) ) ;
#25495=CARTESIAN_POINT ( 'NONE',  ( -3.535250795749689387E-16, -26.12499999726881583, -5.773502691896257311 ) ) ;
#25497=CARTESIAN_POINT ( 'NONE',  ( -1.339745962155610925, -14.79465819873851729, 5.000000000000000000 ) ) ;
#25498=CARTESIAN_POINT ( 'NONE',  ( -4.458734124999999437, 28.60416666803226349, -2.574251347313719407 ) ) ;
#25500=CARTESIAN_POINT ( 'NONE',  ( 4.458734124999998549, -47.72916666530106511, -2.574251347313721627 ) ) ;
#25501=CARTESIAN_POINT ( 'NONE',  ( -4.458734124999999437, -30.64583333196774007, -2.574251347313719407 ) ) ;
#25504=CARTESIAN_POINT ( 'NONE',  ( 2.499999999999998668, 22.66666666666666430, -4.330127018922193649 ) ) ;
#25506=CARTESIAN_POINT ( 'NONE',  ( 6.158835246850666199E-14, 7.875000002731183280, -4.999999999999999112 ) ) ;
#25507=CARTESIAN_POINT ( 'NONE',  ( -3.152548672688508926E-16, -42.56249999863440792, -5.148502694627439702 ) ) ;
#25508=CARTESIAN_POINT ( 'NONE',  ( -2.499999999999996447, -75.70833333060214443, 4.330127018922195425 ) ) ;
#25511=( BOUNDED_CURVE ( )  B_SPLINE_CURVE ( 2, ( #54382, #29597, #39248, #25422, #6456, #45041, #1008, #24787, #19638 ),
 .UNSPECIFIED., .F., .F. ) 
 B_SPLINE_CURVE_WITH_KNOTS ( ( 3, 2, 2, 2, 3 ),
 ( 0.6875000000000000000, 0.6880952380952380931, 0.6892857142857142794, 0.6904761904761904656, 0.6910714285714285587 ),
 .UNSPECIFIED. ) 
 CURVE ( )  GEOMETRIC_REPRESENTATION_ITEM ( )  RATIONAL_B_SPLINE_CURVE ( ( 0.9330127018922194093, 0.9330127018922194093, 1.000000000000000000, 0.8660254037844387076, 1.000000000000000000, 0.8660254037844387076, 1.000000000000000000, 0.9330127018922194093, 0.9330127018922194093 ) ) 
 REPRESENTATION_ITEM ( '' )  );
#25514=CARTESIAN_POINT ( 'NONE',  ( 2.229367062499998831, -77.89583333196773651, -3.861377020970580887 ) ) ;
#25516=LINE ( 'NONE', #45134, #19380 ) ;
#25517=CARTESIAN_POINT ( 'NONE',  ( 5.000000000000000888, 13.54166666939785202, 2.886751345948126879 ) ) ;
#25518=CARTESIAN_POINT ( 'NONE',  ( -5.000000000000000000, -30.08333333333333215, -2.886751345948128211 ) ) ;
#25525=CARTESIAN_POINT ( 'NONE',  ( 5.000000000000000000, 21.70833333606451987, -2.886751345948129988 ) ) ;
#25534=CARTESIAN_POINT ( 'NONE',  ( -4.999999999999998224, -74.79166666393547303, 2.886751345948131764 ) ) ;
#25537=CARTESIAN_POINT ( 'NONE',  ( 2.229367062500001939, -12.22916666530107044, 3.861377020970579999 ) ) ;
#25542=ORIENTED_EDGE ( 'NONE', *, *, #10174, .F. ) ;
#25547=CARTESIAN_POINT ( 'NONE',  ( 5.000000000000000000, -9.291666663935483683, -2.886751345948130876 ) ) ;
#25549=ORIENTED_EDGE ( 'NONE', *, *, #18788, .F. ) ;
#25550=CARTESIAN_POINT ( 'NONE',  ( 2.499999999999998668, -99.33333333333332860, -4.330127018922193649 ) ) ;
#25552=DIRECTION ( 'NONE',  ( -0.000000000000000000, 1.000000000000000000, -0.000000000000000000 ) ) ;
#25554=EDGE_CURVE ( 'NONE', #42628, #42363, #31414, .T. ) ;
#25555=ORIENTED_EDGE ( 'NONE', *, *, #58971, .T. ) ;
#25559=CARTESIAN_POINT ( 'NONE',  ( 9.457646018065525792E-16, 12.93750000136559386, 5.148502694627439702 ) ) ;
#25563=CARTESIAN_POINT ( 'NONE',  ( 1.975475456537005874E-15, -17.75000000000000355, 5.000000000000000000 ) ) ;
#25564=CARTESIAN_POINT ( 'NONE',  ( 1.339745962155612702, -25.29465819873852439, -5.000000000000000000 ) ) ;
#25565=( BOUNDED_CURVE ( )  B_SPLINE_CURVE ( 2, ( #38421, #29711, #9775, #58047, #24585, #13977, #38728, #4638, #49342 ),
 .UNSPECIFIED., .F., .F. ) 
 B_SPLINE_CURVE_WITH_KNOTS ( ( 3, 2, 2, 2, 3 ),
 ( 0.9017857142857143016, 0.9023809523809523947, 0.9035714285714285809, 0.9047619047619047672, 0.9053571428571428603 ),
 .UNSPECIFIED. ) 
 CURVE ( )  GEOMETRIC_REPRESENTATION_ITEM ( )  RATIONAL_B_SPLINE_CURVE ( ( 0.9330127018922194093, 0.9330127018922194093, 1.000000000000000000, 0.8660254037844387076, 1.000000000000000000, 0.8660254037844387076, 1.000000000000000000, 0.9330127018922194093, 0.9330127018922194093 ) ) 
 REPRESENTATION_ITEM ( '' )  );
#25566=CYLINDRICAL_SURFACE ( 'NONE', #3506, 5.000000000000000000 ) ;
#25567=CARTESIAN_POINT ( 'NONE',  ( -3.152548672688508926E-16, -63.56249999863440792, -5.148502694627439702 ) ) ;
#25568=LINE ( 'NONE', #60317, #45871 ) ;
#25569=CARTESIAN_POINT ( 'NONE',  ( 4.458734124999998549, 19.27083333469893134, -2.574251347313721627 ) ) ;
#25570=AXIS2_PLACEMENT_3D ( 'NONE', #36960, #12510, #51757 ) ;
#25572=CARTESIAN_POINT ( 'NONE',  ( -6.972266317189433020E-16, -31.12499999726880873, -5.000000000000000000 ) ) ;
#25573=CARTESIAN_POINT ( 'NONE',  ( 2.229367062500001939, -49.22916666530107221, 3.861377020970579999 ) ) ;
#25574=CARTESIAN_POINT ( 'NONE',  ( 2.500000000000002220, -9.541666663935483683, 4.330127018922192761 ) ) ;
#25575=CARTESIAN_POINT ( 'NONE',  ( 1.339745962155615144, -25.58034179853029144, 4.999999999999999112 ) ) ;
#25577=CARTESIAN_POINT ( 'NONE',  ( -1.339745962155610925, -65.66965819600733312, 5.000000000000000000 ) ) ;
#25580=CARTESIAN_POINT ( 'NONE',  ( -3.152548672688508926E-16, -17.81249999863440792, -5.148502694627439702 ) ) ;
#25581=ORIENTED_EDGE ( 'NONE', *, *, #59025, .F. ) ;
#25583=CARTESIAN_POINT ( 'NONE',  ( 4.458734124999998549, -104.7291666653010509, -2.574251347313721627 ) ) ;
#25586=CARTESIAN_POINT ( 'NONE',  ( -4.458734124999999437, -98.64583333196773651, -2.574251347313719407 ) ) ;
#25587=CARTESIAN_POINT ( 'NONE',  ( 1.243387493232115550E-13, -8.250000000000003553, -5.000000000000000000 ) ) ;
#25588=CARTESIAN_POINT ( 'NONE',  ( -2.500000000000000444, -55.04166666393548013, -4.330127018922193649 ) ) ;
#25592=CARTESIAN_POINT ( 'NONE',  ( -3.152548672688508926E-16, -24.56249999863440792, -5.148502694627439702 ) ) ;
#25593=CARTESIAN_POINT ( 'NONE',  ( 4.458734125000001214, 5.854166668032262599, 2.574251347313718519 ) ) ;
#25595=CARTESIAN_POINT ( 'NONE',  ( -4.458734124999999437, -66.64583333196773651, -2.574251347313719407 ) ) ;
#25600=CARTESIAN_POINT ( 'NONE',  ( 1.060575238724906964E-15, -13.75000000000000000, 5.773502691896257311 ) ) ;
#25608=CARTESIAN_POINT ( 'NONE',  ( 1.339745962155615144, -93.70534180126149693, 4.999999999999999112 ) ) ;
#25612=CARTESIAN_POINT ( 'NONE',  ( -5.000000000000000000, -73.00000000000000000, 0.000000000000000000 ) ) ;
#25615=CARTESIAN_POINT ( 'NONE',  ( -6.972266317189433020E-16, -98.24999999999998579, -5.000000000000000000 ) ) ;
#25616=ORIENTED_EDGE ( 'NONE', *, *, #20817, .T. ) ;
#25618=( BOUNDED_CURVE ( )  B_SPLINE_CURVE ( 2, ( #32647, #61299, #17221, #17855, #31698, #2139, #51959, #61936, #1817 ),
 .UNSPECIFIED., .F., .F. ) 
 B_SPLINE_CURVE_WITH_KNOTS ( ( 3, 2, 2, 2, 3 ),
 ( 0.8089285714285714413, 0.8095238095238095344, 0.8107142857142857206, 0.8119047619047619069, 0.8125000000000000000 ),
 .UNSPECIFIED. ) 
 CURVE ( )  GEOMETRIC_REPRESENTATION_ITEM ( )  RATIONAL_B_SPLINE_CURVE ( ( 0.9330127018922194093, 0.9330127018922194093, 1.000000000000000000, 0.8660254037844387076, 1.000000000000000000, 0.8660254037844387076, 1.000000000000000000, 0.9330127018922194093, 0.9330127018922194093 ) ) 
 REPRESENTATION_ITEM ( '' )  );
#25621=AXIS2_PLACEMENT_3D ( 'NONE', #32961, #8830, #33275 ) ;
#25623=ORIENTED_EDGE ( 'NONE', *, *, #48453, .F. ) ;
#25630=VERTEX_POINT ( 'NONE', #41068 ) ;
#25634=EDGE_CURVE ( 'NONE', #18331, #22810, #46860, .T. ) ;
#25637=CARTESIAN_POINT ( 'NONE',  ( -3.152548672688508926E-16, 27.43750000136559564, -5.148502694627439702 ) ) ;
#25639=ORIENTED_EDGE ( 'NONE', *, *, #43115, .F. ) ;
#25644=CARTESIAN_POINT ( 'NONE',  ( -4.458734124999999437, -43.39583333196773651, -2.574251347313719407 ) ) ;
#25648=CARTESIAN_POINT ( 'NONE',  ( -3.152548672688508926E-16, -50.56249999863440792, -5.148502694627439702 ) ) ;
#25650=EDGE_CURVE ( 'NONE', #11315, #35606, #25329, .T. ) ;
#25651=CARTESIAN_POINT ( 'NONE',  ( 4.458734124999999437, -16.81249999863440436, -5.460374474430324690E-16 ) ) ;
#25653=CARTESIAN_POINT ( 'NONE',  ( -3.535250795749689387E-16, -100.2500000000000142, -5.773502691896257311 ) ) ;
#25655=CARTESIAN_POINT ( 'NONE',  ( 9.457646018065525792E-16, -35.31249999863440792, 5.148502694627439702 ) ) ;
#25656=CARTESIAN_POINT ( 'NONE',  ( -2.499999999999996447, 4.291666669397852907, 4.330127018922195425 ) ) ;
#25664=CARTESIAN_POINT ( 'NONE',  ( 2.229367062499998831, -1.895833331967737623, -3.861377020970580887 ) ) ;
#25665=VERTEX_POINT ( 'NONE', #62611 ) ;
#25669=CARTESIAN_POINT ( 'NONE',  ( -2.229367062500000163, -86.47916666530107932, -3.861377020970580443 ) ) ;
#25670=CARTESIAN_POINT ( 'NONE',  ( -4.458734124999999437, -34.31249999863440792, 0.000000000000000000 ) ) ;
#25671=CARTESIAN_POINT ( 'NONE',  ( 2.500000000000002220, -9.666666666666664298, 4.330127018922192761 ) ) ;
#25672=CARTESIAN_POINT ( 'NONE',  ( -4.458734124999999437, -83.56249999863439371, 0.000000000000000000 ) ) ;
#25673=VECTOR ( 'NONE', #42684, 1000.000000000000000 ) ;
#25675=CARTESIAN_POINT ( 'NONE',  ( -6.972266317189433020E-16, -30.12499999726880873, -5.000000000000000000 ) ) ;
#25678=CARTESIAN_POINT ( 'NONE',  ( -4.458734124999999437, -6.395833331967741842, -2.574251347313719407 ) ) ;
#25679=CARTESIAN_POINT ( 'NONE',  ( 2.229367062500001939, 22.77083333469892423, 3.861377020970579999 ) ) ;
#25680=CARTESIAN_POINT ( 'NONE',  ( -2.229367062499996610, -48.39583333196772941, 3.861377020970582219 ) ) ;
#25681=CARTESIAN_POINT ( 'NONE',  ( 2.500000000000002220, -105.6666666666666572, 4.330127018922192761 ) ) ;
#25684=VERTEX_POINT ( 'NONE', #29104 ) ;
#25687=CARTESIAN_POINT ( 'NONE',  ( 9.457646018065525792E-16, -77.06249999863440792, 5.148502694627439702 ) ) ;
#25688=CARTESIAN_POINT ( 'NONE',  ( 2.500000000000002220, -110.5416666639354730, 4.330127018922192761 ) ) ;
#25692=CARTESIAN_POINT ( 'NONE',  ( 5.000000000000000000, -57.41666666666667140, -2.886751345948129988 ) ) ;
#25693=CARTESIAN_POINT ( 'NONE',  ( 2.499999999999998668, -36.20833333060213732, -4.330127018922193649 ) ) ;
#25697=CARTESIAN_POINT ( 'NONE',  ( 1.339745962155612702, -52.16965819600733312, -5.000000000000000000 ) ) ;
#25702=( BOUNDED_CURVE ( )  B_SPLINE_CURVE ( 2, ( #9770, #53842, #15575, #63196, #24901, #10099, #15245, #10419, #49010 ),
 .UNSPECIFIED., .F., .F. ) 
 B_SPLINE_CURVE_WITH_KNOTS ( ( 3, 2, 2, 2, 3 ),
 ( 0.8589285714285714857, 0.8595238095238095788, 0.8607142857142857650, 0.8619047619047619513, 0.8625000000000000444 ),
 .UNSPECIFIED. ) 
 CURVE ( )  GEOMETRIC_REPRESENTATION_ITEM ( )  RATIONAL_B_SPLINE_CURVE ( ( 0.9330127018922194093, 0.9330127018922256266, 1.000000000000000000, 0.8660254037844387076, 1.000000000000000000, 0.8660254037844387076, 1.000000000000000000, 0.9330127018922194093, 0.9330127018922194093 ) ) 
 REPRESENTATION_ITEM ( '' )  );
#25705=ORIENTED_EDGE ( 'NONE', *, *, #5596, .F. ) ;
#25709=ORIENTED_EDGE ( 'NONE', *, *, #4707, .T. ) ;
#25714=CARTESIAN_POINT ( 'NONE',  ( -4.458734124999999437, -44.56249999863440081, 0.000000000000000000 ) ) ;
#25718=VECTOR ( 'NONE', #27351, 1000.000000000000000 ) ;
#25724=CARTESIAN_POINT ( 'NONE',  ( 4.458734124999999437, -96.06249999863440792, -5.460374474430324690E-16 ) ) ;
#25726=ORIENTED_EDGE ( 'NONE', *, *, #48430, .F. ) ;
#25727=CYLINDRICAL_SURFACE ( 'NONE', #25210, 5.000000000000000000 ) ;
#25731=ORIENTED_EDGE ( 'NONE', *, *, #38859, .T. ) ;
#25732=CARTESIAN_POINT ( 'NONE',  ( -4.458734124999999437, -3.395833331967739177, -2.574251347313719407 ) ) ;
#25733=CARTESIAN_POINT ( 'NONE',  ( 1.975475456537005874E-15, -106.7499999999999858, 5.000000000000000000 ) ) ;
#25734=CARTESIAN_POINT ( 'NONE',  ( -4.458734124999999437, -19.56249999863440081, 0.000000000000000000 ) ) ;
#25735=CYLINDRICAL_SURFACE ( 'NONE', #7604, 5.000000000000000000 ) ;
#25739=CARTESIAN_POINT ( 'NONE',  ( -3.152548672688508926E-16, 13.18750000136559208, -5.148502694627439702 ) ) ;
#25742=CARTESIAN_POINT ( 'NONE',  ( -2.499999999999996447, -12.83333333333333570, 4.330127018922195425 ) ) ;
#25743=CARTESIAN_POINT ( 'NONE',  ( 4.458734124999998549, -17.72916666530106866, -2.574251347313721627 ) ) ;
#25747=CARTESIAN_POINT ( 'NONE',  ( -5.000000000000000000, -48.95833333060213732, -2.886751345948128211 ) ) ;
#25749=CARTESIAN_POINT ( 'NONE',  ( 2.229367062500001939, 14.02083333469892779, 3.861377020970579999 ) ) ;
#25750=CARTESIAN_POINT ( 'NONE',  ( 0.000000000000000000, -120.0000000000000000, 0.000000000000000000 ) ) ;
#25753=CARTESIAN_POINT ( 'NONE',  ( -4.458734124999998549, -65.22916666530106511, 2.574251347313722516 ) ) ;
#25754=ORIENTED_EDGE ( 'NONE', *, *, #55138, .T. ) ;
#25757=CARTESIAN_POINT ( 'NONE',  ( 5.000000000000000000, 6.583333333333333037, -2.886751345948129988 ) ) ;
#25759=CARTESIAN_POINT ( 'NONE',  ( -6.972266317189433020E-16, 21.75000000000000000, -5.000000000000000000 ) ) ;
#25760=VECTOR ( 'NONE', #29224, 1000.000000000000000 ) ;
#25761=CARTESIAN_POINT ( 'NONE',  ( -4.458734124999998549, -57.22916666530107932, 2.574251347313722516 ) ) ;
#25762=CARTESIAN_POINT ( 'NONE',  ( 1.060575238724906964E-15, -95.62499999726881583, 5.773502691896257311 ) ) ;
#25763=CARTESIAN_POINT ( 'NONE',  ( -4.458734124999999437, -33.39583333196772941, -2.574251347313719407 ) ) ;
#25764=CARTESIAN_POINT ( 'NONE',  ( -5.000000000000000000, -41.95833333060214443, -2.886751345948128211 ) ) ;
#25769=CARTESIAN_POINT ( 'NONE',  ( -5.000000000000000000, -42.08333333333333570, -2.886751345948128211 ) ) ;
#25772=ORIENTED_EDGE ( 'NONE', *, *, #38200, .T. ) ;
#25773=CARTESIAN_POINT ( 'NONE',  ( -4.458734124999999437, -106.3124999986343937, 0.000000000000000000 ) ) ;
#25774=CARTESIAN_POINT ( 'NONE',  ( 4.458734124999998549, 3.020833334698928674, -2.574251347313721627 ) ) ;
#25775=( BOUNDED_CURVE ( )  B_SPLINE_CURVE ( 2, ( #34070, #9625, #29233, #19908, #39841, #59484, #310, #24426, #39207 ),
 .UNSPECIFIED., .F., .F. ) 
 B_SPLINE_CURVE_WITH_KNOTS ( ( 3, 2, 2, 2, 3 ),
 ( 0.3839285714285714524, 0.3845238095238095455, 0.3857142857142857317, 0.3869047619047619180, 0.3875000000000000111 ),
 .UNSPECIFIED. ) 
 CURVE ( )  GEOMETRIC_REPRESENTATION_ITEM ( )  RATIONAL_B_SPLINE_CURVE ( ( 0.9330127018922194093, 0.9330127018922194093, 1.000000000000000000, 0.8660254037844387076, 1.000000000000000000, 0.8660254037844387076, 1.000000000000000000, 0.9330127018922194093, 0.9330127018922194093 ) ) 
 REPRESENTATION_ITEM ( '' )  );
#25776=CARTESIAN_POINT ( 'NONE',  ( -2.500000000000000444, -97.04166666393545881, -4.330127018922193649 ) ) ;
#25789=CARTESIAN_POINT ( 'NONE',  ( -4.458734124999999437, -32.64583333196774362, -2.574251347313719407 ) ) ;
#25790=DIRECTION ( 'NONE',  ( -0.000000000000000000, 1.000000000000000000, -0.000000000000000000 ) ) ;
#25797=CARTESIAN_POINT ( 'NONE',  ( -4.999999999999998224, -82.79166666393547303, 2.886751345948131764 ) ) ;
#25799=CARTESIAN_POINT ( 'NONE',  ( 9.457646018065525792E-16, -78.31249999863442213, 5.148502694627439702 ) ) ;
#25801=CARTESIAN_POINT ( 'NONE',  ( -1.339745962155613812, -15.08034179853029322, -5.000000000000000000 ) ) ;
#25805=CARTESIAN_POINT ( 'NONE',  ( -4.458734124999998549, -3.479166665301069994, 2.574251347313722516 ) ) ;
#25806=ORIENTED_EDGE ( 'NONE', *, *, #58253, .T. ) ;
#25814=VERTEX_POINT ( 'NONE', #37841 ) ;
#25815=CARTESIAN_POINT ( 'NONE',  ( 2.229367062499998831, -79.64583333196773651, -3.861377020970580887 ) ) ;
#25816=CARTESIAN_POINT ( 'NONE',  ( -4.999999999999998224, -96.91666666666665719, 2.886751345948131764 ) ) ;
#25817=CARTESIAN_POINT ( 'NONE',  ( -3.152548672688508926E-16, -1.562499998634406140, -5.148502694627439702 ) ) ;
#25819=FACE_OUTER_BOUND ( 'NONE', #39196, .T. ) ;
#25820=CARTESIAN_POINT ( 'NONE',  ( -4.458734124999999437, -68.56249999863439371, 0.000000000000000000 ) ) ;
#25821=CARTESIAN_POINT ( 'NONE',  ( 5.000000000000000000, -33.37499999726880873, -6.123233995736766282E-16 ) ) ;
#25825=CARTESIAN_POINT ( 'NONE',  ( -4.458734124999999437, -52.31249999863440792, 0.000000000000000000 ) ) ;
#25826=CARTESIAN_POINT ( 'NONE',  ( 4.458734124999998549, -30.97916666530106866, -2.574251347313721627 ) ) ;
#25828=CARTESIAN_POINT ( 'NONE',  ( -2.500000000000000444, 21.83333333333333215, -4.330127018922193649 ) ) ;
#25830=FACE_OUTER_BOUND ( 'NONE', #61689, .T. ) ;
#25831=CARTESIAN_POINT ( 'NONE',  ( -4.458734124999998549, -42.22916666530107932, 2.574251347313722516 ) ) ;
#25832=CARTESIAN_POINT ( 'NONE',  ( 2.500000000000002220, -79.54166666393547303, 4.330127018922192761 ) ) ;
#25836=CARTESIAN_POINT ( 'NONE',  ( 4.458734124999998549, -77.97916666530106511, -2.574251347313721627 ) ) ;
#25839=CARTESIAN_POINT ( 'NONE',  ( 5.000000000000000888, -28.58333333333333570, 2.886751345948126879 ) ) ;
#25845=CARTESIAN_POINT ( 'NONE',  ( 2.499999999999998668, 20.79166666939784847, -4.330127018922193649 ) ) ;
#25858=CARTESIAN_POINT ( 'NONE',  ( -4.458734124999999437, -12.56249999863440259, 0.000000000000000000 ) ) ;
#25866=CARTESIAN_POINT ( 'NONE',  ( -5.926426369611017623E-15, 25.37500000273118062, 5.000000000000000000 ) ) ;
#25869=CARTESIAN_POINT ( 'NONE',  ( -6.972266317189433020E-16, -21.24999999999999289, -5.000000000000000000 ) ) ;
#25875=LINE ( 'NONE', #45491, #49844 ) ;
#25879=CARTESIAN_POINT ( 'NONE',  ( -4.458734124999999437, 15.68750000136559564, 0.000000000000000000 ) ) ;
#25884=ORIENTED_EDGE ( 'NONE', *, *, #27958, .T. ) ;
#25885=CARTESIAN_POINT ( 'NONE',  ( 2.229367062499998831, -63.64583333196772941, -3.861377020970580887 ) ) ;
#25887=CARTESIAN_POINT ( 'NONE',  ( 2.229367062500001939, 12.02083333469892601, 3.861377020970579999 ) ) ;
#25888=( BOUNDED_CURVE ( )  B_SPLINE_CURVE ( 2, ( #19125, #43258, #23964, #24599, #43567, #34546, #39064, #13992, #44205 ),
 .UNSPECIFIED., .F., .F. ) 
 B_SPLINE_CURVE_WITH_KNOTS ( ( 3, 2, 2, 2, 3 ),
 ( 0.5875000000000000222, 0.5880952380952381153, 0.5892857142857143016, 0.5904761904761904878, 0.5910714285714285809 ),
 .UNSPECIFIED. ) 
 CURVE ( )  GEOMETRIC_REPRESENTATION_ITEM ( )  RATIONAL_B_SPLINE_CURVE ( ( 0.9330127018922194093, 0.9330127018922194093, 1.000000000000000000, 0.8660254037844387076, 1.000000000000000000, 0.8660254037844387076, 1.000000000000000000, 0.9330127018922194093, 0.9330127018922194093 ) ) 
 REPRESENTATION_ITEM ( '' )  );
#25889=FACE_OUTER_BOUND ( 'NONE', #31424, .T. ) ;
#25890=CARTESIAN_POINT ( 'NONE',  ( -4.458734124999999437, -56.56249999863440081, 0.000000000000000000 ) ) ;
#25891=CARTESIAN_POINT ( 'NONE',  ( -2.499999999999996447, -12.70833333060214798, 4.330127018922195425 ) ) ;
#25894=CARTESIAN_POINT ( 'NONE',  ( -1.339745962155613812, 14.79465819873851906, -5.000000000000000000 ) ) ;
#25896=CARTESIAN_POINT ( 'NONE',  ( -4.458734124999999437, -17.56249999863440792, 0.000000000000000000 ) ) ;
#25898=CARTESIAN_POINT ( 'NONE',  ( 5.000000000000000888, 23.41666666666666430, 2.886751345948126879 ) ) ;
#25899=CARTESIAN_POINT ( 'NONE',  ( -4.458734124999999437, -104.3958333319677365, -2.574251347313719407 ) ) ;
#25901=ORIENTED_EDGE ( 'NONE', *, *, #26824, .T. ) ;
#25902=CARTESIAN_POINT ( 'NONE',  ( 9.457646018065525792E-16, -101.3124999986344079, 5.148502694627439702 ) ) ;
#25903=CARTESIAN_POINT ( 'NONE',  ( 4.458734124999999437, -24.81249999863440436, -5.460374474430324690E-16 ) ) ;
#25904=CARTESIAN_POINT ( 'NONE',  ( 5.000000000000000888, -56.45833333060213732, 2.886751345948126879 ) ) ;
#25907=CARTESIAN_POINT ( 'NONE',  ( 9.457646018065525792E-16, -26.06249999863440792, 5.148502694627439702 ) ) ;
#25908=CARTESIAN_POINT ( 'NONE',  ( -4.458734124999999437, -63.56249999863440792, 0.000000000000000000 ) ) ;
#25909=CARTESIAN_POINT ( 'NONE',  ( 1.339745962155641346, 8.705341801261479162, -4.999999999999983125 ) ) ;
#25913=CARTESIAN_POINT ( 'NONE',  ( -2.500000000000000444, -9.166666666666662522, -4.330127018922193649 ) ) ;
#25924=CARTESIAN_POINT ( 'NONE',  ( -6.972266317189433020E-16, -86.12499999726880162, -5.000000000000000000 ) ) ;
#25926=CARTESIAN_POINT ( 'NONE',  ( -2.500000000000000444, -80.16666666666665719, -4.330127018922193649 ) ) ;
#25928=ORIENTED_EDGE ( 'NONE', *, *, #62273, .F. ) ;
#25931=CARTESIAN_POINT ( 'NONE',  ( 2.500000000000002220, -85.66666666666667140, 4.330127018922192761 ) ) ;
#25939=ORIENTED_EDGE ( 'NONE', *, *, #53972, .F. ) ;
#25941=FACE_OUTER_BOUND ( 'NONE', #11768, .T. ) ;
#25944=( BOUNDED_CURVE ( )  B_SPLINE_CURVE ( 2, ( #58056, #3725, #57136, #8543, #37495, #9165, #13052, #43252, #42947 ),
 .UNSPECIFIED., .F., .F. ) 
 B_SPLINE_CURVE_WITH_KNOTS ( ( 3, 2, 2, 2, 3 ),
 ( 0.9410714285714285587, 0.9416666666666666519, 0.9428571428571428381, 0.9440476190476190244, 0.9446428571428571175 ),
 .UNSPECIFIED. ) 
 CURVE ( )  GEOMETRIC_REPRESENTATION_ITEM ( )  RATIONAL_B_SPLINE_CURVE ( ( 0.9330127018922194093, 0.9330127018922194093, 1.000000000000000000, 0.8660254037844387076, 1.000000000000000000, 0.8660254037844387076, 1.000000000000000000, 0.9330127018922194093, 0.9330127018922194093 ) ) 
 REPRESENTATION_ITEM ( '' )  );
#25947=EDGE_LOOP ( 'NONE', ( #62269, #16678, #42623, #7136 ) ) ;
#25953=CARTESIAN_POINT ( 'NONE',  ( -4.458734124999999437, -79.31249999863440792, 0.000000000000000000 ) ) ;
#25954=CARTESIAN_POINT ( 'NONE',  ( -2.229367062499996610, -110.3958333319677507, 3.861377020970582219 ) ) ;
#25955=CARTESIAN_POINT ( 'NONE',  ( 5.000000000000000000, 20.58333333333333215, -2.886751345948130876 ) ) ;
#25960=CARTESIAN_POINT ( 'NONE',  ( 2.229367062499998831, -41.64583333196773651, -3.861377020970580887 ) ) ;
#25963=CARTESIAN_POINT ( 'NONE',  ( 2.229367062500001939, -51.97916666530107221, 3.861377020970579999 ) ) ;
#25965=CARTESIAN_POINT ( 'NONE',  ( 4.458734125000001214, 28.10416666803225993, 2.574251347313718519 ) ) ;
#25966=EDGE_CURVE ( 'NONE', #51908, #63455, #15607, .T. ) ;
#25967=CARTESIAN_POINT ( 'NONE',  ( -2.229367062500000163, -16.47916666530107577, -3.861377020970580443 ) ) ;
#25968=CARTESIAN_POINT ( 'NONE',  ( 2.500000000000002220, -100.6666666666666572, 4.330127018922192761 ) ) ;
#25970=CARTESIAN_POINT ( 'NONE',  ( 2.229367062499998831, -39.89583333196773651, -3.861377020970580887 ) ) ;
#25971=CARTESIAN_POINT ( 'NONE',  ( 5.000000000000000888, 6.541666669397851130, 2.886751345948126879 ) ) ;
#25972=CARTESIAN_POINT ( 'NONE',  ( -5.000000000000000000, -6.874999997268812280, 0.000000000000000000 ) ) ;
#25974=( BOUNDED_CURVE ( )  B_SPLINE_CURVE ( 2, ( #29371, #49004, #33594, #23639, #58037, #24574, #13968, #28758, #146 ),
 .UNSPECIFIED., .F., .F. ) 
 B_SPLINE_CURVE_WITH_KNOTS ( ( 3, 2, 2, 2, 3 ),
 ( 0.1732142857142857095, 0.1738095238095238027, 0.1749999999999999889, 0.1761904761904762029, 0.1767857142857142960 ),
 .UNSPECIFIED. ) 
 CURVE ( )  GEOMETRIC_REPRESENTATION_ITEM ( )  RATIONAL_B_SPLINE_CURVE ( ( 0.9330127018922194093, 0.9330127018922194093, 1.000000000000000000, 0.8660254037844387076, 1.000000000000000000, 0.8660254037844387076, 1.000000000000000000, 0.9330127018922194093, 0.9330127018922194093 ) ) 
 REPRESENTATION_ITEM ( '' )  );
#25976=CARTESIAN_POINT ( 'NONE',  ( -2.500000000000000444, 5.833333333333333037, -4.330127018922193649 ) ) ;
#25978=CARTESIAN_POINT ( 'NONE',  ( -2.229367062499996610, -2.395833331967737845, 3.861377020970582219 ) ) ;
#25980=CARTESIAN_POINT ( 'NONE',  ( 1.339745962155608039, 24.41965820146970145, 5.000000000000003553 ) ) ;
#25982=CARTESIAN_POINT ( 'NONE',  ( -4.458734124999998549, -88.22916666530107932, 2.574251347313722516 ) ) ;
#25983=CARTESIAN_POINT ( 'NONE',  ( -4.458734124999999437, -33.31249999863440792, 0.000000000000000000 ) ) ;
#25985=CARTESIAN_POINT ( 'NONE',  ( -4.458734124999999437, -81.56249999863440792, 0.000000000000000000 ) ) ;
#25987=CARTESIAN_POINT ( 'NONE',  ( -5.000000000000000000, -53.08333333333332860, -2.886751345948128211 ) ) ;
#25989=CARTESIAN_POINT ( 'NONE',  ( 9.457646018065525792E-16, -5.062499998634402587, 5.148502694627439702 ) ) ;
#25990=CARTESIAN_POINT ( 'NONE',  ( -2.229367062499996610, 24.60416666803225993, 3.861377020970582219 ) ) ;
#25991=CARTESIAN_POINT ( 'NONE',  ( -4.458734124999999437, -49.64583333196772941, -2.574251347313719407 ) ) ;
#25992=CARTESIAN_POINT ( 'NONE',  ( 5.000000000000000000, -105.4166666666666572, -2.886751345948130876 ) ) ;
#26000=CARTESIAN_POINT ( 'NONE',  ( -2.229367062500000163, -73.47916666530106511, -3.861377020970580443 ) ) ;
#26001=CARTESIAN_POINT ( 'NONE',  ( -2.229367062499996610, 27.60416666803225993, 3.861377020970582219 ) ) ;
#26004=ADVANCED_FACE ( 'NONE', ( #25889 ), #34566, .T. ) ;
#26006=FACE_OUTER_BOUND ( 'NONE', #53555, .T. ) ;
#26008=CARTESIAN_POINT ( 'NONE',  ( 2.499999999999998668, -57.33333333333333570, -4.330127018922193649 ) ) ;
#26009=EDGE_CURVE ( 'NONE', #51626, #59975, #44287, .T. ) ;
#26010=CARTESIAN_POINT ( 'NONE',  ( 5.000000000000000000, -90.37499999726880162, -6.123233995736766282E-16 ) ) ;
#26012=ORIENTED_EDGE ( 'NONE', *, *, #19220, .F. ) ;
#26013=CARTESIAN_POINT ( 'NONE',  ( -6.972266317189433020E-16, -57.25000000000000000, -5.000000000000000000 ) ) ;
#26014=CARTESIAN_POINT ( 'NONE',  ( 5.000000000000000000, -67.41666666666667140, -2.886751345948130876 ) ) ;
#26022=VERTEX_POINT ( 'NONE', #39710 ) ;
#26026=EDGE_LOOP ( 'NONE', ( #2306, #7786, #41991, #24893 ) ) ;
#26030=CARTESIAN_POINT ( 'NONE',  ( 4.458734124999998549, -46.97916666530106511, -2.574251347313721627 ) ) ;
#26034=DIRECTION ( 'NONE',  ( -0.000000000000000000, 1.000000000000000000, -0.000000000000000000 ) ) ;
#26040=CARTESIAN_POINT ( 'NONE',  ( 4.458734125000001214, -94.14583333196773651, 2.574251347313718519 ) ) ;
#26048=CARTESIAN_POINT ( 'NONE',  ( 4.458734125000001214, -1.895833331967737623, 2.574251347313718519 ) ) ;
#26050=CARTESIAN_POINT ( 'NONE',  ( 2.500000000000002220, 6.333333333333333037, 4.330127018922192761 ) ) ;
#26051=CARTESIAN_POINT ( 'NONE',  ( 4.458734124999999437, -17.06249999863440792, -5.460374474430324690E-16 ) ) ;
#26056=CARTESIAN_POINT ( 'NONE',  ( 4.458734124999998549, 14.02083333469892779, -2.574251347313721627 ) ) ;
#26059=CARTESIAN_POINT ( 'NONE',  ( -5.000000000000000000, -21.08333333333333570, -2.886751345948128211 ) ) ;
#26060=CARTESIAN_POINT ( 'NONE',  ( 2.229367062500001939, -20.97916666530107221, 3.861377020970579999 ) ) ;
#26064=CARTESIAN_POINT ( 'NONE',  ( -2.499999999999996447, -46.70833333060214443, 4.330127018922195425 ) ) ;
#26065=DIRECTION ( 'NONE',  ( -0.000000000000000000, 1.000000000000000000, -0.000000000000000000 ) ) ;
#26066=CARTESIAN_POINT ( 'NONE',  ( 4.458734125000000326, 7.104166668032259935, 2.574251347313718519 ) ) ;
#26068=CARTESIAN_POINT ( 'NONE',  ( 1.975475456537005874E-15, -47.62499999726880873, 5.000000000000000000 ) ) ;
#26070=CARTESIAN_POINT ( 'NONE',  ( -2.229367062499996610, -67.14583333196773651, 3.861377020970582219 ) ) ;
#26072=CARTESIAN_POINT ( 'NONE',  ( -2.499999999999996447, 0.1666666666666656582, 4.330127018922195425 ) ) ;
#26075=CARTESIAN_POINT ( 'NONE',  ( -2.229367062500000163, -60.47916666530106511, -3.861377020970580443 ) ) ;
#26076=CARTESIAN_POINT ( 'NONE',  ( 2.499999999999998668, -93.20833333060214443, -4.330127018922193649 ) ) ;
#26077=( BOUNDED_CURVE ( )  B_SPLINE_CURVE ( 2, ( #51888, #3328, #7829, #46741, #62500, #8768, #37722, #18418, #37408 ),
 .UNSPECIFIED., .F., .F. ) 
 B_SPLINE_CURVE_WITH_KNOTS ( ( 3, 2, 2, 2, 3 ),
 ( 0.6660714285714285365, 0.6666666666666666297, 0.6678571428571428159, 0.6690476190476190022, 0.6696428571428570953 ),
 .UNSPECIFIED. ) 
 CURVE ( )  GEOMETRIC_REPRESENTATION_ITEM ( )  RATIONAL_B_SPLINE_CURVE ( ( 0.9330127018922194093, 0.9330127018922194093, 1.000000000000000000, 0.8660254037844387076, 1.000000000000000000, 0.8660254037844387076, 1.000000000000000000, 0.9330127018922194093, 0.9330127018922194093 ) ) 
 REPRESENTATION_ITEM ( '' )  );
#26079=CARTESIAN_POINT ( 'NONE',  ( 1.339745962155612702, -56.29465819873852439, -5.000000000000000000 ) ) ;
#26082=CARTESIAN_POINT ( 'NONE',  ( 2.500000000000002220, -44.66666666666665719, 4.330127018922192761 ) ) ;
#26084=CARTESIAN_POINT ( 'NONE',  ( 5.000000000000000000, -6.374999997268812280, -6.123233995736766282E-16 ) ) ;
#26086=CARTESIAN_POINT ( 'NONE',  ( 2.229367062499998831, -104.6458333319677365, -3.861377020970580887 ) ) ;
#26087=CARTESIAN_POINT ( 'NONE',  ( 9.457646018065525792E-16, -1.312499998634405918, 5.148502694627439702 ) ) ;
#26088=CARTESIAN_POINT ( 'NONE',  ( -2.480964764533239819E-13, -59.75000000000000711, 5.000000000000000000 ) ) ;
#26096=VERTEX_POINT ( 'NONE', #60639 ) ;
#26097=CARTESIAN_POINT ( 'NONE',  ( 5.000000000000000888, -6.583333333333329485, 2.886751345948126879 ) ) ;
#26100=CARTESIAN_POINT ( 'NONE',  ( 5.000000000000000888, -101.4583333306021302, 2.886751345948126879 ) ) ;
#26102=EDGE_CURVE ( 'NONE', #56905, #58717, #53318, .T. ) ;
#26103=CARTESIAN_POINT ( 'NONE',  ( 2.229367062500001939, -29.22916666530107221, 3.861377020970579999 ) ) ;
#26107=EDGE_CURVE ( 'NONE', #53853, #57442, #33965, .T. ) ;
#26111=EDGE_CURVE ( 'NONE', #14367, #30949, #12191, .T. ) ;
#26112=VERTEX_POINT ( 'NONE', #37677 ) ;
#26113=CARTESIAN_POINT ( 'NONE',  ( 1.975475456537005874E-15, -93.62499999726881583, 5.000000000000000000 ) ) ;
#26115=CARTESIAN_POINT ( 'NONE',  ( 4.458734125000001214, -76.14583333196773651, 2.574251347313718519 ) ) ;
#26120=CARTESIAN_POINT ( 'NONE',  ( -4.458734124999998549, -5.479166665301072214, 2.574251347313722516 ) ) ;
#26121=ORIENTED_EDGE ( 'NONE', *, *, #1204, .F. ) ;
#26122=CARTESIAN_POINT ( 'NONE',  ( 1.975475456537005874E-15, -84.74999999999998579, 5.000000000000000000 ) ) ;
#26123=DIRECTION ( 'NONE',  ( 0.000000000000000000, 0.000000000000000000, 1.000000000000000000 ) ) ;
#26129=CARTESIAN_POINT ( 'NONE',  ( 5.000000000000000888, -75.45833333060214443, 2.886751345948126879 ) ) ;
#26130=ORIENTED_EDGE ( 'NONE', *, *, #31521, .F. ) ;
#26131=CARTESIAN_POINT ( 'NONE',  ( -3.152548672688508926E-16, -88.56249999863439371, -5.148502694627439702 ) ) ;
#26133=CARTESIAN_POINT ( 'NONE',  ( -4.458734124999998549, -5.229166665301072214, 2.574251347313722516 ) ) ;
#26136=CARTESIAN_POINT ( 'NONE',  ( -4.999999999999999112, -30.79166666393548013, 2.886751345948131764 ) ) ;
#26138=CARTESIAN_POINT ( 'NONE',  ( 4.458734125000000326, 23.10416666803225993, 2.574251347313718519 ) ) ;
#26139=CARTESIAN_POINT ( 'NONE',  ( -4.999999999999998224, -37.79166666393548724, 2.886751345948131764 ) ) ;
#26141=CARTESIAN_POINT ( 'NONE',  ( 4.458734124999999437, -50.81249999863440792, -5.460374474430324690E-16 ) ) ;
#26142=CARTESIAN_POINT ( 'NONE',  ( 4.458734124999998549, -38.97916666530107221, -2.574251347313721627 ) ) ;
#26145=CARTESIAN_POINT ( 'NONE',  ( 2.500000000000002220, 22.33333333333333215, 4.330127018922192761 ) ) ;
#26147=CARTESIAN_POINT ( 'NONE',  ( 5.000000000000000888, -26.45833333060214798, 2.886751345948126879 ) ) ;
#26148=CARTESIAN_POINT ( 'NONE',  ( -4.458734124999999437, -44.31249999863440081, 0.000000000000000000 ) ) ;
#26149=CARTESIAN_POINT ( 'NONE',  ( 5.000000000000000000, -76.37499999726880162, -6.123233995736766282E-16 ) ) ;
#26153=CARTESIAN_POINT ( 'NONE',  ( -2.229367062500000163, -81.72916666530106511, -3.861377020970580443 ) ) ;
#26156=CARTESIAN_POINT ( 'NONE',  ( 5.000000000000000000, -28.41666666666666430, -2.886751345948129988 ) ) ;
#26160=EDGE_LOOP ( 'NONE', ( #26850, #29150, #9181, #14623 ) ) ;
#26161=CARTESIAN_POINT ( 'NONE',  ( 2.229367062500001939, -88.97916666530106511, 3.861377020970579999 ) ) ;
#26162=CARTESIAN_POINT ( 'NONE',  ( 4.458734125000001214, 12.85416666803226171, 2.574251347313718519 ) ) ;
#26163=CARTESIAN_POINT ( 'NONE',  ( 1.060575238724906964E-15, 18.37500000273118772, 5.773502691896257311 ) ) ;
#26169=CARTESIAN_POINT ( 'NONE',  ( 1.975475456537005874E-15, 15.37500000273118417, 5.000000000000000000 ) ) ;
#26170=CARTESIAN_POINT ( 'NONE',  ( 0.000000000000000000, -120.0000000000000000, 0.000000000000000000 ) ) ;
#26174=( BOUNDED_CURVE ( )  B_SPLINE_CURVE ( 2, ( #35463, #51221, #16158, #25485, #55084, #26129, #35785, #46065, #45426 ),
 .UNSPECIFIED., .F., .F. ) 
 B_SPLINE_CURVE_WITH_KNOTS ( ( 3, 2, 2, 2, 3 ),
 ( 0.7446428571428571619, 0.7452380952380952550, 0.7464285714285714413, 0.7476190476190476275, 0.7482142857142857206 ),
 .UNSPECIFIED. ) 
 CURVE ( )  GEOMETRIC_REPRESENTATION_ITEM ( )  RATIONAL_B_SPLINE_CURVE ( ( 0.9330127018922194093, 0.9330127018922194093, 1.000000000000000000, 0.8660254037844387076, 1.000000000000000000, 0.8660254037844387076, 1.000000000000000000, 0.9330127018922194093, 0.9330127018922194093 ) ) 
 REPRESENTATION_ITEM ( '' )  );
#26176=CARTESIAN_POINT ( 'NONE',  ( 2.229367062500001939, -13.22916666530107221, 3.861377020970579999 ) ) ;
#26182=AXIS2_PLACEMENT_3D ( 'NONE', #16857, #61253, #17507 ) ;
#26186=EDGE_LOOP ( 'NONE', ( #45533, #43034, #228, #62752 ) ) ;
#26190=VERTEX_POINT ( 'NONE', #36183 ) ;
#26191=CARTESIAN_POINT ( 'NONE',  ( -1.339745962155613812, -8.080341798530294994, -5.000000000000000000 ) ) ;
#26195=VERTEX_POINT ( 'NONE', #37999 ) ;
#26196=CARTESIAN_POINT ( 'NONE',  ( 2.500000000000002220, 11.33333333333333393, 4.330127018922192761 ) ) ;
#26197=CARTESIAN_POINT ( 'NONE',  ( -4.458734124999999437, 11.60416666803225993, -2.574251347313719407 ) ) ;
#26203=CARTESIAN_POINT ( 'NONE',  ( 4.458734125000000326, -66.89583333196773651, 2.574251347313718519 ) ) ;
#26204=CARTESIAN_POINT ( 'NONE',  ( -6.972266317189433020E-16, -50.12499999726881583, -5.000000000000000000 ) ) ;
#26205=CARTESIAN_POINT ( 'NONE',  ( 2.229367062500001939, 14.02083333469892779, 3.861377020970579999 ) ) ;
#26206=EDGE_CURVE ( 'NONE', #4115, #36130, #9350, .T. ) ;
#26209=CARTESIAN_POINT ( 'NONE',  ( 4.458734125000001214, -53.14583333196773651, 2.574251347313718519 ) ) ;
#26210=CARTESIAN_POINT ( 'NONE',  ( 2.500000000000002220, -16.54166666393548368, 4.330127018922192761 ) ) ;
#26213=CARTESIAN_POINT ( 'NONE',  ( 2.499999999999998668, -64.20833333060213022, -4.330127018922193649 ) ) ;
#26214=CARTESIAN_POINT ( 'NONE',  ( 2.229367062500001939, -17.22916666530106866, 3.861377020970579999 ) ) ;
#26217=CARTESIAN_POINT ( 'NONE',  ( 4.458734125000001214, -105.8958333319677365, 2.574251347313718519 ) ) ;
#26220=CARTESIAN_POINT ( 'NONE',  ( 4.458734124999998549, -103.9791666653010509, -2.574251347313721627 ) ) ;
#26221=CARTESIAN_POINT ( 'NONE',  ( 2.229367062500001939, -28.97916666530107221, 3.861377020970579999 ) ) ;
#26222=CARTESIAN_POINT ( 'NONE',  ( 2.499999999999998668, -62.20833333060214443, -4.330127018922193649 ) ) ;
#26225=CARTESIAN_POINT ( 'NONE',  ( -2.229367062499996610, -22.14583333196773651, 3.861377020970582219 ) ) ;
#26226=CARTESIAN_POINT ( 'NONE',  ( -2.229367062499996610, -65.39583333196773651, 3.861377020970582219 ) ) ;
#26231=CARTESIAN_POINT ( 'NONE',  ( -4.999999999999999112, -9.916666666666662522, 2.886751345948131764 ) ) ;
#26235=CARTESIAN_POINT ( 'NONE',  ( 1.464175926609780648E-14, 21.87500000273118062, -5.000000000000000000 ) ) ;
#26246=CARTESIAN_POINT ( 'NONE',  ( 1.975475456537005874E-15, -53.62499999726880162, 5.000000000000000000 ) ) ;
#26250=ORIENTED_EDGE ( 'NONE', *, *, #13469, .T. ) ;
#26252=ORIENTED_EDGE ( 'NONE', *, *, #601, .F. ) ;
#26257=ORIENTED_EDGE ( 'NONE', *, *, #18075, .T. ) ;
#26261=ORIENTED_EDGE ( 'NONE', *, *, #6177, .T. ) ;
#26264=CARTESIAN_POINT ( 'NONE',  ( 4.458734124999999437, -74.81249999863440792, -5.460374474430324690E-16 ) ) ;
#26265=CARTESIAN_POINT ( 'NONE',  ( -4.458734124999999437, 29.60416666803225993, -2.574251347313719407 ) ) ;
#26266=CARTESIAN_POINT ( 'NONE',  ( 1.975475456537005874E-15, -18.74999999999999645, 5.000000000000000000 ) ) ;
#26267=ORIENTED_EDGE ( 'NONE', *, *, #10187, .F. ) ;
#26272=CARTESIAN_POINT ( 'NONE',  ( 9.457646018065525792E-16, -44.06249999863439371, 5.148502694627439702 ) ) ;
#26275=CARTESIAN_POINT ( 'NONE',  ( -4.458734124999997661, -48.22916666530106511, 2.574251347313722516 ) ) ;
#26277=CARTESIAN_POINT ( 'NONE',  ( -2.229367062500000163, 28.52083333469892779, -3.861377020970580443 ) ) ;
#26278=ADVANCED_FACE ( 'NONE', ( #56121 ), #12044, .T. ) ;
#26279=CARTESIAN_POINT ( 'NONE',  ( -2.499999999999996447, -98.83333333333332860, 4.330127018922195425 ) ) ;
#26281=CARTESIAN_POINT ( 'NONE',  ( 2.229367062499998831, -40.89583333196773651, -3.861377020970580887 ) ) ;
#26282=CARTESIAN_POINT ( 'NONE',  ( -2.499999999999996447, 0.2916666693978525737, 4.330127018922195425 ) ) ;
#26283=CARTESIAN_POINT ( 'NONE',  ( 0.000000000000000000, -120.0000000000000000, 0.000000000000000000 ) ) ;
#26287=CARTESIAN_POINT ( 'NONE',  ( 2.229367062500001939, -97.97916666530105090, 3.861377020970579999 ) ) ;
#26289=CARTESIAN_POINT ( 'NONE',  ( -2.229367062500000163, 0.2708333346989263979, -3.861377020970580443 ) ) ;
#26292=CARTESIAN_POINT ( 'NONE',  ( 9.457646018065525792E-16, -89.06249999863439371, 5.148502694627439702 ) ) ;
#26294=CARTESIAN_POINT ( 'NONE',  ( 4.458734124999999437, -88.06249999863439371, -5.460374474430324690E-16 ) ) ;
#26296=FACE_OUTER_BOUND ( 'NONE', #40405, .T. ) ;
#26299=CARTESIAN_POINT ( 'NONE',  ( 4.458734124999999437, -5.812499998634403475, -5.460374474430324690E-16 ) ) ;
#26300=CARTESIAN_POINT ( 'NONE',  ( 4.458734124999998549, 18.02083333469892779, -2.574251347313721627 ) ) ;
#26302=CARTESIAN_POINT ( 'NONE',  ( 9.457646018065525792E-16, -50.31249999863440792, 5.148502694627439702 ) ) ;
#26307=ORIENTED_EDGE ( 'NONE', *, *, #47442, .F. ) ;
#26310=CARTESIAN_POINT ( 'NONE',  ( -2.229367062499996610, -72.14583333196773651, 3.861377020970582219 ) ) ;
#26311=CARTESIAN_POINT ( 'NONE',  ( 4.458734124999998549, 27.02083333469892423, -2.574251347313721627 ) ) ;
#26319=CARTESIAN_POINT ( 'NONE',  ( 1.060575238724906964E-15, -65.75000000000000000, 5.773502691896257311 ) ) ;
#26323=ORIENTED_EDGE ( 'NONE', *, *, #42923, .F. ) ;
#26324=CARTESIAN_POINT ( 'NONE',  ( -6.972266317189433020E-16, -73.12499999726878741, -5.000000000000000000 ) ) ;
#26333=VERTEX_POINT ( 'NONE', #14170 ) ;
#26340=CARTESIAN_POINT ( 'NONE',  ( 9.457646018065525792E-16, -45.31249999863440081, 5.148502694627439702 ) ) ;
#26347=CARTESIAN_POINT ( 'NONE',  ( 5.000000000000000000, 22.50000000000000000, -6.123233995736766282E-16 ) ) ;
#26349=CARTESIAN_POINT ( 'NONE',  ( -4.458734124999999437, -94.64583333196773651, -2.574251347313719407 ) ) ;
#26350=CARTESIAN_POINT ( 'NONE',  ( 5.000000000000000000, -2.416666666666663410, -2.886751345948130876 ) ) ;
#26351=ORIENTED_EDGE ( 'NONE', *, *, #40084, .F. ) ;
#26358=CARTESIAN_POINT ( 'NONE',  ( 4.458734124999998549, -1.729166665301068440, -2.574251347313721627 ) ) ;
#26359=EDGE_CURVE ( 'NONE', #8589, #56396, #45056, .T. ) ;
#26360=EDGE_CURVE ( 'NONE', #35996, #16789, #38609, .T. ) ;
#26361=CARTESIAN_POINT ( 'NONE',  ( 5.000000000000000000, -1.291666663935479908, -2.886751345948130876 ) ) ;
#26362=CARTESIAN_POINT ( 'NONE',  ( 2.229367062500001939, -24.22916666530107577, 3.861377020970579999 ) ) ;
#26366=CARTESIAN_POINT ( 'NONE',  ( 5.000000000000000000, 23.70833333606451632, -2.886751345948130876 ) ) ;
#26369=CARTESIAN_POINT ( 'NONE',  ( -3.152548672688508926E-16, 18.18750000136559564, -5.148502694627439702 ) ) ;
#26370=ORIENTED_EDGE ( 'NONE', *, *, #34199, .T. ) ;
#26371=CARTESIAN_POINT ( 'NONE',  ( 6.123233995736766282E-16, -120.0000000000000000, -5.000000000000000000 ) ) ;
#26372=CARTESIAN_POINT ( 'NONE',  ( 1.339745962155615144, -71.58034179853027013, 4.999999999999999112 ) ) ;
#26373=CARTESIAN_POINT ( 'NONE',  ( 2.499999999999998668, -86.33333333333332860, -4.330127018922193649 ) ) ;
#26374=CARTESIAN_POINT ( 'NONE',  ( 4.458734124999999437, -19.81249999863440081, -5.460374474430324690E-16 ) ) ;
#26376=EDGE_CURVE ( 'NONE', #27636, #40984, #4223, .T. ) ;
#26379=CARTESIAN_POINT ( 'NONE',  ( 5.000000000000000000, -47.37499999726880873, -6.123233995736766282E-16 ) ) ;
#26380=DIRECTION ( 'NONE',  ( -0.000000000000000000, 1.000000000000000000, -0.000000000000000000 ) ) ;
#26381=CARTESIAN_POINT ( 'NONE',  ( -4.458734124999999437, 7.604166668032259935, -2.574251347313719407 ) ) ;
#26386=CARTESIAN_POINT ( 'NONE',  ( 2.229367062500001939, -69.97916666530107932, 3.861377020970579999 ) ) ;
#26388=CARTESIAN_POINT ( 'NONE',  ( -5.000000000000000000, -0.08333333333333457771, -2.886751345948128211 ) ) ;
#26391=CARTESIAN_POINT ( 'NONE',  ( -3.152548672688508926E-16, -56.56249999863439371, -5.148502694627439702 ) ) ;
#26392=CARTESIAN_POINT ( 'NONE',  ( -2.500000000000000444, -97.04166666393545881, -4.330127018922193649 ) ) ;
#26396=CARTESIAN_POINT ( 'NONE',  ( 2.493747252781420335E-13, -91.12499999726880162, -5.000000000000000000 ) ) ;
#26397=CARTESIAN_POINT ( 'NONE',  ( -5.000000000000000000, -48.00000000000000000, 0.000000000000000000 ) ) ;
#26398=CARTESIAN_POINT ( 'NONE',  ( -2.500000000000000444, 18.83333333333333215, -4.330127018922193649 ) ) ;
#26400=EDGE_LOOP ( 'NONE', ( #47113, #16408, #26429, #17605 ) ) ;
#26401=CARTESIAN_POINT ( 'NONE',  ( 2.229367062500001939, -105.9791666653010651, 3.861377020970579999 ) ) ;
#26402=CARTESIAN_POINT ( 'NONE',  ( 4.458734124999999437, -3.062499998634407472, -5.460374474430324690E-16 ) ) ;
#26404=CARTESIAN_POINT ( 'NONE',  ( -2.480964764533239819E-13, -73.62499999726883004, 5.000000000000000000 ) ) ;
#26408=CARTESIAN_POINT ( 'NONE',  ( -1.230605004983934782E-13, -25.75000000000000355, 5.000000000000000000 ) ) ;
#26411=ORIENTED_EDGE ( 'NONE', *, *, #60517, .F. ) ;
#26412=AXIS2_PLACEMENT_3D ( 'NONE', #23466, #28902, #8661 ) ;
#26413=CARTESIAN_POINT ( 'NONE',  ( 1.339745962155612702, -6.294658198738520838, -5.000000000000000000 ) ) ;
#26415=EDGE_LOOP ( 'NONE', ( #62992, #56814, #51773, #42105 ) ) ;
#26416=CARTESIAN_POINT ( 'NONE',  ( 2.499999999999998668, -101.2083333306021444, -4.330127018922193649 ) ) ;
#26418=CARTESIAN_POINT ( 'NONE',  ( -4.458734124999999437, -30.64583333196774007, -2.574251347313719407 ) ) ;
#26419=CARTESIAN_POINT ( 'NONE',  ( -6.972266317189433020E-16, -10.24999999999999822, -5.000000000000000000 ) ) ;
#26427=CARTESIAN_POINT ( 'NONE',  ( 4.458734125000001214, -81.14583333196773651, 2.574251347313718519 ) ) ;
#26428=CARTESIAN_POINT ( 'NONE',  ( -5.000000000000000000, 13.12500000273118417, 0.000000000000000000 ) ) ;
#26429=ORIENTED_EDGE ( 'NONE', *, *, #31510, .T. ) ;
#26433=CARTESIAN_POINT ( 'NONE',  ( 4.458734125000001214, -11.14583333196774007, 2.574251347313718519 ) ) ;
#26434=ORIENTED_EDGE ( 'NONE', *, *, #60219, .T. ) ;
#26436=ADVANCED_FACE ( 'NONE', ( #19631 ), #58868, .T. ) ;
#26437=CARTESIAN_POINT ( 'NONE',  ( 0.000000000000000000, -120.0000000000000000, 5.000000000000000000 ) ) ;
#26439=CARTESIAN_POINT ( 'NONE',  ( -4.458734124999999437, -7.562499998634404363, 0.000000000000000000 ) ) ;
#26447=CARTESIAN_POINT ( 'NONE',  ( 2.229367062500001939, -86.97916666530107932, 3.861377020970579999 ) ) ;
#26449=CARTESIAN_POINT ( 'NONE',  ( -3.152548672688508926E-16, -5.562499998634402587, -5.148502694627439702 ) ) ;
#26450=AXIS2_PLACEMENT_3D ( 'NONE', #51412, #41423, #16993 ) ;
#26451=EDGE_CURVE ( 'NONE', #50637, #6014, #47138, .T. ) ;
#26452=DIRECTION ( 'NONE',  ( -0.000000000000000000, 1.000000000000000000, -0.000000000000000000 ) ) ;
#26455=CARTESIAN_POINT ( 'NONE',  ( 5.000000000000000888, -28.45833333060214443, 2.886751345948126879 ) ) ;
#26456=CARTESIAN_POINT ( 'NONE',  ( -6.972266317189433020E-16, -77.12499999726881583, -5.000000000000000000 ) ) ;
#26457=CARTESIAN_POINT ( 'NONE',  ( -4.458734124999999437, 24.68750000136559208, 0.000000000000000000 ) ) ;
#26458=CARTESIAN_POINT ( 'NONE',  ( -6.972266317189433020E-16, -110.1249999972688158, -5.000000000000000000 ) ) ;
#26460=EDGE_CURVE ( 'NONE', #19049, #58767, #22533, .T. ) ;
#26461=CARTESIAN_POINT ( 'NONE',  ( -4.458734124999998549, -50.22916666530107221, 2.574251347313722516 ) ) ;
#26462=CARTESIAN_POINT ( 'NONE',  ( -4.458734124999999437, -37.64583333196774362, -2.574251347313719407 ) ) ;
#26465=CARTESIAN_POINT ( 'NONE',  ( 5.000000000000000000, 15.58333333333333215, -2.886751345948129988 ) ) ;
#26466=EDGE_CURVE ( 'NONE', #23647, #43124, #38117, .T. ) ;
#26468=LINE ( 'NONE', #2043, #28459 ) ;
#26469=CARTESIAN_POINT ( 'NONE',  ( 4.458734125000001214, -44.89583333196774362, 2.574251347313718519 ) ) ;
#26470=CARTESIAN_POINT ( 'NONE',  ( 1.060575238724906964E-15, -78.62499999726880162, 5.773502691896257311 ) ) ;
#26473=EDGE_CURVE ( 'NONE', #23523, #57684, #1002, .T. ) ;
#26475=CARTESIAN_POINT ( 'NONE',  ( 4.458734125000000326, -85.14583333196773651, 2.574251347313718519 ) ) ;
#26478=CARTESIAN_POINT ( 'NONE',  ( 2.500000000000002220, -27.66666666666666430, 4.330127018922192761 ) ) ;
#26482=ORIENTED_EDGE ( 'NONE', *, *, #3249, .T. ) ;
#26483=CARTESIAN_POINT ( 'NONE',  ( -2.229367062500000163, -89.47916666530106511, -3.861377020970580443 ) ) ;
#26484=CARTESIAN_POINT ( 'NONE',  ( -4.458734124999999437, 12.43750000136559564, 0.000000000000000000 ) ) ;
#26485=CARTESIAN_POINT ( 'NONE',  ( -2.500000000000000444, 14.95833333606451809, -4.330127018922193649 ) ) ;
#26490=DIRECTION ( 'NONE',  ( -0.000000000000000000, 1.000000000000000000, -0.000000000000000000 ) ) ;
#26492=DIRECTION ( 'NONE',  ( -0.000000000000000000, 1.000000000000000000, -0.000000000000000000 ) ) ;
#26497=CARTESIAN_POINT ( 'NONE',  ( 4.458734124999999437, -15.06249999863440436, -5.460374474430324690E-16 ) ) ;
#26499=CARTESIAN_POINT ( 'NONE',  ( 1.339745962155600711, 17.41965820146970145, 5.000000000000007994 ) ) ;
#26507=ORIENTED_EDGE ( 'NONE', *, *, #17395, .T. ) ;
#26509=CARTESIAN_POINT ( 'NONE',  ( -4.458734124999998549, -64.47916666530106511, 2.574251347313722516 ) ) ;
#26512=ORIENTED_EDGE ( 'NONE', *, *, #26466, .F. ) ;
#26513=CARTESIAN_POINT ( 'NONE',  ( 1.975475456537005874E-15, -7.624999997268812280, 5.000000000000000000 ) ) ;
#26518=CARTESIAN_POINT ( 'NONE',  ( -1.339745962155610925, -109.6696581960073047, 5.000000000000000000 ) ) ;
#26519=CARTESIAN_POINT ( 'NONE',  ( -2.229367062499996610, 9.854166668032261711, 3.861377020970582219 ) ) ;
#26523=CARTESIAN_POINT ( 'NONE',  ( 6.123233995736766282E-16, -120.0000000000000000, -5.000000000000000000 ) ) ;
#26526=CARTESIAN_POINT ( 'NONE',  ( -4.458734124999997661, -71.22916666530107932, 2.574251347313722516 ) ) ;
#26527=CARTESIAN_POINT ( 'NONE',  ( 0.000000000000000000, -120.0000000000000000, 5.000000000000000000 ) ) ;
#26528=CARTESIAN_POINT ( 'NONE',  ( 2.229367062499998831, 10.35416666803225993, -3.861377020970580887 ) ) ;
#26529=CARTESIAN_POINT ( 'NONE',  ( -2.500000000000000444, -63.16666666666666430, -4.330127018922193649 ) ) ;
#26531=CARTESIAN_POINT ( 'NONE',  ( -4.458734124999999437, -56.64583333196773651, -2.574251347313719407 ) ) ;
#26532=CARTESIAN_POINT ( 'NONE',  ( 2.499999999999998668, -15.20833333060214443, -4.330127018922193649 ) ) ;
#26533=DIRECTION ( 'NONE',  ( -0.000000000000000000, 1.000000000000000000, -0.000000000000000000 ) ) ;
#26534=CARTESIAN_POINT ( 'NONE',  ( -2.229367062500000163, -22.72916666530107221, -3.861377020970580443 ) ) ;
#26535=ORIENTED_EDGE ( 'NONE', *, *, #40185, .T. ) ;
#26536=VECTOR ( 'NONE', #2964, 1000.000000000000000 ) ;
#26538=CARTESIAN_POINT ( 'NONE',  ( 5.000000000000000000, 29.50000000000000000, -6.123233995736766282E-16 ) ) ;
#26542=CARTESIAN_POINT ( 'NONE',  ( -3.152548672688508926E-16, -103.8124999986344221, -5.148502694627439702 ) ) ;
#26543=AXIS2_PLACEMENT_3D ( 'NONE', #24269, #34885, #49987 ) ;
#26544=CARTESIAN_POINT ( 'NONE',  ( -4.458734124999999437, -27.31249999863440081, 0.000000000000000000 ) ) ;
#26545=CARTESIAN_POINT ( 'NONE',  ( -2.499999999999996447, -63.70833333060215153, 4.330127018922195425 ) ) ;
#26548=CARTESIAN_POINT ( 'NONE',  ( -3.152548672688508926E-16, -23.56249999863440436, -5.148502694627439702 ) ) ;
#26549=CARTESIAN_POINT ( 'NONE',  ( -2.229367062500000163, -71.72916666530107932, -3.861377020970580443 ) ) ;
#26550=CARTESIAN_POINT ( 'NONE',  ( 0.000000000000000000, -120.0000000000000000, 5.000000000000000000 ) ) ;
#26554=CARTESIAN_POINT ( 'NONE',  ( 2.499999999999998668, -10.33333333333333393, -4.330127018922193649 ) ) ;
#26558=( BOUNDED_CURVE ( )  B_SPLINE_CURVE ( 2, ( #14882, #29994, #40606, #16170, #50584, #25176, #35795, #44148, #39640 ),
 .UNSPECIFIED., .F., .F. ) 
 B_SPLINE_CURVE_WITH_KNOTS ( ( 3, 2, 2, 2, 3 ),
 ( 0.2124999999999999944, 0.2130952380952380876, 0.2142857142857142738, 0.2154761904761904878, 0.2160714285714285809 ),
 .UNSPECIFIED. ) 
 CURVE ( )  GEOMETRIC_REPRESENTATION_ITEM ( )  RATIONAL_B_SPLINE_CURVE ( ( 0.9330127018922194093, 0.9330127018922194093, 1.000000000000000000, 0.8660254037844387076, 1.000000000000000000, 0.8660254037844387076, 1.000000000000000000, 0.9330127018922194093, 0.9330127018922194093 ) ) 
 REPRESENTATION_ITEM ( '' )  );
#26559=CARTESIAN_POINT ( 'NONE',  ( -5.000000000000000000, -2.874999997268815832, 0.000000000000000000 ) ) ;
#26560=CARTESIAN_POINT ( 'NONE',  ( 2.500000000000002220, -90.66666666666665719, 4.330127018922192761 ) ) ;
#26562=AXIS2_PLACEMENT_3D ( 'NONE', #24618, #38454, #58403 ) ;
#26563=CARTESIAN_POINT ( 'NONE',  ( 5.000000000000000000, 25.58333333333333215, -2.886751345948130876 ) ) ;
#26573=ORIENTED_EDGE ( 'NONE', *, *, #12582, .T. ) ;
#26574=CARTESIAN_POINT ( 'NONE',  ( -1.339745962155613812, -54.08034179853029144, -5.000000000000000000 ) ) ;
#26580=ORIENTED_EDGE ( 'NONE', *, *, #50061, .T. ) ;
#26583=VECTOR ( 'NONE', #30029, 1000.000000000000000 ) ;
#26584=CARTESIAN_POINT ( 'NONE',  ( 1.975475456537005874E-15, -55.74999999999999289, 5.000000000000000000 ) ) ;
#26585=ORIENTED_EDGE ( 'NONE', *, *, #39305, .F. ) ;
#26591=CARTESIAN_POINT ( 'NONE',  ( -2.229367062500000163, -76.47916666530106511, -3.861377020970580443 ) ) ;
#26592=CARTESIAN_POINT ( 'NONE',  ( -4.458734124999998549, 28.77083333469892779, 2.574251347313722516 ) ) ;
#26595=CARTESIAN_POINT ( 'NONE',  ( -5.000000000000000000, 5.041666669397853795, -2.886751345948128211 ) ) ;
#26597=EDGE_CURVE ( 'NONE', #14391, #55487, #20606, .T. ) ;
#26600=DIRECTION ( 'NONE',  ( -0.000000000000000000, 1.000000000000000000, -0.000000000000000000 ) ) ;
#26602=CARTESIAN_POINT ( 'NONE',  ( 1.975475456537005874E-15, -48.62499999726880162, 5.000000000000000000 ) ) ;
#26603=CARTESIAN_POINT ( 'NONE',  ( -2.229367062500000163, -54.47916666530107221, -3.861377020970580443 ) ) ;
#26605=CARTESIAN_POINT ( 'NONE',  ( -2.229367062499996610, 27.85416666803225993, 3.861377020970582219 ) ) ;
#26606=CARTESIAN_POINT ( 'NONE',  ( -4.999999999999999112, -107.9166666666666572, 2.886751345948131764 ) ) ;
#26607=CARTESIAN_POINT ( 'NONE',  ( 9.457646018065525792E-16, -36.31249999863440792, 5.148502694627439702 ) ) ;
#26608=CARTESIAN_POINT ( 'NONE',  ( 5.000000000000000888, 3.541666669397852019, 2.886751345948126879 ) ) ;
#26609=CARTESIAN_POINT ( 'NONE',  ( 1.975475456537005874E-15, -28.74999999999999645, 5.000000000000000000 ) ) ;
#26612=CARTESIAN_POINT ( 'NONE',  ( -6.972266317189433020E-16, -76.12499999726880162, -5.000000000000000000 ) ) ;
#26613=CARTESIAN_POINT ( 'NONE',  ( -2.229367062499996610, -98.14583333196773651, 3.861377020970582219 ) ) ;
#26614=CARTESIAN_POINT ( 'NONE',  ( -4.458734124999999437, -7.562499998634404363, 0.000000000000000000 ) ) ;
#26615=VERTEX_POINT ( 'NONE', #35388 ) ;
#26616=DIRECTION ( 'NONE',  ( -0.000000000000000000, 1.000000000000000000, -0.000000000000000000 ) ) ;
#26618=CARTESIAN_POINT ( 'NONE',  ( 2.229367062500001939, -86.97916666530107932, 3.861377020970579999 ) ) ;
#26619=CARTESIAN_POINT ( 'NONE',  ( -4.458734124999999437, -87.56249999863439371, 0.000000000000000000 ) ) ;
#26621=CARTESIAN_POINT ( 'NONE',  ( 2.500000000000002220, -2.541666663935477466, 4.330127018922192761 ) ) ;
#26623=CARTESIAN_POINT ( 'NONE',  ( 2.229367062499998831, -8.645833331967736513, -3.861377020970580887 ) ) ;
#26624=CARTESIAN_POINT ( 'NONE',  ( -4.458734124999999437, 17.43750000136559208, 0.000000000000000000 ) ) ;
#26625=CARTESIAN_POINT ( 'NONE',  ( 4.458734124999999437, -50.06249999863440792, -5.460374474430324690E-16 ) ) ;
#26629=CARTESIAN_POINT ( 'NONE',  ( 1.975475456537005874E-15, -84.74999999999998579, 5.000000000000000000 ) ) ;
#26634=CARTESIAN_POINT ( 'NONE',  ( 4.458734124999999437, -77.81249999863440792, -5.460374474430324690E-16 ) ) ;
#26635=CARTESIAN_POINT ( 'NONE',  ( -3.152548672688508926E-16, 28.18750000136559564, -5.148502694627439702 ) ) ;
#26637=( BOUNDED_CURVE ( )  B_SPLINE_CURVE ( 2, ( #50973, #12041, #15918, #45183, #55802, #30383, #50006, #17189, #26204 ),
 .UNSPECIFIED., .F., .F. ) 
 B_SPLINE_CURVE_WITH_KNOTS ( ( 3, 2, 2, 2, 3 ),
 ( 0.5625000000000000000, 0.5630952380952380931, 0.5642857142857142794, 0.5654761904761904656, 0.5660714285714285587 ),
 .UNSPECIFIED. ) 
 CURVE ( )  GEOMETRIC_REPRESENTATION_ITEM ( )  RATIONAL_B_SPLINE_CURVE ( ( 0.9330127018922194093, 0.9330127018922194093, 1.000000000000000000, 0.8660254037844387076, 1.000000000000000000, 0.8660254037844387076, 1.000000000000000000, 0.9330127018922194093, 0.9330127018922194093 ) ) 
 REPRESENTATION_ITEM ( '' )  );
#26642=CARTESIAN_POINT ( 'NONE',  ( -2.500000000000000444, -65.16666666666667140, -4.330127018922193649 ) ) ;
#26645=VERTEX_POINT ( 'NONE', #40839 ) ;
#26647=CARTESIAN_POINT ( 'NONE',  ( -4.999999999999998224, 9.083333333333333925, 2.886751345948131764 ) ) ;
#26651=EDGE_CURVE ( 'NONE', #63596, #34574, #48796, .T. ) ;
#26660=ORIENTED_EDGE ( 'NONE', *, *, #40155, .T. ) ;
#26663=CARTESIAN_POINT ( 'NONE',  ( 4.458734124999998549, -52.97916666530107932, -2.574251347313721627 ) ) ;
#26670=ADVANCED_FACE ( 'NONE', ( #42107 ), #31833, .F. ) ;
#26671=FACE_OUTER_BOUND ( 'NONE', #41989, .T. ) ;
#26673=ADVANCED_FACE ( 'NONE', ( #7719 ), #27637, .T. ) ;
#26674=CARTESIAN_POINT ( 'NONE',  ( 4.458734125000001214, -96.14583333196772230, 2.574251347313718519 ) ) ;
#26682=VECTOR ( 'NONE', #33429, 1000.000000000000000 ) ;
#26684=CARTESIAN_POINT ( 'NONE',  ( -4.458734124999999437, -2.312499998634407028, 0.000000000000000000 ) ) ;
#26685=CARTESIAN_POINT ( 'NONE',  ( -2.229367062499996610, -93.39583333196773651, 3.861377020970582219 ) ) ;
#26687=CARTESIAN_POINT ( 'NONE',  ( 2.229367062500001939, -21.22916666530107221, 3.861377020970579999 ) ) ;
#26693=CARTESIAN_POINT ( 'NONE',  ( -4.458734124999999437, 17.35416666803225993, -2.574251347313719407 ) ) ;
#26695=CARTESIAN_POINT ( 'NONE',  ( 1.975475456537005874E-15, -52.62499999726880873, 5.000000000000000000 ) ) ;
#26696=DIRECTION ( 'NONE',  ( -0.000000000000000000, 1.000000000000000000, 0.000000000000000000 ) ) ;
#26697=CARTESIAN_POINT ( 'NONE',  ( 1.060575238724906964E-15, -84.74999999999998579, 5.773502691896257311 ) ) ;
#26698=CARTESIAN_POINT ( 'NONE',  ( -4.458734124999998549, -20.22916666530107221, 2.574251347313722516 ) ) ;
#26702=EDGE_CURVE ( 'NONE', #62889, #45023, #42240, .T. ) ;
#26703=CARTESIAN_POINT ( 'NONE',  ( 2.499999999999998668, -48.20833333060215153, -4.330127018922193649 ) ) ;
#26705=CARTESIAN_POINT ( 'NONE',  ( 4.458734124999999437, 7.187500001365594748, -5.460374474430324690E-16 ) ) ;
#26706=LINE ( 'NONE', #8042, #34502 ) ;
#26707=FACE_OUTER_BOUND ( 'NONE', #44046, .T. ) ;
#26709=CARTESIAN_POINT ( 'NONE',  ( 4.458734125000001214, -67.89583333196773651, 2.574251347313718519 ) ) ;
#26712=CARTESIAN_POINT ( 'NONE',  ( 2.500000000000002220, -1.666666666666663410, 4.330127018922192761 ) ) ;
#26714=CARTESIAN_POINT ( 'NONE',  ( -6.972266317189433020E-16, -99.12499999726880162, -5.000000000000000000 ) ) ;
#26715=CARTESIAN_POINT ( 'NONE',  ( 9.457646018065525792E-16, -58.06249999863440081, 5.148502694627439702 ) ) ;
#26716=CARTESIAN_POINT ( 'NONE',  ( 5.000000000000000000, -92.29166666393547303, -2.886751345948129988 ) ) ;
#26718=CARTESIAN_POINT ( 'NONE',  ( 5.000000000000000000, -56.41666666666667140, -2.886751345948130876 ) ) ;
#26720=CARTESIAN_POINT ( 'NONE',  ( -2.499999999999996447, -90.70833333060214443, 4.330127018922195425 ) ) ;
#26721=CARTESIAN_POINT ( 'NONE',  ( 1.060575238724906964E-15, -47.75000000000000000, 5.773502691896257311 ) ) ;
#26722=CARTESIAN_POINT ( 'NONE',  ( 3.044556291839386294E-14, 18.75000000000000355, -5.000000000000000000 ) ) ;
#26725=CARTESIAN_POINT ( 'NONE',  ( 4.458734124999999437, -107.8124999986343937, -5.460374474430324690E-16 ) ) ;
#26726=CARTESIAN_POINT ( 'NONE',  ( -4.458734124999999437, -0.5624999986344053626, 0.000000000000000000 ) ) ;
#26742=CARTESIAN_POINT ( 'NONE',  ( 4.458734124999999437, -32.06249999863440792, -5.460374474430324690E-16 ) ) ;
#26749=CARTESIAN_POINT ( 'NONE',  ( 1.339745962155612702, -70.16965819600731891, -5.000000000000000000 ) ) ;
#26752=CARTESIAN_POINT ( 'NONE',  ( 4.458734124999999437, -76.06249999863440792, -5.460374474430324690E-16 ) ) ;
#26755=CARTESIAN_POINT ( 'NONE',  ( 0.000000000000000000, -120.0000000000000000, 0.000000000000000000 ) ) ;
#26756=( BOUNDED_CURVE ( )  B_SPLINE_CURVE ( 2, ( #46699, #21943, #32858, #42499, #56370, #8725, #18055, #37676, #33177 ),
 .UNSPECIFIED., .F., .F. ) 
 B_SPLINE_CURVE_WITH_KNOTS ( ( 3, 2, 2, 2, 3 ),
 ( 0.6982142857142856762, 0.6988095238095237693, 0.6999999999999999556, 0.7011904761904761418, 0.7017857142857142350 ),
 .UNSPECIFIED. ) 
 CURVE ( )  GEOMETRIC_REPRESENTATION_ITEM ( )  RATIONAL_B_SPLINE_CURVE ( ( 0.9330127018922194093, 0.9330127018922194093, 1.000000000000000000, 0.8660254037844387076, 1.000000000000000000, 0.8660254037844387076, 1.000000000000000000, 0.9330127018922194093, 0.9330127018922194093 ) ) 
 REPRESENTATION_ITEM ( '' )  );
#26757=DIRECTION ( 'NONE',  ( -0.000000000000000000, 1.000000000000000000, -0.000000000000000000 ) ) ;
#26759=CARTESIAN_POINT ( 'NONE',  ( 4.458734124999999437, -7.062499998634404363, -5.460374474430324690E-16 ) ) ;
#26760=ORIENTED_EDGE ( 'NONE', *, *, #40084, .T. ) ;
#26761=CARTESIAN_POINT ( 'NONE',  ( 1.975475456537005874E-15, 19.37500000273118772, 5.000000000000000000 ) ) ;
#26762=CARTESIAN_POINT ( 'NONE',  ( -2.229367062500000163, -6.729166665301073103, -3.861377020970580443 ) ) ;
#26763=FACE_OUTER_BOUND ( 'NONE', #13542, .T. ) ;
#26765=CARTESIAN_POINT ( 'NONE',  ( 5.000000000000000000, -64.50000000000000000, -6.123233995736766282E-16 ) ) ;
#26769=CARTESIAN_POINT ( 'NONE',  ( -2.229367062500000163, -85.47916666530107932, -3.861377020970580443 ) ) ;
#26770=CARTESIAN_POINT ( 'NONE',  ( -4.458734124999999437, -3.312499998634407916, 0.000000000000000000 ) ) ;
#26773=CARTESIAN_POINT ( 'NONE',  ( 2.500000000000002220, -51.66666666666666430, 4.330127018922192761 ) ) ;
#26774=CARTESIAN_POINT ( 'NONE',  ( 5.000000000000000000, -30.37499999726881228, -6.123233995736766282E-16 ) ) ;
#26776=CARTESIAN_POINT ( 'NONE',  ( -3.152548672688508926E-16, 23.43750000136559564, -5.148502694627439702 ) ) ;
#26777=CARTESIAN_POINT ( 'NONE',  ( -1.339745962155613812, -21.08034179853029144, -5.000000000000000000 ) ) ;
#26779=CARTESIAN_POINT ( 'NONE',  ( -4.458734124999999437, -50.31249999863440792, 0.000000000000000000 ) ) ;
#26780=CARTESIAN_POINT ( 'NONE',  ( 9.457646018065525792E-16, -35.31249999863440792, 5.148502694627439702 ) ) ;
#26782=CARTESIAN_POINT ( 'NONE',  ( 2.500000000000002220, 15.33333333333333215, 4.330127018922192761 ) ) ;
#26784=VECTOR ( 'NONE', #27771, 1000.000000000000000 ) ;
#26785=DIRECTION ( 'NONE',  ( -0.000000000000000000, 1.000000000000000000, -0.000000000000000000 ) ) ;
#26786=CARTESIAN_POINT ( 'NONE',  ( -4.458734124999999437, -40.31249999863440081, 0.000000000000000000 ) ) ;
#26787=CARTESIAN_POINT ( 'NONE',  ( 5.000000000000000888, -80.45833333060213022, 2.886751345948126879 ) ) ;
#26789=CARTESIAN_POINT ( 'NONE',  ( 2.499999999999998668, -65.20833333060213022, -4.330127018922193649 ) ) ;
#26791=CARTESIAN_POINT ( 'NONE',  ( 2.229367062500001939, -83.22916666530106511, 3.861377020970579999 ) ) ;
#26794=CARTESIAN_POINT ( 'NONE',  ( -5.000000000000000000, -34.00000000000000000, 0.000000000000000000 ) ) ;
#26798=ORIENTED_EDGE ( 'NONE', *, *, #8658, .F. ) ;
#26799=CARTESIAN_POINT ( 'NONE',  ( -4.458734124999998549, -90.22916666530106511, 2.574251347313722516 ) ) ;
#26800=CARTESIAN_POINT ( 'NONE',  ( -4.458734124999999437, 11.35416666803225993, -2.574251347313719407 ) ) ;
#26801=CARTESIAN_POINT ( 'NONE',  ( 1.060575238724906964E-15, 14.37500000273118594, 5.773502691896257311 ) ) ;
#26805=EDGE_CURVE ( 'NONE', #62283, #33389, #61977, .T. ) ;
#26807=CARTESIAN_POINT ( 'NONE',  ( -2.499999999999996447, 20.16666666666666430, 4.330127018922195425 ) ) ;
#26808=CARTESIAN_POINT ( 'NONE',  ( -6.972266317189433020E-16, -107.2499999999999858, -5.000000000000000000 ) ) ;
#26809=CARTESIAN_POINT ( 'NONE',  ( 5.000000000000000888, -33.45833333060215153, 2.886751345948126879 ) ) ;
#26810=EDGE_CURVE ( 'NONE', #25630, #7254, #22910, .T. ) ;
#26811=CARTESIAN_POINT ( 'NONE',  ( 2.500000000000002220, -11.54166666393547835, 4.330127018922192761 ) ) ;
#26815=CARTESIAN_POINT ( 'NONE',  ( -4.458734124999999437, -14.56249999863440436, 0.000000000000000000 ) ) ;
#26820=AXIS2_PLACEMENT_3D ( 'NONE', #2446, #13662, #56796 ) ;
#26823=EDGE_CURVE ( 'NONE', #45741, #39400, #29067, .T. ) ;
#26824=EDGE_CURVE ( 'NONE', #29833, #57689, #53656, .T. ) ;
#26829=VERTEX_POINT ( 'NONE', #29198 ) ;
#26830=CARTESIAN_POINT ( 'NONE',  ( -4.458734124999998549, -63.47916666530106511, 2.574251347313722516 ) ) ;
#26832=CARTESIAN_POINT ( 'NONE',  ( -4.999999999999998224, -85.91666666666667140, 2.886751345948131764 ) ) ;
#26834=EDGE_CURVE ( 'NONE', #44276, #1660, #59916, .T. ) ;
#26835=VERTEX_POINT ( 'NONE', #33722 ) ;
#26842=ORIENTED_EDGE ( 'NONE', *, *, #10250, .T. ) ;
#26844=CARTESIAN_POINT ( 'NONE',  ( -6.972266317189433020E-16, -76.24999999999998579, -5.000000000000000000 ) ) ;
#26845=CARTESIAN_POINT ( 'NONE',  ( 4.458734125000001214, 6.104166668032262599, 2.574251347313718519 ) ) ;
#26848=CARTESIAN_POINT ( 'NONE',  ( 1.339745962155615144, -78.58034179853028434, 4.999999999999999112 ) ) ;
#26850=ORIENTED_EDGE ( 'NONE', *, *, #15034, .F. ) ;
#26851=CARTESIAN_POINT ( 'NONE',  ( 4.458734124999998549, -69.72916666530107932, -2.574251347313721627 ) ) ;
#26853=CARTESIAN_POINT ( 'NONE',  ( 4.458734124999998549, 14.27083333469892779, -2.574251347313721627 ) ) ;
#26855=CARTESIAN_POINT ( 'NONE',  ( 2.493747252781420335E-13, -42.25000000000000711, -5.000000000000000000 ) ) ;
#26856=CARTESIAN_POINT ( 'NONE',  ( 4.458734125000001214, -54.14583333196773651, 2.574251347313718519 ) ) ;
#26857=CARTESIAN_POINT ( 'NONE',  ( -2.500000000000000444, -13.04166666393548013, -4.330127018922193649 ) ) ;
#26861=CARTESIAN_POINT ( 'NONE',  ( 2.229367062500001939, -21.22916666530107221, 3.861377020970579999 ) ) ;
#26864=CARTESIAN_POINT ( 'NONE',  ( 4.458734125000001214, -108.8958333319677365, 2.574251347313718519 ) ) ;
#26867=CARTESIAN_POINT ( 'NONE',  ( 2.229367062499998831, -100.8958333319677365, -3.861377020970580887 ) ) ;
#26869=CARTESIAN_POINT ( 'NONE',  ( 4.458734124999998549, -24.72916666530106866, -2.574251347313721627 ) ) ;
#26870=CARTESIAN_POINT ( 'NONE',  ( -3.535250795749689387E-16, -65.12499999726881583, -5.773502691896257311 ) ) ;
#26873=CARTESIAN_POINT ( 'NONE',  ( 2.229367062499998831, -25.64583333196773651, -3.861377020970580887 ) ) ;
#26874=CARTESIAN_POINT ( 'NONE',  ( 4.458734125000000326, -72.14583333196773651, 2.574251347313718519 ) ) ;
#26875=CARTESIAN_POINT ( 'NONE',  ( -2.500000000000000444, -40.04166666393548013, -4.330127018922193649 ) ) ;
#26878=CARTESIAN_POINT ( 'NONE',  ( -2.499999999999996447, -15.83333333333333037, 4.330127018922195425 ) ) ;
#26886=CARTESIAN_POINT ( 'NONE',  ( 1.339745962155615144, -76.58034179853029855, 4.999999999999999112 ) ) ;
#26888=CARTESIAN_POINT ( 'NONE',  ( 1.339745962155615144, 1.419658201469705672, 4.999999999999999112 ) ) ;
#26893=ORIENTED_EDGE ( 'NONE', *, *, #9368, .F. ) ;
#26900=ORIENTED_EDGE ( 'NONE', *, *, #1416, .T. ) ;
#26905=EDGE_CURVE ( 'NONE', #14930, #53159, #14096, .T. ) ;
#26907=ORIENTED_EDGE ( 'NONE', *, *, #63066, .T. ) ;
#26914=CARTESIAN_POINT ( 'NONE',  ( 2.229367062500001939, -77.97916666530106511, 3.861377020970579999 ) ) ;
#26915=CARTESIAN_POINT ( 'NONE',  ( -2.229367062499996610, 25.85416666803225993, 3.861377020970582219 ) ) ;
#26917=EDGE_LOOP ( 'NONE', ( #31961, #13931, #55545, #62440 ) ) ;
#26918=CARTESIAN_POINT ( 'NONE',  ( -4.999999999999998224, 5.208333336064518981, 2.886751345948131764 ) ) ;
#26920=VECTOR ( 'NONE', #20332, 1000.000000000000000 ) ;
#26923=CARTESIAN_POINT ( 'NONE',  ( -6.972266317189433020E-16, 15.87500000273118417, -5.000000000000000000 ) ) ;
#26925=CARTESIAN_POINT ( 'NONE',  ( -3.152548672688508926E-16, -52.56249999863440792, -5.148502694627439702 ) ) ;
#26927=CARTESIAN_POINT ( 'NONE',  ( 4.458734125000001214, 26.10416666803225993, 2.574251347313718519 ) ) ;
#26928=CARTESIAN_POINT ( 'NONE',  ( 5.000000000000000000, -106.4166666666666572, -2.886751345948129988 ) ) ;
#26930=CARTESIAN_POINT ( 'NONE',  ( -2.229367062500000163, -40.72916666530107221, -3.861377020970580443 ) ) ;
#26931=CARTESIAN_POINT ( 'NONE',  ( -3.535250795749689387E-16, -0.1249999972688133065, -5.773502691896257311 ) ) ;
#26935=CARTESIAN_POINT ( 'NONE',  ( 5.000000000000000888, 24.41666666666666785, 2.886751345948126879 ) ) ;
#26936=CARTESIAN_POINT ( 'NONE',  ( -2.229367062500000163, -101.4791666653010651, -3.861377020970580443 ) ) ;
#26937=( BOUNDED_CURVE ( )  B_SPLINE_CURVE ( 2, ( #49922, #739, #45104, #20676, #15842, #19703, #54446, #59595, #5875 ),
 .UNSPECIFIED., .F., .F. ) 
 B_SPLINE_CURVE_WITH_KNOTS ( ( 3, 2, 2, 2, 3 ),
 ( 0.5446428571428570953, 0.5452380952380951884, 0.5464285714285713746, 0.5476190476190476719, 0.5482142857142857650 ),
 .UNSPECIFIED. ) 
 CURVE ( )  GEOMETRIC_REPRESENTATION_ITEM ( )  RATIONAL_B_SPLINE_CURVE ( ( 0.9330127018922194093, 0.9330127018922194093, 1.000000000000000000, 0.8660254037844387076, 1.000000000000000000, 0.8660254037844387076, 1.000000000000000000, 0.9330127018922194093, 0.9330127018922194093 ) ) 
 REPRESENTATION_ITEM ( '' )  );
#26938=CARTESIAN_POINT ( 'NONE',  ( -3.152548672688508926E-16, -5.812499998634404363, -5.148502694627439702 ) ) ;
#26939=VERTEX_POINT ( 'NONE', #926 ) ;
#26940=DIRECTION ( 'NONE',  ( -0.000000000000000000, 1.000000000000000000, -0.000000000000000000 ) ) ;
#26941=CARTESIAN_POINT ( 'NONE',  ( -2.499999999999996447, -35.70833333060213732, 4.330127018922195425 ) ) ;
#26942=CARTESIAN_POINT ( 'NONE',  ( 2.229367062499998831, -93.64583333196772230, -3.861377020970580887 ) ) ;
#26944=CARTESIAN_POINT ( 'NONE',  ( 2.229367062500001939, -89.22916666530106511, 3.861377020970579999 ) ) ;
#26946=DIRECTION ( 'NONE',  ( 0.000000000000000000, 0.000000000000000000, 1.000000000000000000 ) ) ;
#26948=CARTESIAN_POINT ( 'NONE',  ( 2.229367062499998831, -9.645833331967738289, -3.861377020970580887 ) ) ;
#26949=CARTESIAN_POINT ( 'NONE',  ( -2.229367062500000163, 14.27083333469892601, -3.861377020970580443 ) ) ;
#26950=CARTESIAN_POINT ( 'NONE',  ( 2.229367062499998831, -53.89583333196773651, -3.861377020970580887 ) ) ;
#26957=CARTESIAN_POINT ( 'NONE',  ( -4.458734124999998549, -82.22916666530107932, 2.574251347313722516 ) ) ;
#26958=CARTESIAN_POINT ( 'NONE',  ( 2.229367062500001939, 26.77083333469892423, 3.861377020970579999 ) ) ;
#26961=CARTESIAN_POINT ( 'NONE',  ( -5.000000000000000000, -94.08333333333332860, -2.886751345948128211 ) ) ;
#26964=CARTESIAN_POINT ( 'NONE',  ( 5.000000000000000000, -63.50000000000000000, -6.123233995736766282E-16 ) ) ;
#26965=CYLINDRICAL_SURFACE ( 'NONE', #20296, 5.000000000000000000 ) ;
#26968=CARTESIAN_POINT ( 'NONE',  ( -5.000000000000000000, 27.99999999999999645, 0.000000000000000000 ) ) ;
#26969=CARTESIAN_POINT ( 'NONE',  ( -1.339745962155613812, -107.0803417985302843, -5.000000000000000000 ) ) ;
#26975=ORIENTED_EDGE ( 'NONE', *, *, #55500, .T. ) ;
#26976=CARTESIAN_POINT ( 'NONE',  ( 5.000000000000000000, -28.49999999999999645, -6.123233995736766282E-16 ) ) ;
#26981=CARTESIAN_POINT ( 'NONE',  ( -2.229367062499996610, -53.39583333196773651, 3.861377020970582219 ) ) ;
#26982=CARTESIAN_POINT ( 'NONE',  ( -6.972266317189433020E-16, -96.25000000000000000, -5.000000000000000000 ) ) ;
#26990=CARTESIAN_POINT ( 'NONE',  ( -3.152548672688508926E-16, -100.8124999986343937, -5.148502694627439702 ) ) ;
#26991=CARTESIAN_POINT ( 'NONE',  ( 1.339745962155641346, -2.294658198738521726, -4.999999999999983125 ) ) ;
#26996=CARTESIAN_POINT ( 'NONE',  ( 4.458734125000001214, 0.1041666680322607674, 2.574251347313718519 ) ) ;
#26997=CARTESIAN_POINT ( 'NONE',  ( 4.458734125000000326, -93.14583333196773651, 2.574251347313718519 ) ) ;
#26999=CARTESIAN_POINT ( 'NONE',  ( -4.458734124999998549, -25.47916666530106866, 2.574251347313722516 ) ) ;
#27000=CARTESIAN_POINT ( 'NONE',  ( 1.975475456537005874E-15, -46.74999999999999289, 5.000000000000000000 ) ) ;
#27006=CARTESIAN_POINT ( 'NONE',  ( 4.458734124999998549, 12.02083333469892601, -2.574251347313721627 ) ) ;
#27007=ORIENTED_EDGE ( 'NONE', *, *, #11313, .F. ) ;
#27008=CARTESIAN_POINT ( 'NONE',  ( 1.975475456537005874E-15, -4.749999999999999112, 5.000000000000000000 ) ) ;
#27010=CARTESIAN_POINT ( 'NONE',  ( -3.535250795749689387E-16, -88.25000000000000000, -5.773502691896257311 ) ) ;
#27011=CARTESIAN_POINT ( 'NONE',  ( 2.229367062500001939, -25.97916666530106866, 3.861377020970579999 ) ) ;
#27012=CARTESIAN_POINT ( 'NONE',  ( 4.458734124999998549, -72.97916666530107932, -2.574251347313721627 ) ) ;
#27014=DIRECTION ( 'NONE',  ( -0.000000000000000000, 1.000000000000000000, -0.000000000000000000 ) ) ;
#27015=CARTESIAN_POINT ( 'NONE',  ( -6.972266317189433020E-16, 14.74999999999999822, -5.000000000000000000 ) ) ;
#27016=( BOUNDED_CURVE ( )  B_SPLINE_CURVE ( 2, ( #40393, #11445, #30099, #60034, #45543, #867, #41030, #1503, #29779 ),
 .UNSPECIFIED., .F., .F. ) 
 B_SPLINE_CURVE_WITH_KNOTS ( ( 3, 2, 2, 2, 3 ),
 ( 0.02678571428571428770, 0.02738095238095238082, 0.02857142857142857054, 0.02976190476190476025, 0.03035714285714285685 ),
 .UNSPECIFIED. ) 
 CURVE ( )  GEOMETRIC_REPRESENTATION_ITEM ( )  RATIONAL_B_SPLINE_CURVE ( ( 0.9330127018922194093, 0.9330127018922195203, 1.000000000000000000, 0.8660254037844387076, 1.000000000000000000, 0.8660254037844387076, 1.000000000000000000, 0.9330127018922194093, 0.9330127018922194093 ) ) 
 REPRESENTATION_ITEM ( '' )  );
#27018=CARTESIAN_POINT ( 'NONE',  ( -5.000000000000000000, -51.87499999726881583, 0.000000000000000000 ) ) ;
#27019=CARTESIAN_POINT ( 'NONE',  ( 2.499999999999998668, -24.33333333333333215, -4.330127018922193649 ) ) ;
#27020=CARTESIAN_POINT ( 'NONE',  ( -3.152548672688508926E-16, 8.437500001365595637, -5.148502694627439702 ) ) ;
#27022=DIRECTION ( 'NONE',  ( -0.000000000000000000, 1.000000000000000000, -0.000000000000000000 ) ) ;
#27024=CARTESIAN_POINT ( 'NONE',  ( 2.229367062500001939, -72.97916666530107932, 3.861377020970579999 ) ) ;
#27026=CARTESIAN_POINT ( 'NONE',  ( 5.000000000000000000, -0.4166666666666659080, -2.886751345948129988 ) ) ;
#27029=CARTESIAN_POINT ( 'NONE',  ( 4.458734125000001214, -64.89583333196773651, 2.574251347313718519 ) ) ;
#27030=CARTESIAN_POINT ( 'NONE',  ( -4.999999999999999112, -94.79166666393547303, 2.886751345948131764 ) ) ;
#27036=CARTESIAN_POINT ( 'NONE',  ( -2.500000000000000444, -47.16666666666666430, -4.330127018922193649 ) ) ;
#27039=ORIENTED_EDGE ( 'NONE', *, *, #28102, .F. ) ;
#27040=CARTESIAN_POINT ( 'NONE',  ( 0.000000000000000000, -120.0000000000000000, 5.000000000000000000 ) ) ;
#27041=CARTESIAN_POINT ( 'NONE',  ( -3.152548672688508926E-16, -2.812499998634407028, -5.148502694627439702 ) ) ;
#27045=CARTESIAN_POINT ( 'NONE',  ( -1.339745962155610925, -4.669658196007337558, 5.000000000000000000 ) ) ;
#27049=CARTESIAN_POINT ( 'NONE',  ( 2.500000000000002220, -81.66666666666667140, 4.330127018922192761 ) ) ;
#27055=CARTESIAN_POINT ( 'NONE',  ( 2.229367062500001939, -33.22916666530106511, 3.861377020970579999 ) ) ;
#27056=CARTESIAN_POINT ( 'NONE',  ( -2.499999999999996447, -86.83333333333332860, 4.330127018922195425 ) ) ;
#27065=CARTESIAN_POINT ( 'NONE',  ( -2.229367062499996610, -78.39583333196773651, 3.861377020970582219 ) ) ;
#27071=CARTESIAN_POINT ( 'NONE',  ( 2.229367062499998831, -7.895833331967735624, -3.861377020970580887 ) ) ;
#27075=CARTESIAN_POINT ( 'NONE',  ( -4.458734124999998549, -8.479166665301073991, 2.574251347313722516 ) ) ;
#27081=CARTESIAN_POINT ( 'NONE',  ( 2.229367062500001939, 28.77083333469892779, 3.861377020970579999 ) ) ;
#27082=VERTEX_POINT ( 'NONE', #60088 ) ;
#27083=CARTESIAN_POINT ( 'NONE',  ( 2.229367062500001939, -87.97916666530107932, 3.861377020970579999 ) ) ;
#27085=CARTESIAN_POINT ( 'NONE',  ( 2.229367062499998831, -8.645833331967736513, -3.861377020970580887 ) ) ;
#27089=CARTESIAN_POINT ( 'NONE',  ( -5.000000000000000000, -32.95833333060215153, -2.886751345948128211 ) ) ;
#27090=CARTESIAN_POINT ( 'NONE',  ( 0.000000000000000000, -120.0000000000000000, 5.000000000000000000 ) ) ;
#27091=CARTESIAN_POINT ( 'NONE',  ( -2.229367062499996610, 25.85416666803225993, 3.861377020970582219 ) ) ;
#27092=CARTESIAN_POINT ( 'NONE',  ( 1.975475456537005874E-15, -7.750000000000000000, 5.000000000000000000 ) ) ;
#27094=CARTESIAN_POINT ( 'NONE',  ( -2.229367062500000163, -51.47916666530107221, -3.861377020970580443 ) ) ;
#27095=CARTESIAN_POINT ( 'NONE',  ( 2.229367062500001939, -37.22916666530107221, 3.861377020970579999 ) ) ;
#27098=CARTESIAN_POINT ( 'NONE',  ( -5.000000000000000000, 13.00000000000000178, 0.000000000000000000 ) ) ;
#27101=EDGE_CURVE ( 'NONE', #26096, #62985, #35673, .T. ) ;
#27102=CARTESIAN_POINT ( 'NONE',  ( -2.229367062499996610, -48.14583333196772941, 3.861377020970582219 ) ) ;
#27103=CARTESIAN_POINT ( 'NONE',  ( -3.535250795749689387E-16, -79.12499999726881583, -5.773502691896257311 ) ) ;
#27105=AXIS2_PLACEMENT_3D ( 'NONE', #12906, #32529, #27704 ) ;
#27107=CARTESIAN_POINT ( 'NONE',  ( -5.000000000000000000, -63.87499999726880873, 0.000000000000000000 ) ) ;
#27108=EDGE_CURVE ( 'NONE', #1919, #7754, #35001, .T. ) ;
#27109=CARTESIAN_POINT ( 'NONE',  ( -2.229367062500000163, -85.72916666530107932, -3.861377020970580443 ) ) ;
#27111=CARTESIAN_POINT ( 'NONE',  ( 1.060575238724906964E-15, -30.75000000000000000, 5.773502691896257311 ) ) ;
#27116=CARTESIAN_POINT ( 'NONE',  ( 2.229367062500001939, -91.97916666530106511, 3.861377020970579999 ) ) ;
#27117=CARTESIAN_POINT ( 'NONE',  ( 2.229367062500001939, 15.77083333469892601, 3.861377020970579999 ) ) ;
#27118=CARTESIAN_POINT ( 'NONE',  ( -5.000000000000000000, 17.04166666939785202, -2.886751345948128211 ) ) ;
#27119=CARTESIAN_POINT ( 'NONE',  ( 1.975475456537005874E-15, -34.62499999726880873, 5.000000000000000000 ) ) ;
#27123=CARTESIAN_POINT ( 'NONE',  ( 5.000000000000000000, -78.50000000000000000, -6.123233995736766282E-16 ) ) ;
#27124=CARTESIAN_POINT ( 'NONE',  ( -6.972266317189433020E-16, -13.12499999726881050, -5.000000000000000000 ) ) ;
#27125=CARTESIAN_POINT ( 'NONE',  ( -2.500000000000000444, -13.04166666393548013, -4.330127018922193649 ) ) ;
#27128=CARTESIAN_POINT ( 'NONE',  ( 1.975475456537005874E-15, -88.62499999726880162, 5.000000000000000000 ) ) ;
#27130=CARTESIAN_POINT ( 'NONE',  ( -2.229367062500000163, -17.72916666530106866, -3.861377020970580443 ) ) ;
#27142=VERTEX_POINT ( 'NONE', #30152 ) ;
#27143=CARTESIAN_POINT ( 'NONE',  ( -4.458734124999999437, -64.64583333196772230, -2.574251347313719407 ) ) ;
#27148=FACE_OUTER_BOUND ( 'NONE', #16472, .T. ) ;
#27151=ORIENTED_EDGE ( 'NONE', *, *, #31884, .F. ) ;
#27152=AXIS2_PLACEMENT_3D ( 'NONE', #63124, #5204, #49267 ) ;
#27154=CARTESIAN_POINT ( 'NONE',  ( -4.458734124999999437, 6.687500001365593860, 0.000000000000000000 ) ) ;
#27158=CARTESIAN_POINT ( 'NONE',  ( 1.975475456537005874E-15, -23.75000000000000000, 5.000000000000000000 ) ) ;
#27159=ORIENTED_EDGE ( 'NONE', *, *, #49870, .F. ) ;
#27160=CARTESIAN_POINT ( 'NONE',  ( 4.458734125000000326, -71.89583333196773651, 2.574251347313718519 ) ) ;
#27162=CARTESIAN_POINT ( 'NONE',  ( -3.152548672688508926E-16, 11.43750000136559386, -5.148502694627439702 ) ) ;
#27163=EDGE_CURVE ( 'NONE', #42248, #59111, #2804, .T. ) ;
#27166=CARTESIAN_POINT ( 'NONE',  ( 9.457646018065525792E-16, -55.31249999863439371, 5.148502694627439702 ) ) ;
#27167=CARTESIAN_POINT ( 'NONE',  ( 5.000000000000000000, -16.37499999726881228, -6.123233995736766282E-16 ) ) ;
#27168=CARTESIAN_POINT ( 'NONE',  ( -2.500000000000000444, -19.16666666666666430, -4.330127018922193649 ) ) ;
#27169=CARTESIAN_POINT ( 'NONE',  ( 6.123233995736766282E-16, -120.0000000000000000, -5.000000000000000000 ) ) ;
#27170=CARTESIAN_POINT ( 'NONE',  ( -4.458734124999998549, -34.22916666530107221, 2.574251347313722516 ) ) ;
#27171=CARTESIAN_POINT ( 'NONE',  ( -4.458734124999999437, -23.64583333196773651, -2.574251347313719407 ) ) ;
#27174=CARTESIAN_POINT ( 'NONE',  ( -5.000000000000000000, 28.99999999999999645, 0.000000000000000000 ) ) ;
#27177=CARTESIAN_POINT ( 'NONE',  ( -4.458734124999999437, -103.5624999986344079, 0.000000000000000000 ) ) ;
#27178=CARTESIAN_POINT ( 'NONE',  ( 4.458734124999998549, -28.72916666530107221, -2.574251347313721627 ) ) ;
#27179=CARTESIAN_POINT ( 'NONE',  ( 5.000000000000000888, -63.45833333060215153, 2.886751345948126879 ) ) ;
#27183=CARTESIAN_POINT ( 'NONE',  ( -3.152548672688508926E-16, -30.56249999863440436, -5.148502694627439702 ) ) ;
#27185=CARTESIAN_POINT ( 'NONE',  ( 4.458734124999998549, -71.97916666530107932, -2.574251347313721627 ) ) ;
#27187=CARTESIAN_POINT ( 'NONE',  ( 1.339745962155615144, -32.58034179853029144, 4.999999999999999112 ) ) ;
#27189=CARTESIAN_POINT ( 'NONE',  ( 1.060575238724906964E-15, -15.75000000000000178, 5.773502691896257311 ) ) ;
#27191=EDGE_LOOP ( 'NONE', ( #10978, #23086, #57197, #1476 ) ) ;
#27195=CARTESIAN_POINT ( 'NONE',  ( 5.000000000000000000, -81.37499999726881583, -6.123233995736766282E-16 ) ) ;
#27201=CARTESIAN_POINT ( 'NONE',  ( 1.975475456537005874E-15, -62.62499999726880873, 5.000000000000000000 ) ) ;
#27204=ORIENTED_EDGE ( 'NONE', *, *, #22999, .T. ) ;
#27212=ORIENTED_EDGE ( 'NONE', *, *, #18886, .F. ) ;
#27220=CARTESIAN_POINT ( 'NONE',  ( -4.999999999999998224, 23.20833333606451632, 2.886751345948131764 ) ) ;
#27222=CARTESIAN_POINT ( 'NONE',  ( -2.229367062499996610, -78.14583333196773651, 3.861377020970582219 ) ) ;
#27223=CARTESIAN_POINT ( 'NONE',  ( 4.458734125000001214, 22.10416666803225993, 2.574251347313718519 ) ) ;
#27224=ORIENTED_EDGE ( 'NONE', *, *, #56265, .F. ) ;
#27229=CARTESIAN_POINT ( 'NONE',  ( 2.499999999999998668, -74.20833333060214443, -4.330127018922193649 ) ) ;
#27232=CARTESIAN_POINT ( 'NONE',  ( -3.152548672688508926E-16, -55.56249999863440081, -5.148502694627439702 ) ) ;
#27235=CARTESIAN_POINT ( 'NONE',  ( -5.000000000000000000, -109.0833333333333286, -2.886751345948128211 ) ) ;
#27237=DIRECTION ( 'NONE',  ( -0.000000000000000000, 1.000000000000000000, -0.000000000000000000 ) ) ;
#27238=EDGE_CURVE ( 'NONE', #15898, #51084, #31151, .T. ) ;
#27239=CARTESIAN_POINT ( 'NONE',  ( -4.458734124999999437, -36.56249999863440792, 0.000000000000000000 ) ) ;
#27240=CARTESIAN_POINT ( 'NONE',  ( -4.999999999999999112, 2.208333336064519870, 2.886751345948131764 ) ) ;
#27243=CARTESIAN_POINT ( 'NONE',  ( -4.458734124999999437, -101.3958333319677365, -2.574251347313719407 ) ) ;
#27244=CARTESIAN_POINT ( 'NONE',  ( -4.458734124999997661, -3.479166665301069994, 2.574251347313722516 ) ) ;
#27245=ORIENTED_EDGE ( 'NONE', *, *, #57454, .F. ) ;
#27247=CARTESIAN_POINT ( 'NONE',  ( -3.152548672688508926E-16, -93.56249999863439371, -5.148502694627439702 ) ) ;
#27249=CARTESIAN_POINT ( 'NONE',  ( 2.229367062500001939, -85.22916666530107932, 3.861377020970579999 ) ) ;
#27253=CARTESIAN_POINT ( 'NONE',  ( 2.229367062499998831, -10.64583333196773829, -3.861377020970580887 ) ) ;
#27254=CARTESIAN_POINT ( 'NONE',  ( 9.457646018065525792E-16, 14.68750000136559208, 5.148502694627439702 ) ) ;
#27255=CARTESIAN_POINT ( 'NONE',  ( 2.229367062499998831, -51.89583333196773651, -3.861377020970580887 ) ) ;
#27260=CARTESIAN_POINT ( 'NONE',  ( 1.339745962155612702, -106.1696581960073331, -5.000000000000000000 ) ) ;
#27262=ORIENTED_EDGE ( 'NONE', *, *, #46048, .F. ) ;
#27265=EDGE_CURVE ( 'NONE', #100, #16461, #46872, .T. ) ;
#27266=FACE_OUTER_BOUND ( 'NONE', #40866, .T. ) ;
#27267=CARTESIAN_POINT ( 'NONE',  ( 4.458734125000001214, -78.89583333196772230, 2.574251347313718519 ) ) ;
#27268=CARTESIAN_POINT ( 'NONE',  ( -4.458734124999998549, 22.52083333469892423, 2.574251347313722516 ) ) ;
#27272=CARTESIAN_POINT ( 'NONE',  ( -1.339745962155613812, -58.08034179853029144, -5.000000000000000000 ) ) ;
#27275=CARTESIAN_POINT ( 'NONE',  ( 1.060575238724906964E-15, -63.75000000000000000, 5.773502691896257311 ) ) ;
#27276=FACE_OUTER_BOUND ( 'NONE', #26400, .T. ) ;
#27281=CARTESIAN_POINT ( 'NONE',  ( 0.000000000000000000, -120.0000000000000000, 0.000000000000000000 ) ) ;
#27284=CARTESIAN_POINT ( 'NONE',  ( 5.000000000000000888, 18.41666666666666430, 2.886751345948126879 ) ) ;
#27288=VERTEX_POINT ( 'NONE', #12454 ) ;
#27294=CARTESIAN_POINT ( 'NONE',  ( -3.152548672688508926E-16, -52.81249999863440792, -5.148502694627439702 ) ) ;
#27303=CARTESIAN_POINT ( 'NONE',  ( -2.229367062499996610, -101.3958333319677365, 3.861377020970582219 ) ) ;
#27304=CARTESIAN_POINT ( 'NONE',  ( 1.339745962155615144, -2.705341801261480050, 4.999999999999999112 ) ) ;
#27305=ORIENTED_EDGE ( 'NONE', *, *, #58230, .F. ) ;
#27310=CARTESIAN_POINT ( 'NONE',  ( 4.458734125000001214, -6.895833331967734736, 2.574251347313718519 ) ) ;
#27311=CARTESIAN_POINT ( 'NONE',  ( 2.229367062500001939, -94.22916666530106511, 3.861377020970579999 ) ) ;
#27313=CARTESIAN_POINT ( 'NONE',  ( 4.458734124999998549, -21.97916666530107221, -2.574251347313721627 ) ) ;
#27314=CARTESIAN_POINT ( 'NONE',  ( 0.000000000000000000, -120.0000000000000000, 0.000000000000000000 ) ) ;
#27318=CARTESIAN_POINT ( 'NONE',  ( 0.000000000000000000, -120.0000000000000000, 5.000000000000000000 ) ) ;
#27320=CARTESIAN_POINT ( 'NONE',  ( 9.457646018065525792E-16, 11.68750000136559564, 5.148502694627439702 ) ) ;
#27323=CARTESIAN_POINT ( 'NONE',  ( -4.999999999999999112, -90.91666666666665719, 2.886751345948131764 ) ) ;
#27324=CARTESIAN_POINT ( 'NONE',  ( 9.457646018065525792E-16, -23.06249999863440792, 5.148502694627439702 ) ) ;
#27326=CARTESIAN_POINT ( 'NONE',  ( 4.458734125000001214, -72.14583333196773651, 2.574251347313718519 ) ) ;
#27330=FACE_OUTER_BOUND ( 'NONE', #6438, .T. ) ;
#27331=CARTESIAN_POINT ( 'NONE',  ( -4.458734124999997661, 6.770833334698928674, 2.574251347313722516 ) ) ;
#27332=CARTESIAN_POINT ( 'NONE',  ( 0.000000000000000000, -120.0000000000000000, 0.000000000000000000 ) ) ;
#27335=CARTESIAN_POINT ( 'NONE',  ( -4.458734124999999437, -72.39583333196775072, -2.574251347313719407 ) ) ;
#27337=CARTESIAN_POINT ( 'NONE',  ( 2.499999999999998668, -2.333333333333333037, -4.330127018922193649 ) ) ;
#27339=CARTESIAN_POINT ( 'NONE',  ( -3.152548672688508926E-16, -66.56249999863440792, -5.148502694627439702 ) ) ;
#27340=CARTESIAN_POINT ( 'NONE',  ( -5.000000000000000000, -101.8749999972688158, 0.000000000000000000 ) ) ;
#27341=CARTESIAN_POINT ( 'NONE',  ( 1.339745962155615144, 5.419658201469705894, 4.999999999999999112 ) ) ;
#27343=CARTESIAN_POINT ( 'NONE',  ( -5.000000000000000000, -90.87499999726880162, 0.000000000000000000 ) ) ;
#27345=CARTESIAN_POINT ( 'NONE',  ( -5.000000000000000000, -50.08333333333332149, -2.886751345948128211 ) ) ;
#27346=CARTESIAN_POINT ( 'NONE',  ( -1.339745962155613812, -23.20534180126147916, -5.000000000000000000 ) ) ;
#27351=DIRECTION ( 'NONE',  ( -0.000000000000000000, 1.000000000000000000, -0.000000000000000000 ) ) ;
#27354=ORIENTED_EDGE ( 'NONE', *, *, #38202, .T. ) ;
#27357=ORIENTED_EDGE ( 'NONE', *, *, #19324, .F. ) ;
#27361=CARTESIAN_POINT ( 'NONE',  ( 2.229367062500001939, -35.22916666530107221, 3.861377020970579999 ) ) ;
#27370=CARTESIAN_POINT ( 'NONE',  ( 2.500000000000002220, -70.54166666393547303, 4.330127018922192761 ) ) ;
#27371=CARTESIAN_POINT ( 'NONE',  ( 4.458734125000001214, -85.14583333196773651, 2.574251347313718519 ) ) ;
#27374=CARTESIAN_POINT ( 'NONE',  ( -6.972266317189433020E-16, -64.12499999726880162, -5.000000000000000000 ) ) ;
#27377=CARTESIAN_POINT ( 'NONE',  ( -4.458734124999999437, -37.31249999863440792, 0.000000000000000000 ) ) ;
#27378=CARTESIAN_POINT ( 'NONE',  ( 4.458734124999999437, -9.062499998634406140, -5.460374474430324690E-16 ) ) ;
#27379=VERTEX_POINT ( 'NONE', #22751 ) ;
#27380=( BOUNDED_CURVE ( )  B_SPLINE_CURVE ( 2, ( #17785, #55450, #26807, #46739, #2684, #38001, #17444, #22592, #42189 ),
 .UNSPECIFIED., .F., .F. ) 
 B_SPLINE_CURVE_WITH_KNOTS ( ( 3, 2, 2, 2, 3 ),
 ( 0.06964285714285714524, 0.07023809523809523836, 0.07142857142857142461, 0.07261904761904762473, 0.07321428571428571785 ),
 .UNSPECIFIED. ) 
 CURVE ( )  GEOMETRIC_REPRESENTATION_ITEM ( )  RATIONAL_B_SPLINE_CURVE ( ( 0.9330127018922194093, 0.9330127018922194093, 1.000000000000000000, 0.8660254037844387076, 1.000000000000000000, 0.8660254037844387076, 1.000000000000000000, 0.9330127018922194093, 0.9330127018922194093 ) ) 
 REPRESENTATION_ITEM ( '' )  );
#27382=CARTESIAN_POINT ( 'NONE',  ( 5.000000000000000888, 17.41666666666666430, 2.886751345948126879 ) ) ;
#27383=CARTESIAN_POINT ( 'NONE',  ( -4.458734124999999437, -8.645833331967736513, -2.574251347313719407 ) ) ;
#27388=CARTESIAN_POINT ( 'NONE',  ( 2.229367062499998831, 28.10416666803225993, -3.861377020970580887 ) ) ;
#27390=CARTESIAN_POINT ( 'NONE',  ( -2.229367062499996610, -88.14583333196773651, 3.861377020970582219 ) ) ;
#27392=CARTESIAN_POINT ( 'NONE',  ( 4.458734125000001214, -7.895833331967735624, 2.574251347313718519 ) ) ;
#27393=CARTESIAN_POINT ( 'NONE',  ( -6.972266317189433020E-16, -51.25000000000000000, -5.000000000000000000 ) ) ;
#27395=( BOUNDED_CURVE ( )  B_SPLINE_CURVE ( 2, ( #39401, #15617, #49056, #44552, #45195, #10457, #35234, #5329, #1162 ),
 .UNSPECIFIED., .F., .F. ) 
 B_SPLINE_CURVE_WITH_KNOTS ( ( 3, 2, 2, 2, 3 ),
 ( 0.5410714285714285365, 0.5416666666666666297, 0.5428571428571428159, 0.5440476190476190022, 0.5446428571428570953 ),
 .UNSPECIFIED. ) 
 CURVE ( )  GEOMETRIC_REPRESENTATION_ITEM ( )  RATIONAL_B_SPLINE_CURVE ( ( 0.9330127018922194093, 0.9330127018922194093, 1.000000000000000000, 0.8660254037844387076, 1.000000000000000000, 0.8660254037844387076, 1.000000000000000000, 0.9330127018922194093, 0.9330127018922194093 ) ) 
 REPRESENTATION_ITEM ( '' )  );
#27397=CARTESIAN_POINT ( 'NONE',  ( 5.000000000000000000, -38.29166666393548013, -2.886751345948129988 ) ) ;
#27398=DIRECTION ( 'NONE',  ( 0.000000000000000000, 0.000000000000000000, 1.000000000000000000 ) ) ;
#27399=CARTESIAN_POINT ( 'NONE',  ( -2.229367062499996610, 26.85416666803225993, 3.861377020970582219 ) ) ;
#27400=CARTESIAN_POINT ( 'NONE',  ( -2.500000000000000444, -98.04166666393545881, -4.330127018922193649 ) ) ;
#27402=CARTESIAN_POINT ( 'NONE',  ( 4.458734125000001214, -54.89583333196773651, 2.574251347313718519 ) ) ;
#27405=CARTESIAN_POINT ( 'NONE',  ( 5.000000000000000000, 13.49999999999999822, -6.123233995736766282E-16 ) ) ;
#27408=CARTESIAN_POINT ( 'NONE',  ( 9.457646018065525792E-16, -48.06249999863440081, 5.148502694627439702 ) ) ;
#27409=CARTESIAN_POINT ( 'NONE',  ( -3.535250795749689387E-16, -84.12499999726880162, -5.773502691896257311 ) ) ;
#27410=VECTOR ( 'NONE', #40770, 1000.000000000000000 ) ;
#27412=CARTESIAN_POINT ( 'NONE',  ( 2.499999999999998668, -37.20833333060213732, -4.330127018922193649 ) ) ;
#27414=CARTESIAN_POINT ( 'NONE',  ( -4.458734124999997661, -85.47916666530107932, 2.574251347313722516 ) ) ;
#27416=CARTESIAN_POINT ( 'NONE',  ( -3.535250795749689387E-16, -34.25000000000000711, -5.773502691896257311 ) ) ;
#27417=CARTESIAN_POINT ( 'NONE',  ( 2.499999999999998668, 8.791666669397853795, -4.330127018922193649 ) ) ;
#27420=EDGE_LOOP ( 'NONE', ( #17099, #4121, #48566, #21082 ) ) ;
#27421=CARTESIAN_POINT ( 'NONE',  ( -4.458734124999998549, -94.22916666530106511, 2.574251347313722516 ) ) ;
#27422=CARTESIAN_POINT ( 'NONE',  ( 9.457646018065525792E-16, 13.68750000136559208, 5.148502694627439702 ) ) ;
#27423=CARTESIAN_POINT ( 'NONE',  ( -2.499999999999996447, 18.29166666939785202, 4.330127018922195425 ) ) ;
#27424=CARTESIAN_POINT ( 'NONE',  ( -5.000000000000000000, -34.95833333060213732, -2.886751345948128211 ) ) ;
#27428=CARTESIAN_POINT ( 'NONE',  ( 5.000000000000000000, -81.50000000000000000, -6.123233995736766282E-16 ) ) ;
#27430=CARTESIAN_POINT ( 'NONE',  ( 1.975475456537005874E-15, -12.62499999726881050, 5.000000000000000000 ) ) ;
#27431=CARTESIAN_POINT ( 'NONE',  ( 1.975475456537005874E-15, -109.7499999999999858, 5.000000000000000000 ) ) ;
#27434=CARTESIAN_POINT ( 'NONE',  ( -1.339745962155613812, 13.79465819873852084, -5.000000000000000000 ) ) ;
#27435=CARTESIAN_POINT ( 'NONE',  ( 4.458734124999999437, -20.06249999863440081, -5.460374474430324690E-16 ) ) ;
#27436=CARTESIAN_POINT ( 'NONE',  ( 2.499999999999998668, -107.2083333306021444, -4.330127018922193649 ) ) ;
#27440=EDGE_CURVE ( 'NONE', #52254, #44414, #31912, .T. ) ;
#27444=VERTEX_POINT ( 'NONE', #61987 ) ;
#27446=EDGE_LOOP ( 'NONE', ( #20504, #34162, #45393, #4212 ) ) ;
#27447=CARTESIAN_POINT ( 'NONE',  ( -2.229367062499996610, -66.39583333196773651, 3.861377020970582219 ) ) ;
#27449=CARTESIAN_POINT ( 'NONE',  ( -5.000000000000000000, -5.958333330602149758, -2.886751345948128211 ) ) ;
#27451=( BOUNDED_CURVE ( )  B_SPLINE_CURVE ( 2, ( #55292, #11530, #16679, #45630, #60117, #36300, #15723, #11838, #26013 ),
 .UNSPECIFIED., .F., .F. ) 
 B_SPLINE_CURVE_WITH_KNOTS ( ( 3, 2, 2, 2, 3 ),
 ( 0.6196428571428571619, 0.6202380952380952550, 0.6214285714285714413, 0.6226190476190476275, 0.6232142857142857206 ),
 .UNSPECIFIED. ) 
 CURVE ( )  GEOMETRIC_REPRESENTATION_ITEM ( )  RATIONAL_B_SPLINE_CURVE ( ( 0.9330127018922194093, 0.9330127018922194093, 1.000000000000000000, 0.8660254037844387076, 1.000000000000000000, 0.8660254037844387076, 1.000000000000000000, 0.9330127018922194093, 0.9330127018922194093 ) ) 
 REPRESENTATION_ITEM ( '' )  );
#27459=ADVANCED_FACE ( 'NONE', ( #17907 ), #21801, .T. ) ;
#27462=CARTESIAN_POINT ( 'NONE',  ( -3.152548672688508926E-16, 9.437500001365593860, -5.148502694627439702 ) ) ;
#27466=FACE_OUTER_BOUND ( 'NONE', #16127, .T. ) ;
#27467=ORIENTED_EDGE ( 'NONE', *, *, #53033, .F. ) ;
#27468=CARTESIAN_POINT ( 'NONE',  ( -4.458734124999999437, -69.31249999863439371, 0.000000000000000000 ) ) ;
#27469=DIRECTION ( 'NONE',  ( -0.000000000000000000, 1.000000000000000000, -0.000000000000000000 ) ) ;
#27470=CARTESIAN_POINT ( 'NONE',  ( 2.229367062500001939, 6.020833334698927786, 3.861377020970579999 ) ) ;
#27473=CARTESIAN_POINT ( 'NONE',  ( -4.458734124999999437, -61.56249999863440081, 0.000000000000000000 ) ) ;
#27474=CARTESIAN_POINT ( 'NONE',  ( 5.000000000000000000, -21.37499999726881228, -6.123233995736766282E-16 ) ) ;
#27475=CARTESIAN_POINT ( 'NONE',  ( -2.500000000000000444, -33.04166666393547303, -4.330127018922193649 ) ) ;
#27478=CARTESIAN_POINT ( 'NONE',  ( -4.458734124999998549, -42.22916666530107932, 2.574251347313722516 ) ) ;
#27479=CARTESIAN_POINT ( 'NONE',  ( 4.458734125000000326, -22.14583333196773296, 2.574251347313718519 ) ) ;
#27481=CARTESIAN_POINT ( 'NONE',  ( 1.975475456537005874E-15, -101.7499999999999858, 5.000000000000000000 ) ) ;
#27482=CARTESIAN_POINT ( 'NONE',  ( 2.499999999999998668, 28.66666666666666785, -4.330127018922193649 ) ) ;
#27485=CARTESIAN_POINT ( 'NONE',  ( 4.458734124999999437, -108.0624999986343937, -5.460374474430324690E-16 ) ) ;
#27486=CARTESIAN_POINT ( 'NONE',  ( 9.457646018065525792E-16, -34.06249999863440792, 5.148502694627439702 ) ) ;
#27487=CARTESIAN_POINT ( 'NONE',  ( 1.060575238724906964E-15, -61.62499999726880873, 5.773502691896257311 ) ) ;
#27491=CARTESIAN_POINT ( 'NONE',  ( -2.229367062500000163, -26.47916666530106866, -3.861377020970580443 ) ) ;
#27492=CARTESIAN_POINT ( 'NONE',  ( -2.229367062500000163, -69.72916666530107932, -3.861377020970580443 ) ) ;
#27496=DIRECTION ( 'NONE',  ( 0.000000000000000000, 0.000000000000000000, 1.000000000000000000 ) ) ;
#27497=CARTESIAN_POINT ( 'NONE',  ( -2.499999999999996447, -14.83333333333333037, 4.330127018922195425 ) ) ;
#27499=EDGE_LOOP ( 'NONE', ( #36961, #58750, #60695, #19927 ) ) ;
#27503=CARTESIAN_POINT ( 'NONE',  ( 0.000000000000000000, -120.0000000000000000, 5.000000000000000000 ) ) ;
#27506=CARTESIAN_POINT ( 'NONE',  ( 5.000000000000000888, 25.41666666666666430, 2.886751345948126879 ) ) ;
#27509=CARTESIAN_POINT ( 'NONE',  ( 0.000000000000000000, -120.0000000000000000, 0.000000000000000000 ) ) ;
#27510=FACE_OUTER_BOUND ( 'NONE', #47699, .T. ) ;
#27512=VERTEX_POINT ( 'NONE', #4071 ) ;
#27513=CARTESIAN_POINT ( 'NONE',  ( 1.975475456537005874E-15, -29.62499999726881228, 5.000000000000000000 ) ) ;
#27515=DIRECTION ( 'NONE',  ( -0.000000000000000000, 1.000000000000000000, -0.000000000000000000 ) ) ;
#27521=EDGE_CURVE ( 'NONE', #39916, #62968, #3757, .T. ) ;
#27531=CARTESIAN_POINT ( 'NONE',  ( 4.458734124999999437, -84.81249999863439371, -5.460374474430324690E-16 ) ) ;
#27532=EDGE_CURVE ( 'NONE', #942, #11069, #11427, .T. ) ;
#27533=CARTESIAN_POINT ( 'NONE',  ( 2.229367062500001939, 25.02083333469892779, 3.861377020970579999 ) ) ;
#27534=CARTESIAN_POINT ( 'NONE',  ( -5.000000000000000000, -54.08333333333332860, -2.886751345948128211 ) ) ;
#27540=CARTESIAN_POINT ( 'NONE',  ( 1.975475456537005874E-15, 0.3750000027311862216, 5.000000000000000000 ) ) ;
#27543=CARTESIAN_POINT ( 'NONE',  ( 4.458734125000000326, -55.89583333196773651, 2.574251347313718519 ) ) ;
#27544=CARTESIAN_POINT ( 'NONE',  ( 1.975475456537005874E-15, 10.24999999999999822, 5.000000000000000000 ) ) ;
#27545=CARTESIAN_POINT ( 'NONE',  ( 2.229367062499998831, 25.35416666803225993, -3.861377020970580887 ) ) ;
#27546=CARTESIAN_POINT ( 'NONE',  ( 5.000000000000000000, -104.5000000000000142, -6.123233995736766282E-16 ) ) ;
#27548=CARTESIAN_POINT ( 'NONE',  ( 2.229367062500001939, -46.22916666530106511, 3.861377020970579999 ) ) ;
#27549=CARTESIAN_POINT ( 'NONE',  ( -5.000000000000000000, 0.04166666939785235169, -2.886751345948128211 ) ) ;
#27550=CARTESIAN_POINT ( 'NONE',  ( 6.123233995736766282E-16, -120.0000000000000000, -5.000000000000000000 ) ) ;
#27553=CARTESIAN_POINT ( 'NONE',  ( -2.229367062500000163, -100.4791666653010651, -3.861377020970580443 ) ) ;
#27554=CARTESIAN_POINT ( 'NONE',  ( -4.458734124999999437, -4.562499998634401699, 0.000000000000000000 ) ) ;
#27555=ORIENTED_EDGE ( 'NONE', *, *, #26805, .F. ) ;
#27557=CARTESIAN_POINT ( 'NONE',  ( -4.458734124999999437, -92.39583333196773651, -2.574251347313719407 ) ) ;
#27559=CARTESIAN_POINT ( 'NONE',  ( 4.458734125000001214, -86.14583333196775072, 2.574251347313718519 ) ) ;
#27561=CYLINDRICAL_SURFACE ( 'NONE', #58218, 5.000000000000000000 ) ;
#27563=CARTESIAN_POINT ( 'NONE',  ( 4.458734125000000326, -11.89583333196774184, 2.574251347313718519 ) ) ;
#27564=CARTESIAN_POINT ( 'NONE',  ( 4.458734125000001214, 16.85416666803225638, 2.574251347313718519 ) ) ;
#27565=CARTESIAN_POINT ( 'NONE',  ( -2.229367062499996610, -55.39583333196773651, 3.861377020970582219 ) ) ;
#27569=CARTESIAN_POINT ( 'NONE',  ( 5.000000000000000888, -84.58333333333332860, 2.886751345948126879 ) ) ;
#27574=CARTESIAN_POINT ( 'NONE',  ( -3.152548672688508926E-16, -79.56249999863440792, -5.148502694627439702 ) ) ;
#27575=CARTESIAN_POINT ( 'NONE',  ( 4.458734125000001214, 23.85416666803225993, 2.574251347313718519 ) ) ;
#27576=( BOUNDED_CURVE ( )  B_SPLINE_CURVE ( 2, ( #29649, #10989, #40577, #25797, #403, #19687, #20976, #29317, #39934 ),
 .UNSPECIFIED., .F., .F. ) 
 B_SPLINE_CURVE_WITH_KNOTS ( ( 3, 2, 2, 2, 3 ),
 ( 0.7982142857142857650, 0.7988095238095238582, 0.8000000000000000444, 0.8011904761904762307, 0.8017857142857143238 ),
 .UNSPECIFIED. ) 
 CURVE ( )  GEOMETRIC_REPRESENTATION_ITEM ( )  RATIONAL_B_SPLINE_CURVE ( ( 0.9330127018922194093, 0.9330127018922194093, 1.000000000000000000, 0.8660254037844387076, 1.000000000000000000, 0.8660254037844387076, 1.000000000000000000, 0.9330127018922194093, 0.9330127018922194093 ) ) 
 REPRESENTATION_ITEM ( '' )  );
#27578=CARTESIAN_POINT ( 'NONE',  ( 0.000000000000000000, -120.0000000000000000, 0.000000000000000000 ) ) ;
#27579=CARTESIAN_POINT ( 'NONE',  ( 1.975475456537005874E-15, -6.749999999999999112, 5.000000000000000000 ) ) ;
#27581=CARTESIAN_POINT ( 'NONE',  ( -4.999999999999999112, -65.91666666666665719, 2.886751345948131764 ) ) ;
#27582=CARTESIAN_POINT ( 'NONE',  ( 1.339745962155612702, -63.16965819600734022, -5.000000000000000000 ) ) ;
#27586=VECTOR ( 'NONE', #8412, 1000.000000000000000 ) ;
#27587=CARTESIAN_POINT ( 'NONE',  ( 1.339745962155612702, 7.705341801261479162, -5.000000000000000000 ) ) ;
#27590=VECTOR ( 'NONE', #60772, 1000.000000000000000 ) ;
#27596=ORIENTED_EDGE ( 'NONE', *, *, #57044, .F. ) ;
#27600=EDGE_CURVE ( 'NONE', #25203, #7464, #51279, .T. ) ;
#27603=CARTESIAN_POINT ( 'NONE',  ( -4.458734124999999437, -53.64583333196772941, -2.574251347313719407 ) ) ;
#27604=ADVANCED_FACE ( 'NONE', ( #34914 ), #25258, .T. ) ;
#27607=ORIENTED_EDGE ( 'NONE', *, *, #29741, .T. ) ;
#27611=EDGE_CURVE ( 'NONE', #58224, #38122, #27395, .T. ) ;
#27615=CARTESIAN_POINT ( 'NONE',  ( -4.458734124999999437, -101.6458333319677365, -2.574251347313719407 ) ) ;
#27621=EDGE_CURVE ( 'NONE', #18331, #27768, #36049, .T. ) ;
#27623=CARTESIAN_POINT ( 'NONE',  ( -2.229367062499996610, -9.145833331967736513, 3.861377020970582219 ) ) ;
#27624=CARTESIAN_POINT ( 'NONE',  ( -4.458734124999999437, -96.64583333196773651, -2.574251347313719407 ) ) ;
#27625=ADVANCED_FACE ( 'NONE', ( #37458 ), #21401, .F. ) ;
#27627=CARTESIAN_POINT ( 'NONE',  ( -4.458734124999999437, -25.64583333196773651, -2.574251347313719407 ) ) ;
#27628=CARTESIAN_POINT ( 'NONE',  ( 5.000000000000000000, -46.50000000000000000, -6.123233995736766282E-16 ) ) ;
#27632=CARTESIAN_POINT ( 'NONE',  ( 1.339745962155612702, -70.29465819873850307, -5.000000000000000000 ) ) ;
#27633=CARTESIAN_POINT ( 'NONE',  ( 5.000000000000000000, -88.29166666393548724, -2.886751345948130876 ) ) ;
#27635=CARTESIAN_POINT ( 'NONE',  ( -4.458734124999999437, 10.35416666803225993, -2.574251347313719407 ) ) ;
#27636=VERTEX_POINT ( 'NONE', #60965 ) ;
#27637=CYLINDRICAL_SURFACE ( 'NONE', #9393, 5.000000000000000000 ) ;
#27638=CARTESIAN_POINT ( 'NONE',  ( -5.000000000000000000, -92.08333333333334281, -2.886751345948128211 ) ) ;
#27639=CARTESIAN_POINT ( 'NONE',  ( 2.229367062500001939, -22.97916666530107221, 3.861377020970579999 ) ) ;
#27640=CARTESIAN_POINT ( 'NONE',  ( -2.500000000000000444, -77.04166666393547303, -4.330127018922193649 ) ) ;
#27641=CARTESIAN_POINT ( 'NONE',  ( -4.458734124999999437, -70.56249999863439371, 0.000000000000000000 ) ) ;
#27643=CARTESIAN_POINT ( 'NONE',  ( -4.769696007084728073, -114.9999999999999858, -1.500000000000000000 ) ) ;
#27646=CARTESIAN_POINT ( 'NONE',  ( -4.458734124999997661, 5.770833334698928674, 2.574251347313722516 ) ) ;
#27650=CARTESIAN_POINT ( 'NONE',  ( -4.458734124999998549, -74.22916666530106511, 2.574251347313722516 ) ) ;
#27652=CARTESIAN_POINT ( 'NONE',  ( -3.535250795749689387E-16, -7.249999999999999112, -5.773502691896257311 ) ) ;
#27655=CARTESIAN_POINT ( 'NONE',  ( 4.458734124999998549, -61.72916666530106511, -2.574251347313721627 ) ) ;
#27656=CARTESIAN_POINT ( 'NONE',  ( 5.000000000000000000, -98.29166666393545881, -2.886751345948129988 ) ) ;
#27657=CARTESIAN_POINT ( 'NONE',  ( 3.044556291839386294E-14, 16.87500000273118417, -5.000000000000000000 ) ) ;
#27659=CARTESIAN_POINT ( 'NONE',  ( 9.457646018065525792E-16, -106.3124999986343937, 5.148502694627439702 ) ) ;
#27661=CARTESIAN_POINT ( 'NONE',  ( 5.000000000000000000, -46.50000000000000000, -6.123233995736766282E-16 ) ) ;
#27662=CARTESIAN_POINT ( 'NONE',  ( 1.339745962155615144, -72.58034179853027013, 4.999999999999999112 ) ) ;
#27663=DIRECTION ( 'NONE',  ( -3.614007241618347908E-17, 0.000000000000000000, 1.000000000000000000 ) ) ;
#27674=CARTESIAN_POINT ( 'NONE',  ( 5.000000000000000888, -81.58333333333332860, 2.886751345948126879 ) ) ;
#27676=VERTEX_POINT ( 'NONE', #17532 ) ;
#27677=CARTESIAN_POINT ( 'NONE',  ( 0.000000000000000000, -120.0000000000000000, 0.000000000000000000 ) ) ;
#27680=CARTESIAN_POINT ( 'NONE',  ( 9.457646018065525792E-16, -34.31249999863440792, 5.148502694627439702 ) ) ;
#27682=CARTESIAN_POINT ( 'NONE',  ( -1.339745962155610925, -86.79465819873851729, 5.000000000000000000 ) ) ;
#27684=( BOUNDED_CURVE ( )  B_SPLINE_CURVE ( 2, ( #16435, #1348, #21583, #36056, #25443, #10961, #55684, #11598, #36368 ),
 .UNSPECIFIED., .F., .F. ) 
 B_SPLINE_CURVE_WITH_KNOTS ( ( 3, 2, 2, 2, 3 ),
 ( 0.3303571428571428492, 0.3309523809523809423, 0.3321428571428571286, 0.3333333333333333148, 0.3339285714285714080 ),
 .UNSPECIFIED. ) 
 CURVE ( )  GEOMETRIC_REPRESENTATION_ITEM ( )  RATIONAL_B_SPLINE_CURVE ( ( 0.9330127018922194093, 0.9330127018922194093, 1.000000000000000000, 0.8660254037844387076, 1.000000000000000000, 0.8660254037844387076, 1.000000000000000000, 0.9330127018922194093, 0.9330127018922194093 ) ) 
 REPRESENTATION_ITEM ( '' )  );
#27686=FACE_OUTER_BOUND ( 'NONE', #19225, .T. ) ;
#27692=CARTESIAN_POINT ( 'NONE',  ( -4.458734124999999437, -83.56249999863439371, 0.000000000000000000 ) ) ;
#27698=CARTESIAN_POINT ( 'NONE',  ( 2.229367062500001939, -9.229166665301075767, 3.861377020970579999 ) ) ;
#27702=CARTESIAN_POINT ( 'NONE',  ( 6.123233995736766282E-16, -120.0000000000000000, -5.000000000000000000 ) ) ;
#27703=CARTESIAN_POINT ( 'NONE',  ( -4.458734124999998549, -6.479166665301073103, 2.574251347313722516 ) ) ;
#27704=DIRECTION ( 'NONE',  ( 0.000000000000000000, 0.000000000000000000, 1.000000000000000000 ) ) ;
#27706=CARTESIAN_POINT ( 'NONE',  ( 0.000000000000000000, -120.0000000000000000, 0.000000000000000000 ) ) ;
#27708=CARTESIAN_POINT ( 'NONE',  ( -4.458734124999997661, 25.52083333469892423, 2.574251347313722516 ) ) ;
#27709=ORIENTED_EDGE ( 'NONE', *, *, #13018, .T. ) ;
#27710=CARTESIAN_POINT ( 'NONE',  ( -4.458734124999999437, -92.31249999863440792, 0.000000000000000000 ) ) ;
#27712=CARTESIAN_POINT ( 'NONE',  ( -3.152548672688508926E-16, -8.562499998634404363, -5.148502694627439702 ) ) ;
#27715=CARTESIAN_POINT ( 'NONE',  ( 1.975475456537005874E-15, 15.25000000000000000, 5.000000000000000000 ) ) ;
#27716=CARTESIAN_POINT ( 'NONE',  ( 2.500000000000002220, -38.54166666393548013, 4.330127018922192761 ) ) ;
#27718=CARTESIAN_POINT ( 'NONE',  ( -4.458734124999999437, 19.60416666803225993, -2.574251347313719407 ) ) ;
#27721=CARTESIAN_POINT ( 'NONE',  ( 4.458734124999998549, -54.72916666530107932, -2.574251347313721627 ) ) ;
#27723=FACE_OUTER_BOUND ( 'NONE', #3771, .T. ) ;
#27724=CARTESIAN_POINT ( 'NONE',  ( 1.060575238724906964E-15, 13.24999999999999822, 5.773502691896257311 ) ) ;
#27727=CARTESIAN_POINT ( 'NONE',  ( -4.458734124999999437, -50.31249999863440792, 0.000000000000000000 ) ) ;
#27728=CARTESIAN_POINT ( 'NONE',  ( 2.500000000000002220, -84.54166666393547303, 4.330127018922192761 ) ) ;
#27731=CARTESIAN_POINT ( 'NONE',  ( -2.500000000000000444, -105.0416666639354730, -4.330127018922193649 ) ) ;
#27732=CARTESIAN_POINT ( 'NONE',  ( 2.229367062500001939, -85.22916666530107932, 3.861377020970579999 ) ) ;
#27734=CARTESIAN_POINT ( 'NONE',  ( -2.499999999999996447, -34.83333333333332860, 4.330127018922195425 ) ) ;
#27735=CARTESIAN_POINT ( 'NONE',  ( -1.339745962155613812, 23.79465819873851729, -5.000000000000000000 ) ) ;
#27738=ORIENTED_EDGE ( 'NONE', *, *, #5996, .F. ) ;
#27739=CARTESIAN_POINT ( 'NONE',  ( 4.458734124999998549, -97.72916666530106511, -2.574251347313721627 ) ) ;
#27740=CARTESIAN_POINT ( 'NONE',  ( -3.152548672688508926E-16, 7.187500001365594748, -5.148502694627439702 ) ) ;
#27741=CARTESIAN_POINT ( 'NONE',  ( 2.500000000000002220, 11.45833333606451809, 4.330127018922192761 ) ) ;
#27742=CARTESIAN_POINT ( 'NONE',  ( 1.975475456537005874E-15, -43.62499999726880873, 5.000000000000000000 ) ) ;
#27745=CARTESIAN_POINT ( 'NONE',  ( 1.975475456537005874E-15, -39.75000000000000000, 5.000000000000000000 ) ) ;
#27746=CARTESIAN_POINT ( 'NONE',  ( 5.000000000000000888, -80.58333333333332860, 2.886751345948126879 ) ) ;
#27752=CARTESIAN_POINT ( 'NONE',  ( -2.480964764533239819E-13, -107.7500000000000000, 5.000000000000000000 ) ) ;
#27754=CARTESIAN_POINT ( 'NONE',  ( -4.458734124999998549, -22.47916666530107577, 2.574251347313722516 ) ) ;
#27755=CARTESIAN_POINT ( 'NONE',  ( 1.243387493232115550E-13, -8.250000000000003553, -5.000000000000000000 ) ) ;
#27764=CARTESIAN_POINT ( 'NONE',  ( -6.972266317189433020E-16, -93.12499999726881583, -5.000000000000000000 ) ) ;
#27766=CARTESIAN_POINT ( 'NONE',  ( 9.457646018065525792E-16, -67.31249999863440792, 5.148502694627439702 ) ) ;
#27768=VERTEX_POINT ( 'NONE', #46790 ) ;
#27770=CYLINDRICAL_SURFACE ( 'NONE', #26182, 5.000000000000000000 ) ;
#27771=DIRECTION ( 'NONE',  ( -0.000000000000000000, 1.000000000000000000, -0.000000000000000000 ) ) ;
#27775=( BOUNDED_CURVE ( )  B_SPLINE_CURVE ( 2, ( #44748, #49894, #26416, #45398, #15500, #26100, #16132, #46033, #36070 ),
 .UNSPECIFIED., .F., .F. ) 
 B_SPLINE_CURVE_WITH_KNOTS ( ( 3, 2, 2, 2, 3 ),
 ( 0.9303571428571428825, 0.9309523809523809756, 0.9321428571428571619, 0.9333333333333333481, 0.9339285714285714413 ),
 .UNSPECIFIED. ) 
 CURVE ( )  GEOMETRIC_REPRESENTATION_ITEM ( )  RATIONAL_B_SPLINE_CURVE ( ( 0.9330127018922194093, 0.9330127018922194093, 1.000000000000000000, 0.8660254037844387076, 1.000000000000000000, 0.8660254037844387076, 1.000000000000000000, 0.9330127018922194093, 0.9330127018922194093 ) ) 
 REPRESENTATION_ITEM ( '' )  );
#27777=CARTESIAN_POINT ( 'NONE',  ( -2.229367062499996610, 6.854166668032259935, 3.861377020970582219 ) ) ;
#27780=CARTESIAN_POINT ( 'NONE',  ( 5.000000000000000888, 16.41666666666666785, 2.886751345948126879 ) ) ;
#27783=CARTESIAN_POINT ( 'NONE',  ( -3.152548672688508926E-16, -71.56249999863439371, -5.148502694627439702 ) ) ;
#27785=CARTESIAN_POINT ( 'NONE',  ( 2.229367062499998831, 5.354166668032261711, -3.861377020970580887 ) ) ;
#27787=CARTESIAN_POINT ( 'NONE',  ( -4.458734124999998549, -58.47916666530106511, 2.574251347313722516 ) ) ;
#27788=CARTESIAN_POINT ( 'NONE',  ( -5.000000000000000000, -21.87499999726881228, 0.000000000000000000 ) ) ;
#27793=CARTESIAN_POINT ( 'NONE',  ( -2.229367062499996610, -43.14583333196773651, 3.861377020970582219 ) ) ;
#27794=CARTESIAN_POINT ( 'NONE',  ( -4.458734124999999437, -22.64583333196773651, -2.574251347313719407 ) ) ;
#27796=LINE ( 'NONE', #13007, #53425 ) ;
#27797=CARTESIAN_POINT ( 'NONE',  ( 4.458734125000001214, -109.8958333319677365, 2.574251347313718519 ) ) ;
#27800=CARTESIAN_POINT ( 'NONE',  ( -4.458734124999999437, -109.6458333319677365, -2.574251347313719407 ) ) ;
#27802=CARTESIAN_POINT ( 'NONE',  ( -2.229367062499996610, -30.14583333196773651, 3.861377020970582219 ) ) ;
#27803=CARTESIAN_POINT ( 'NONE',  ( 2.500000000000002220, -68.54166666393547303, 4.330127018922192761 ) ) ;
#27806=CARTESIAN_POINT ( 'NONE',  ( 4.458734125000000326, -30.89583333196773651, 2.574251347313718519 ) ) ;
#27807=CARTESIAN_POINT ( 'NONE',  ( 4.458734125000000326, -68.14583333196773651, 2.574251347313718519 ) ) ;
#27810=CARTESIAN_POINT ( 'NONE',  ( 1.339745962155612702, -32.16965819600733312, -5.000000000000000000 ) ) ;
#27812=CARTESIAN_POINT ( 'NONE',  ( 5.000000000000000888, -17.58333333333333215, 2.886751345948126879 ) ) ;
#27814=ORIENTED_EDGE ( 'NONE', *, *, #53861, .T. ) ;
#27817=CARTESIAN_POINT ( 'NONE',  ( -1.339745962155585168, -3.080341798530293662, -5.000000000000015987 ) ) ;
#27818=CARTESIAN_POINT ( 'NONE',  ( -6.972266317189433020E-16, -81.12499999726881583, -5.000000000000000000 ) ) ;
#27824=CARTESIAN_POINT ( 'NONE',  ( -2.500000000000000444, -52.04166666393547303, -4.330127018922193649 ) ) ;
#27827=ORIENTED_EDGE ( 'NONE', *, *, #40459, .F. ) ;
#27828=DIRECTION ( 'NONE',  ( -0.000000000000000000, 1.000000000000000000, -0.000000000000000000 ) ) ;
#27837=ORIENTED_EDGE ( 'NONE', *, *, #43993, .T. ) ;
#27838=CARTESIAN_POINT ( 'NONE',  ( 5.000000000000000888, -53.58333333333333570, 2.886751345948126879 ) ) ;
#27845=CARTESIAN_POINT ( 'NONE',  ( -2.229367062499996610, -85.14583333196773651, 3.861377020970582219 ) ) ;
#27846=CARTESIAN_POINT ( 'NONE',  ( -4.458734124999999437, 23.68750000136559564, 0.000000000000000000 ) ) ;
#27847=FACE_OUTER_BOUND ( 'NONE', #42945, .T. ) ;
#27848=ORIENTED_EDGE ( 'NONE', *, *, #58331, .T. ) ;
#27849=CARTESIAN_POINT ( 'NONE',  ( 5.000000000000000888, 14.41666666666666430, 2.886751345948126879 ) ) ;
#27853=FACE_OUTER_BOUND ( 'NONE', #59392, .T. ) ;
#27857=CARTESIAN_POINT ( 'NONE',  ( -2.229367062499996610, -52.14583333196773651, 3.861377020970582219 ) ) ;
#27859=VECTOR ( 'NONE', #25137, 1000.000000000000000 ) ;
#27860=CARTESIAN_POINT ( 'NONE',  ( 2.229367062500001939, 25.02083333469892779, 3.861377020970579999 ) ) ;
#27861=CARTESIAN_POINT ( 'NONE',  ( -3.535250795749689387E-16, -108.2499999999999858, -5.773502691896257311 ) ) ;
#27863=CARTESIAN_POINT ( 'NONE',  ( 9.457646018065525792E-16, -45.31249999863440081, 5.148502694627439702 ) ) ;
#27864=CARTESIAN_POINT ( 'NONE',  ( -2.500000000000000444, -6.041666663935481019, -4.330127018922193649 ) ) ;
#27865=DIRECTION ( 'NONE',  ( -0.000000000000000000, 1.000000000000000000, -0.000000000000000000 ) ) ;
#27868=CARTESIAN_POINT ( 'NONE',  ( -4.458734124999999437, -104.3124999986344079, 0.000000000000000000 ) ) ;
#27869=CARTESIAN_POINT ( 'NONE',  ( 4.458734124999999437, -5.062499998634402587, -5.460374474430324690E-16 ) ) ;
#27872=CARTESIAN_POINT ( 'NONE',  ( -3.152548672688508926E-16, -90.56249999863440792, -5.148502694627439702 ) ) ;
#27874=CARTESIAN_POINT ( 'NONE',  ( -2.229367062500000163, -93.72916666530106511, -3.861377020970580443 ) ) ;
#27879=CARTESIAN_POINT ( 'NONE',  ( 4.458734124999999437, -10.81249999863440792, -5.460374474430324690E-16 ) ) ;
#27880=CARTESIAN_POINT ( 'NONE',  ( 4.458734124999999437, 12.93750000136559208, -5.460374474430324690E-16 ) ) ;
#27881=CARTESIAN_POINT ( 'NONE',  ( 2.229367062500001939, -56.22916666530107221, 3.861377020970579999 ) ) ;
#27883=CARTESIAN_POINT ( 'NONE',  ( -1.230605004983934782E-13, -36.75000000000000711, 5.000000000000000000 ) ) ;
#27885=CARTESIAN_POINT ( 'NONE',  ( 0.000000000000000000, -120.0000000000000000, 5.000000000000000000 ) ) ;
#27886=EDGE_LOOP ( 'NONE', ( #46775, #54671, #22114, #61945 ) ) ;
#27889=CARTESIAN_POINT ( 'NONE',  ( 1.975475456537005874E-15, -76.75000000000000000, 5.000000000000000000 ) ) ;
#27890=EDGE_CURVE ( 'NONE', #44569, #62283, #5229, .T. ) ;
#27892=CARTESIAN_POINT ( 'NONE',  ( 2.229367062499998831, -79.64583333196773651, -3.861377020970580887 ) ) ;
#27893=CARTESIAN_POINT ( 'NONE',  ( -2.229367062500000163, 25.27083333469892779, -3.861377020970580443 ) ) ;
#27895=FACE_OUTER_BOUND ( 'NONE', #49982, .T. ) ;
#27899=CARTESIAN_POINT ( 'NONE',  ( -4.999999999999999112, -69.91666666666667140, 2.886751345948131764 ) ) ;
#27902=CYLINDRICAL_SURFACE ( 'NONE', #18092, 5.000000000000000000 ) ;
#27911=CARTESIAN_POINT ( 'NONE',  ( 5.000000000000000888, -28.58333333333333570, 2.886751345948126879 ) ) ;
#27916=CARTESIAN_POINT ( 'NONE',  ( 2.229367062500001939, -53.22916666530107221, 3.861377020970579999 ) ) ;
#27927=CARTESIAN_POINT ( 'NONE',  ( -3.152548672688508926E-16, -98.81249999863440792, -5.148502694627439702 ) ) ;
#27932=LINE ( 'NONE', #3503, #60999 ) ;
#27933=CARTESIAN_POINT ( 'NONE',  ( 9.457646018065525792E-16, -7.062499998634404363, 5.148502694627439702 ) ) ;
#27934=CARTESIAN_POINT ( 'NONE',  ( 4.458734124999999437, -97.06249999863440792, -5.460374474430324690E-16 ) ) ;
#27936=CARTESIAN_POINT ( 'NONE',  ( 2.229367062499998831, -25.89583333196773651, -3.861377020970580887 ) ) ;
#27937=CARTESIAN_POINT ( 'NONE',  ( -1.339745962155613812, -67.20534180126149693, -5.000000000000000000 ) ) ;
#27940=FACE_OUTER_BOUND ( 'NONE', #47671, .T. ) ;
#27941=CARTESIAN_POINT ( 'NONE',  ( 0.000000000000000000, -120.0000000000000000, 0.000000000000000000 ) ) ;
#27943=CARTESIAN_POINT ( 'NONE',  ( -2.229367062500000163, 11.27083333469892601, -3.861377020970580443 ) ) ;
#27944=ORIENTED_EDGE ( 'NONE', *, *, #5070, .F. ) ;
#27945=CARTESIAN_POINT ( 'NONE',  ( 7.204675194429079505E-15, 26.87500000273118417, -5.000000000000000000 ) ) ;
#27947=CARTESIAN_POINT ( 'NONE',  ( -5.000000000000000000, -91.08333333333334281, -2.886751345948128211 ) ) ;
#27948=CARTESIAN_POINT ( 'NONE',  ( -4.458734124999999437, -24.39583333196773651, -2.574251347313719407 ) ) ;
#27949=DIRECTION ( 'NONE',  ( -0.000000000000000000, 1.000000000000000000, -0.000000000000000000 ) ) ;
#27950=CARTESIAN_POINT ( 'NONE',  ( -4.458734124999999437, -78.56249999863440792, 0.000000000000000000 ) ) ;
#27953=( BOUNDED_CURVE ( )  B_SPLINE_CURVE ( 2, ( #729, #34471, #30294, #50239, #59912, #45415, #10680, #11311, #55074 ),
 .UNSPECIFIED., .F., .F. ) 
 B_SPLINE_CURVE_WITH_KNOTS ( ( 3, 2, 2, 2, 3 ),
 ( 0.1553571428571428603, 0.1559523809523809534, 0.1571428571428571397, 0.1583333333333333259, 0.1589285714285714191 ),
 .UNSPECIFIED. ) 
 CURVE ( )  GEOMETRIC_REPRESENTATION_ITEM ( )  RATIONAL_B_SPLINE_CURVE ( ( 0.9330127018922194093, 0.9330127018922194093, 1.000000000000000000, 0.8660254037844387076, 1.000000000000000000, 0.8660254037844387076, 1.000000000000000000, 0.9330127018922194093, 0.9330127018922194093 ) ) 
 REPRESENTATION_ITEM ( '' )  );
#27955=EDGE_CURVE ( 'NONE', #62968, #10267, #63482, .T. ) ;
#27957=CARTESIAN_POINT ( 'NONE',  ( -2.229367062499996610, 1.854166668032262377, 3.861377020970582219 ) ) ;
#27958=EDGE_CURVE ( 'NONE', #46124, #38768, #27796, .T. ) ;
#27960=CARTESIAN_POINT ( 'NONE',  ( 9.457646018065525792E-16, -71.06249999863440792, 5.148502694627439702 ) ) ;
#27962=CARTESIAN_POINT ( 'NONE',  ( -4.999999999999999112, -4.916666666666666075, 2.886751345948131764 ) ) ;
#27965=CARTESIAN_POINT ( 'NONE',  ( -4.458734124999999437, -64.31249999863440792, 0.000000000000000000 ) ) ;
#27966=CARTESIAN_POINT ( 'NONE',  ( 2.499999999999998668, -98.20833333060214443, -4.330127018922193649 ) ) ;
#27970=CARTESIAN_POINT ( 'NONE',  ( -1.339745962155610925, -63.79465819873851729, 5.000000000000000000 ) ) ;
#27972=CARTESIAN_POINT ( 'NONE',  ( -3.152548672688508926E-16, -105.8124999986344221, -5.148502694627439702 ) ) ;
#27974=CARTESIAN_POINT ( 'NONE',  ( -4.999999999999999112, -52.91666666666666430, 2.886751345948131764 ) ) ;
#27977=ORIENTED_EDGE ( 'NONE', *, *, #51779, .F. ) ;
#27982=ADVANCED_FACE ( 'NONE', ( #48043 ), #18767, .T. ) ;
#27984=CARTESIAN_POINT ( 'NONE',  ( 1.975475456537005874E-15, -4.624999997268815832, 5.000000000000000000 ) ) ;
#27987=ORIENTED_EDGE ( 'NONE', *, *, #21742, .F. ) ;
#27990=ORIENTED_EDGE ( 'NONE', *, *, #16484, .F. ) ;
#27994=CARTESIAN_POINT ( 'NONE',  ( 9.457646018065525792E-16, -37.31249999863440792, 5.148502694627439702 ) ) ;
#28003=CARTESIAN_POINT ( 'NONE',  ( 2.229367062499998831, -83.89583333196773651, -3.861377020970580887 ) ) ;
#28004=CARTESIAN_POINT ( 'NONE',  ( 1.975475456537005874E-15, -3.624999997268814056, 5.000000000000000000 ) ) ;
#28005=( BOUNDED_CURVE ( )  B_SPLINE_CURVE ( 2, ( #63206, #20082, #39057, #13984, #24268, #15260, #33614, #49026, #33921 ),
 .UNSPECIFIED., .F., .F. ) 
 B_SPLINE_CURVE_WITH_KNOTS ( ( 3, 2, 2, 2, 3 ),
 ( 0.2446428571428571341, 0.2452380952380952273, 0.2464285714285714413, 0.2476190476190476275, 0.2482142857142857206 ),
 .UNSPECIFIED. ) 
 CURVE ( )  GEOMETRIC_REPRESENTATION_ITEM ( )  RATIONAL_B_SPLINE_CURVE ( ( 0.9330127018922194093, 0.9330127018922194093, 1.000000000000000000, 0.8660254037844387076, 1.000000000000000000, 0.8660254037844387076, 1.000000000000000000, 0.9330127018922194093, 0.9330127018922194093 ) ) 
 REPRESENTATION_ITEM ( '' )  );
#28008=( BOUNDED_CURVE ( )  B_SPLINE_CURVE ( 2, ( #10818, #30430, #60365, #16918, #41037, #45231, #25931, #35589, #2152 ),
 .UNSPECIFIED., .F., .F. ) 
 B_SPLINE_CURVE_WITH_KNOTS ( ( 3, 2, 2, 2, 3 ),
 ( 0.8232142857142856762, 0.8238095238095237693, 0.8249999999999999556, 0.8261904761904761418, 0.8267857142857142350 ),
 .UNSPECIFIED. ) 
 CURVE ( )  GEOMETRIC_REPRESENTATION_ITEM ( )  RATIONAL_B_SPLINE_CURVE ( ( 0.9330127018922194093, 0.9330127018922194093, 1.000000000000000000, 0.8660254037844387076, 1.000000000000000000, 0.8660254037844387076, 1.000000000000000000, 0.9330127018922194093, 0.9330127018922194093 ) ) 
 REPRESENTATION_ITEM ( '' )  );
#28009=CARTESIAN_POINT ( 'NONE',  ( 2.499999999999998668, -82.20833333060214443, -4.330127018922193649 ) ) ;
#28012=ORIENTED_EDGE ( 'NONE', *, *, #13304, .F. ) ;
#28015=CARTESIAN_POINT ( 'NONE',  ( -4.458734124999999437, -9.562499998634406140, 0.000000000000000000 ) ) ;
#28016=CARTESIAN_POINT ( 'NONE',  ( -5.000000000000000000, -35.00000000000000000, 0.000000000000000000 ) ) ;
#28020=CARTESIAN_POINT ( 'NONE',  ( -2.229367062500000163, 25.27083333469892779, -3.861377020970580443 ) ) ;
#28021=ORIENTED_EDGE ( 'NONE', *, *, #3544, .F. ) ;
#28022=CARTESIAN_POINT ( 'NONE',  ( -3.152548672688508926E-16, -94.56249999863440792, -5.148502694627439702 ) ) ;
#28023=CARTESIAN_POINT ( 'NONE',  ( -2.500000000000000444, -97.16666666666665719, -4.330127018922193649 ) ) ;
#28024=DIRECTION ( 'NONE',  ( -0.000000000000000000, 1.000000000000000000, -0.000000000000000000 ) ) ;
#28025=CARTESIAN_POINT ( 'NONE',  ( 9.457646018065525792E-16, -9.062499998634406140, 5.148502694627439702 ) ) ;
#28026=LINE ( 'NONE', #42502, #22150 ) ;
#28027=CARTESIAN_POINT ( 'NONE',  ( 1.975475456537005874E-15, -27.62499999726880873, 5.000000000000000000 ) ) ;
#28028=LINE ( 'NONE', #60325, #8903 ) ;
#28030=CARTESIAN_POINT ( 'NONE',  ( 5.000000000000000000, -35.29166666393547303, -2.886751345948129988 ) ) ;
#28032=CARTESIAN_POINT ( 'NONE',  ( -2.229367062499996610, 20.85416666803226349, 3.861377020970582219 ) ) ;
#28033=CARTESIAN_POINT ( 'NONE',  ( 1.975475456537005874E-15, -20.62499999726881228, 5.000000000000000000 ) ) ;
#28036=CARTESIAN_POINT ( 'NONE',  ( -2.229367062500000163, -56.47916666530107221, -3.861377020970580443 ) ) ;
#28039=CARTESIAN_POINT ( 'NONE',  ( 5.000000000000000000, 8.500000000000000000, -6.123233995736766282E-16 ) ) ;
#28042=CARTESIAN_POINT ( 'NONE',  ( -4.458734124999999437, -48.31249999863440792, 0.000000000000000000 ) ) ;
#28043=CARTESIAN_POINT ( 'NONE',  ( -2.499999999999996447, -82.70833333060214443, 4.330127018922195425 ) ) ;
#28046=FACE_OUTER_BOUND ( 'NONE', #56436, .T. ) ;
#28047=CARTESIAN_POINT ( 'NONE',  ( 4.458734124999999437, -92.06249999863440792, -5.460374474430324690E-16 ) ) ;
#28049=CARTESIAN_POINT ( 'NONE',  ( 5.000000000000000888, -39.58333333333333570, 2.886751345948126879 ) ) ;
#28054=ORIENTED_EDGE ( 'NONE', *, *, #3151, .T. ) ;
#28055=CARTESIAN_POINT ( 'NONE',  ( -4.458734124999999437, -96.39583333196772230, -2.574251347313719407 ) ) ;
#28056=CARTESIAN_POINT ( 'NONE',  ( 2.229367062500001939, 6.770833334698928674, 3.861377020970579999 ) ) ;
#28057=CARTESIAN_POINT ( 'NONE',  ( -4.999999999999999112, 11.20833333606451632, 2.886751345948131764 ) ) ;
#28059=CARTESIAN_POINT ( 'NONE',  ( -1.339745962155613812, -35.08034179853028434, -5.000000000000000000 ) ) ;
#28064=EDGE_CURVE ( 'NONE', #62355, #50926, #28113, .T. ) ;
#28070=CARTESIAN_POINT ( 'NONE',  ( -6.972266317189433020E-16, -21.24999999999999289, -5.000000000000000000 ) ) ;
#28072=CARTESIAN_POINT ( 'NONE',  ( 9.457646018065525792E-16, -19.31249999863440792, 5.148502694627439702 ) ) ;
#28083=CARTESIAN_POINT ( 'NONE',  ( -2.229367062500000163, -65.72916666530106511, -3.861377020970580443 ) ) ;
#28089=CARTESIAN_POINT ( 'NONE',  ( -2.229367062500000163, 0.2708333346989263979, -3.861377020970580443 ) ) ;
#28090=ORIENTED_EDGE ( 'NONE', *, *, #54696, .F. ) ;
#28091=CYLINDRICAL_SURFACE ( 'NONE', #11099, 5.000000000000000000 ) ;
#28092=CARTESIAN_POINT ( 'NONE',  ( 4.458734124999998549, 4.270833334698926897, -2.574251347313721627 ) ) ;
#28095=CARTESIAN_POINT ( 'NONE',  ( -1.339745962155613812, 5.919658201469705894, -5.000000000000000000 ) ) ;
#28098=CARTESIAN_POINT ( 'NONE',  ( -2.229367062500000163, -76.47916666530106511, -3.861377020970580443 ) ) ;
#28099=FACE_OUTER_BOUND ( 'NONE', #46207, .T. ) ;
#28100=CARTESIAN_POINT ( 'NONE',  ( -3.152548672688508926E-16, 5.437500001365592084, -5.148502694627439702 ) ) ;
#28101=VECTOR ( 'NONE', #26757, 1000.000000000000000 ) ;
#28102=EDGE_CURVE ( 'NONE', #20861, #53594, #23922, .T. ) ;
#28104=CARTESIAN_POINT ( 'NONE',  ( -3.152548672688508926E-16, -62.81249999863440792, -5.148502694627439702 ) ) ;
#28105=CARTESIAN_POINT ( 'NONE',  ( -2.499999999999996447, -22.70833333060214443, 4.330127018922195425 ) ) ;
#28107=CARTESIAN_POINT ( 'NONE',  ( -6.972266317189433020E-16, -28.12499999726880873, -5.000000000000000000 ) ) ;
#28110=CARTESIAN_POINT ( 'NONE',  ( 1.975475456537005874E-15, -54.74999999999999289, 5.000000000000000000 ) ) ;
#28111=CARTESIAN_POINT ( 'NONE',  ( -2.229367062499996610, -40.14583333196773651, 3.861377020970582219 ) ) ;
#28112=CARTESIAN_POINT ( 'NONE',  ( -2.229367062499996610, -28.39583333196774007, 3.861377020970582219 ) ) ;
#28113=LINE ( 'NONE', #47730, #42141 ) ;
#28114=CARTESIAN_POINT ( 'NONE',  ( 1.060575238724906964E-15, 24.24999999999999645, 5.773502691896257311 ) ) ;
#28117=CARTESIAN_POINT ( 'NONE',  ( -2.229367062499996610, -110.3958333319677507, 3.861377020970582219 ) ) ;
#28118=CARTESIAN_POINT ( 'NONE',  ( -4.458734124999999437, -32.31249999863440792, 0.000000000000000000 ) ) ;
#28119=CARTESIAN_POINT ( 'NONE',  ( 5.000000000000000000, -70.29166666393547303, -2.886751345948129988 ) ) ;
#28122=CARTESIAN_POINT ( 'NONE',  ( -2.229367062500000163, -28.47916666530107221, -3.861377020970580443 ) ) ;
#28123=CARTESIAN_POINT ( 'NONE',  ( 2.229367062499998831, -76.89583333196773651, -3.861377020970580887 ) ) ;
#28128=CARTESIAN_POINT ( 'NONE',  ( -4.999999999999999112, -18.91666666666666430, 2.886751345948131764 ) ) ;
#28130=ORIENTED_EDGE ( 'NONE', *, *, #18075, .F. ) ;
#28131=LINE ( 'NONE', #57110, #60529 ) ;
#28133=CARTESIAN_POINT ( 'NONE',  ( 2.500000000000002220, 28.45833333606451987, 4.330127018922192761 ) ) ;
#28134=CARTESIAN_POINT ( 'NONE',  ( 5.000000000000000888, -81.45833333060213022, 2.886751345948126879 ) ) ;
#28136=( BOUNDED_CURVE ( )  B_SPLINE_CURVE ( 2, ( #27764, #53158, #38363, #43492, #38665, #13611, #14225, #24199, #33542 ),
 .UNSPECIFIED., .F., .F. ) 
 B_SPLINE_CURVE_WITH_KNOTS ( ( 3, 2, 2, 2, 3 ),
 ( 0.8732142857142857206, 0.8738095238095238138, 0.8750000000000000000, 0.8761904761904761862, 0.8767857142857142794 ),
 .UNSPECIFIED. ) 
 CURVE ( )  GEOMETRIC_REPRESENTATION_ITEM ( )  RATIONAL_B_SPLINE_CURVE ( ( 0.9330127018922194093, 0.9330127018922194093, 1.000000000000000000, 0.8660254037844387076, 1.000000000000000000, 0.8660254037844387076, 1.000000000000000000, 0.9330127018922194093, 0.9330127018922194093 ) ) 
 REPRESENTATION_ITEM ( '' )  );
#28142=VERTEX_POINT ( 'NONE', #1087 ) ;
#28143=CARTESIAN_POINT ( 'NONE',  ( -6.972266317189433020E-16, -39.25000000000000000, -5.000000000000000000 ) ) ;
#28144=VERTEX_POINT ( 'NONE', #4932 ) ;
#28145=CARTESIAN_POINT ( 'NONE',  ( 0.000000000000000000, -120.0000000000000000, 0.000000000000000000 ) ) ;
#28153=ORIENTED_EDGE ( 'NONE', *, *, #24234, .T. ) ;
#28154=CARTESIAN_POINT ( 'NONE',  ( 1.975475456537005874E-15, 21.24999999999999289, 5.000000000000000000 ) ) ;
#28157=DIRECTION ( 'NONE',  ( -0.000000000000000000, 1.000000000000000000, -0.000000000000000000 ) ) ;
#28161=EDGE_LOOP ( 'NONE', ( #52852, #39183, #25549, #22675 ) ) ;
#28162=CARTESIAN_POINT ( 'NONE',  ( -4.458734124999999437, -83.39583333196772230, -2.574251347313719407 ) ) ;
#28163=CARTESIAN_POINT ( 'NONE',  ( 9.457646018065525792E-16, 23.93750000136559564, 5.148502694627439702 ) ) ;
#28164=CARTESIAN_POINT ( 'NONE',  ( 0.000000000000000000, -120.0000000000000000, 5.000000000000000000 ) ) ;
#28165=ORIENTED_EDGE ( 'NONE', *, *, #58181, .F. ) ;
#28169=DIRECTION ( 'NONE',  ( 0.000000000000000000, 0.000000000000000000, 1.000000000000000000 ) ) ;
#28171=CARTESIAN_POINT ( 'NONE',  ( -4.458734124999999437, -60.31249999863440081, 0.000000000000000000 ) ) ;
#28173=CARTESIAN_POINT ( 'NONE',  ( -3.152548672688508926E-16, 23.43750000136559564, -5.148502694627439702 ) ) ;
#28176=CARTESIAN_POINT ( 'NONE',  ( -2.229367062500000163, -41.72916666530107932, -3.861377020970580443 ) ) ;
#28177=CARTESIAN_POINT ( 'NONE',  ( 1.060575238724906964E-15, -6.624999997268813168, 5.773502691896257311 ) ) ;
#28178=CARTESIAN_POINT ( 'NONE',  ( 5.000000000000000888, -31.58333333333333215, 2.886751345948126879 ) ) ;
#28181=CARTESIAN_POINT ( 'NONE',  ( 2.229367062499998831, -104.6458333319677365, -3.861377020970580887 ) ) ;
#28182=CARTESIAN_POINT ( 'NONE',  ( 4.458734124999999437, -10.06249999863440614, -5.460374474430324690E-16 ) ) ;
#28185=CARTESIAN_POINT ( 'NONE',  ( -3.152548672688508926E-16, -95.56249999863442213, -5.148502694627439702 ) ) ;
#28187=CARTESIAN_POINT ( 'NONE',  ( 2.229367062499998831, -93.89583333196772230, -3.861377020970580887 ) ) ;
#28188=CARTESIAN_POINT ( 'NONE',  ( -2.499999999999996447, -51.70833333060213732, 4.330127018922195425 ) ) ;
#28189=CARTESIAN_POINT ( 'NONE',  ( 1.975475456537005874E-15, 10.37500000273118417, 5.000000000000000000 ) ) ;
#28192=CARTESIAN_POINT ( 'NONE',  ( -4.458734124999997661, -11.22916666530107044, 2.574251347313722516 ) ) ;
#28193=CARTESIAN_POINT ( 'NONE',  ( 4.458734124999999437, 11.93750000136559564, -5.460374474430324690E-16 ) ) ;
#28194=CARTESIAN_POINT ( 'NONE',  ( -2.229367062500000163, -55.72916666530107221, -3.861377020970580443 ) ) ;
#28202=CYLINDRICAL_SURFACE ( 'NONE', #30475, 5.000000000000000000 ) ;
#28203=CARTESIAN_POINT ( 'NONE',  ( 1.975475456537005874E-15, -8.750000000000000000, 5.000000000000000000 ) ) ;
#28205=CARTESIAN_POINT ( 'NONE',  ( -4.458734124999999437, -86.39583333196772230, -2.574251347313719407 ) ) ;
#28206=CARTESIAN_POINT ( 'NONE',  ( -4.458734124999999437, 24.43750000136559208, 0.000000000000000000 ) ) ;
#28211=CARTESIAN_POINT ( 'NONE',  ( -3.535250795749689387E-16, -69.24999999999998579, -5.773502691896257311 ) ) ;
#28213=ORIENTED_EDGE ( 'NONE', *, *, #1370, .T. ) ;
#28214=CARTESIAN_POINT ( 'NONE',  ( -6.972266317189433020E-16, -18.12499999726881228, -5.000000000000000000 ) ) ;
#28216=CARTESIAN_POINT ( 'NONE',  ( 5.000000000000000888, -40.58333333333334281, 2.886751345948126879 ) ) ;
#28219=CARTESIAN_POINT ( 'NONE',  ( 5.000000000000000000, 18.50000000000000000, -6.123233995736766282E-16 ) ) ;
#28228=CARTESIAN_POINT ( 'NONE',  ( 2.229367062500001939, -55.22916666530107221, 3.861377020970579999 ) ) ;
#28238=AXIS2_PLACEMENT_3D ( 'NONE', #13297, #58547, #39861 ) ;
#28241=CARTESIAN_POINT ( 'NONE',  ( -3.152548672688508926E-16, -99.81249999863442213, -5.148502694627439702 ) ) ;
#28242=CARTESIAN_POINT ( 'NONE',  ( -1.339745962155669101, -26.66965819600733667, 4.999999999999966249 ) ) ;
#28246=CARTESIAN_POINT ( 'NONE',  ( -2.499999999999996447, 1.291666669397853351, 4.330127018922195425 ) ) ;
#28247=CARTESIAN_POINT ( 'NONE',  ( 4.458734124999999437, -9.812499998634406140, -5.460374474430324690E-16 ) ) ;
#28248=CARTESIAN_POINT ( 'NONE',  ( -2.229367062500000163, -101.7291666653010651, -3.861377020970580443 ) ) ;
#28249=ADVANCED_FACE ( 'NONE', ( #45122 ), #44156, .T. ) ;
#28251=CARTESIAN_POINT ( 'NONE',  ( 9.457646018065525792E-16, -28.31249999863440081, 5.148502694627439702 ) ) ;
#28256=CARTESIAN_POINT ( 'NONE',  ( 0.000000000000000000, -120.0000000000000000, 0.000000000000000000 ) ) ;
#28259=CARTESIAN_POINT ( 'NONE',  ( 9.457646018065525792E-16, 7.687500001365596525, 5.148502694627439702 ) ) ;
#28262=CARTESIAN_POINT ( 'NONE',  ( 5.000000000000000000, 9.583333333333332149, -2.886751345948130876 ) ) ;
#28263=CARTESIAN_POINT ( 'NONE',  ( -5.000000000000000000, -90.08333333333332860, -2.886751345948128211 ) ) ;
#28264=CARTESIAN_POINT ( 'NONE',  ( 4.458734124999999437, -26.81249999863440081, -5.460374474430324690E-16 ) ) ;
#28265=DIRECTION ( 'NONE',  ( -0.000000000000000000, 1.000000000000000000, -0.000000000000000000 ) ) ;
#28266=CARTESIAN_POINT ( 'NONE',  ( -3.152548672688508926E-16, -76.81249999863440792, -5.148502694627439702 ) ) ;
#28270=CARTESIAN_POINT ( 'NONE',  ( -4.458734124999997661, 2.770833334698928674, 2.574251347313722516 ) ) ;
#28271=CARTESIAN_POINT ( 'NONE',  ( 2.229367062500001939, 28.77083333469892779, 3.861377020970579999 ) ) ;
#28272=CARTESIAN_POINT ( 'NONE',  ( -4.458734124999999437, -37.56249999863440792, 0.000000000000000000 ) ) ;
#28276=CARTESIAN_POINT ( 'NONE',  ( -4.458734124999999437, -70.39583333196773651, -2.574251347313719407 ) ) ;
#28279=CARTESIAN_POINT ( 'NONE',  ( 4.458734124999998549, -63.72916666530107221, -2.574251347313721627 ) ) ;
#28280=CARTESIAN_POINT ( 'NONE',  ( -2.500000000000000444, -99.04166666393545881, -4.330127018922193649 ) ) ;
#28281=AXIS2_PLACEMENT_3D ( 'NONE', #33928, #24597, #10117 ) ;
#28286=CARTESIAN_POINT ( 'NONE',  ( 4.458734124999998549, -103.9791666653010509, -2.574251347313721627 ) ) ;
#28288=CARTESIAN_POINT ( 'NONE',  ( -5.000000000000000000, -52.99999999999999289, 0.000000000000000000 ) ) ;
#28289=CARTESIAN_POINT ( 'NONE',  ( 1.975475456537005874E-15, -72.62499999726878741, 5.000000000000000000 ) ) ;
#28301=DIRECTION ( 'NONE',  ( -0.000000000000000000, 1.000000000000000000, -0.000000000000000000 ) ) ;
#28306=CARTESIAN_POINT ( 'NONE',  ( 4.458734124999998549, -36.97916666530107221, -2.574251347313721627 ) ) ;
#28311=EDGE_CURVE ( 'NONE', #42248, #43569, #48983, .T. ) ;
#28316=CARTESIAN_POINT ( 'NONE',  ( 1.975475456537005874E-15, -54.74999999999999289, 5.000000000000000000 ) ) ;
#28318=CARTESIAN_POINT ( 'NONE',  ( -2.229367062499996610, -83.39583333196773651, 3.861377020970582219 ) ) ;
#28328=CARTESIAN_POINT ( 'NONE',  ( 5.000000000000000000, -78.41666666666667140, -2.886751345948130876 ) ) ;
#28329=CARTESIAN_POINT ( 'NONE',  ( 9.457646018065525792E-16, -11.31249999863440792, 5.148502694627439702 ) ) ;
#28330=EDGE_CURVE ( 'NONE', #49599, #60646, #12616, .T. ) ;
#28335=CARTESIAN_POINT ( 'NONE',  ( -3.152548672688508926E-16, 24.18750000136559564, -5.148502694627439702 ) ) ;
#28337=CARTESIAN_POINT ( 'NONE',  ( -2.229367062499996610, -91.14583333196773651, 3.861377020970582219 ) ) ;
#28339=CARTESIAN_POINT ( 'NONE',  ( -4.458734124999999437, -7.312499998634404363, 0.000000000000000000 ) ) ;
#28340=CYLINDRICAL_SURFACE ( 'NONE', #24194, 5.000000000000000000 ) ;
#28342=CARTESIAN_POINT ( 'NONE',  ( 5.000000000000000000, -38.37499999726881583, -6.123233995736766282E-16 ) ) ;
#28344=CARTESIAN_POINT ( 'NONE',  ( 2.229367062499998831, 18.35416666803225993, -3.861377020970580887 ) ) ;
#28347=CARTESIAN_POINT ( 'NONE',  ( 4.458734124999998549, -55.72916666530107221, -2.574251347313721627 ) ) ;
#28350=CARTESIAN_POINT ( 'NONE',  ( 2.500000000000002220, 12.33333333333333215, 4.330127018922192761 ) ) ;
#28352=CARTESIAN_POINT ( 'NONE',  ( -2.229367062500000163, -46.47916666530106511, -3.861377020970580443 ) ) ;
#28353=CARTESIAN_POINT ( 'NONE',  ( 1.060575238724906964E-15, -84.62499999726880162, 5.773502691896257311 ) ) ;
#28355=CARTESIAN_POINT ( 'NONE',  ( 2.500000000000002220, -37.54166666393548013, 4.330127018922192761 ) ) ;
#28356=DIRECTION ( 'NONE',  ( -0.000000000000000000, 1.000000000000000000, -0.000000000000000000 ) ) ;
#28357=CARTESIAN_POINT ( 'NONE',  ( -2.229367062500000163, -90.72916666530106511, -3.861377020970580443 ) ) ;
#28359=CARTESIAN_POINT ( 'NONE',  ( 2.499999999999998668, -36.33333333333332860, -4.330127018922193649 ) ) ;
#28363=ORIENTED_EDGE ( 'NONE', *, *, #12667, .F. ) ;
#28364=CARTESIAN_POINT ( 'NONE',  ( -4.458734124999998549, -95.22916666530106511, 2.574251347313722516 ) ) ;
#28365=CARTESIAN_POINT ( 'NONE',  ( 4.458734124999999437, 5.937500001365593860, -5.460374474430324690E-16 ) ) ;
#28366=CARTESIAN_POINT ( 'NONE',  ( -3.535250795749689387E-16, 9.875000002731184168, -5.773502691896257311 ) ) ;
#28372=CARTESIAN_POINT ( 'NONE',  ( -4.999999999999998224, 15.20833333606451987, 2.886751345948131764 ) ) ;
#28378=CARTESIAN_POINT ( 'NONE',  ( 1.243387493232115550E-13, -19.25000000000000000, -5.000000000000000000 ) ) ;
#28382=CARTESIAN_POINT ( 'NONE',  ( 2.229367062499998831, -18.89583333196774007, -3.861377020970580887 ) ) ;
#28390=EDGE_CURVE ( 'NONE', #60295, #37393, #46753, .T. ) ;
#28394=CARTESIAN_POINT ( 'NONE',  ( -2.229367062500000163, -66.72916666530106511, -3.861377020970580443 ) ) ;
#28396=( NAMED_UNIT ( * ) PLANE_ANGLE_UNIT ( ) SI_UNIT ( $, .RADIAN. ) );
#28398=EDGE_CURVE ( 'NONE', #56025, #17652, #31529, .T. ) ;
#28402=CARTESIAN_POINT ( 'NONE',  ( 2.229367062500001939, 0.7708333346989268975, 3.861377020970579999 ) ) ;
#28403=VERTEX_POINT ( 'NONE', #11974 ) ;
#28404=CARTESIAN_POINT ( 'NONE',  ( 4.458734125000001214, 1.104166668032261711, 2.574251347313718519 ) ) ;
#28412=CARTESIAN_POINT ( 'NONE',  ( -4.458734124999999437, -78.31249999863440792, 0.000000000000000000 ) ) ;
#28414=CARTESIAN_POINT ( 'NONE',  ( 4.458734125000001214, 9.104166668032261711, 2.574251347313718519 ) ) ;
#28415=AXIS2_PLACEMENT_3D ( 'NONE', #57125, #13040, #51969 ) ;
#28416=AXIS2_PLACEMENT_3D ( 'NONE', #49391, #20125, #60015 ) ;
#28418=LINE ( 'NONE', #58950, #41823 ) ;
#28419=CARTESIAN_POINT ( 'NONE',  ( 2.229367062500001939, -59.22916666530106511, 3.861377020970579999 ) ) ;
#28421=CARTESIAN_POINT ( 'NONE',  ( 5.000000000000000000, -20.37499999726880873, -6.123233995736766282E-16 ) ) ;
#28423=CYLINDRICAL_SURFACE ( 'NONE', #10041, 5.000000000000000000 ) ;
#28425=CARTESIAN_POINT ( 'NONE',  ( -1.339745962155610925, -105.6696581960073473, 5.000000000000000000 ) ) ;
#28426=CARTESIAN_POINT ( 'NONE',  ( 1.975475456537005874E-15, -38.75000000000000000, 5.000000000000000000 ) ) ;
#28427=CARTESIAN_POINT ( 'NONE',  ( 9.457646018065525792E-16, -42.06249999863440081, 5.148502694627439702 ) ) ;
#28428=CARTESIAN_POINT ( 'NONE',  ( 9.457646018065525792E-16, -26.31249999863440792, 5.148502694627439702 ) ) ;
#28430=CARTESIAN_POINT ( 'NONE',  ( 6.123233995736766282E-16, -120.0000000000000000, -5.000000000000000000 ) ) ;
#28431=CARTESIAN_POINT ( 'NONE',  ( -2.499999999999996447, 27.16666666666666430, 4.330127018922195425 ) ) ;
#28434=CARTESIAN_POINT ( 'NONE',  ( 9.457646018065525792E-16, -106.3124999986343795, 5.148502694627439702 ) ) ;
#28435=CARTESIAN_POINT ( 'NONE',  ( 2.229367062500001939, -32.97916666530106511, 3.861377020970579999 ) ) ;
#28436=CARTESIAN_POINT ( 'NONE',  ( -4.999999999999999112, -68.79166666393547303, 2.886751345948131764 ) ) ;
#28439=CARTESIAN_POINT ( 'NONE',  ( -2.229367062500000163, -29.47916666530107221, -3.861377020970580443 ) ) ;
#28440=CARTESIAN_POINT ( 'NONE',  ( -2.229367062499996610, -72.39583333196773651, 3.861377020970582219 ) ) ;
#28442=CARTESIAN_POINT ( 'NONE',  ( 0.000000000000000000, -120.0000000000000000, 0.000000000000000000 ) ) ;
#28444=CARTESIAN_POINT ( 'NONE',  ( -5.000000000000000000, -22.00000000000000000, 0.000000000000000000 ) ) ;
#28446=ORIENTED_EDGE ( 'NONE', *, *, #15284, .T. ) ;
#28449=CARTESIAN_POINT ( 'NONE',  ( 5.000000000000000000, 25.62500000273118417, -6.123233995736766282E-16 ) ) ;
#28454=CARTESIAN_POINT ( 'NONE',  ( -5.000000000000000000, -51.95833333060214443, -2.886751345948128211 ) ) ;
#28455=CYLINDRICAL_SURFACE ( 'NONE', #12212, 5.000000000000000000 ) ;
#28459=VECTOR ( 'NONE', #35485, 1000.000000000000000 ) ;
#28460=CARTESIAN_POINT ( 'NONE',  ( -6.972266317189433020E-16, 10.87500000273118417, -5.000000000000000000 ) ) ;
#28467=AXIS2_PLACEMENT_3D ( 'NONE', #19870, #921, #59120 ) ;
#28469=ORIENTED_EDGE ( 'NONE', *, *, #15253, .F. ) ;
#28473=ORIENTED_EDGE ( 'NONE', *, *, #20483, .F. ) ;
#28474=CARTESIAN_POINT ( 'NONE',  ( 1.975475456537005874E-15, -38.62499999726880873, 5.000000000000000000 ) ) ;
#28478=CARTESIAN_POINT ( 'NONE',  ( -4.458734124999998549, -83.22916666530106511, 2.574251347313722516 ) ) ;
#28479=CARTESIAN_POINT ( 'NONE',  ( 9.457646018065525792E-16, 20.93750000136558853, 5.148502694627439702 ) ) ;
#28480=CARTESIAN_POINT ( 'NONE',  ( -1.339745962155610925, -17.66965819600733312, 5.000000000000000000 ) ) ;
#28486=CARTESIAN_POINT ( 'NONE',  ( 1.339745962155615144, -39.70534180126147561, 4.999999999999999112 ) ) ;
#28487=CARTESIAN_POINT ( 'NONE',  ( 5.000000000000000888, 4.416666666666666075, 2.886751345948126879 ) ) ;
#28488=CARTESIAN_POINT ( 'NONE',  ( -3.152548672688508926E-16, -59.56249999863440081, -5.148502694627439702 ) ) ;
#28489=CARTESIAN_POINT ( 'NONE',  ( -2.229367062499996610, 25.85416666803225993, 3.861377020970582219 ) ) ;
#28490=CARTESIAN_POINT ( 'NONE',  ( 1.975475456537005874E-15, -97.74999999999998579, 5.000000000000000000 ) ) ;
#28491=CARTESIAN_POINT ( 'NONE',  ( -6.972266317189433020E-16, -44.25000000000000000, -5.000000000000000000 ) ) ;
#28492=CARTESIAN_POINT ( 'NONE',  ( -4.458734124999998549, -44.47916666530106511, 2.574251347313722516 ) ) ;
#28493=CARTESIAN_POINT ( 'NONE',  ( 5.000000000000000888, -6.458333330602148870, 2.886751345948126879 ) ) ;
#28494=CARTESIAN_POINT ( 'NONE',  ( -2.500000000000000444, -93.16666666666665719, -4.330127018922193649 ) ) ;
#28497=CARTESIAN_POINT ( 'NONE',  ( 4.458734125000000326, -109.8958333319677365, 2.574251347313718519 ) ) ;
#28498=CARTESIAN_POINT ( 'NONE',  ( -2.229367062500000163, -11.72916666530107044, -3.861377020970580443 ) ) ;
#28501=CARTESIAN_POINT ( 'NONE',  ( -3.152548672688508926E-16, -100.5624999986344079, -5.148502694627439702 ) ) ;
#28503=CARTESIAN_POINT ( 'NONE',  ( -2.229367062500000163, -94.72916666530106511, -3.861377020970580443 ) ) ;
#28504=CARTESIAN_POINT ( 'NONE',  ( 1.060575238724906964E-15, -52.62499999726881583, 5.773502691896257311 ) ) ;
#28505=CARTESIAN_POINT ( 'NONE',  ( -5.000000000000000000, -36.95833333060213022, -2.886751345948128211 ) ) ;
#28506=AXIS2_PLACEMENT_3D ( 'NONE', #17858, #7275, #60672 ) ;
#28510=CARTESIAN_POINT ( 'NONE',  ( 4.458734125000000326, -10.89583333196773651, 2.574251347313718519 ) ) ;
#28511=CARTESIAN_POINT ( 'NONE',  ( 4.458734124999998549, 9.020833334698927786, -2.574251347313721627 ) ) ;
#28512=CARTESIAN_POINT ( 'NONE',  ( -2.229367062499996610, -57.39583333196773651, 3.861377020970582219 ) ) ;
#28513=CARTESIAN_POINT ( 'NONE',  ( -6.972266317189433020E-16, -52.25000000000000711, -5.000000000000000000 ) ) ;
#28514=CARTESIAN_POINT ( 'NONE',  ( 5.000000000000000888, -15.45833333060214443, 2.886751345948126879 ) ) ;
#28521=DIRECTION ( 'NONE',  ( -0.000000000000000000, 1.000000000000000000, -0.000000000000000000 ) ) ;
#28523=CARTESIAN_POINT ( 'NONE',  ( 9.457646018065525792E-16, -85.06249999863440792, 5.148502694627439702 ) ) ;
#28524=CARTESIAN_POINT ( 'NONE',  ( -4.458734124999999437, 21.43750000136559208, 0.000000000000000000 ) ) ;
#28527=CARTESIAN_POINT ( 'NONE',  ( -4.330127018922101279, 45.00000000000000000, 7.500000000000002665 ) ) ;
#28529=CARTESIAN_POINT ( 'NONE',  ( 1.060575238724906964E-15, -67.75000000000000000, 5.773502691896257311 ) ) ;
#28532=CARTESIAN_POINT ( 'NONE',  ( -6.972266317189433020E-16, -79.24999999999998579, -5.000000000000000000 ) ) ;
#28542=ORIENTED_EDGE ( 'NONE', *, *, #15425, .F. ) ;
#28545=CARTESIAN_POINT ( 'NONE',  ( 4.458734125000001214, -56.14583333196774362, 2.574251347313718519 ) ) ;
#28546=VECTOR ( 'NONE', #9197, 1000.000000000000000 ) ;
#28549=ORIENTED_EDGE ( 'NONE', *, *, #42487, .F. ) ;
#28555=CARTESIAN_POINT ( 'NONE',  ( -3.152548672688508926E-16, -106.8124999986343795, -5.148502694627439702 ) ) ;
#28556=CARTESIAN_POINT ( 'NONE',  ( -4.999999999999998224, -68.79166666393547303, 2.886751345948131764 ) ) ;
#28557=ORIENTED_EDGE ( 'NONE', *, *, #23713, .T. ) ;
#28560=CARTESIAN_POINT ( 'NONE',  ( -4.458734124999999437, -38.31249999863439371, 0.000000000000000000 ) ) ;
#28562=CARTESIAN_POINT ( 'NONE',  ( -3.152548672688508926E-16, -8.562499998634404363, -5.148502694627439702 ) ) ;
#28563=CARTESIAN_POINT ( 'NONE',  ( 2.229367062499998831, -101.8958333319677365, -3.861377020970580887 ) ) ;
#28565=CARTESIAN_POINT ( 'NONE',  ( -4.458734124999999437, -30.56249999863440436, 0.000000000000000000 ) ) ;
#28569=CARTESIAN_POINT ( 'NONE',  ( -2.500000000000000444, -16.16666666666666785, -4.330127018922193649 ) ) ;
#28570=CARTESIAN_POINT ( 'NONE',  ( -1.339745962155613812, 16.79465819873852084, -5.000000000000000000 ) ) ;
#28572=CARTESIAN_POINT ( 'NONE',  ( 4.458734124999999437, 4.937500001365595637, -5.460374474430324690E-16 ) ) ;
#28574=EDGE_LOOP ( 'NONE', ( #27977, #53888, #29977, #48324 ) ) ;
#28576=CARTESIAN_POINT ( 'NONE',  ( 5.000000000000000000, 9.499999999999998224, -6.123233995736766282E-16 ) ) ;
#28577=CARTESIAN_POINT ( 'NONE',  ( 5.000000000000000000, -93.41666666666667140, -2.886751345948129988 ) ) ;
#28578=CARTESIAN_POINT ( 'NONE',  ( 4.458734124999999437, -31.81249999863440436, -5.460374474430324690E-16 ) ) ;
#28580=CARTESIAN_POINT ( 'NONE',  ( -4.458734124999999437, -73.64583333196773651, -2.574251347313719407 ) ) ;
#28584=CARTESIAN_POINT ( 'NONE',  ( -2.229367062499996610, 3.854166668032260823, 3.861377020970582219 ) ) ;
#28585=CARTESIAN_POINT ( 'NONE',  ( -4.458734124999999437, 27.43750000136559208, 0.000000000000000000 ) ) ;
#28586=CARTESIAN_POINT ( 'NONE',  ( 4.458734124999999437, -43.06249999863440081, -5.460374474430324690E-16 ) ) ;
#28590=AXIS2_PLACEMENT_3D ( 'NONE', #53171, #10047, #25159 ) ;
#28592=CARTESIAN_POINT ( 'NONE',  ( 9.457646018065525792E-16, -70.06249999863439371, 5.148502694627439702 ) ) ;
#28593=CARTESIAN_POINT ( 'NONE',  ( 2.499999999999998668, -102.2083333306021444, -4.330127018922193649 ) ) ;
#28594=EDGE_CURVE ( 'NONE', #60902, #25319, #23849, .T. ) ;
#28595=VECTOR ( 'NONE', #14605, 1000.000000000000000 ) ;
#28597=CYLINDRICAL_SURFACE ( 'NONE', #63642, 5.000000000000000000 ) ;
#28598=CARTESIAN_POINT ( 'NONE',  ( -3.152548672688508926E-16, -104.8124999986344079, -5.148502694627439702 ) ) ;
#28600=CARTESIAN_POINT ( 'NONE',  ( -2.499999999999996447, -51.83333333333332860, 4.330127018922195425 ) ) ;
#28601=CARTESIAN_POINT ( 'NONE',  ( -6.972266317189433020E-16, -22.24999999999999645, -5.000000000000000000 ) ) ;
#28610=ADVANCED_FACE ( 'NONE', ( #13248 ), #57012, .T. ) ;
#28614=CARTESIAN_POINT ( 'NONE',  ( 2.499999999999998668, -45.20833333060214443, -4.330127018922193649 ) ) ;
#28617=VERTEX_POINT ( 'NONE', #23217 ) ;
#28621=CARTESIAN_POINT ( 'NONE',  ( 9.457646018065525792E-16, -42.31249999863440081, 5.148502694627439702 ) ) ;
#28624=DIRECTION ( 'NONE',  ( -0.000000000000000000, 1.000000000000000000, -0.000000000000000000 ) ) ;
#28630=CARTESIAN_POINT ( 'NONE',  ( 4.458734124999998549, -86.97916666530106511, -2.574251347313721627 ) ) ;
#28631=CARTESIAN_POINT ( 'NONE',  ( 1.975475456537005874E-15, -108.7499999999999858, 5.000000000000000000 ) ) ;
#28632=ORIENTED_EDGE ( 'NONE', *, *, #18079, .T. ) ;
#28638=ORIENTED_EDGE ( 'NONE', *, *, #17400, .T. ) ;
#28641=CARTESIAN_POINT ( 'NONE',  ( 4.458734124999998549, -11.97916666530107044, -2.574251347313721627 ) ) ;
#28642=CARTESIAN_POINT ( 'NONE',  ( 2.500000000000002220, -105.5416666639354730, 4.330127018922192761 ) ) ;
#28644=CARTESIAN_POINT ( 'NONE',  ( -2.480964764533239819E-13, -95.62499999726883004, 5.000000000000000000 ) ) ;
#28646=CARTESIAN_POINT ( 'NONE',  ( 4.458734124999999437, 19.93750000136559208, -5.460374474430324690E-16 ) ) ;
#28648=CARTESIAN_POINT ( 'NONE',  ( -3.152548672688508926E-16, -90.56249999863440792, -5.148502694627439702 ) ) ;
#28651=CARTESIAN_POINT ( 'NONE',  ( -4.458734124999999437, -12.39583333196774184, -2.574251347313719407 ) ) ;
#28653=CARTESIAN_POINT ( 'NONE',  ( -5.000000000000000000, -73.08333333333332860, -2.886751345948128211 ) ) ;
#28655=CARTESIAN_POINT ( 'NONE',  ( -2.500000000000000444, -38.04166666393548013, -4.330127018922193649 ) ) ;
#28656=CYLINDRICAL_SURFACE ( 'NONE', #3139, 5.000000000000000000 ) ;
#28657=CARTESIAN_POINT ( 'NONE',  ( -4.458734124999999437, 20.68750000136559208, 0.000000000000000000 ) ) ;
#28658=CARTESIAN_POINT ( 'NONE',  ( -6.972266317189433020E-16, -46.12499999726880873, -5.000000000000000000 ) ) ;
#28660=CARTESIAN_POINT ( 'NONE',  ( -4.458734124999998549, -55.22916666530107932, 2.574251347313722516 ) ) ;
#28663=CARTESIAN_POINT ( 'NONE',  ( -2.499999999999996447, 9.166666666666666075, 4.330127018922195425 ) ) ;
#28665=CARTESIAN_POINT ( 'NONE',  ( 9.457646018065525792E-16, -53.06249999863441502, 5.148502694627439702 ) ) ;
#28666=CARTESIAN_POINT ( 'NONE',  ( -2.500000000000000444, -82.04166666393547303, -4.330127018922193649 ) ) ;
#28669=CARTESIAN_POINT ( 'NONE',  ( -6.972266317189433020E-16, -14.12499999726881228, -5.000000000000000000 ) ) ;
#28671=CARTESIAN_POINT ( 'NONE',  ( -3.152548672688508926E-16, -91.81249999863442213, -5.148502694627439702 ) ) ;
#28673=CARTESIAN_POINT ( 'NONE',  ( -2.500000000000000444, -38.16666666666667140, -4.330127018922193649 ) ) ;
#28677=CARTESIAN_POINT ( 'NONE',  ( 4.458734125000001214, -97.89583333196773651, 2.574251347313718519 ) ) ;
#28678=CARTESIAN_POINT ( 'NONE',  ( -4.458734124999999437, 6.354166668032259047, -2.574251347313719407 ) ) ;
#28679=CARTESIAN_POINT ( 'NONE',  ( 5.000000000000000000, 11.62500000273118594, -6.123233995736766282E-16 ) ) ;
#28682=AXIS2_PLACEMENT_3D ( 'NONE', #61382, #6707, #56556 ) ;
#28692=CARTESIAN_POINT ( 'NONE',  ( -5.000000000000000000, -89.95833333060214443, -2.886751345948128211 ) ) ;
#28693=CARTESIAN_POINT ( 'NONE',  ( 9.457646018065525792E-16, -27.31249999863440436, 5.148502694627439702 ) ) ;
#28703=DIRECTION ( 'NONE',  ( 0.000000000000000000, -1.000000000000000000, 0.000000000000000000 ) ) ;
#28705=CARTESIAN_POINT ( 'NONE',  ( 2.229367062499998831, -65.89583333196773651, -3.861377020970580887 ) ) ;
#28707=ORIENTED_EDGE ( 'NONE', *, *, #48087, .F. ) ;
#28711=CARTESIAN_POINT ( 'NONE',  ( 2.229367062499998831, 0.1041666680322607397, -3.861377020970580887 ) ) ;
#28716=CARTESIAN_POINT ( 'NONE',  ( 5.000000000000000000, -92.29166666393547303, -2.886751345948130876 ) ) ;
#28720=CARTESIAN_POINT ( 'NONE',  ( -4.458734124999999437, -77.39583333196772230, -2.574251347313719407 ) ) ;
#28722=CARTESIAN_POINT ( 'NONE',  ( 2.229367062499998831, 6.354166668032262599, -3.861377020970580887 ) ) ;
#28724=CARTESIAN_POINT ( 'NONE',  ( -2.229367062499996610, -66.39583333196773651, 3.861377020970582219 ) ) ;
#28725=CARTESIAN_POINT ( 'NONE',  ( -4.999999999999999112, -18.79166666393547658, 2.886751345948131764 ) ) ;
#28727=CARTESIAN_POINT ( 'NONE',  ( 0.000000000000000000, -120.0000000000000000, 0.000000000000000000 ) ) ;
#28728=CARTESIAN_POINT ( 'NONE',  ( 2.499999999999998668, -49.33333333333332860, -4.330127018922193649 ) ) ;
#28731=CARTESIAN_POINT ( 'NONE',  ( 4.458734124999999437, -39.81249999863440081, -5.460374474430324690E-16 ) ) ;
#28732=CARTESIAN_POINT ( 'NONE',  ( 9.457646018065525792E-16, -25.31249999863440792, 5.148502694627439702 ) ) ;
#28734=CARTESIAN_POINT ( 'NONE',  ( -5.000000000000000000, 23.91666666666666785, -2.886751345948128211 ) ) ;
#28736=CARTESIAN_POINT ( 'NONE',  ( -4.458734124999998549, -106.4791666653010651, 2.574251347313722516 ) ) ;
#28737=CARTESIAN_POINT ( 'NONE',  ( 2.229367062499998831, -29.64583333196773296, -3.861377020970580887 ) ) ;
#28738=CARTESIAN_POINT ( 'NONE',  ( 2.500000000000002220, -65.54166666393547303, 4.330127018922192761 ) ) ;
#28743=CARTESIAN_POINT ( 'NONE',  ( 2.229367062499998831, -74.89583333196773651, -3.861377020970580887 ) ) ;
#28746=ADVANCED_FACE ( 'NONE', ( #27723 ), #47350, .T. ) ;
#28749=CARTESIAN_POINT ( 'NONE',  ( -2.500000000000000444, -20.16666666666666430, -4.330127018922193649 ) ) ;
#28751=VERTEX_POINT ( 'NONE', #21495 ) ;
#28753=CARTESIAN_POINT ( 'NONE',  ( 1.975475456537005874E-15, 1.250000000000000000, 5.000000000000000000 ) ) ;
#28755=( BOUNDED_CURVE ( )  B_SPLINE_CURVE ( 2, ( #2994, #2358, #7495, #46088, #27107, #22611, #56390, #50917, #21968 ),
 .UNSPECIFIED., .F., .F. ) 
 B_SPLINE_CURVE_WITH_KNOTS ( ( 3, 2, 2, 2, 3 ),
 ( 0.6624999999999999778, 0.6630952380952380709, 0.6642857142857142572, 0.6654761904761904434, 0.6660714285714285365 ),
 .UNSPECIFIED. ) 
 CURVE ( )  GEOMETRIC_REPRESENTATION_ITEM ( )  RATIONAL_B_SPLINE_CURVE ( ( 0.9330127018922194093, 0.9330127018922194093, 1.000000000000000000, 0.8660254037844387076, 1.000000000000000000, 0.8660254037844387076, 1.000000000000000000, 0.9330127018922194093, 0.9330127018922194093 ) ) 
 REPRESENTATION_ITEM ( '' )  );
#28757=CARTESIAN_POINT ( 'NONE',  ( -2.500000000000000444, 25.95833333606451632, -4.330127018922193649 ) ) ;
#28758=CARTESIAN_POINT ( 'NONE',  ( 1.339745962155615144, 4.419658201469705894, 4.999999999999999112 ) ) ;
#28760=ADVANCED_FACE ( 'NONE', ( #19645 ), #14813, .T. ) ;
#28761=EDGE_CURVE ( 'NONE', #10189, #42151, #11821, .T. ) ;
#28764=CARTESIAN_POINT ( 'NONE',  ( -1.339745962155613812, -41.08034179853029144, -5.000000000000000000 ) ) ;
#28777=VERTEX_POINT ( 'NONE', #4856 ) ;
#28781=CARTESIAN_POINT ( 'NONE',  ( -6.972266317189433020E-16, -12.24999999999999645, -5.000000000000000000 ) ) ;
#28785=CARTESIAN_POINT ( 'NONE',  ( 2.499999999999998668, -23.20833333060214443, -4.330127018922193649 ) ) ;
#28790=CARTESIAN_POINT ( 'NONE',  ( -2.229367062500000163, -82.47916666530106511, -3.861377020970580443 ) ) ;
#28791=CARTESIAN_POINT ( 'NONE',  ( -4.458734124999999437, 21.60416666803225993, -2.574251347313719407 ) ) ;
#28793=VERTEX_POINT ( 'NONE', #60103 ) ;
#28800=CARTESIAN_POINT ( 'NONE',  ( -2.229367062500000163, -61.47916666530106511, -3.861377020970580443 ) ) ;
#28802=CARTESIAN_POINT ( 'NONE',  ( -4.458734124999998549, 22.77083333469892423, 2.574251347313722516 ) ) ;
#28803=CARTESIAN_POINT ( 'NONE',  ( 5.000000000000000000, -97.50000000000000000, -6.123233995736766282E-16 ) ) ;
#28805=CARTESIAN_POINT ( 'NONE',  ( -4.458734124999998549, -46.47916666530107221, 2.574251347313722516 ) ) ;
#28806=CARTESIAN_POINT ( 'NONE',  ( 5.000000000000000000, -3.374999997268816276, -6.123233995736766282E-16 ) ) ;
#28807=CARTESIAN_POINT ( 'NONE',  ( -2.499999999999996447, -92.83333333333334281, 4.330127018922195425 ) ) ;
#28809=CARTESIAN_POINT ( 'NONE',  ( -4.458734124999997661, -110.2291666653010651, 2.574251347313722516 ) ) ;
#28810=CARTESIAN_POINT ( 'NONE',  ( 2.229367062499998831, -9.895833331967738289, -3.861377020970580887 ) ) ;
#28812=CARTESIAN_POINT ( 'NONE',  ( 1.975475456537005874E-15, -52.75000000000000000, 5.000000000000000000 ) ) ;
#28813=CARTESIAN_POINT ( 'NONE',  ( 4.458734124999998549, -100.7291666653010651, -2.574251347313721627 ) ) ;
#28815=CARTESIAN_POINT ( 'NONE',  ( 4.458734124999999437, -93.06249999863440792, -5.460374474430324690E-16 ) ) ;
#28817=CARTESIAN_POINT ( 'NONE',  ( 5.000000000000000888, -49.45833333060213732, 2.886751345948126879 ) ) ;
#28821=CARTESIAN_POINT ( 'NONE',  ( 4.458734125000000326, -19.89583333196774007, 2.574251347313718519 ) ) ;
#28822=CARTESIAN_POINT ( 'NONE',  ( -2.229367062500000163, 10.27083333469892779, -3.861377020970580443 ) ) ;
#28823=CARTESIAN_POINT ( 'NONE',  ( -4.458734124999999437, -61.56249999863440081, 0.000000000000000000 ) ) ;
#28826=CARTESIAN_POINT ( 'NONE',  ( 1.975475456537005874E-15, -36.62499999726880873, 5.000000000000000000 ) ) ;
#28828=VERTEX_POINT ( 'NONE', #14496 ) ;
#28830=CARTESIAN_POINT ( 'NONE',  ( 6.123233995736766282E-16, -120.0000000000000000, -5.000000000000000000 ) ) ;
#28832=CYLINDRICAL_SURFACE ( 'NONE', #62461, 5.000000000000000000 ) ;
#28833=CARTESIAN_POINT ( 'NONE',  ( -2.229367062500000163, -84.47916666530107932, -3.861377020970580443 ) ) ;
#28834=CARTESIAN_POINT ( 'NONE',  ( 4.458734124999999437, 16.93750000136559564, -5.460374474430324690E-16 ) ) ;
#28836=CARTESIAN_POINT ( 'NONE',  ( -5.000000000000000000, 6.999999999999999112, 0.000000000000000000 ) ) ;
#28839=CARTESIAN_POINT ( 'NONE',  ( 5.000000000000000000, -70.41666666666667140, -2.886751345948129988 ) ) ;
#28841=EDGE_CURVE ( 'NONE', #10579, #57689, #56719, .T. ) ;
#28845=LINE ( 'NONE', #25216, #31998 ) ;
#28849=EDGE_CURVE ( 'NONE', #50783, #34309, #3457, .T. ) ;
#28858=CARTESIAN_POINT ( 'NONE',  ( 4.458734124999998549, -58.97916666530105800, -2.574251347313721627 ) ) ;
#28862=AXIS2_PLACEMENT_3D ( 'NONE', #3475, #23088, #42692 ) ;
#28869=CARTESIAN_POINT ( 'NONE',  ( 2.229367062499998831, -102.8958333319677365, -3.861377020970580887 ) ) ;
#28874=CARTESIAN_POINT ( 'NONE',  ( 4.458734125000000326, -38.89583333196773651, 2.574251347313718519 ) ) ;
#28876=CARTESIAN_POINT ( 'NONE',  ( -2.229367062499996610, -13.14583333196774007, 3.861377020970582219 ) ) ;
#28878=CARTESIAN_POINT ( 'NONE',  ( -2.229367062500000163, -99.72916666530106511, -3.861377020970580443 ) ) ;
#28880=CARTESIAN_POINT ( 'NONE',  ( 2.229367062499998831, -27.89583333196774007, -3.861377020970580887 ) ) ;
#28884=CARTESIAN_POINT ( 'NONE',  ( -6.972266317189433020E-16, -17.25000000000000000, -5.000000000000000000 ) ) ;
#28887=CARTESIAN_POINT ( 'NONE',  ( 2.229367062499998831, 3.104166668032259935, -3.861377020970580887 ) ) ;
#28888=ORIENTED_EDGE ( 'NONE', *, *, #7948, .F. ) ;
#28890=CARTESIAN_POINT ( 'NONE',  ( 5.000000000000000000, 2.499999999999998668, -6.123233995736766282E-16 ) ) ;
#28891=CARTESIAN_POINT ( 'NONE',  ( 1.060575238724906964E-15, -97.75000000000000000, 5.773502691896257311 ) ) ;
#28892=CARTESIAN_POINT ( 'NONE',  ( 2.229367062500001939, -28.97916666530107221, 3.861377020970579999 ) ) ;
#28893=CARTESIAN_POINT ( 'NONE',  ( -1.339745962155613812, -77.08034179853029855, -5.000000000000000000 ) ) ;
#28894=CARTESIAN_POINT ( 'NONE',  ( -3.152548672688508926E-16, -73.81249999863440792, -5.148502694627439702 ) ) ;
#28899=CARTESIAN_POINT ( 'NONE',  ( -2.229367062499996610, 2.854166668032259935, 3.861377020970582219 ) ) ;
#28900=CARTESIAN_POINT ( 'NONE',  ( -4.458734124999998549, 25.52083333469893134, 2.574251347313722516 ) ) ;
#28901=CARTESIAN_POINT ( 'NONE',  ( 9.457646018065525792E-16, -44.31249999863440081, 5.148502694627439702 ) ) ;
#28902=DIRECTION ( 'NONE',  ( -0.000000000000000000, 1.000000000000000000, -0.000000000000000000 ) ) ;
#28908=CARTESIAN_POINT ( 'NONE',  ( 4.458734124999999437, -70.81249999863439371, -5.460374474430324690E-16 ) ) ;
#28909=CARTESIAN_POINT ( 'NONE',  ( -3.535250795749689387E-16, -104.1249999972688158, -5.773502691896257311 ) ) ;
#28910=CARTESIAN_POINT ( 'NONE',  ( -4.458734124999997661, -105.4791666653010509, 2.574251347313722516 ) ) ;
#28912=CARTESIAN_POINT ( 'NONE',  ( 5.000000000000000888, -53.58333333333333570, 2.886751345948126879 ) ) ;
#28913=CARTESIAN_POINT ( 'NONE',  ( -1.339745962155610925, -21.79465819873851729, 5.000000000000000000 ) ) ;
#28914=FACE_OUTER_BOUND ( 'NONE', #34382, .T. ) ;
#28924=ORIENTED_EDGE ( 'NONE', *, *, #55435, .T. ) ;
#28927=ORIENTED_EDGE ( 'NONE', *, *, #33847, .F. ) ;
#28931=CARTESIAN_POINT ( 'NONE',  ( 9.457646018065525792E-16, -39.31249999863439371, 5.148502694627439702 ) ) ;
#28932=LINE ( 'NONE', #48238, #34802 ) ;
#28939=CARTESIAN_POINT ( 'NONE',  ( -4.458734124999999437, -86.64583333196773651, -2.574251347313719407 ) ) ;
#28945=( BOUNDED_CURVE ( )  B_SPLINE_CURVE ( 2, ( #1240, #25020, #55258, #30800, #3367, #55580, #56768, #12689, #41076 ),
 .UNSPECIFIED., .F., .F. ) 
 B_SPLINE_CURVE_WITH_KNOTS ( ( 3, 2, 2, 2, 3 ),
 ( 0.4232142857142857095, 0.4238095238095238027, 0.4249999999999999889, 0.4261904761904761751, 0.4267857142857142683 ),
 .UNSPECIFIED. ) 
 CURVE ( )  GEOMETRIC_REPRESENTATION_ITEM ( )  RATIONAL_B_SPLINE_CURVE ( ( 0.9330127018922194093, 0.9330127018922194093, 1.000000000000000000, 0.8660254037844387076, 1.000000000000000000, 0.8660254037844387076, 1.000000000000000000, 0.9330127018922194093, 0.9330127018922194093 ) ) 
 REPRESENTATION_ITEM ( '' )  );
#28946=CARTESIAN_POINT ( 'NONE',  ( 1.339745962155612702, -43.29465819873851729, -5.000000000000000000 ) ) ;
#28948=ORIENTED_EDGE ( 'NONE', *, *, #48776, .F. ) ;
#28950=CARTESIAN_POINT ( 'NONE',  ( -2.229367062499996610, -10.39583333196773829, 3.861377020970582219 ) ) ;
#28953=CARTESIAN_POINT ( 'NONE',  ( -6.972266317189433020E-16, -12.12499999726881406, -5.000000000000000000 ) ) ;
#28955=CARTESIAN_POINT ( 'NONE',  ( 4.458734124999998549, 20.02083333469892779, -2.574251347313721627 ) ) ;
#28956=VERTEX_POINT ( 'NONE', #62001 ) ;
#28957=CARTESIAN_POINT ( 'NONE',  ( 2.229367062500001939, -89.97916666530106511, 3.861377020970579999 ) ) ;
#28960=CARTESIAN_POINT ( 'NONE',  ( 4.458734124999998549, -12.72916666530107044, -2.574251347313721627 ) ) ;
#28961=CARTESIAN_POINT ( 'NONE',  ( -6.972266317189433020E-16, -85.12499999726880162, -5.000000000000000000 ) ) ;
#28962=CARTESIAN_POINT ( 'NONE',  ( -1.339745962155727277, -72.79465819873851729, 4.999999999999933387 ) ) ;
#28964=CARTESIAN_POINT ( 'NONE',  ( -2.499999999999996447, -41.70833333060214443, 4.330127018922195425 ) ) ;
#28965=CARTESIAN_POINT ( 'NONE',  ( 5.000000000000000000, -29.41666666666666785, -2.886751345948130876 ) ) ;
#28966=CARTESIAN_POINT ( 'NONE',  ( 2.229367062500001939, 21.02083333469892779, 3.861377020970579999 ) ) ;
#28967=CARTESIAN_POINT ( 'NONE',  ( -2.499999999999996447, 12.29166666939785202, 4.330127018922195425 ) ) ;
#28970=CARTESIAN_POINT ( 'NONE',  ( 2.229367062500001939, -62.97916666530106511, 3.861377020970579999 ) ) ;
#28974=CARTESIAN_POINT ( 'NONE',  ( 5.000000000000000000, 10.58333333333333393, -2.886751345948129988 ) ) ;
#28977=CARTESIAN_POINT ( 'NONE',  ( -4.458734124999999437, -53.31249999863439371, 0.000000000000000000 ) ) ;
#28978=CARTESIAN_POINT ( 'NONE',  ( 5.000000000000000000, -88.29166666393547303, -2.886751345948129988 ) ) ;
#28981=CARTESIAN_POINT ( 'NONE',  ( -2.499999999999996447, -91.83333333333334281, 4.330127018922195425 ) ) ;
#28982=CARTESIAN_POINT ( 'NONE',  ( 2.229367062500001939, -89.22916666530106511, 3.861377020970579999 ) ) ;
#28984=CARTESIAN_POINT ( 'NONE',  ( -5.000000000000000000, -39.08333333333332860, -2.886751345948128211 ) ) ;
#28987=CARTESIAN_POINT ( 'NONE',  ( -4.458734124999999437, -102.3124999986344079, 0.000000000000000000 ) ) ;
#28988=CARTESIAN_POINT ( 'NONE',  ( -3.152548672688508926E-16, 8.187500001365595637, -5.148502694627439702 ) ) ;
#28995=CARTESIAN_POINT ( 'NONE',  ( -1.339745962155613812, -11.20534180126147916, -5.000000000000000000 ) ) ;
#28996=DIRECTION ( 'NONE',  ( 0.000000000000000000, 0.000000000000000000, 1.000000000000000000 ) ) ;
#28997=CARTESIAN_POINT ( 'NONE',  ( 1.975475456537005874E-15, -19.75000000000000000, 5.000000000000000000 ) ) ;
#28999=CARTESIAN_POINT ( 'NONE',  ( 5.000000000000000000, 6.708333336064521646, -2.886751345948130876 ) ) ;
#29000=CARTESIAN_POINT ( 'NONE',  ( -4.458734124999999437, -25.56249999863440792, 0.000000000000000000 ) ) ;
#29008=ORIENTED_EDGE ( 'NONE', *, *, #17227, .F. ) ;
#29010=ORIENTED_EDGE ( 'NONE', *, *, #10698, .T. ) ;
#29011=CARTESIAN_POINT ( 'NONE',  ( 4.458734124999999437, -73.06249999863439371, -5.460374474430324690E-16 ) ) ;
#29018=EDGE_CURVE ( 'NONE', #3585, #16917, #39771, .T. ) ;
#29019=CARTESIAN_POINT ( 'NONE',  ( 4.458734124999998549, 2.020833334698927786, -2.574251347313721627 ) ) ;
#29020=EDGE_LOOP ( 'NONE', ( #44310, #54822, #18344, #46572 ) ) ;
#29021=CYLINDRICAL_SURFACE ( 'NONE', #30668, 5.000000000000000000 ) ;
#29026=ORIENTED_EDGE ( 'NONE', *, *, #29090, .F. ) ;
#29027=CARTESIAN_POINT ( 'NONE',  ( 9.457646018065525792E-16, -76.06249999863440792, 5.148502694627439702 ) ) ;
#29028=EDGE_CURVE ( 'NONE', #50534, #5440, #50512, .T. ) ;
#29029=CARTESIAN_POINT ( 'NONE',  ( 5.000000000000000000, -0.3749999972688135008, -6.123233995736766282E-16 ) ) ;
#29030=CARTESIAN_POINT ( 'NONE',  ( 2.229367062499998831, 0.3541666680322609340, -3.861377020970580887 ) ) ;
#29031=DIRECTION ( 'NONE',  ( 0.000000000000000000, 0.000000000000000000, 1.000000000000000000 ) ) ;
#29032=CARTESIAN_POINT ( 'NONE',  ( 2.229367062499998831, -63.89583333196772941, -3.861377020970580887 ) ) ;
#29033=CARTESIAN_POINT ( 'NONE',  ( -2.500000000000000444, -26.04166666393547658, -4.330127018922193649 ) ) ;
#29034=EDGE_CURVE ( 'NONE', #41864, #33407, #13506, .T. ) ;
#29039=CARTESIAN_POINT ( 'NONE',  ( 2.499999999999998668, -43.20833333060214443, -4.330127018922193649 ) ) ;
#29040=CARTESIAN_POINT ( 'NONE',  ( -4.458734124999999437, -44.39583333196773651, -2.574251347313719407 ) ) ;
#29041=CARTESIAN_POINT ( 'NONE',  ( -4.458734124999997661, -27.47916666530107221, 2.574251347313722516 ) ) ;
#29043=CARTESIAN_POINT ( 'NONE',  ( -5.000000000000000000, 27.00000000000000000, 0.000000000000000000 ) ) ;
#29046=CARTESIAN_POINT ( 'NONE',  ( -4.458734124999999437, -35.31249999863440792, 0.000000000000000000 ) ) ;
#29047=CARTESIAN_POINT ( 'NONE',  ( 5.000000000000000888, -65.45833333060214443, 2.886751345948126879 ) ) ;
#29048=( BOUNDED_CURVE ( )  B_SPLINE_CURVE ( 2, ( #59365, #15298, #45202, #34921, #55185, #40374, #59693, #40049, #15938 ),
 .UNSPECIFIED., .F., .F. ) 
 B_SPLINE_CURVE_WITH_KNOTS ( ( 3, 2, 2, 2, 3 ),
 ( 0.6517857142857143016, 0.6523809523809523947, 0.6535714285714285809, 0.6547619047619047672, 0.6553571428571428603 ),
 .UNSPECIFIED. ) 
 CURVE ( )  GEOMETRIC_REPRESENTATION_ITEM ( )  RATIONAL_B_SPLINE_CURVE ( ( 0.9330127018922194093, 0.9330127018922194093, 1.000000000000000000, 0.8660254037844387076, 1.000000000000000000, 0.8660254037844387076, 1.000000000000000000, 0.9330127018922194093, 0.9330127018922194093 ) ) 
 REPRESENTATION_ITEM ( '' )  );
#29051=CARTESIAN_POINT ( 'NONE',  ( -4.458734124999997661, -76.47916666530105090, 2.574251347313722516 ) ) ;
#29054=CARTESIAN_POINT ( 'NONE',  ( -2.500000000000000444, -28.04166666393548013, -4.330127018922193649 ) ) ;
#29056=CARTESIAN_POINT ( 'NONE',  ( 2.500000000000002220, -22.66666666666666785, 4.330127018922192761 ) ) ;
#29060=CARTESIAN_POINT ( 'NONE',  ( -5.000000000000000000, -78.87499999726881583, 0.000000000000000000 ) ) ;
#29062=CARTESIAN_POINT ( 'NONE',  ( -5.000000000000000000, 28.12500000273118417, 0.000000000000000000 ) ) ;
#29063=CARTESIAN_POINT ( 'NONE',  ( 5.000000000000000000, -48.29166666393548724, -2.886751345948130876 ) ) ;
#29065=CARTESIAN_POINT ( 'NONE',  ( -1.339745962155610925, 8.330341803992665106, 5.000000000000000000 ) ) ;
#29067=( BOUNDED_CURVE ( )  B_SPLINE_CURVE ( 2, ( #62696, #53973, #52715, #8649, #28890, #24708, #19874, #63637, #34035 ),
 .UNSPECIFIED., .F., .F. ) 
 B_SPLINE_CURVE_WITH_KNOTS ( ( 3, 2, 2, 2, 3 ),
 ( 0.1946428571428571452, 0.1952380952380952384, 0.1964285714285714246, 0.1976190476190476109, 0.1982142857142857040 ),
 .UNSPECIFIED. ) 
 CURVE ( )  GEOMETRIC_REPRESENTATION_ITEM ( )  RATIONAL_B_SPLINE_CURVE ( ( 0.9330127018922194093, 0.9330127018922194093, 1.000000000000000000, 0.8660254037844387076, 1.000000000000000000, 0.8660254037844387076, 1.000000000000000000, 0.9330127018922194093, 0.9330127018922194093 ) ) 
 REPRESENTATION_ITEM ( '' )  );
#29072=CARTESIAN_POINT ( 'NONE',  ( -1.339745962155613812, -88.08034179853028434, -5.000000000000000000 ) ) ;
#29073=CARTESIAN_POINT ( 'NONE',  ( -3.152548672688508926E-16, -22.56249999863440081, -5.148502694627439702 ) ) ;
#29077=VERTEX_POINT ( 'NONE', #42994 ) ;
#29079=ORIENTED_EDGE ( 'NONE', *, *, #40089, .T. ) ;
#29080=CARTESIAN_POINT ( 'NONE',  ( -6.972266317189433020E-16, -53.24999999999999289, -5.000000000000000000 ) ) ;
#29081=CARTESIAN_POINT ( 'NONE',  ( 5.000000000000000888, -9.458333330602146205, 2.886751345948126879 ) ) ;
#29088=AXIS2_PLACEMENT_3D ( 'NONE', #31892, #16783, #7142 ) ;
#29089=EDGE_CURVE ( 'NONE', #22037, #28828, #20067, .T. ) ;
#29090=EDGE_CURVE ( 'NONE', #50637, #49359, #33037, .T. ) ;
#29092=CARTESIAN_POINT ( 'NONE',  ( 2.229367062499998831, 18.35416666803225993, -3.861377020970580887 ) ) ;
#29100=CARTESIAN_POINT ( 'NONE',  ( -4.458734124999999437, -62.39583333196774362, -2.574251347313719407 ) ) ;
#29101=CARTESIAN_POINT ( 'NONE',  ( 0.000000000000000000, -120.0000000000000000, 5.000000000000000000 ) ) ;
#29102=CARTESIAN_POINT ( 'NONE',  ( 4.458734125000001214, 16.10416666803225993, 2.574251347313718519 ) ) ;
#29104=CARTESIAN_POINT ( 'NONE',  ( 4.330127018922154569, 30.00000000000000000, -7.499999999999971578 ) ) ;
#29105=CARTESIAN_POINT ( 'NONE',  ( -4.458734124999999437, -49.64583333196772941, -2.574251347313719407 ) ) ;
#29106=CARTESIAN_POINT ( 'NONE',  ( -2.500000000000000444, -2.041666663935480575, -4.330127018922193649 ) ) ;
#29109=CYLINDRICAL_SURFACE ( 'NONE', #26562, 5.000000000000000000 ) ;
#29111=CARTESIAN_POINT ( 'NONE',  ( -2.229367062500000163, -108.4791666653010651, -3.861377020970580443 ) ) ;
#29112=CARTESIAN_POINT ( 'NONE',  ( -4.458734124999997661, -13.47916666530107221, 2.574251347313722516 ) ) ;
#29114=ORIENTED_EDGE ( 'NONE', *, *, #16671, .T. ) ;
#29116=CARTESIAN_POINT ( 'NONE',  ( -2.229367062499996610, -100.1458333319677365, 3.861377020970582219 ) ) ;
#29118=CARTESIAN_POINT ( 'NONE',  ( 4.458734125000001214, -90.14583333196773651, 2.574251347313718519 ) ) ;
#29119=DIRECTION ( 'NONE',  ( -0.000000000000000000, 1.000000000000000000, -0.000000000000000000 ) ) ;
#29120=CARTESIAN_POINT ( 'NONE',  ( 1.060575238724906964E-15, -50.62499999726881583, 5.773502691896257311 ) ) ;
#29124=CARTESIAN_POINT ( 'NONE',  ( 2.229367062499998831, -15.64583333196773651, -3.861377020970580887 ) ) ;
#29125=CARTESIAN_POINT ( 'NONE',  ( 4.458734124999999437, 9.937500001365593860, -5.460374474430324690E-16 ) ) ;
#29126=CARTESIAN_POINT ( 'NONE',  ( -3.152548672688508926E-16, -60.81249999863440081, -5.148502694627439702 ) ) ;
#29127=CARTESIAN_POINT ( 'NONE',  ( -4.999999999999998224, -68.91666666666667140, 2.886751345948131764 ) ) ;
#29131=CARTESIAN_POINT ( 'NONE',  ( 2.499999999999998668, -7.333333333333330373, -4.330127018922193649 ) ) ;
#29132=ORIENTED_EDGE ( 'NONE', *, *, #4279, .F. ) ;
#29134=FACE_OUTER_BOUND ( 'NONE', #14521, .T. ) ;
#29136=LINE ( 'NONE', #13432, #44996 ) ;
#29137=CARTESIAN_POINT ( 'NONE',  ( -3.152548672688508926E-16, -87.56249999863440792, -5.148502694627439702 ) ) ;
#29138=CARTESIAN_POINT ( 'NONE',  ( -4.458734124999999437, 17.43750000136559208, 0.000000000000000000 ) ) ;
#29139=VECTOR ( 'NONE', #49669, 1000.000000000000000 ) ;
#29145=CARTESIAN_POINT ( 'NONE',  ( 2.499999999999998668, -74.33333333333332860, -4.330127018922193649 ) ) ;
#29148=CYLINDRICAL_SURFACE ( 'NONE', #10969, 5.000000000000000000 ) ;
#29150=ORIENTED_EDGE ( 'NONE', *, *, #43262, .F. ) ;
#29160=ORIENTED_EDGE ( 'NONE', *, *, #18546, .T. ) ;
#29163=CARTESIAN_POINT ( 'NONE',  ( -4.458734124999999437, -56.56249999863440081, 0.000000000000000000 ) ) ;
#29164=( BOUNDED_CURVE ( )  B_SPLINE_CURVE ( 2, ( #11009, #30631, #50253, #25816, #1394, #57318, #28023, #52792, #2647 ),
 .UNSPECIFIED., .F., .F. ) 
 B_SPLINE_CURVE_WITH_KNOTS ( ( 3, 2, 2, 2, 3 ),
 ( 0.9053571428571428603, 0.9059523809523809534, 0.9071428571428571397, 0.9083333333333333259, 0.9089285714285714191 ),
 .UNSPECIFIED. ) 
 CURVE ( )  GEOMETRIC_REPRESENTATION_ITEM ( )  RATIONAL_B_SPLINE_CURVE ( ( 0.9330127018922194093, 0.9330127018922194093, 1.000000000000000000, 0.8660254037844387076, 1.000000000000000000, 0.8660254037844387076, 1.000000000000000000, 0.9330127018922194093, 0.9330127018922194093 ) ) 
 REPRESENTATION_ITEM ( '' )  );
#29171=ADVANCED_FACE ( 'NONE', ( #52653 ), #57802, .T. ) ;
#29174=CARTESIAN_POINT ( 'NONE',  ( -3.152548672688508926E-16, -102.8124999986344221, -5.148502694627439702 ) ) ;
#29176=ORIENTED_EDGE ( 'NONE', *, *, #31046, .F. ) ;
#29179=CARTESIAN_POINT ( 'NONE',  ( 2.229367062499998831, -38.64583333196773651, -3.861377020970580887 ) ) ;
#29181=CARTESIAN_POINT ( 'NONE',  ( -1.339745962155585168, -2.205341801261480938, -5.000000000000015987 ) ) ;
#29182=CARTESIAN_POINT ( 'NONE',  ( 4.458734124999998549, -11.72916666530107044, -2.574251347313721627 ) ) ;
#29183=CARTESIAN_POINT ( 'NONE',  ( 9.457646018065525792E-16, -100.3124999986343937, 5.148502694627439702 ) ) ;
#29186=CARTESIAN_POINT ( 'NONE',  ( 4.458734125000001214, -31.14583333196773651, 2.574251347313718519 ) ) ;
#29191=CARTESIAN_POINT ( 'NONE',  ( 2.500000000000002220, -17.66666666666666430, 4.330127018922192761 ) ) ;
#29194=CARTESIAN_POINT ( 'NONE',  ( -4.458734124999997661, 4.520833334698926897, 2.574251347313722516 ) ) ;
#29195=ORIENTED_EDGE ( 'NONE', *, *, #1286, .T. ) ;
#29196=DIRECTION ( 'NONE',  ( -0.000000000000000000, 1.000000000000000000, -0.000000000000000000 ) ) ;
#29198=CARTESIAN_POINT ( 'NONE',  ( 1.975475456537005874E-15, -42.62499999726880873, 5.000000000000000000 ) ) ;
#29199=CARTESIAN_POINT ( 'NONE',  ( -5.000000000000000000, -96.00000000000000000, 0.000000000000000000 ) ) ;
#29200=CARTESIAN_POINT ( 'NONE',  ( -2.229367062500000163, -32.47916666530106511, -3.861377020970580443 ) ) ;
#29201=CARTESIAN_POINT ( 'NONE',  ( -6.972266317189433020E-16, -36.25000000000000000, -5.000000000000000000 ) ) ;
#29202=CARTESIAN_POINT ( 'NONE',  ( 4.458734124999998549, -77.97916666530106511, -2.574251347313721627 ) ) ;
#29206=CARTESIAN_POINT ( 'NONE',  ( 2.229367062499998831, -4.645833331967740065, -3.861377020970580887 ) ) ;
#29207=CARTESIAN_POINT ( 'NONE',  ( 4.458734125000001214, 25.85416666803225638, 2.574251347313718519 ) ) ;
#29208=CARTESIAN_POINT ( 'NONE',  ( 2.229367062499998831, -40.89583333196773651, -3.861377020970580887 ) ) ;
#29213=CARTESIAN_POINT ( 'NONE',  ( 4.458734125000001214, -66.89583333196773651, 2.574251347313718519 ) ) ;
#29214=CARTESIAN_POINT ( 'NONE',  ( -5.000000000000000000, -107.9583333306021444, -2.886751345948128211 ) ) ;
#29219=CARTESIAN_POINT ( 'NONE',  ( -5.000000000000000000, -53.08333333333332860, -2.886751345948128211 ) ) ;
#29223=FACE_OUTER_BOUND ( 'NONE', #56744, .T. ) ;
#29224=DIRECTION ( 'NONE',  ( -0.000000000000000000, 1.000000000000000000, -0.000000000000000000 ) ) ;
#29233=CARTESIAN_POINT ( 'NONE',  ( -2.499999999999996447, -23.83333333333333215, 4.330127018922195425 ) ) ;
#29236=ORIENTED_EDGE ( 'NONE', *, *, #9875, .T. ) ;
#29240=CARTESIAN_POINT ( 'NONE',  ( 4.458734124999998549, -42.97916666530107221, -2.574251347313721627 ) ) ;
#29243=CYLINDRICAL_SURFACE ( 'NONE', #55992, 5.000000000000000000 ) ;
#29250=CARTESIAN_POINT ( 'NONE',  ( 9.457646018065525792E-16, -90.31249999863439371, 5.148502694627439702 ) ) ;
#29252=VERTEX_POINT ( 'NONE', #28826 ) ;
#29253=CARTESIAN_POINT ( 'NONE',  ( 0.000000000000000000, -120.0000000000000000, 5.000000000000000000 ) ) ;
#29257=ORIENTED_EDGE ( 'NONE', *, *, #43199, .F. ) ;
#29258=CARTESIAN_POINT ( 'NONE',  ( -4.999999999999998224, -13.91666666666666785, 2.886751345948131764 ) ) ;
#29259=CARTESIAN_POINT ( 'NONE',  ( 4.458734125000001214, -14.14583333196774184, 2.574251347313718519 ) ) ;
#29260=CARTESIAN_POINT ( 'NONE',  ( -1.339745962155613812, -35.20534180126148271, -5.000000000000000000 ) ) ;
#29264=CARTESIAN_POINT ( 'NONE',  ( 9.457646018065525792E-16, 18.68750000136559208, 5.148502694627439702 ) ) ;
#29266=CARTESIAN_POINT ( 'NONE',  ( 2.229367062500001939, -98.97916666530105090, 3.861377020970579999 ) ) ;
#29268=CARTESIAN_POINT ( 'NONE',  ( -4.458734124999999437, -14.31249999863440436, 0.000000000000000000 ) ) ;
#29269=CARTESIAN_POINT ( 'NONE',  ( 0.000000000000000000, -120.0000000000000000, 0.000000000000000000 ) ) ;
#29271=CARTESIAN_POINT ( 'NONE',  ( -1.339745962155610925, -87.79465819873851729, 5.000000000000000000 ) ) ;
#29272=CARTESIAN_POINT ( 'NONE',  ( -2.499999999999996447, -43.70833333060214443, 4.330127018922195425 ) ) ;
#29273=DIRECTION ( 'NONE',  ( 0.000000000000000000, 0.000000000000000000, 1.000000000000000000 ) ) ;
#29274=CARTESIAN_POINT ( 'NONE',  ( 2.229367062500001939, 16.02083333469892779, 3.861377020970579999 ) ) ;
#29278=CARTESIAN_POINT ( 'NONE',  ( 4.458734125000001214, -62.89583333196775072, 2.574251347313718519 ) ) ;
#29281=CARTESIAN_POINT ( 'NONE',  ( -3.535250795749689387E-16, 11.74999999999999822, -5.773502691896257311 ) ) ;
#29284=CARTESIAN_POINT ( 'NONE',  ( 4.458734124999999437, -55.81249999863440081, -5.460374474430324690E-16 ) ) ;
#29285=CARTESIAN_POINT ( 'NONE',  ( 1.060575238724906964E-15, -87.62499999726880162, 5.773502691896257311 ) ) ;
#29288=LINE ( 'NONE', #34436, #46012 ) ;
#29290=( BOUNDED_CURVE ( )  B_SPLINE_CURVE ( 2, ( #6317, #60355, #50686, #35579, #55206, #36527, #32019, #26888, #40391 ),
 .UNSPECIFIED., .F., .F. ) 
 B_SPLINE_CURVE_WITH_KNOTS ( ( 3, 2, 2, 2, 3 ),
 ( 0.1946428571428571452, 0.1952380952380952384, 0.1964285714285714246, 0.1976190476190476109, 0.1982142857142857040 ),
 .UNSPECIFIED. ) 
 CURVE ( )  GEOMETRIC_REPRESENTATION_ITEM ( )  RATIONAL_B_SPLINE_CURVE ( ( 0.9330127018922194093, 0.9330127018922194093, 1.000000000000000000, 0.8660254037844387076, 1.000000000000000000, 0.8660254037844387076, 1.000000000000000000, 0.9330127018922194093, 0.9330127018922194093 ) ) 
 REPRESENTATION_ITEM ( '' )  );
#29291=CARTESIAN_POINT ( 'NONE',  ( -5.000000000000000000, -36.00000000000000711, 0.000000000000000000 ) ) ;
#29295=CARTESIAN_POINT ( 'NONE',  ( 4.458734124999998549, -99.72916666530105090, -2.574251347313721627 ) ) ;
#29296=CARTESIAN_POINT ( 'NONE',  ( -2.229367062500000163, 2.270833334698928230, -3.861377020970580443 ) ) ;
#29297=CARTESIAN_POINT ( 'NONE',  ( 2.499999999999998668, -80.33333333333332860, -4.330127018922193649 ) ) ;
#29303=ORIENTED_EDGE ( 'NONE', *, *, #21379, .T. ) ;
#29304=LINE ( 'NONE', #63123, #49160 ) ;
#29308=CARTESIAN_POINT ( 'NONE',  ( 4.458734124999999437, -24.06249999863440436, -5.460374474430324690E-16 ) ) ;
#29313=AXIS2_PLACEMENT_3D ( 'NONE', #49541, #6452, #29915 ) ;
#29317=CARTESIAN_POINT ( 'NONE',  ( -1.339745962155613812, -83.08034179853028434, -5.000000000000000000 ) ) ;
#29318=VERTEX_POINT ( 'NONE', #3770 ) ;
#29319=CARTESIAN_POINT ( 'NONE',  ( 2.229367062499998831, -74.89583333196773651, -3.861377020970580887 ) ) ;
#29323=CARTESIAN_POINT ( 'NONE',  ( 1.339745962155670655, -20.16965819600734022, -4.999999999999966249 ) ) ;
#29326=CARTESIAN_POINT ( 'NONE',  ( 4.458734125000001214, 1.854166668032262155, 2.574251347313718519 ) ) ;
#29327=ORIENTED_EDGE ( 'NONE', *, *, #55522, .F. ) ;
#29328=CARTESIAN_POINT ( 'NONE',  ( -2.499999999999996447, -19.83333333333333570, 4.330127018922195425 ) ) ;
#29329=CARTESIAN_POINT ( 'NONE',  ( 0.000000000000000000, 30.00000000000000000, 0.000000000000000000 ) ) ;
#29334=( BOUNDED_CURVE ( )  B_SPLINE_CURVE ( 2, ( #34243, #43578, #42961, #62604, #4356, #63221, #38147, #4055, #43271 ),
 .UNSPECIFIED., .F., .F. ) 
 B_SPLINE_CURVE_WITH_KNOTS ( ( 3, 2, 2, 2, 3 ),
 ( 0.2374999999999999889, 0.2380952380952380820, 0.2392857142857142960, 0.2404761904761904823, 0.2410714285714285754 ),
 .UNSPECIFIED. ) 
 CURVE ( )  GEOMETRIC_REPRESENTATION_ITEM ( )  RATIONAL_B_SPLINE_CURVE ( ( 0.9330127018922194093, 0.9330127018922194093, 1.000000000000000000, 0.8660254037844387076, 1.000000000000000000, 0.8660254037844387076, 1.000000000000000000, 0.9330127018922194093, 0.9330127018922194093 ) ) 
 REPRESENTATION_ITEM ( '' )  );
#29335=VERTEX_POINT ( 'NONE', #48447 ) ;
#29336=CARTESIAN_POINT ( 'NONE',  ( -2.229367062500000163, -75.47916666530106511, -3.861377020970580443 ) ) ;
#29338=CARTESIAN_POINT ( 'NONE',  ( 2.229367062500001939, 3.020833334698928674, 3.861377020970579999 ) ) ;
#29340=CARTESIAN_POINT ( 'NONE',  ( -2.229367062499996610, -65.39583333196773651, 3.861377020970582219 ) ) ;
#29341=CARTESIAN_POINT ( 'NONE',  ( 2.499999999999998668, -25.20833333060214443, -4.330127018922193649 ) ) ;
#29342=DIRECTION ( 'NONE',  ( -0.000000000000000000, 1.000000000000000000, -0.000000000000000000 ) ) ;
#29343=CARTESIAN_POINT ( 'NONE',  ( 5.000000000000000888, -28.45833333060214443, 2.886751345948126879 ) ) ;
#29345=CARTESIAN_POINT ( 'NONE',  ( 1.975475456537005874E-15, -3.624999997268814056, 5.000000000000000000 ) ) ;
#29346=CARTESIAN_POINT ( 'NONE',  ( 2.229367062499998831, -47.64583333196774362, -3.861377020970580887 ) ) ;
#29347=CARTESIAN_POINT ( 'NONE',  ( 4.458734125000000326, -26.14583333196773651, 2.574251347313718519 ) ) ;
#29350=CARTESIAN_POINT ( 'NONE',  ( -5.000000000000000000, 27.99999999999999645, 0.000000000000000000 ) ) ;
#29353=CARTESIAN_POINT ( 'NONE',  ( 2.229367062500001939, -39.97916666530107221, 3.861377020970579999 ) ) ;
#29354=CARTESIAN_POINT ( 'NONE',  ( 2.500000000000002220, -74.54166666393547303, 4.330127018922192761 ) ) ;
#29359=CARTESIAN_POINT ( 'NONE',  ( 4.458734124999998549, -76.97916666530106511, -2.574251347313721627 ) ) ;
#29362=DIRECTION ( 'NONE',  ( -0.000000000000000000, 1.000000000000000000, -0.000000000000000000 ) ) ;
#29364=CARTESIAN_POINT ( 'NONE',  ( -3.535250795749689387E-16, -23.25000000000000000, -5.773502691896257311 ) ) ;
#29366=VERTEX_POINT ( 'NONE', #38180 ) ;
#29368=EDGE_LOOP ( 'NONE', ( #31251, #2390, #34092, #35524 ) ) ;
#29370=CARTESIAN_POINT ( 'NONE',  ( -3.535250795749689387E-16, 21.87500000273118062, -5.773502691896257311 ) ) ;
#29371=CARTESIAN_POINT ( 'NONE',  ( -6.972266317189433020E-16, 4.875000002731184168, -5.000000000000000000 ) ) ;
#29378=CARTESIAN_POINT ( 'NONE',  ( 1.975475456537005874E-15, -12.74999999999999822, 5.000000000000000000 ) ) ;
#29379=CARTESIAN_POINT ( 'NONE',  ( -2.916731409357579869E-14, 18.24999999999999645, 5.000000000000000888 ) ) ;
#29380=CARTESIAN_POINT ( 'NONE',  ( -3.152548672688508926E-16, -23.56249999863440436, -5.148502694627439702 ) ) ;
#29381=CARTESIAN_POINT ( 'NONE',  ( 2.499999999999998668, 10.79166666939785202, -4.330127018922193649 ) ) ;
#29391=CARTESIAN_POINT ( 'NONE',  ( 0.000000000000000000, -114.9999999999999858, 0.000000000000000000 ) ) ;
#29394=AXIS2_PLACEMENT_3D ( 'NONE', #52117, #27663, #42766 ) ;
#29395=DIRECTION ( 'NONE',  ( -0.000000000000000000, 1.000000000000000000, -0.000000000000000000 ) ) ;
#29397=CARTESIAN_POINT ( 'NONE',  ( -6.972266317189433020E-16, -13.25000000000000000, -5.000000000000000000 ) ) ;
#29400=EDGE_CURVE ( 'NONE', #7429, #32043, #25274, .T. ) ;
#29402=CARTESIAN_POINT ( 'NONE',  ( 9.457646018065525792E-16, 17.93750000136559208, 5.148502694627439702 ) ) ;
#29404=VERTEX_POINT ( 'NONE', #11433 ) ;
#29408=CARTESIAN_POINT ( 'NONE',  ( 5.000000000000000000, -100.5000000000000000, -6.123233995736766282E-16 ) ) ;
#29410=CARTESIAN_POINT ( 'NONE',  ( -4.458734124999997661, -58.22916666530106511, 2.574251347313722516 ) ) ;
#29411=CARTESIAN_POINT ( 'NONE',  ( 0.000000000000000000, -120.0000000000000000, 5.000000000000000000 ) ) ;
#29412=CARTESIAN_POINT ( 'NONE',  ( -3.152548672688508926E-16, 15.43750000136559564, -5.148502694627439702 ) ) ;
#29413=( BOUNDED_CURVE ( )  B_SPLINE_CURVE ( 2, ( #17350, #7393, #51140, #41461, #27628, #12206, #62055, #56602, #27000 ),
 .UNSPECIFIED., .F., .F. ) 
 B_SPLINE_CURVE_WITH_KNOTS ( ( 3, 2, 2, 2, 3 ),
 ( 0.5446428571428570953, 0.5452380952380951884, 0.5464285714285713746, 0.5476190476190476719, 0.5482142857142857650 ),
 .UNSPECIFIED. ) 
 CURVE ( )  GEOMETRIC_REPRESENTATION_ITEM ( )  RATIONAL_B_SPLINE_CURVE ( ( 0.9330127018922194093, 0.9330127018922194093, 1.000000000000000000, 0.8660254037844387076, 1.000000000000000000, 0.8660254037844387076, 1.000000000000000000, 0.9330127018922194093, 0.9330127018922194093 ) ) 
 REPRESENTATION_ITEM ( '' )  );
#29415=CARTESIAN_POINT ( 'NONE',  ( 4.458734124999998549, -47.97916666530107221, -2.574251347313721627 ) ) ;
#29416=ADVANCED_FACE ( 'NONE', ( #20777 ), #49399, .T. ) ;
#29417=CARTESIAN_POINT ( 'NONE',  ( 2.500000000000002220, -7.541666663935481907, 4.330127018922192761 ) ) ;
#29419=LINE ( 'NONE', #14331, #46072 ) ;
#29420=CARTESIAN_POINT ( 'NONE',  ( -1.339745962155610925, -73.79465819873853150, 5.000000000000000000 ) ) ;
#29421=CARTESIAN_POINT ( 'NONE',  ( -3.152548672688508926E-16, -107.5624999986343937, -5.148502694627439702 ) ) ;
#29422=CARTESIAN_POINT ( 'NONE',  ( 4.458734124999998549, -10.97916666530107044, -2.574251347313721627 ) ) ;
#29423=ORIENTED_EDGE ( 'NONE', *, *, #40113, .F. ) ;
#29425=CARTESIAN_POINT ( 'NONE',  ( -2.229367062500000163, -99.47916666530106511, -3.861377020970580443 ) ) ;
#29427=CARTESIAN_POINT ( 'NONE',  ( -4.458734124999998549, -99.47916666530105090, 2.574251347313722516 ) ) ;
#29428=CARTESIAN_POINT ( 'NONE',  ( -1.339745962155610925, -7.794658198738519950, 5.000000000000000000 ) ) ;
#29429=CARTESIAN_POINT ( 'NONE',  ( -4.999999999999999112, -56.79166666393548013, 2.886751345948131764 ) ) ;
#29430=CARTESIAN_POINT ( 'NONE',  ( -5.000000000000000000, -36.87499999726881583, 0.000000000000000000 ) ) ;
#29434=CARTESIAN_POINT ( 'NONE',  ( 4.458734125000000326, -15.89583333196773651, 2.574251347313718519 ) ) ;
#29435=CARTESIAN_POINT ( 'NONE',  ( -4.458734124999999437, 8.437500001365595637, 0.000000000000000000 ) ) ;
#29436=CARTESIAN_POINT ( 'NONE',  ( -4.458734124999999437, -58.64583333196773651, -2.574251347313719407 ) ) ;
#29437=CARTESIAN_POINT ( 'NONE',  ( 0.000000000000000000, -120.0000000000000000, 0.000000000000000000 ) ) ;
#29441=CARTESIAN_POINT ( 'NONE',  ( -3.535250795749689387E-16, -8.250000000000000000, -5.773502691896257311 ) ) ;
#29446=CARTESIAN_POINT ( 'NONE',  ( -2.229367062500000163, -85.47916666530107932, -3.861377020970580443 ) ) ;
#29447=CARTESIAN_POINT ( 'NONE',  ( -4.458734124999999437, 18.43750000136559564, 0.000000000000000000 ) ) ;
#29451=ADVANCED_FACE ( 'NONE', ( #40382 ), #44895, .T. ) ;
#29452=ADVANCED_FACE ( 'NONE', ( #49716 ), #855, .T. ) ;
#29453=CARTESIAN_POINT ( 'NONE',  ( 1.975475456537005874E-15, -93.74999999999998579, 5.000000000000000000 ) ) ;
#29458=CARTESIAN_POINT ( 'NONE',  ( -5.000000000000000000, -73.08333333333334281, -2.886751345948128211 ) ) ;
#29460=ORIENTED_EDGE ( 'NONE', *, *, #62903, .T. ) ;
#29461=CARTESIAN_POINT ( 'NONE',  ( 5.000000000000000000, -102.5000000000000142, -6.123233995736766282E-16 ) ) ;
#29472=ORIENTED_EDGE ( 'NONE', *, *, #55804, .F. ) ;
#29475=CARTESIAN_POINT ( 'NONE',  ( -2.229367062500000163, -59.72916666530106511, -3.861377020970580443 ) ) ;
#29481=ORIENTED_EDGE ( 'NONE', *, *, #53011, .T. ) ;
#29483=CARTESIAN_POINT ( 'NONE',  ( -4.458734124999999437, -103.6458333319677223, -2.574251347313719407 ) ) ;
#29488=CARTESIAN_POINT ( 'NONE',  ( 4.458734124999998549, -37.72916666530107221, -2.574251347313721627 ) ) ;
#29490=( BOUNDED_CURVE ( )  B_SPLINE_CURVE ( 2, ( #13098, #2828, #13722, #52025, #61369, #47811, #56859, #52345, #57495 ),
 .UNSPECIFIED., .F., .F. ) 
 B_SPLINE_CURVE_WITH_KNOTS ( ( 3, 2, 2, 2, 3 ),
 ( 0.9696428571428571397, 0.9702380952380952328, 0.9714285714285714191, 0.9726190476190476053, 0.9732142857142856984 ),
 .UNSPECIFIED. ) 
 CURVE ( )  GEOMETRIC_REPRESENTATION_ITEM ( )  RATIONAL_B_SPLINE_CURVE ( ( 0.9330127018922194093, 0.9330127018922194093, 1.000000000000000000, 0.8660254037844387076, 1.000000000000000000, 0.8660254037844387076, 1.000000000000000000, 0.9330127018922194093, 0.9330127018922194093 ) ) 
 REPRESENTATION_ITEM ( '' )  );
#29495=CARTESIAN_POINT ( 'NONE',  ( -4.458734124999999437, -13.31249999863440259, 0.000000000000000000 ) ) ;
#29497=CARTESIAN_POINT ( 'NONE',  ( 4.458734124999998549, -101.9791666653010651, -2.574251347313721627 ) ) ;
#29500=CARTESIAN_POINT ( 'NONE',  ( -4.458734124999999437, -32.64583333196774362, -2.574251347313719407 ) ) ;
#29501=VECTOR ( 'NONE', #62912, 1000.000000000000000 ) ;
#29502=CARTESIAN_POINT ( 'NONE',  ( -5.000000000000000000, 5.125000002731184168, 0.000000000000000000 ) ) ;
#29508=CARTESIAN_POINT ( 'NONE',  ( -3.152548672688508926E-16, 6.187500001365593860, -5.148502694627439702 ) ) ;
#29509=EDGE_LOOP ( 'NONE', ( #38410, #47913, #2223, #1321 ) ) ;
#29510=CARTESIAN_POINT ( 'NONE',  ( -1.339745962155613812, 1.794658198738520616, -5.000000000000000000 ) ) ;
#29512=CARTESIAN_POINT ( 'NONE',  ( -5.000000000000000000, -95.00000000000000000, 0.000000000000000000 ) ) ;
#29513=CARTESIAN_POINT ( 'NONE',  ( 4.458734125000001214, -28.89583333196774007, 2.574251347313718519 ) ) ;
#29514=CARTESIAN_POINT ( 'NONE',  ( 5.000000000000000000, -9.416666666666662522, -2.886751345948130876 ) ) ;
#29515=CARTESIAN_POINT ( 'NONE',  ( -4.458734124999999437, -81.64583333196773651, -2.574251347313719407 ) ) ;
#29519=CARTESIAN_POINT ( 'NONE',  ( 4.458734124999998549, -2.729166665301069550, -2.574251347313721627 ) ) ;
#29520=CARTESIAN_POINT ( 'NONE',  ( -4.458734124999998549, 23.52083333469892779, 2.574251347313722516 ) ) ;
#29521=CARTESIAN_POINT ( 'NONE',  ( -4.458734124999997661, -41.47916666530107932, 2.574251347313722516 ) ) ;
#29522=CARTESIAN_POINT ( 'NONE',  ( 1.975475456537005874E-15, -9.750000000000000000, 5.000000000000000000 ) ) ;
#29525=( BOUNDED_CURVE ( )  B_SPLINE_CURVE ( 2, ( #19105, #14918, #34525, #58043, #38722, #53220, #59309, #44185, #58989 ),
 .UNSPECIFIED., .F., .F. ) 
 B_SPLINE_CURVE_WITH_KNOTS ( ( 3, 2, 2, 2, 3 ),
 ( 0.7624999999999999556, 0.7630952380952380487, 0.7642857142857142350, 0.7654761904761904212, 0.7660714285714286254 ),
 .UNSPECIFIED. ) 
 CURVE ( )  GEOMETRIC_REPRESENTATION_ITEM ( )  RATIONAL_B_SPLINE_CURVE ( ( 0.9330127018922194093, 0.9330127018922194093, 1.000000000000000000, 0.8660254037844387076, 1.000000000000000000, 0.8660254037844387076, 1.000000000000000000, 0.9330127018922130810, 0.9330127018922194093 ) ) 
 REPRESENTATION_ITEM ( '' )  );
#29526=CARTESIAN_POINT ( 'NONE',  ( 4.458734124999998549, -70.72916666530107932, -2.574251347313721627 ) ) ;
#29527=CARTESIAN_POINT ( 'NONE',  ( 2.499999999999998668, -103.2083333306021444, -4.330127018922193649 ) ) ;
#29529=EDGE_CURVE ( 'NONE', #3800, #34229, #20458, .T. ) ;
#29532=CARTESIAN_POINT ( 'NONE',  ( 4.458734124999999437, -110.0624999986343937, -5.460374474430324690E-16 ) ) ;
#29534=CARTESIAN_POINT ( 'NONE',  ( -2.499999999999996447, -59.83333333333333570, 4.330127018922195425 ) ) ;
#29535=EDGE_CURVE ( 'NONE', #12722, #12555, #17639, .T. ) ;
#29540=VECTOR ( 'NONE', #41312, 1000.000000000000000 ) ;
#29547=EDGE_CURVE ( 'NONE', #20024, #12722, #4108, .T. ) ;
#29552=CARTESIAN_POINT ( 'NONE',  ( -1.339745962155610925, -75.66965819600731891, 5.000000000000000000 ) ) ;
#29555=VERTEX_POINT ( 'NONE', #46490 ) ;
#29558=EDGE_CURVE ( 'NONE', #63269, #51535, #51326, .T. ) ;
#29560=CARTESIAN_POINT ( 'NONE',  ( 2.229367062500001939, -43.22916666530107932, 3.861377020970579999 ) ) ;
#29563=EDGE_CURVE ( 'NONE', #4102, #454, #6941, .T. ) ;
#29565=CARTESIAN_POINT ( 'NONE',  ( -6.972266317189433020E-16, -26.12499999726881583, -5.000000000000000000 ) ) ;
#29571=CARTESIAN_POINT ( 'NONE',  ( 4.458734124999999437, -89.06249999863439371, -5.460374474430324690E-16 ) ) ;
#29572=CARTESIAN_POINT ( 'NONE',  ( 5.000000000000000000, -108.4999999999999858, -6.123233995736766282E-16 ) ) ;
#29573=ORIENTED_EDGE ( 'NONE', *, *, #27101, .T. ) ;
#29579=CARTESIAN_POINT ( 'NONE',  ( -4.458734124999999437, 1.604166668032262155, -2.574251347313719407 ) ) ;
#29580=CARTESIAN_POINT ( 'NONE',  ( -2.500000000000000444, -71.04166666393547303, -4.330127018922193649 ) ) ;
#29581=CARTESIAN_POINT ( 'NONE',  ( -2.229367062499996610, -18.39583333196774007, 3.861377020970582219 ) ) ;
#29584=CARTESIAN_POINT ( 'NONE',  ( -2.480964764533239819E-13, -73.62499999726883004, 5.000000000000000000 ) ) ;
#29587=CARTESIAN_POINT ( 'NONE',  ( 4.458734125000000326, 22.85416666803225993, 2.574251347313718519 ) ) ;
#29589=CARTESIAN_POINT ( 'NONE',  ( -4.458734124999999437, -98.31249999863440792, 0.000000000000000000 ) ) ;
#29590=DIRECTION ( 'NONE',  ( 0.000000000000000000, 0.000000000000000000, 1.000000000000000000 ) ) ;
#29592=CARTESIAN_POINT ( 'NONE',  ( 4.458734125000001214, -11.89583333196774007, 2.574251347313718519 ) ) ;
#29596=CARTESIAN_POINT ( 'NONE',  ( 1.060575238724906964E-15, -39.62499999726880873, 5.773502691896257311 ) ) ;
#29597=CARTESIAN_POINT ( 'NONE',  ( 1.339745962155612702, -67.16965819600733312, -5.000000000000000000 ) ) ;
#29598=CARTESIAN_POINT ( 'NONE',  ( 2.229367062500001939, 12.02083333469892601, 3.861377020970579999 ) ) ;
#29599=CARTESIAN_POINT ( 'NONE',  ( 1.339745962155615144, -51.58034179853028434, 4.999999999999999112 ) ) ;
#29603=CARTESIAN_POINT ( 'NONE',  ( 4.458734124999998549, -61.72916666530106511, -2.574251347313721627 ) ) ;
#29606=CARTESIAN_POINT ( 'NONE',  ( 5.000000000000000000, -109.3749999972688016, -6.123233995736766282E-16 ) ) ;
#29607=CARTESIAN_POINT ( 'NONE',  ( -4.999999999999999112, 5.083333333333332149, 2.886751345948131764 ) ) ;
#29610=CARTESIAN_POINT ( 'NONE',  ( 2.229367062499998831, -51.64583333196773651, -3.861377020970580887 ) ) ;
#29611=CARTESIAN_POINT ( 'NONE',  ( -5.000000000000000000, -86.95833333060214443, -2.886751345948128211 ) ) ;
#29612=CARTESIAN_POINT ( 'NONE',  ( 4.458734125000000326, -33.89583333196772941, 2.574251347313718519 ) ) ;
#29618=CARTESIAN_POINT ( 'NONE',  ( 2.500000000000002220, -42.66666666666667140, 4.330127018922192761 ) ) ;
#29622=CARTESIAN_POINT ( 'NONE',  ( 2.229367062499998831, -101.6458333319677365, -3.861377020970580887 ) ) ;
#29623=CARTESIAN_POINT ( 'NONE',  ( 2.229367062499998831, 4.104166668032260823, -3.861377020970580887 ) ) ;
#29631=VERTEX_POINT ( 'NONE', #2438 ) ;
#29635=CARTESIAN_POINT ( 'NONE',  ( -6.972266317189433020E-16, -100.1249999972688016, -5.000000000000000000 ) ) ;
#29638=CARTESIAN_POINT ( 'NONE',  ( 9.457646018065525792E-16, -24.31249999863440792, 5.148502694627439702 ) ) ;
#29647=EDGE_CURVE ( 'NONE', #1425, #37461, #23824, .T. ) ;
#29649=CARTESIAN_POINT ( 'NONE',  ( 1.975475456537005874E-15, -82.62499999726878741, 5.000000000000000000 ) ) ;
#29650=ORIENTED_EDGE ( 'NONE', *, *, #47515, .F. ) ;
#29651=CARTESIAN_POINT ( 'NONE',  ( 2.229367062500001939, -71.22916666530107932, 3.861377020970579999 ) ) ;
#29652=CARTESIAN_POINT ( 'NONE',  ( -5.000000000000000000, 28.91666666666666430, -2.886751345948128211 ) ) ;
#29655=DIRECTION ( 'NONE',  ( -3.614007241618347908E-17, 0.000000000000000000, -1.000000000000000000 ) ) ;
#29658=CARTESIAN_POINT ( 'NONE',  ( 2.229367062499998831, -1.895833331967737623, -3.861377020970580887 ) ) ;
#29659=ORIENTED_EDGE ( 'NONE', *, *, #22758, .T. ) ;
#29661=CARTESIAN_POINT ( 'NONE',  ( -5.000000000000000000, -45.08333333333333570, -2.886751345948128211 ) ) ;
#29664=FACE_OUTER_BOUND ( 'NONE', #56272, .T. ) ;
#29667=CARTESIAN_POINT ( 'NONE',  ( -4.458734124999999437, -83.39583333196773651, -2.574251347313719407 ) ) ;
#29668=CARTESIAN_POINT ( 'NONE',  ( -4.458734124999999437, -0.3958333319677397322, -2.574251347313719407 ) ) ;
#29669=CARTESIAN_POINT ( 'NONE',  ( 5.000000000000000000, -83.49999999999998579, -6.123233995736766282E-16 ) ) ;
#29671=CARTESIAN_POINT ( 'NONE',  ( -4.458734124999998549, -66.47916666530106511, 2.574251347313722516 ) ) ;
#29672=CARTESIAN_POINT ( 'NONE',  ( -2.500000000000000444, -27.04166666393548013, -4.330127018922193649 ) ) ;
#29673=FACE_OUTER_BOUND ( 'NONE', #12697, .T. ) ;
#29674=CARTESIAN_POINT ( 'NONE',  ( -2.229367062500000163, 27.52083333469892779, -3.861377020970580443 ) ) ;
#29675=CARTESIAN_POINT ( 'NONE',  ( -2.500000000000000444, -65.04166666393547303, -4.330127018922193649 ) ) ;
#29677=DIRECTION ( 'NONE',  ( -0.000000000000000000, 1.000000000000000000, -0.000000000000000000 ) ) ;
#29678=CARTESIAN_POINT ( 'NONE',  ( 2.229367062499998831, -43.64583333196773651, -3.861377020970580887 ) ) ;
#29679=CARTESIAN_POINT ( 'NONE',  ( -4.458734124999999437, -32.64583333196773651, -2.574251347313719407 ) ) ;
#29681=( GEOMETRIC_REPRESENTATION_CONTEXT ( 3 ) GLOBAL_UNCERTAINTY_ASSIGNED_CONTEXT ( ( #33040 ) ) GLOBAL_UNIT_ASSIGNED_CONTEXT ( ( #13615, #28396, #12664 ) ) REPRESENTATION_CONTEXT ( 'NONE', 'WORKASPACE' ) );
#29683=CARTESIAN_POINT ( 'NONE',  ( 5.000000000000000888, 20.41666666666666430, 2.886751345948126879 ) ) ;
#29685=CARTESIAN_POINT ( 'NONE',  ( -2.229367062499996610, -36.14583333196773651, 3.861377020970582219 ) ) ;
#29686=CARTESIAN_POINT ( 'NONE',  ( -4.999999999999999112, -75.79166666393545881, 2.886751345948131764 ) ) ;
#29689=CARTESIAN_POINT ( 'NONE',  ( -4.458734124999997661, -81.47916666530106511, 2.574251347313722516 ) ) ;
#29694=CARTESIAN_POINT ( 'NONE',  ( -5.000000000000000000, -23.00000000000000000, 0.000000000000000000 ) ) ;
#29700=CARTESIAN_POINT ( 'NONE',  ( -5.000000000000000000, 20.12500000273118772, 0.000000000000000000 ) ) ;
#29706=CARTESIAN_POINT ( 'NONE',  ( -2.500000000000000444, -41.04166666393548013, -4.330127018922193649 ) ) ;
#29709=CARTESIAN_POINT ( 'NONE',  ( -6.972266317189433020E-16, -36.12499999726880162, -5.000000000000000000 ) ) ;
#29710=CARTESIAN_POINT ( 'NONE',  ( 4.458734124999999437, -20.81249999863440081, -5.460374474430324690E-16 ) ) ;
#29711=CARTESIAN_POINT ( 'NONE',  ( 1.339745962155612702, -97.16965819600731891, -5.000000000000000000 ) ) ;
#29715=EDGE_LOOP ( 'NONE', ( #24843, #45383, #58856, #39933 ) ) ;
#29718=CYLINDRICAL_SURFACE ( 'NONE', #59465, 5.000000000000000000 ) ;
#29722=( BOUNDED_CURVE ( )  B_SPLINE_CURVE ( 2, ( #7099, #17060, #55026, #6466, #36677, #6144, #20936, #45692, #25759 ),
 .UNSPECIFIED., .F., .F. ) 
 B_SPLINE_CURVE_WITH_KNOTS ( ( 3, 2, 2, 2, 3 ),
 ( 0.05535714285714286170, 0.05595238095238095483, 0.05714285714285714107, 0.05833333333333333426, 0.05892857142857142738 ),
 .UNSPECIFIED. ) 
 CURVE ( )  GEOMETRIC_REPRESENTATION_ITEM ( )  RATIONAL_B_SPLINE_CURVE ( ( 0.9330127018922194093, 0.9330127018922197424, 1.000000000000000000, 0.8660254037844387076, 1.000000000000000000, 0.8660254037844387076, 1.000000000000000000, 0.9330127018922194093, 0.9330127018922194093 ) ) 
 REPRESENTATION_ITEM ( '' )  );
#29726=VECTOR ( 'NONE', #41110, 1000.000000000000000 ) ;
#29730=CARTESIAN_POINT ( 'NONE',  ( 9.457646018065525792E-16, 13.93750000136559564, 5.148502694627439702 ) ) ;
#29735=CARTESIAN_POINT ( 'NONE',  ( -2.916731409357579869E-14, 12.37500000273118594, 5.000000000000000888 ) ) ;
#29736=CARTESIAN_POINT ( 'NONE',  ( -6.972266317189433020E-16, -6.249999999999999112, -5.000000000000000000 ) ) ;
#29737=CARTESIAN_POINT ( 'NONE',  ( -6.972266317189433020E-16, -29.12499999726881228, -5.000000000000000000 ) ) ;
#29738=CARTESIAN_POINT ( 'NONE',  ( 4.458734125000000326, -63.89583333196772941, 2.574251347313718519 ) ) ;
#29740=CARTESIAN_POINT ( 'NONE',  ( 9.457646018065525792E-16, 15.93750000136559564, 5.148502694627439702 ) ) ;
#29741=EDGE_CURVE ( 'NONE', #46354, #4805, #13123, .T. ) ;
#29742=CARTESIAN_POINT ( 'NONE',  ( -1.339745962155599601, 17.79465819873852439, -5.000000000000007994 ) ) ;
#29743=CARTESIAN_POINT ( 'NONE',  ( 9.457646018065525792E-16, -47.31249999863440792, 5.148502694627439702 ) ) ;
#29744=CARTESIAN_POINT ( 'NONE',  ( -5.000000000000000000, -7.874999997268813168, 0.000000000000000000 ) ) ;
#29748=CARTESIAN_POINT ( 'NONE',  ( -4.458734124999999437, -106.3124999986343937, 0.000000000000000000 ) ) ;
#29749=CARTESIAN_POINT ( 'NONE',  ( -2.229367062499996610, -17.39583333196773651, 3.861377020970582219 ) ) ;
#29750=ORIENTED_EDGE ( 'NONE', *, *, #60151, .T. ) ;
#29752=CARTESIAN_POINT ( 'NONE',  ( 4.458734124999998549, -98.72916666530105090, -2.574251347313721627 ) ) ;
#29754=CARTESIAN_POINT ( 'NONE',  ( 2.229367062500001939, -95.22916666530106511, 3.861377020970579999 ) ) ;
#29755=CARTESIAN_POINT ( 'NONE',  ( -6.972266317189433020E-16, -7.124999997268814056, -5.000000000000000000 ) ) ;
#29756=CARTESIAN_POINT ( 'NONE',  ( 1.060575238724906964E-15, -56.62499999726880162, 5.773502691896257311 ) ) ;
#29757=DIRECTION ( 'NONE',  ( 0.000000000000000000, 0.000000000000000000, 1.000000000000000000 ) ) ;
#29760=CARTESIAN_POINT ( 'NONE',  ( -4.458734124999997661, -19.22916666530106866, 2.574251347313722516 ) ) ;
#29761=CARTESIAN_POINT ( 'NONE',  ( 4.458734124999999437, 5.937500001365593860, -5.460374474430324690E-16 ) ) ;
#29762=CARTESIAN_POINT ( 'NONE',  ( -4.458734124999997661, -61.47916666530106511, 2.574251347313722516 ) ) ;
#29767=CARTESIAN_POINT ( 'NONE',  ( 2.500000000000002220, -6.666666666666667851, 4.330127018922192761 ) ) ;
#29768=VERTEX_POINT ( 'NONE', #18162 ) ;
#29771=CARTESIAN_POINT ( 'NONE',  ( 1.339745962155612702, -66.29465819873851729, -5.000000000000000000 ) ) ;
#29773=CARTESIAN_POINT ( 'NONE',  ( -4.458734124999999437, -88.31249999863439371, 0.000000000000000000 ) ) ;
#29774=CARTESIAN_POINT ( 'NONE',  ( -4.458734124999999437, 19.43750000136559208, 0.000000000000000000 ) ) ;
#29779=CARTESIAN_POINT ( 'NONE',  ( -6.972266317189433020E-16, 25.74999999999999645, -5.000000000000000000 ) ) ;
#29781=CARTESIAN_POINT ( 'NONE',  ( 1.060575238724906964E-15, -73.75000000000000000, 5.773502691896257311 ) ) ;
#29783=ORIENTED_EDGE ( 'NONE', *, *, #30346, .T. ) ;
#29784=DIRECTION ( 'NONE',  ( -0.000000000000000000, 1.000000000000000000, -0.000000000000000000 ) ) ;
#29785=EDGE_LOOP ( 'NONE', ( #55540, #48394, #35044, #5114 ) ) ;
#29793=ORIENTED_EDGE ( 'NONE', *, *, #42834, .T. ) ;
#29796=CARTESIAN_POINT ( 'NONE',  ( 2.229367062499998831, -63.89583333196772941, -3.861377020970580887 ) ) ;
#29800=EDGE_LOOP ( 'NONE', ( #39308, #61511, #22171, #167 ) ) ;
#29805=( BOUNDED_CURVE ( )  B_SPLINE_CURVE ( 2, ( #38432, #51671, #46834, #7612, #42001, #61642, #37193, #37499, #38741 ),
 .UNSPECIFIED., .F., .F. ) 
 B_SPLINE_CURVE_WITH_KNOTS ( ( 3, 2, 2, 2, 3 ),
 ( 0.5696428571428571175, 0.5702380952380952106, 0.5714285714285713969, 0.5726190476190475831, 0.5732142857142856762 ),
 .UNSPECIFIED. ) 
 CURVE ( )  GEOMETRIC_REPRESENTATION_ITEM ( )  RATIONAL_B_SPLINE_CURVE ( ( 0.9330127018922194093, 0.9330127018922194093, 1.000000000000000000, 0.8660254037844387076, 1.000000000000000000, 0.8660254037844387076, 1.000000000000000000, 0.9330127018922194093, 0.9330127018922194093 ) ) 
 REPRESENTATION_ITEM ( '' )  );
#29808=CARTESIAN_POINT ( 'NONE',  ( 4.458734125000001214, -104.1458333319677365, 2.574251347313718519 ) ) ;
#29812=VECTOR ( 'NONE', #15771, 1000.000000000000000 ) ;
#29815=CARTESIAN_POINT ( 'NONE',  ( 9.457646018065525792E-16, -46.06249999863440081, 5.148502694627439702 ) ) ;
#29819=CARTESIAN_POINT ( 'NONE',  ( -2.229367062500000163, -13.47916666530107221, -3.861377020970580443 ) ) ;
#29820=CARTESIAN_POINT ( 'NONE',  ( 5.000000000000000000, -101.4166666666666572, -2.886751345948129988 ) ) ;
#29823=CARTESIAN_POINT ( 'NONE',  ( 1.975475456537005874E-15, -10.62499999726881228, 5.000000000000000000 ) ) ;
#29824=CARTESIAN_POINT ( 'NONE',  ( 2.229367062499998831, -34.89583333196772941, -3.861377020970580887 ) ) ;
#29825=CARTESIAN_POINT ( 'NONE',  ( -4.999999999999999112, 6.208333336064520758, 2.886751345948131764 ) ) ;
#29826=CYLINDRICAL_SURFACE ( 'NONE', #14956, 5.000000000000000000 ) ;
#29832=CARTESIAN_POINT ( 'NONE',  ( 4.458734124999999437, 3.937500001365595192, -5.460374474430324690E-16 ) ) ;
#29833=VERTEX_POINT ( 'NONE', #63179 ) ;
#29836=CARTESIAN_POINT ( 'NONE',  ( 5.000000000000000000, -98.50000000000000000, -6.123233995736766282E-16 ) ) ;
#29837=CARTESIAN_POINT ( 'NONE',  ( -4.458734124999999437, -31.39583333196773296, -2.574251347313719407 ) ) ;
#29839=CARTESIAN_POINT ( 'NONE',  ( -5.000000000000000000, -36.08333333333332860, -2.886751345948128211 ) ) ;
#29840=CARTESIAN_POINT ( 'NONE',  ( -2.229367062499996610, -83.39583333196773651, 3.861377020970582219 ) ) ;
#29844=CARTESIAN_POINT ( 'NONE',  ( 4.458734124999999437, -0.8124999986344055847, -5.460374474430324690E-16 ) ) ;
#29845=CARTESIAN_POINT ( 'NONE',  ( 4.458734125000001214, 23.85416666803225993, 2.574251347313718519 ) ) ;
#29847=CARTESIAN_POINT ( 'NONE',  ( -3.152548672688508926E-16, -40.81249999863440081, -5.148502694627439702 ) ) ;
#29848=CARTESIAN_POINT ( 'NONE',  ( -6.972266317189433020E-16, -105.2500000000000000, -5.000000000000000000 ) ) ;
#29851=CARTESIAN_POINT ( 'NONE',  ( -3.152548672688508926E-16, -68.56249999863439371, -5.148502694627439702 ) ) ;
#29852=CARTESIAN_POINT ( 'NONE',  ( -5.000000000000000000, -106.8749999972687874, 0.000000000000000000 ) ) ;
#29854=CARTESIAN_POINT ( 'NONE',  ( -2.499999999999996447, -64.83333333333332860, 4.330127018922195425 ) ) ;
#29857=CARTESIAN_POINT ( 'NONE',  ( -5.000000000000000000, -60.08333333333333570, -2.886751345948128211 ) ) ;
#29860=VERTEX_POINT ( 'NONE', #57728 ) ;
#29866=AXIS2_PLACEMENT_3D ( 'NONE', #3246, #51803, #62093 ) ;
#29872=CARTESIAN_POINT ( 'NONE',  ( 5.000000000000000888, -35.45833333060213732, 2.886751345948126879 ) ) ;
#29879=CARTESIAN_POINT ( 'NONE',  ( 2.229367062499998831, -41.89583333196773651, -3.861377020970580887 ) ) ;
#29889=CARTESIAN_POINT ( 'NONE',  ( 4.458734124999998549, -88.97916666530107932, -2.574251347313721627 ) ) ;
#29890=DIRECTION ( 'NONE',  ( -0.000000000000000000, 1.000000000000000000, -0.000000000000000000 ) ) ;
#29891=ORIENTED_EDGE ( 'NONE', *, *, #55046, .F. ) ;
#29892=DIRECTION ( 'NONE',  ( 0.000000000000000000, 0.000000000000000000, 1.000000000000000000 ) ) ;
#29896=VERTEX_POINT ( 'NONE', #52893 ) ;
#29897=CARTESIAN_POINT ( 'NONE',  ( -4.458734124999998549, 2.770833334698928674, 2.574251347313722516 ) ) ;
#29898=EDGE_CURVE ( 'NONE', #45305, #41928, #34203, .T. ) ;
#29900=CARTESIAN_POINT ( 'NONE',  ( 5.000000000000000000, -106.4999999999999858, -6.123233995736766282E-16 ) ) ;
#29901=CARTESIAN_POINT ( 'NONE',  ( -4.458734124999999437, -15.64583333196773474, -2.574251347313719407 ) ) ;
#29902=ADVANCED_FACE ( 'NONE', ( #39032 ), #33894, .T. ) ;
#29903=FACE_OUTER_BOUND ( 'NONE', #15095, .T. ) ;
#29905=CARTESIAN_POINT ( 'NONE',  ( -1.339745962155727277, -73.66965819600733312, 4.999999999999933387 ) ) ;
#29908=CARTESIAN_POINT ( 'NONE',  ( 2.229367062499998831, 23.10416666803225993, -3.861377020970580887 ) ) ;
#29910=CARTESIAN_POINT ( 'NONE',  ( 4.458734125000000326, -94.89583333196775072, 2.574251347313718519 ) ) ;
#29911=CARTESIAN_POINT ( 'NONE',  ( -2.500000000000000444, -34.04166666393547303, -4.330127018922193649 ) ) ;
#29912=CARTESIAN_POINT ( 'NONE',  ( 5.000000000000000888, -57.45833333060214443, 2.886751345948126879 ) ) ;
#29913=CARTESIAN_POINT ( 'NONE',  ( 4.458734124999998549, -14.72916666530107399, -2.574251347313721627 ) ) ;
#29915=DIRECTION ( 'NONE',  ( 0.000000000000000000, 0.000000000000000000, 1.000000000000000000 ) ) ;
#29919=CARTESIAN_POINT ( 'NONE',  ( 5.000000000000000888, -39.45833333060214443, 2.886751345948126879 ) ) ;
#29920=CARTESIAN_POINT ( 'NONE',  ( -1.339745962155618253, 21.33034180399265978, 4.999999999999996447 ) ) ;
#29921=CARTESIAN_POINT ( 'NONE',  ( 4.458734124999999437, 13.18750000136559208, -5.460374474430324690E-16 ) ) ;
#29923=ADVANCED_FACE ( 'NONE', ( #42916 ), #18482, .T. ) ;
#29925=CARTESIAN_POINT ( 'NONE',  ( 2.229367062499998831, -59.64583333196774362, -3.861377020970580887 ) ) ;
#29928=CARTESIAN_POINT ( 'NONE',  ( 2.499999999999998668, 5.666666666666666963, -4.330127018922193649 ) ) ;
#29932=CARTESIAN_POINT ( 'NONE',  ( 4.458734124999999437, -54.81249999863440081, -5.460374474430324690E-16 ) ) ;
#29933=CARTESIAN_POINT ( 'NONE',  ( -5.000000000000000000, -87.95833333060213022, -2.886751345948128211 ) ) ;
#29934=CARTESIAN_POINT ( 'NONE',  ( -4.458734124999997661, -32.22916666530106511, 2.574251347313722516 ) ) ;
#29935=DIRECTION ( 'NONE',  ( -0.000000000000000000, 1.000000000000000000, -0.000000000000000000 ) ) ;
#29939=CARTESIAN_POINT ( 'NONE',  ( -4.999999999999999112, -41.91666666666667140, 2.886751345948131764 ) ) ;
#29940=CARTESIAN_POINT ( 'NONE',  ( 1.339745962155612702, -98.16965819600733312, -5.000000000000000000 ) ) ;
#29943=CARTESIAN_POINT ( 'NONE',  ( -4.458734124999999437, -101.3958333319677365, -2.574251347313719407 ) ) ;
#29944=CARTESIAN_POINT ( 'NONE',  ( 4.458734124999999437, 3.937500001365595192, -5.460374474430324690E-16 ) ) ;
#29945=CARTESIAN_POINT ( 'NONE',  ( 0.000000000000000000, -120.0000000000000000, 5.000000000000000000 ) ) ;
#29955=CARTESIAN_POINT ( 'NONE',  ( -2.499999999999996447, -55.70833333060214443, 4.330127018922195425 ) ) ;
#29958=CARTESIAN_POINT ( 'NONE',  ( -3.152548672688508926E-16, -24.81249999863440436, -5.148502694627439702 ) ) ;
#29966=ORIENTED_EDGE ( 'NONE', *, *, #62981, .T. ) ;
#29967=CARTESIAN_POINT ( 'NONE',  ( 5.000000000000000000, -20.37499999726880873, -6.123233995736766282E-16 ) ) ;
#29968=ORIENTED_EDGE ( 'NONE', *, *, #59618, .F. ) ;
#29969=CARTESIAN_POINT ( 'NONE',  ( -4.458734124999999437, -72.56249999863439371, 0.000000000000000000 ) ) ;
#29970=CARTESIAN_POINT ( 'NONE',  ( 0.000000000000000000, -120.0000000000000000, 0.000000000000000000 ) ) ;
#29971=ORIENTED_EDGE ( 'NONE', *, *, #9514, .F. ) ;
#29972=VECTOR ( 'NONE', #5218, 1000.000000000000000 ) ;
#29976=CARTESIAN_POINT ( 'NONE',  ( 2.229367062499998831, -5.895833331967740953, -3.861377020970580887 ) ) ;
#29977=ORIENTED_EDGE ( 'NONE', *, *, #34178, .T. ) ;
#29978=EDGE_CURVE ( 'NONE', #31397, #14365, #10668, .T. ) ;
#29979=CARTESIAN_POINT ( 'NONE',  ( -5.000000000000000000, -20.08333333333333925, -2.886751345948128211 ) ) ;
#29986=CARTESIAN_POINT ( 'NONE',  ( -3.152548672688508926E-16, -83.56249999863440792, -5.148502694627439702 ) ) ;
#29988=CARTESIAN_POINT ( 'NONE',  ( -4.458734124999999437, 1.604166668032262155, -2.574251347313719407 ) ) ;
#29989=CARTESIAN_POINT ( 'NONE',  ( 5.000000000000000000, -85.41666666666665719, -2.886751345948129988 ) ) ;
#29991=CARTESIAN_POINT ( 'NONE',  ( -2.229367062500000163, -63.72916666530106511, -3.861377020970580443 ) ) ;
#29992=CARTESIAN_POINT ( 'NONE',  ( -2.500000000000000444, -23.04166666393548013, -4.330127018922193649 ) ) ;
#29994=CARTESIAN_POINT ( 'NONE',  ( -1.339745962155610925, -0.6696581960073348938, 5.000000000000000000 ) ) ;
#29995=CARTESIAN_POINT ( 'NONE',  ( -5.000000000000000000, -37.87499999726881583, 0.000000000000000000 ) ) ;
#29996=CARTESIAN_POINT ( 'NONE',  ( 1.975475456537005874E-15, -8.750000000000000000, 5.000000000000000000 ) ) ;
#29998=CARTESIAN_POINT ( 'NONE',  ( -4.458734124999998549, -46.22916666530106511, 2.574251347313722516 ) ) ;
#29999=CARTESIAN_POINT ( 'NONE',  ( -4.458734124999997661, -30.47916666530107221, 2.574251347313722516 ) ) ;
#30002=CARTESIAN_POINT ( 'NONE',  ( -2.499999999999996447, 22.16666666666666785, 4.330127018922195425 ) ) ;
#30003=EDGE_CURVE ( 'NONE', #14537, #14586, #25516, .T. ) ;
#30006=CARTESIAN_POINT ( 'NONE',  ( 9.457646018065525792E-16, -38.06249999863441502, 5.148502694627439702 ) ) ;
#30007=CARTESIAN_POINT ( 'NONE',  ( 2.499999999999998668, -72.20833333060214443, -4.330127018922193649 ) ) ;
#30010=CARTESIAN_POINT ( 'NONE',  ( -6.972266317189433020E-16, -61.12499999726880162, -5.000000000000000000 ) ) ;
#30012=CARTESIAN_POINT ( 'NONE',  ( 1.339745962155615144, -15.58034179853029499, 4.999999999999999112 ) ) ;
#30013=CARTESIAN_POINT ( 'NONE',  ( 4.458734124999999437, -79.06249999863440792, -5.460374474430324690E-16 ) ) ;
#30015=DIRECTION ( 'NONE',  ( -0.000000000000000000, 1.000000000000000000, -0.000000000000000000 ) ) ;
#30016=FACE_OUTER_BOUND ( 'NONE', #52919, .T. ) ;
#30017=CARTESIAN_POINT ( 'NONE',  ( -4.999999999999999112, -26.91666666666666075, 2.886751345948131764 ) ) ;
#30023=CARTESIAN_POINT ( 'NONE',  ( -3.535250795749689387E-16, 23.87500000273118417, -5.773502691896257311 ) ) ;
#30029=DIRECTION ( 'NONE',  ( -0.000000000000000000, 1.000000000000000000, -0.000000000000000000 ) ) ;
#30031=CARTESIAN_POINT ( 'NONE',  ( -1.339745962155613812, -80.08034179853028434, -5.000000000000000000 ) ) ;
#30032=CARTESIAN_POINT ( 'NONE',  ( 0.000000000000000000, -120.0000000000000000, 0.000000000000000000 ) ) ;
#30034=CARTESIAN_POINT ( 'NONE',  ( 2.229367062500001939, -22.97916666530107221, 3.861377020970579999 ) ) ;
#30039=VERTEX_POINT ( 'NONE', #54142 ) ;
#30043=DIRECTION ( 'NONE',  ( 0.000000000000000000, 0.000000000000000000, 1.000000000000000000 ) ) ;
#30044=CARTESIAN_POINT ( 'NONE',  ( -2.499999999999996447, -2.833333333333333481, 4.330127018922195425 ) ) ;
#30046=ORIENTED_EDGE ( 'NONE', *, *, #38208, .F. ) ;
#30053=CARTESIAN_POINT ( 'NONE',  ( 9.457646018065525792E-16, 15.93750000136559564, 5.148502694627439702 ) ) ;
#30054=( BOUNDED_CURVE ( )  B_SPLINE_CURVE ( 2, ( #54990, #10594, #11237, #11556, #36010, #55641, #16067, #30861, #5460 ),
 .UNSPECIFIED., .F., .F. ) 
 B_SPLINE_CURVE_WITH_KNOTS ( ( 3, 2, 2, 2, 3 ),
 ( 0.9767857142857142572, 0.9773809523809523503, 0.9785714285714285365, 0.9797619047619047228, 0.9803571428571428159 ),
 .UNSPECIFIED. ) 
 CURVE ( )  GEOMETRIC_REPRESENTATION_ITEM ( )  RATIONAL_B_SPLINE_CURVE ( ( 0.9330127018922194093, 0.9330127018922194093, 1.000000000000000000, 0.8660254037844387076, 1.000000000000000000, 0.8660254037844387076, 1.000000000000000000, 0.9330127018922194093, 0.9330127018922194093 ) ) 
 REPRESENTATION_ITEM ( '' )  );
#30061=CARTESIAN_POINT ( 'NONE',  ( -4.458734124999997661, -64.22916666530106511, 2.574251347313722516 ) ) ;
#30062=CARTESIAN_POINT ( 'NONE',  ( 2.229367062500001939, 20.02083333469892779, 3.861377020970579999 ) ) ;
#30064=CARTESIAN_POINT ( 'NONE',  ( 2.229367062500001939, -47.22916666530106511, 3.861377020970579999 ) ) ;
#30065=CARTESIAN_POINT ( 'NONE',  ( 5.000000000000000000, -10.37499999726881583, -6.123233995736766282E-16 ) ) ;
#30067=CARTESIAN_POINT ( 'NONE',  ( -2.500000000000000444, -66.04166666393547303, -4.330127018922193649 ) ) ;
#30068=CARTESIAN_POINT ( 'NONE',  ( -1.339745962155613812, -74.20534180126145429, -5.000000000000000000 ) ) ;
#30070=CARTESIAN_POINT ( 'NONE',  ( 4.458734125000000326, -18.14583333196773651, 2.574251347313718519 ) ) ;
#30072=CARTESIAN_POINT ( 'NONE',  ( -4.458734124999999437, -106.3124999986343937, 0.000000000000000000 ) ) ;
#30075=CARTESIAN_POINT ( 'NONE',  ( 4.458734125000001214, -96.14583333196772230, 2.574251347313718519 ) ) ;
#30076=CARTESIAN_POINT ( 'NONE',  ( 1.060575238724906964E-15, -58.62499999726880873, 5.773502691896257311 ) ) ;
#30077=FACE_OUTER_BOUND ( 'NONE', #3721, .T. ) ;
#30080=CARTESIAN_POINT ( 'NONE',  ( 2.229367062499998831, -18.64583333196774007, -3.861377020970580887 ) ) ;
#30081=CARTESIAN_POINT ( 'NONE',  ( -2.229367062499996610, 7.604166668032260823, 3.861377020970582219 ) ) ;
#30082=( BOUNDED_CURVE ( )  B_SPLINE_CURVE ( 2, ( #1497, #60985, #6949, #36211, #44903, #50043, #45219, #51334, #1185 ),
 .UNSPECIFIED., .F., .F. ) 
 B_SPLINE_CURVE_WITH_KNOTS ( ( 3, 2, 2, 2, 3 ),
 ( 0.8732142857142857206, 0.8738095238095238138, 0.8750000000000000000, 0.8761904761904761862, 0.8767857142857142794 ),
 .UNSPECIFIED. ) 
 CURVE ( )  GEOMETRIC_REPRESENTATION_ITEM ( )  RATIONAL_B_SPLINE_CURVE ( ( 0.9330127018922194093, 0.9330127018922194093, 1.000000000000000000, 0.8660254037844387076, 1.000000000000000000, 0.8660254037844387076, 1.000000000000000000, 0.9330127018922194093, 0.9330127018922194093 ) ) 
 REPRESENTATION_ITEM ( '' )  );
#30083=CARTESIAN_POINT ( 'NONE',  ( 9.457646018065525792E-16, -63.31249999863440792, 5.148502694627439702 ) ) ;
#30088=CARTESIAN_POINT ( 'NONE',  ( -5.000000000000000000, -11.08333333333333393, -2.886751345948128211 ) ) ;
#30095=CARTESIAN_POINT ( 'NONE',  ( -4.458734124999998549, -92.22916666530106511, 2.574251347313722516 ) ) ;
#30097=CARTESIAN_POINT ( 'NONE',  ( 1.339745962155612702, -93.29465819873853150, -5.000000000000000000 ) ) ;
#30099=CARTESIAN_POINT ( 'NONE',  ( -2.499999999999996447, 26.16666666666666430, 4.330127018922195425 ) ) ;
#30101=CARTESIAN_POINT ( 'NONE',  ( 5.000000000000000000, -76.41666666666665719, -2.886751345948129988 ) ) ;
#30107=CARTESIAN_POINT ( 'NONE',  ( -5.000000000000000000, -51.00000000000000711, 0.000000000000000000 ) ) ;
#30114=ORIENTED_EDGE ( 'NONE', *, *, #63423, .F. ) ;
#30117=CARTESIAN_POINT ( 'NONE',  ( 4.458734124999999437, -61.06249999863440081, -5.460374474430324690E-16 ) ) ;
#30127=CARTESIAN_POINT ( 'NONE',  ( -2.229367062500000163, 29.52083333469892779, -3.861377020970580443 ) ) ;
#30133=CARTESIAN_POINT ( 'NONE',  ( -4.458734124999997661, -46.22916666530106511, 2.574251347313722516 ) ) ;
#30136=CARTESIAN_POINT ( 'NONE',  ( 9.457646018065525792E-16, -47.06249999863440792, 5.148502694627439702 ) ) ;
#30137=CARTESIAN_POINT ( 'NONE',  ( 0.000000000000000000, -120.0000000000000000, 0.000000000000000000 ) ) ;
#30138=CARTESIAN_POINT ( 'NONE',  ( -2.229367062500000163, -14.47916666530107221, -3.861377020970580443 ) ) ;
#30139=CARTESIAN_POINT ( 'NONE',  ( 2.500000000000002220, -101.6666666666666572, 4.330127018922192761 ) ) ;
#30141=CARTESIAN_POINT ( 'NONE',  ( 4.458734125000001214, -35.14583333196772941, 2.574251347313718519 ) ) ;
#30142=CARTESIAN_POINT ( 'NONE',  ( -2.500000000000000444, 8.958333336064518093, -4.330127018922193649 ) ) ;
#30147=CARTESIAN_POINT ( 'NONE',  ( -6.972266317189433020E-16, 20.87500000273118062, -5.000000000000000000 ) ) ;
#30149=CARTESIAN_POINT ( 'NONE',  ( 4.458734124999999437, -2.062499998634406584, -5.460374474430324690E-16 ) ) ;
#30152=CARTESIAN_POINT ( 'NONE',  ( 1.975475456537005874E-15, -34.75000000000000000, 5.000000000000000000 ) ) ;
#30153=CARTESIAN_POINT ( 'NONE',  ( -4.458734124999998549, -89.22916666530106511, 2.574251347313722516 ) ) ;
#30154=CARTESIAN_POINT ( 'NONE',  ( 4.458734125000001214, -37.89583333196772941, 2.574251347313718519 ) ) ;
#30155=CARTESIAN_POINT ( 'NONE',  ( 1.975475456537005874E-15, -35.75000000000000711, 5.000000000000000000 ) ) ;
#30156=CARTESIAN_POINT ( 'NONE',  ( 4.458734125000001214, -81.14583333196773651, 2.574251347313718519 ) ) ;
#30160=CARTESIAN_POINT ( 'NONE',  ( -2.229367062499996610, -2.145833331967737845, 3.861377020970582219 ) ) ;
#30161=CARTESIAN_POINT ( 'NONE',  ( -3.152548672688508926E-16, 20.18750000136559208, -5.148502694627439702 ) ) ;
#30162=CARTESIAN_POINT ( 'NONE',  ( 4.458734124999999437, -46.06249999863440081, -5.460374474430324690E-16 ) ) ;
#30163=CARTESIAN_POINT ( 'NONE',  ( 2.499999999999998668, -15.33333333333333037, -4.330127018922193649 ) ) ;
#30168=CARTESIAN_POINT ( 'NONE',  ( -2.229367062500000163, -75.47916666530106511, -3.861377020970580443 ) ) ;
#30169=CARTESIAN_POINT ( 'NONE',  ( 2.499999999999998668, -105.2083333306021444, -4.330127018922193649 ) ) ;
#30172=DIRECTION ( 'NONE',  ( -0.000000000000000000, 1.000000000000000000, -0.000000000000000000 ) ) ;
#30174=CARTESIAN_POINT ( 'NONE',  ( -2.500000000000000444, -59.16666666666665719, -4.330127018922193649 ) ) ;
#30175=CARTESIAN_POINT ( 'NONE',  ( -6.972266317189433020E-16, -35.25000000000000000, -5.000000000000000000 ) ) ;
#30178=CARTESIAN_POINT ( 'NONE',  ( -5.000000000000000000, -72.87499999726880162, 0.000000000000000000 ) ) ;
#30179=CARTESIAN_POINT ( 'NONE',  ( 5.000000000000000000, -67.50000000000000000, -6.123233995736766282E-16 ) ) ;
#30188=CARTESIAN_POINT ( 'NONE',  ( -2.500000000000000444, -76.04166666393547303, -4.330127018922193649 ) ) ;
#30191=ORIENTED_EDGE ( 'NONE', *, *, #43018, .T. ) ;
#30195=CARTESIAN_POINT ( 'NONE',  ( -4.458734124999999437, -48.64583333196773651, -2.574251347313719407 ) ) ;
#30203=( BOUNDED_CURVE ( )  B_SPLINE_CURVE ( 2, ( #3636, #42541, #2378, #3014, #56725, #41906, #12645, #18100, #27431 ),
 .UNSPECIFIED., .F., .F. ) 
 B_SPLINE_CURVE_WITH_KNOTS ( ( 3, 2, 2, 2, 3 ),
 ( 0.9946428571428571619, 0.9952380952380952550, 0.9964285714285714413, 0.9976190476190476275, 0.9982142857142857206 ),
 .UNSPECIFIED. ) 
 CURVE ( )  GEOMETRIC_REPRESENTATION_ITEM ( )  RATIONAL_B_SPLINE_CURVE ( ( 0.9330127018922194093, 0.9330127018922194093, 1.000000000000000000, 0.8660254037844387076, 1.000000000000000000, 0.8660254037844387076, 1.000000000000000000, 0.9330127018922194093, 0.9330127018922194093 ) ) 
 REPRESENTATION_ITEM ( '' )  );
#30204=EDGE_CURVE ( 'NONE', #1698, #2721, #18428, .T. ) ;
#30207=EDGE_CURVE ( 'NONE', #54038, #23647, #17253, .T. ) ;
#30208=CARTESIAN_POINT ( 'NONE',  ( 2.229367062499998831, -91.89583333196773651, -3.861377020970580887 ) ) ;
#30210=EDGE_LOOP ( 'NONE', ( #60768, #39004, #13843, #38492 ) ) ;
#30211=CARTESIAN_POINT ( 'NONE',  ( -6.972266317189433020E-16, -98.12499999726880162, -5.000000000000000000 ) ) ;
#30214=CARTESIAN_POINT ( 'NONE',  ( 1.339745962155615144, -38.70534180126146850, 4.999999999999999112 ) ) ;
#30215=ORIENTED_EDGE ( 'NONE', *, *, #14895, .T. ) ;
#30217=CARTESIAN_POINT ( 'NONE',  ( 2.229367062500001939, 2.020833334698927786, 3.861377020970579999 ) ) ;
#30218=LINE ( 'NONE', #6749, #12369 ) ;
#30219=CARTESIAN_POINT ( 'NONE',  ( 4.458734124999999437, -15.06249999863440436, -5.460374474430324690E-16 ) ) ;
#30222=DIRECTION ( 'NONE',  ( -0.000000000000000000, 1.000000000000000000, -0.000000000000000000 ) ) ;
#30224=CARTESIAN_POINT ( 'NONE',  ( -2.229367062499996610, 14.60416666803226171, 3.861377020970582219 ) ) ;
#30227=CARTESIAN_POINT ( 'NONE',  ( -2.500000000000000444, -21.16666666666666785, -4.330127018922193649 ) ) ;
#30228=CARTESIAN_POINT ( 'NONE',  ( -4.458734124999999437, -17.39583333196773651, -2.574251347313719407 ) ) ;
#30229=CYLINDRICAL_SURFACE ( 'NONE', #29313, 5.000000000000000000 ) ;
#30233=CARTESIAN_POINT ( 'NONE',  ( 5.000000000000000888, -43.45833333060214443, 2.886751345948126879 ) ) ;
#30235=CARTESIAN_POINT ( 'NONE',  ( 4.458734124999998549, 15.27083333469893134, -2.574251347313721627 ) ) ;
#30239=CARTESIAN_POINT ( 'NONE',  ( -4.458734124999998549, -63.22916666530106511, 2.574251347313722516 ) ) ;
#30242=CARTESIAN_POINT ( 'NONE',  ( 5.000000000000000000, 5.583333333333332149, -2.886751345948129988 ) ) ;
#30245=CARTESIAN_POINT ( 'NONE',  ( -2.229367062500000163, -57.47916666530107932, -3.861377020970580443 ) ) ;
#30246=CARTESIAN_POINT ( 'NONE',  ( -4.999999999999999112, -86.79166666393548724, 2.886751345948131764 ) ) ;
#30247=CARTESIAN_POINT ( 'NONE',  ( 4.458734125000000326, -32.89583333196774362, 2.574251347313718519 ) ) ;
#30248=AXIS2_PLACEMENT_3D ( 'NONE', #23585, #62195, #63451 ) ;
#30249=DIRECTION ( 'NONE',  ( 0.000000000000000000, 0.000000000000000000, 1.000000000000000000 ) ) ;
#30251=CARTESIAN_POINT ( 'NONE',  ( 1.975475456537005874E-15, -16.62499999726881583, 5.000000000000000000 ) ) ;
#30252=CARTESIAN_POINT ( 'NONE',  ( 1.975475456537005874E-15, -16.62499999726881583, 5.000000000000000000 ) ) ;
#30254=CARTESIAN_POINT ( 'NONE',  ( -3.535250795749689387E-16, -44.25000000000000000, -5.773502691896257311 ) ) ;
#30256=CARTESIAN_POINT ( 'NONE',  ( -1.339745962155613812, -108.2053418012614543, -5.000000000000000000 ) ) ;
#30258=CARTESIAN_POINT ( 'NONE',  ( 4.458734124999999437, -103.8124999986344079, -5.460374474430324690E-16 ) ) ;
#30259=CARTESIAN_POINT ( 'NONE',  ( 4.458734124999999437, 4.937500001365595637, -5.460374474430324690E-16 ) ) ;
#30260=( BOUNDED_SURFACE ( )  B_SPLINE_SURFACE ( 1, 2, ( 
 ( #23776, #9912, #4159, #24088, #43683, #58176, #8975, #63329, #28271, #24399, #44000, #37936, #43378, #62390, #19246, #47578, #33731, #3530, #47886, #19567, #38862, #3844, #14422, #23464, #28585, #53349, #39179, #9599, #48206, #63023, #13798, #18311, #43067, #57569, #52726, #13494, #38253, #18930, #62705, #23139, #33110, #18631, #57874, #29207, #9284, #38546, #33418, #28900, #53037, #48520, #4461, #58498, #34044, #53666, #48832, #4772, #63648, #58804, #25990, #1564, #16344, #45609, #55592, #30488, #49478, #5098, #40773, #29845, #21166, #50110, #35966, #29520, #20540, #6065, #39497, #39815, #59456, #25033, #60419, #40137, #25679, #603, #45287, #49154, #10871, #5416, #59781, #44643, #34681, #15705, #24717, #1253, #15388, #285, #35323, #30813, #20856, #35013, #10551, #44321, #60098, #19884, #59133, #15069, #20213, #54300, #55272, #11191, #16019, #54626, #25354, #30161, #54944, #50445, #40458, #10242, #49790, #35646, #5736, #44972, #6385, #937, #21809, #22444, #50750, #1887, #7016, #56543, #46881, #32073, #41716, #17614, #21490, #2825, #12143, #61367, #42041, #26300, #52022, #17288, #51077, #2506, #31435, #3141, #26624, #37230, #36912, #41088, #45924, #60735, #46244, #27564, #31763, #61682, #11511, #31127, #56856, #12774, #56223, #11816, #2205, #6695, #12462, #41404, #51710, #7651, #51396, #7338, #22760, #16656, #32396, #61056, #16976, #7966, #36281, #55905, #36587, #27254, #47197, #42357, #61996, #17916, #26949, #37538, #46566, #22124, #24002, #8276, #33968, #43300, #33032, #48129, #13411, #48748, #52648, #19162, #18850, #23066, #27880, #47501, #8582, #9518, #57797, #48443, #57177, #13095, #38780, #58419, #38175, #57492, #28193, #32714, #38471, #23389, #58097, #14027, #33342, #52958, #4690, #3452, #14346, #42989, #3765, #13718, #42671, #8896, #62310, #37859, #62936, #9209, #28822, #52342, #4080, #18234, #29125, #33656, #53588, #24312, #43919, #63566, #19486, #53274, #47808, #62631, #18553, #28511, #23703, #4383, #43604, #63248, #59369, #5657, #29435, #34586, #54218, #39412, #45207, #15303, #25270, #14978, #44890, #1173, #30081, #19803, #34925, #59050, #5015, #54546, #5988, #49712, #10156, #53899, #10469, #10795, #851, #49395, #5339, #40378, #40053, #60019, #20773, #50031, #29761, #25593, #35245, #54864, #59697, #24957, #520, #44562, #20455, #30407, #15628, #39099, #20130, #58728, #49068, #14654, #34273, #39730, #9824, #24634, #44241, #205, #63460, #57692, #57997, #43500, #4908, #58627, #13924, #33549, #62830, #47706, #33237, #3661, #38063, #62523, #23593, #48334, #52856, #19697, #99, #13619, #39307, #14547, #38674, #34166, #53789, #29019, #18746, #29326, #18442, #33860, #52548, #19378, #8789, #58934, #38993, #24528, #23274, #43190, #32925, #43814, #28402, #48643, #48022, #8480, #9721, #38371, #28089, #63144, #28711, #53480, #48956, #3973, #44131, #9409, #4584, #53168, #42878, #4280, #9103, #24208, #23897, #19056, #58313, #14235, #35451, #40276, #25477, #54105, #49914, #35775, #30296, #15835, #29658, #54757, #10045, #45098, #34473, #59914, #40902, #5868, #14862, #55076, #55397, #49289, #10683, #5227, #1693, #50242, #1063, #20670, #21296, #25805, #6191, #10997, #34816, #45740, #20342, #24847, #16149, #15192, #45417, #44453, #30620, #1384, #20984, #40585, #60229, #413, #35142, #11314, #30939, #50565, #39942, #6508, #59260, #26120, #20015, #39622, #54439, #10367, #29976, #49604, #5545, #25157, #44771, #732, #59589, #15523, #47326, #60546, #51526, #17430, #6827, #7144, #26759, #56032, #52152, #7463, #56673, #31576, #12591, #8095, #41851, #36402, #27071, #11949, #2016, #46688, #56985, #37045, #46376, #31250, #2634, #61811, #61500, #2324, #41530, #3277, #27378, #22888, #27698, #12900, #51210, #16468, #22577, #42174, #47011, #21931, #56359, #61180, #22254, #17737, #32204, #36089, #17103, #51833, #50884, #55717, #7775, #36727, #12279, #2960, #11630, #26433, #31894, #37355, #32524, #46054, #21619, #41213, #60859, #16785, #16208, #60921, #12340, #55771, #25537, #6248, #61237, #41271, #25858, #56088, #50300, #50622, #36150, #17160, #51272, #6561, #26176, #55458, #40328, #45474, #59971, #30683, #55131, #35836, #40961, #1438, #31950, #56416, #21040, #51582, #7205, #31307, #26815, #46436, #21682, #11374, #21992, #11058, #26497, #45154, #12008, #40647, #1120, #31635, #36782, #15892, #30996, #20724, #36461, #60286, #16840, #45795, #35511, #2382, #1755, #21356, #11688, #60609, #46113, #41585, #16526, #50943, #6884, #2075, #33220, #3641, #37415, #3954, #37110, #8464, #27130, #57675, #56729, #13905, #13601, #62811, #41911, #17791, #33533, #18422, #12649, #23252, #32264, #46746, #28382, #61875, #2691, #18104, #3333, #28072, #48001, #51893, #38043, #47689, #42860, #7834, #52838, #22949, #27435, #62504, #22311, #61556, #57360, #8772, #23576, #32907, #37727, #17489, #42545, #43171, #62184, #18729, #47068, #47382, #3018, #13281, #22633, #52530, #7520, #38354, #42232, #57980, #57049, #12960, #32585, #52207, #8155, #27754, #48939, #4887, #59571, #394, #44433, #19676, #9390, #20322, #58608, #4262, #54420, #53460, #19996, #39923, #49273, #44112, #75, #39604, #29308, #15504, #9702, #29638, #5208, #39288, #14528, #24827, #33841, #29958, #58915, #43795, #63128, #63442, #59240, #53148, #14844, #9083, #29000, #25140, #15173, #48625, #34797, #14213, #34148, #34456, #44751, #10349, #53770, #24509, #19359, #23880, #4564, #43483, #58295, #19039, #38971, #54087, #24188, #28693, #48312, #10026, #49583, #5525, #712, #38656, #11615, #59897, #46035, #50548, #15817, #6809, #10661, #25459, #21277, #31235, #55701, #60528, #45723, #30277, #6492, #56017, #26103, #36072, #49897, #11296, #5851, #1675, #54740, #16453, #61165, #40884, #35125, #50867, #11930, #45080, #30921, #1047, #21915, #26418, #1998, #21603, #41512, #41197, #60842, #16768, #55057, #2312, #40569, #20653, #36386, #35432, #31561, #40257, #51194, #7126, #26742, #46358, #10981, #30601, #55380, #50222, #6172, #25789, #60210, #45400, #1367, #20969, #16134, #35756, #27055, #7758, #52458, #3878, #47308, #17088, #61481, #52765, #32829, #17414, #47614, #41836, #42158, #27680, #8694, #42785, #61794, #17721, #46995, #31876, #37029, #51510, #22236, #46673, #27361, #32505, #56655, #23497, #47920, #12572, #43099, #62430, #22873, #18348, #37971, #13207, #2943, #13531, #2618, #18026, #36709, #3567, #32185, #56342, #23174, #28306, #7447, #22557, #12262, #27994, #51816, #8393, #37335, #56968, #57604, #12887, #52137, #3261, #8079, #37648, #42466, #33151, #62107, #57291, #62740, #18662, #44354, #317, #43721, #63054, #38580, #38284, #24433, #28931, #2039, #19602, #38896, #58531, #54343, #13833, #19915, #48554, #9317, #63366, #48236, #19281, #4194, #43409, #4810, #14768, #34386, #57910, #9632, #53069, #15099, #44035, #59167, #34716, #49509, #10275, #25066, #39214, #18965, #33452, #29879, #58211, #5448, #58839, #9009, #28621, #53700, #54014, #23807, #4493, #24121, #14138, #33765, #29240, #9944, #53384, #29560, #14455, #49193, #34077, #48865, #5131, #24749, #39529, #41123, #1603, #54978, #15427, #55311, #45957, #45645, #50145, #25714, #51113, #11545, #7050, #11854, #60771, #20575, #36315, #6730, #26340, #31162, #15740, #40493, #6100, #35683, #1922, #11226, #44676, #30522, #40807, #35048, #55939, #16380, #59818, #10907, #55630, #20246, #54660, #40182, #26030, #36000, #21201, #30850, #50792, #35357, #21527, #10583, #45325, #16696, #59491, #31472, #50480, #1293, #6420, #973, #636, #20890, #39848, #60455, #30195, #49824, #5768, #25386, #45007, #60134, #16055, #61404, #22483, #51746, #17649, #47538, #37264, #52685, #12498, #22798, #17011, #37897, #62031, #41754, #36950, #37573, #2240, #36627, #22160, #8000, #17949, #47236, #56892, #32751, #17328, #3488, #56259, #2544, #57213, #41440, #23102, #12812, #56577, #32433, #46600, #18270, #32110, #52379, #52062, #12184, #61089, #31798, #7688, #42705, #27294, #13132, #26663, #46282, #8317, #27916, #46919, #26981, #2861, #21844, #27603, #42078, #3179, #42391, #61720, #62349, #57526, #51431, #13448, #33072, #7373, #53310, #57836, #9244, #13755, #52991, #14380, #24355, #43955, #28228, #19202, #62667, #24671, #34004, #5053, #44279, #59089, #241, #34630, #9558, #28545, #47844, #19839, #8932, #39453, #29163, #15015, #8620, #63285, #48788, #18587, #18891, #38505, #4118, #3802, #38815, #4730, #43333, #63603, #23424, #53627, #48165, #58457, #23738, #33377, #19523, #43027, #39137, #58133, #38211, #58764, #9865, #14693, #14064, #28858, #62975, #34312, #33689, #48480, #4417, #24042, #43644, #53935, #29475, #49107, #54255, #46125, #12019, #558, #883, #20491, #49747, #46758, #2089, #51284, #25307, #7217, #2703, #36473, #30117, #21693, #5691, #59409, #41283, #51596, #31649, #40090, #24991, #60933, #56428, #56099, #59732, #35276, #61566, #22003, #17500, #22322, #7531, #44928, #41924, #17170, #36796, #41597, #15658, #50954, #54898, #16852, #12350, #26830, #10196, #11699, #46447, #44598, #29796, #2393, #31319, #6895, #61248, #49429, #20166, #26509, #31962, #27143, #5373, #39763, #15341, #34964, #54580, #10502, #12972, #3966, #51906, #13917, #23267, #32595, #28083, #57061, #28705, #52221, #62824, #62518, #3029, #7845, #27447, #8166, #53160, #37740, #28394, #37122, #56741, #18741, #38365, #18116, #37428, #27766, #12662, #18434, #3344, #38055, #57687, #13293, #32918, #48325, #47081, #57991, #22960, #47393, #57372, #22645, #52541, #42245, #17803, #42871, #52849, #8783, #32277, #47700, #61886, #9098, #13613, #33544, #4274, #23892, #43494, #63139, #33231, #42557, #62198, #8475, #48013, #23587, #43182, #3654, #58305, #54098, #39936, #34467, #20008, #33854, #58927, #14227, #29651, #38667, #405, #45092, #10037, #19052, #39616, #59582, #53471, #14855, #9402, #5862, #54432, #49282, #5220, #25469, #29969, #10360, #24840, #38983, #49908, #24522, #29011, #20334, #19371, #49596, #48637, #15184, #44446, #59253, #5538, #34809, #4576, #39299, #25151, #44763, #724, #44123, #15516, #63453, #35136, #54751, #9715, #24201, #29319, #10674, #43807, #30289, #58621, #14540, #34160, #53781, #48950, #4899, #89, #19690, #11624, #36721, #26752, #26115, #1687, #30932, #15828, #1378, #35443, #6185, #30612, #55391, #16462, #20978, #51520, #31887, #45410, #7457, #46369, #6821, #2319, #21924, #60852, #50558, #61174, #50235, #2010, #20663, #51203, #25799, #27065, #7137, #56352, #55069, #11307, #1057, #11943, #40579, #16778, #60222, #40268, #41522, #6502, #59908, #31244, #60540, #21613, #17097, #16144, #31570, #41206, #36395, #35767, #12273, #36081, #45734, #56026, #10991, #21288, #50878, #40894, #46045, #55711, #26427, #13216, #52775, #17730, #23506, #37038, #22570, #13540, #61493, #43109, #32839, #42167, #37659, #2952, #38294, #61803, #8703, #8404, #12583, #17424, #56666, #37347, #62750, #47320, #37982, #46681, #2628, #28318, #47935, #27692, #47004, #56978, #22248, #28003, #12894, #47622, #3578, #22882, #42479, #57922, #32197, #3888, #32515, #52146, #3270, #51826, #62118, #7767, #27371, #52467, #62438, #18356, #41845, #57300, #8088, #18671, #23185, #13841, #33461, #53084, #9020, #18036, #42798, #57613, #33161, #39857, #28939, #646, #49202, #15439, #28630, #19612, #5142, #38589, #38909, #58543, #24130, #20259, #39224, #24761, #63376, #44365, #59500, #9956, #4504, #58848, #43733, #33777, #14778, #25075, #326, #14464, #63063, #34395, #29889, #29571, #34086, #9642, #35057, #59176, #54669, #48247, #44685, #19291, #4203, #54354, #10284, #15110, #53709, #24441, #29250, #54022, #49519, #19925, #23816, #48874, #39538, #18975, #43420, #34726, #4822, #44044, #5459, #58222, #14151, #11, #53395, #9326, #48564, #30208, #60782, #59828, #17023, #16708, #2250, #45016, #20900, #36638, #21538, #40192, #6741, #15750, #49833, #31481, #1304, #5776, #21212, #6428, #11555, #51125, #54989, #41134, #31173, #50805, #35366, #36323, #26040, #10916, #45971, #25398, #982, #60465, #26349, #1936, #36009, #40819, #20585, #45655, #7061, #1612, #55950, #30533, #50489, #50155, #16390, #6109, #55640, #10593, #11865, #25724, #26674, #46293, #45334, #21854, #40503, #61099, #41449, #60144, #16066, #35694, #55321, #11236, #30860, #12509, #23436, #61730, #7383, #57537, #56589, #47548, #43037, #52392, #47246, #3192, #42716, #32442, #18599, #12821, #32762, #8327, #22808, #17659, #27927, #36959, #33081, #42401, #46928, #2555, #2877, #3498, #62677, #62043, #56270, #32120, #28241, #23112, #51756, #62359, #17339, #37275, #17959, #47855, #18282, #56903, #52071, #22492, #26990, #7700, #46609, #61416, #22169, #42088, #8012, #27303, #12194, #31809, #27615, #51444, #37907, #37582, #13462, #52694, #8629, #3812, #41766, #57223, #13143, #53946, #18901, #15026, #29174, #28869, #48176, #48491, #9876, #24999, #4739, #38225, #38516, #10206, #29483, #58143, #5061, #62989, #63293, #48799, #29808, #251, #19211, #38828, #4428, #53002, #14073, #8941, #43345, #4128, #24054, #53635, #33701, #44608, #5383, #53321, #568, #19849, #43966, #39463, #59099, #34321, #43652, #34642, #23751, #39146, #57847, #24681, #9254, #13765, #44289, #49441, #28555, #58465, #33387, #49119, #14389, #54266, #34012, #9567, #24364, #63612, #19532, #58773, #14702, #21131, #60701, #895, #31093, #40736, #60383, #44937, #50714, #35608, #20502, #55558, #59422, #10513, #6349, #16309, #35930, #45570, #30778, #15351, #55234, #41055, #11156, #11472, #34975, #60059, #54591, #50399, #39775, #1527, #46209, #25954, #20177, #6658 ),
 ( #20819, #26265, #30127, #49756, #1849, #21455, #1219, #40100, #6981, #51038, #59744, #26592, #45887, #16621, #36242, #55870, #11782, #50076, #31400, #5702, #25317, #15669, #35288, #54908, #10836, #30451, #6034, #25637, #45253, #40419, #15983, #31732, #61964, #51362, #41369, #23037, #56508, #21777, #12743, #61648, #3109, #42639, #46532, #13060, #22726, #42324, #26915, #32679, #17582, #2473, #37506, #61015, #56185, #51987, #17885, #57145, #27533, #32363, #16941, #37199, #62282, #56825, #52311, #36554, #42008, #12105, #7930, #7303, #47165, #28163, #8246, #2171, #27846, #18203, #22086, #47467, #41685, #52615, #3421, #37824, #57457, #8550, #13378, #32999, #61332, #17256, #36878, #7618, #12430, #32041, #51678, #27223, #46843, #2790, #22409, #13997, #58065, #28791, #49036, #4351, #24282, #43884, #58387, #9179, #63532, #28479, #24603, #38748, #13688, #23356, #4980, #38438, #3735, #14313, #43572, #48719, #44209, #48094, #58697, #4659, #19455, #8864, #14625, #63216, #4049, #39068, #42955, #38141, #33935, #34238, #53867, #9481, #53557, #62598, #19131, #174, #29092, #9794, #18520, #23970, #57766, #29402, #33307, #19774, #10123, #39382, #47778, #59013, #14944, #52927, #34553, #23667, #54185, #43264, #62904, #18818, #33625, #53243, #48407, #59989, #49682, #60630, #35215, #44532, #31016, #30053, #21059, #16549, #25879, #20743, #59666, #40022, #10764, #50644, #49999, #6273, #45495, #40347, #54835, #1459, #10440, #6582, #15912, #20422, #39699, #15597, #40665, #36174, #35532, #29730, #5628, #1779, #60308, #25239, #16237, #54517, #30376, #55160, #21378, #55482, #5950, #25559, #45177, #489, #44854, #20092, #1143, #40986, #5306, #817, #11080, #55795, #49362, #30702, #24924, #11398, #50327, #26197, #45817, #35856, #59339, #15271, #34895, #12675, #31330, #61896, #60945, #18125, #17813, #3352, #46135, #22014, #37752, #22657, #41296, #7856, #42568, #17182, #26519, #12982, #12033, #3038, #62208, #27462, #2716, #41608, #61258, #56438, #32607, #31973, #51915, #47091, #22338, #36808, #42255, #56110, #52233, #41936, #2402, #21704, #12360, #37439, #11712, #61577, #50965, #31659, #47401, #57070, #51295, #8175, #36484, #51609, #17512, #22969, #27777, #7541, #27154, #46770, #2103, #7230, #16866, #37132, #6908, #26845, #46458, #56751, #32289, #25406, #38068, #45024, #20266, #335, #39865, #59512, #54365, #24449, #54677, #23278, #59186, #13305, #44693, #42881, #992, #657, #49842, #28092, #4830, #20595, #5469, #62526, #10292, #18445, #32928, #15447, #48884, #52551, #5148, #54030, #15118, #35065, #57695, #25084, #34736, #29897, #13622, #10601, #9967, #33240, #49527, #8483, #47710, #44374, #30217, #5786, #19935, #24769, #3664, #29579, #57384, #49212, #52860, #8793, #34401, #28404, #39547, #44053, #19, #19621, #39232, #58857, #14788, #61106, #2561, #36017, #30541, #26996, #11872, #55649, #11563, #46615, #51134, #31489, #6748, #60154, #40200, #7389, #36644, #16076, #31819, #2257, #21861, #7069, #11245, #31182, #1620, #50811, #17030, #26358, #59836, #26048, #36331, #50163, #51451, #55959, #26684, #1945, #6439, #15758, #6118, #35701, #21546, #46300, #60789, #45979, #41456, #30868, #56276, #25732, #55328, #12200, #54998, #35375, #41141, #50497, #16714, #45663, #10924, #21222, #45345, #1312, #20908, #40511, #40829, #60473, #16399, #22816, #13471, #22175, #41776, #61737, #57230, #51762, #17964, #17666, #61422, #47556, #52080, #23118, #42722, #62049, #37588, #13773, #36968, #3821, #8017, #32448, #3198, #7706, #42406, #27310, #2885, #27933, #37912, #57543, #17346, #32768, #12515, #38233, #3504, #18605, #57853, #8950, #33395, #48183, #62366, #42094, #56597, #53009, #22498, #28562, #18290, #32126, #46935, #13148, #33087, #37281, #27623, #47253, #56909, #12828, #52402, #52701, #8334, #8636, #28247, #47861, #23442, #43044, #62684, #9262, #58781, #579, #24691, #14399, #38523, #14711, #5393, #5071, #9575, #48809, #10524, #34655, #25010, #24373, #44297, #261, #34329, #29182, #19858, #48498, #44619, #53955, #58473, #14080, #34021, #39472, #54602, #9887, #4136, #4435, #39789, #59109, #24064, #54276, #28876, #4747, #29495, #59435, #29819, #43976, #63621, #53642, #18908, #43660, #58151, #19543, #15363, #43352, #38836, #63301, #30138, #34987, #19222, #23757, #49451, #49128, #20188, #63000, #15038, #39156, #33708, #53328, #10215, #49767, #1540, #40114, #5713, #21144, #11488, #20515, #6044, #25327, #40749, #15681, #25967, #35299, #908, #35943, #25651, #44949, #6362, #11168, #60398, #59755, #1232, #31106, #16322, #55572, #20831, #54920, #45583, #40433, #10846, #50090, #45265, #30462, #60072, #15997, #35621, #55249, #50418, #30791, #792, #58993, #44507, #58366, #19751, #19108, #54160, #63198, #24905, #5928, #14922, #43552, #471, #20400, #38726, #39362, #33912, #30352, #15249, #34528, #10102, #49977, #54496, #34875, #29710, #63512, #10744, #49013, #14293, #44830, #43864, #10422, #53537, #39678, #49341, #9774, #53845, #24584, #5287, #19436, #35198, #39048, #5602, #20072, #9463, #29073, #48697, #58677, #59646, #44190, #30034, #4637, #24261, #14604, #59313, #34219, #49663, #29380, #4962, #25219, #155, #39999, #15579, #54813, #36833, #2126, #22039, #51318, #6298, #41322, #60013, #26869, #25903, #46795, #46481, #31999, #11104, #50667, #2741, #7256, #45521, #36506, #1481, #15936, #61284, #31042, #35559, #50993, #36197, #60970, #17206, #21084, #2427, #16890, #56137, #40689, #41630, #55818, #60334, #12058, #55183, #30728, #26544, #31683, #56463, #21727, #6932, #50351, #11734, #12385, #31351, #51632, #16262, #16576, #35880, #46164, #55509, #7566, #40372, #27178, #11424, #6608, #26221, #45841, #1803, #21407, #41010, #60652, #18151, #37779, #28737, #33266, #13646, #52576, #42281, #53197, #27802, #37156, #23622, #22681, #52885, #9131, #18474, #13331, #52261, #32632, #3378, #43219, #42596, #62553, #38094, #32952, #47427, #57720, #3064, #62859, #8508, #13012, #32312, #8199, #8819, #48363, #28118, #22361, #61920, #58022, #4001, #18772, #47735, #38399, #28435, #51941, #23305, #41961, #48048, #7883, #61602, #13950, #33576, #56780, #22995, #17537, #12699, #27486, #47115, #17840, #37463, #57093, #62233, #57411, #3691, #42905, #5258, #44802, #48671, #15219, #24879, #44480, #29046, #34848, #19724, #4611, #39650, #43527, #58339, #54134, #439, #20045, #29685, #14893, #63172, #39333, #25187, #58966, #59288, #19082, #44161, #38702, #34500, #23926, #49315, #30324, #10073, #4307, #54469, #765, #14268, #130, #33887, #54787, #10396, #30006, #49636, #10717, #5573, #20373, #39974, #24235, #35171, #9748, #53507, #59619, #43840, #15550, #9437, #63486, #19410, #34195, #14572, #48988, #39024, #24557, #58652, #53818, #29353, #4935, #2044, #30651, #26786, #40929, #40618, #59942, #60261, #21649, #36756, #16498, #49946, #50273, #21961, #41242, #6219, #16812, #11027, #11346, #60576, #41557, #11978, #30969, #50594, #16180, #1091, #25831, #20700, #45767, #61208, #25507, #21011, #45447, #56386, #17132, #1411, #12313, #31607, #55742, #40304, #15865, #35805, #2354, #6534, #60888, #5901, #45127, #55430, #21329, #35486, #1723, #26148, #55103, #11658, #36119, #50912, #6854, #31278, #26469, #46084, #36432, #56062, #51242, #7178, #46404, #17460, #32554, #37082, #12620, #37694, #47662, #3614, #51553, #42517, #22282, #47970, #57336, #28352, #3925, #18703, #23544, #57957, #32876, #51864, #7488, #43144, #32232, #62784, #52504, #38328, #31925, #22925, #8438, #41882, #42203, #61847, #27408, #27102, #62154, #28042, #2989, #23221, #46717, #13252, #7807, #18073, #47040, #56702, #42832, #2662, #62476, #17766, #61528, #18396, #33194, #38017, #37383, #12932, #22607, #57648, #57016, #52179, #8124, #27727, #47354, #13576, #52809, #8747, #3303, #9676, #38945, #4859, #34767, #24480, #39895, #63414, #9997, #4238, #25111, #29610, #49240, #39260, #43768, #53121, #23853, #9364, #58886, #5184, #34431, #44086, #19967, #48599, #54393, #43456, #53432, #44405, #28665, #10320, #51, #28977, #19649, #33813, #5498, #4539, #39577, #14817, #63101, #48283, #15146, #14187, #24800, #685, #364, #54059, #19332, #24165, #58582, #29932, #34121, #59215, #49556, #44723, #14500, #20294, #58266, #13878, #33506, #53744, #19013, #29284, #9055, #38626, #48914, #59541, #40230, #31525, #11591, #59865, #26391, #20624, #20937, #6467, #51167, #21573, #40541, #60182, #25761, #10632, #15789, #30245, #55357, #7100, #35092, #30569, #35405, #46330, #26715, #55027, #2288, #41172, #1650, #60818, #55990, #21249, #16743, #6780, #25434, #60499, #15476, #46009, #45052, #21891, #1974, #54713, #49868, #6145, #5816, #36360, #1019, #55676, #10950, #50193, #11905, #45373, #1338, #26075, #11271, #16427, #16104, #35728, #30897, #36047, #31211, #50525, #45693, #40856, #50840, #13181, #17061, #31850, #27655, #37621, #62082, #3231, #52109, #36678, #12861, #62399, #56940, #42439, #56309, #17697, #12236, #8051, #61139, #22849, #3849, #32480, #41487, #17995, #18320, #51483, #37311, #7420, #28279, #32803, #47282, #57262, #47893, #52432, #8365, #27965, #61455, #8667, #46970, #57578, #42127, #47588, #27029, #46647, #17385, #3539, #2592, #23148, #37004, #22212, #42756, #7735, #37945, #13504, #33120, #52736, #41809, #56631, #12545, #32157, #51793, #22531, #27339, #61770, #2918, #4167, #29213, #39186, #58812, #43074, #34051, #13805, #39504, #48838, #19889, #59139, #10248, #15073, #49484, #24405, #43384, #62711, #34686, #23782, #54308, #44008, #29851, #23470, #14427, #63654, #33425, #33738, #53355, #18936, #18637, #53672, #19573, #58184, #14742, #38259, #4778, #63029, #9605, #38552, #28592, #34358, #57880, #53988, #9290, #53044, #9916, #24723, #29526, #28908, #4468, #8981, #49161, #48212, #14112, #48528, #24095, #43690, #5105, #44327, #291, #63337, #19253, #38868, #58504, #26310, #60107, #31444, #54951, #1574, #59463, #16668, #21174, #40782, #30824, #35331, #44649, #15395, #946, #50454, #60428, #26000, #35655, #11520, #40145, #45932, #35020, #44980, #35975, #20220, #1895, #55282, #20548, #16028, #25361, #60744, #59790, #31135, #6394, #54633, #39821, #10557, #15713, #25038, #55603, #30168, #11825, #50760, #36290, #49798, #10880, #5422, #16354, #5742, #6704, #30497, #611, #21501, #50118, #6074, #11201, #1261, #45618, #41097, #25687, #55913, #45296, #20864, #40467, #62006, #2835, #12153, #22771, #26634, #41415, #37241, #47208, #7976, #12784, #61693, #46254, #22453, #8287, #42051, #52034, #2214, #27267, #21817, #17624, #7025, #32406, #13421, #56866, #51087, #27574, #27892, #61065, #46892, #16985, #37872, #42367, #3152, #17925, #57505, #37547, #57187, #13108, #7346, #18246, #56552, #36597, #52352, #51404, #32725, #56232, #47513, #3464, #17297, #61376, #32083, #23077, #7661, #42681, #62322, #31772, #12473, #26957, #46575, #2517, #22132, #41727, #36923, #51720, #4702, #19815, #63259, #33044, #13731, #5027, #48760, #33353, #63578, #57808, #58109, #43616, #24646, #58740, #14037, #33665, #62947, #47819, #52969, #3776, #28833, #44253, #8594, #4092, #8907, #39423, #217, #28523, #59065, #14667, #38791, #34287, #29446, #58429, #53910, #43930, #62645, #33979, #9836, #48456, #53600, #23400, #9220, #28205, #19176, #52660, #14357, #43000, #4394, #18564, #9532, #49080, #38187, #24013, #48140, #23715, #24326, #29137, #19497, #43312, #39112, #18861, #38481, #53284, #46729, #21342, #29773, #17146, #15316, #7191, #2674, #11994, #6868, #45780, #26161, #60592, #36770, #36133, #56074, #31621, #26483, #40942, #51256, #59382, #56400, #46097, #5671, #24969, #1739, #26799, #22296, #2057, #14990, #34938, #51565, #46419, #54559, #2368, #39741, #16512, #21665, #7504, #41570, #55755, #11672, #31291, #49407, #10482, #5351, #50927, #27116, #54230, #49725, #30095, #41895, #34600, #41256, #10169, #61222, #60903, #12326, #31937, #16826, #44575, #21977, #532, #36445, #20145, #47985, #47052, #4249, #3939, #53135, #32248, #8136, #23864, #8758, #27421, #57661, #3002, #37094, #18715, #52191, #17473, #8451, #57347, #62490, #38340, #42215, #28364, #18408, #38029, #22619, #23558, #13264, #61860, #33206, #56713, #51878, #47674, #13587, #52821, #23233, #28055, #12631, #32888, #52516, #43156, #32569, #62796, #9067, #42847, #37396, #3626, #57031, #17777, #57967, #13890, #33517, #27739, #7818, #28677, #48296, #61540, #3316, #42530, #12945, #47368, #22936, #62167, #18087, #37710, #35108, #5507, #25122, #10333, #14511, #39271, #4873, #34442, #695, #54071, #5830, #29295, #39589, #33825, #54725, #59226, #15158, #5194, #9687, #19024, #53444, #38955, #24812, #34779, #376, #10010, #49568, #34133, #20308, #9376, #19343, #29943, #58280, #39908, #29622, #58593, #49253, #63426, #10645, #53754, #44735, #44415, #28987, #14199, #48611, #48924, #59553, #44098, #54403, #43467, #63113, #24493, #14828, #4550, #58899, #62, #38638, #19980, #19659, #15488, #30258, #49881, #24175, #43779, #31220, #60828, #10963, #35741, #6478, #30585, #26086, #50207, #6157, #50851, #41183, #16753, #45065, #36058, #15801, #41497, #6793, #21900, #61150, #12247, #17072, #51493, #26401, #45384, #1031, #36691, #25773, #56324, #46021, #31860, #25445, #16437, #1983, #35418, #55367, #11282, #20952, #20636, #40242, #21585, #55686, #30908, #50535, #45707, #26725, #1661, #36370, #56001, #11600, #21260, #11916, #1350, #2298, #31539, #16113, #55038, #40867, #51178, #59880, #7110, #40554, #60195, #60511, #46341, #51802, #37956, #32169, #32490, #18009, #43084, #33132, #52119, #8063, #37321, #22222 ) ),
 .UNSPECIFIED., .F., .F., .F. ) 
 B_SPLINE_SURFACE_WITH_KNOTS ( ( 2, 2 ),
 ( 3, 2, 2, 2, 2, 2, 2, 2, 2, 2, 2, 2, 2, 2, 2, 2, 2, 2, 2, 2, 2, 2, 2, 2, 2, 2, 2, 2, 2, 2, 2, 2, 2, 2, 2, 2, 2, 2, 2, 2, 2, 2, 2, 2, 2, 2, 2, 2, 2, 2, 2, 2, 2, 2, 2, 2, 2, 2, 2, 2, 2, 2, 2, 2, 2, 2, 2, 2, 2, 2, 2, 2, 2, 2, 2, 2, 2, 2, 2, 2, 2, 2, 2, 2, 2, 2, 2, 2, 2, 2, 2, 2, 2, 2, 2, 2, 2, 2, 2, 2, 2, 2, 2, 2, 2, 2, 2, 2, 2, 2, 2, 2, 2, 2, 2, 2, 2, 2, 2, 2, 2, 2, 2, 2, 2, 2, 2, 2, 2, 2, 2, 2, 2, 2, 2, 2, 2, 2, 2, 2, 2, 2, 2, 2, 2, 2, 2, 2, 2, 2, 2, 2, 2, 2, 2, 2, 2, 2, 2, 2, 2, 2, 2, 2, 2, 2, 2, 2, 2, 2, 2, 2, 2, 2, 2, 2, 2, 2, 2, 2, 2, 2, 2, 2, 2, 2, 2, 2, 2, 2, 2, 2, 2, 2, 2, 2, 2, 2, 2, 2, 2, 2, 2, 2, 2, 2, 2, 2, 2, 2, 2, 2, 2, 2, 2, 2, 2, 2, 2, 2, 2, 2, 2, 2, 2, 2, 2, 2, 2, 2, 2, 2, 2, 2, 2, 2, 2, 2, 2, 2, 2, 2, 2, 2, 2, 2, 2, 2, 2, 2, 2, 2, 2, 2, 2, 2, 2, 2, 2, 2, 2, 2, 2, 2, 2, 2, 2, 2, 2, 2, 2, 2, 2, 2, 2, 2, 2, 2, 2, 2, 2, 2, 2, 2, 2, 2, 2, 2, 2, 2, 2, 2, 2, 2, 2, 2, 2, 2, 2, 2, 2, 2, 2, 2, 2, 2, 2, 2, 2, 2, 2, 2, 2, 2, 2, 2, 2, 2, 2, 2, 2, 2, 2, 2, 2, 2, 2, 2, 2, 2, 2, 2, 2, 2, 2, 2, 2, 2, 2, 2, 2, 2, 2, 2, 2, 2, 2, 2, 2, 2, 2, 2, 2, 2, 2, 2, 2, 2, 2, 2, 2, 2, 2, 2, 2, 2, 2, 2, 2, 2, 2, 2, 2, 2, 2, 2, 2, 2, 2, 2, 2, 2, 2, 2, 2, 2, 2, 2, 2, 2, 2, 2, 2, 2, 2, 2, 2, 2, 2, 2, 2, 2, 2, 2, 2, 2, 2, 2, 2, 2, 2, 2, 2, 2, 2, 2, 2, 2, 2, 2, 2, 2, 2, 2, 2, 2, 2, 2, 2, 2, 2, 2, 2, 2, 2, 2, 2, 2, 2, 2, 2, 2, 2, 2, 2, 2, 2, 2, 2, 2, 2, 2, 2, 2, 2, 2, 2, 2, 2, 2, 2, 2, 2, 2, 2, 2, 2, 2, 2, 2, 2, 2, 2, 2, 2, 2, 2, 2, 2, 2, 2, 2, 2, 2, 2, 2, 2, 2, 2, 2, 2, 2, 2, 2, 2, 2, 2, 2, 2, 2, 2, 2, 2, 2, 2, 2, 2, 2, 2, 2, 2, 2, 2, 2, 2, 2, 2, 2, 2, 2, 2, 2, 2, 2, 2, 2, 2, 2, 2, 2, 2, 2, 2, 2, 2, 2, 2, 2, 2, 2, 2, 2, 2, 2, 2, 2, 2, 2, 2, 2, 2, 2, 2, 2, 2, 2, 2, 2, 2, 2, 2, 2, 2, 2, 2, 2, 2, 2, 2, 2, 2, 2, 2, 2, 2, 2, 2, 2, 2, 2, 2, 2, 2, 2, 2, 2, 2, 2, 2, 2, 2, 2, 2, 2, 2, 2, 2, 2, 2, 2, 2, 2, 2, 2, 2, 2, 2, 2, 2, 2, 2, 2, 2, 2, 2, 2, 2, 2, 2, 2, 2, 2, 2, 2, 2, 2, 2, 2, 2, 2, 2, 2, 2, 2, 2, 2, 2, 2, 2, 2, 2, 2, 2, 2, 2, 2, 2, 2, 2, 2, 2, 2, 2, 2, 2, 2, 2, 2, 2, 2, 2, 2, 2, 2, 2, 2, 2, 2, 2, 2, 2, 2, 2, 2, 2, 2, 2, 2, 2, 2, 2, 2, 2, 2, 2, 2, 2, 2, 2, 2, 2, 2, 2, 2, 2, 2, 2, 2, 2, 2, 2, 2, 2, 2, 2, 2, 2, 2, 2, 2, 2, 2, 2, 2, 2, 2, 2, 2, 2, 2, 2, 2, 2, 2, 2, 2, 2, 2, 2, 2, 2, 2, 2, 2, 2, 2, 2, 2, 2, 2, 2, 2, 2, 2, 2, 2, 2, 2, 2, 2, 2, 2, 2, 2, 2, 2, 2, 2, 2, 2, 2, 2, 2, 2, 2, 2, 2, 2, 2, 2, 2, 2, 2, 2, 2, 2, 2, 2, 2, 2, 2, 2, 2, 2, 2, 2, 2, 2, 2, 2, 2, 2, 2, 2, 2, 2, 2, 2, 2, 2, 2, 2, 2, 2, 2, 2, 2, 2, 2, 2, 2, 2, 2, 2, 2, 2, 2, 2, 2, 2, 2, 2, 2, 2, 2, 2, 2, 2, 2, 2, 2, 2, 2, 2, 2, 2, 2, 2, 2, 2, 3 ),
 ( 0.000000000000000000, 1.000000000000000000 ),
 ( 0.000000000000000000, 0.001190476190476190584, 0.002380952380952381167, 0.003571428571428571317, 0.004761904761904762334, 0.005952380952380952051, 0.007142857142857142634, 0.008333333333333333218, 0.009523809523809524669, 0.01071428571428571438, 0.01190476190476190410, 0.01309523809523809555, 0.01428571428571428527, 0.01547619047619047672, 0.01666666666666666644, 0.01785714285714285615, 0.01904761904761904934, 0.02023809523809523905, 0.02142857142857142877, 0.02261904761904761849, 0.02380952380952380820, 0.02500000000000000139, 0.02619047619047619110, 0.02738095238095238082, 0.02857142857142857054, 0.02976190476190476025, 0.03095238095238095344, 0.03214285714285713969, 0.03333333333333333287, 0.03452380952380952606, 0.03571428571428571230, 0.03690476190476190549, 0.03809523809523809867, 0.03928571428571428492, 0.04047619047619047811, 0.04166666666666666435, 0.04285714285714285754, 0.04404761904761905073, 0.04523809523809523697, 0.04642857142857143016, 0.04761904761904761640, 0.04880952380952380959, 0.05000000000000000278, 0.05119047619047618902, 0.05238095238095238221, 0.05357142857142856845, 0.05476190476190476164, 0.05595238095238095483, 0.05714285714285714107, 0.05833333333333333426, 0.05952380952380952051, 0.06071428571428571369, 0.06190476190476190688, 0.06309523809523809312, 0.06428571428571427937, 0.06547619047619047949, 0.06666666666666666574, 0.06785714285714285199, 0.06904761904761905211, 0.07023809523809523836, 0.07142857142857142461, 0.07261904761904762473, 0.07380952380952381098, 0.07499999999999999722, 0.07619047619047619735, 0.07738095238095238360, 0.07857142857142856984, 0.07976190476190475609, 0.08095238095238095621, 0.08214285714285714246, 0.08333333333333332871, 0.08452380952380952883, 0.08571428571428571508, 0.08690476190476190133, 0.08809523809523810145, 0.08928571428571428770, 0.09047619047619047394, 0.09166666666666666019, 0.09285714285714286031, 0.09404761904761904656, 0.09523809523809523281, 0.09642857142857143293, 0.09761904761904761918, 0.09880952380952380543, 0.1000000000000000056, 0.1011904761904761918, 0.1023809523809523780, 0.1035714285714285782, 0.1047619047619047644, 0.1059523809523809507, 0.1071428571428571369, 0.1083333333333333370, 0.1095238095238095233, 0.1107142857142857095, 0.1119047619047619097, 0.1130952380952380959, 0.1142857142857142821, 0.1154761904761904823, 0.1166666666666666685, 0.1178571428571428548, 0.1190476190476190410, 0.1202380952380952411, 0.1214285714285714274, 0.1226190476190476136, 0.1238095238095238138, 0.1250000000000000000, 0.1261904761904761862, 0.1273809523809523725, 0.1285714285714285587, 0.1297619047619047727, 0.1309523809523809590, 0.1321428571428571452, 0.1333333333333333315, 0.1345238095238095177, 0.1357142857142857040, 0.1369047619047619180, 0.1380952380952381042, 0.1392857142857142905, 0.1404761904761904767, 0.1416666666666666630, 0.1428571428571428492, 0.1440476190476190355, 0.1452380952380952495, 0.1464285714285714357, 0.1476190476190476220, 0.1488095238095238082, 0.1499999999999999944, 0.1511904761904761807, 0.1523809523809523947, 0.1535714285714285809, 0.1547619047619047672, 0.1559523809523809534, 0.1571428571428571397, 0.1583333333333333259, 0.1595238095238095122, 0.1607142857142857262, 0.1619047619047619124, 0.1630952380952380987, 0.1642857142857142849, 0.1654761904761904712, 0.1666666666666666574, 0.1678571428571428437, 0.1690476190476190577, 0.1702380952380952439, 0.1714285714285714302, 0.1726190476190476164, 0.1738095238095238027, 0.1749999999999999889, 0.1761904761904762029, 0.1773809523809523891, 0.1785714285714285754, 0.1797619047619047616, 0.1809523809523809479, 0.1821428571428571341, 0.1833333333333333204, 0.1845238095238095344, 0.1857142857142857206, 0.1869047619047619069, 0.1880952380952380931, 0.1892857142857142794, 0.1904761904761904656, 0.1916666666666666796, 0.1928571428571428659, 0.1940476190476190521, 0.1952380952380952384, 0.1964285714285714246, 0.1976190476190476109, 0.1988095238095237971, 0.2000000000000000111, 0.2011904761904761973, 0.2023809523809523836, 0.2035714285714285698, 0.2047619047619047561, 0.2059523809523809423, 0.2071428571428571563, 0.2083333333333333426, 0.2095238095238095288, 0.2107142857142857151, 0.2119047619047619013, 0.2130952380952380876, 0.2142857142857142738, 0.2154761904761904878, 0.2166666666666666741, 0.2178571428571428603, 0.2190476190476190466, 0.2202380952380952328, 0.2214285714285714191, 0.2226190476190476053, 0.2238095238095238193, 0.2250000000000000056, 0.2261904761904761918, 0.2273809523809523780, 0.2285714285714285643, 0.2297619047619047505, 0.2309523809523809645, 0.2321428571428571508, 0.2333333333333333370, 0.2345238095238095233, 0.2357142857142857095, 0.2369047619047618958, 0.2380952380952380820, 0.2392857142857142960, 0.2404761904761904823, 0.2416666666666666685, 0.2428571428571428548, 0.2440476190476190410, 0.2452380952380952273, 0.2464285714285714413, 0.2476190476190476275, 0.2488095238095238138, 0.2500000000000000000, 0.2511904761904761862, 0.2523809523809523725, 0.2535714285714285587, 0.2547619047619047450, 0.2559523809523809312, 0.2571428571428571175, 0.2583333333333333592, 0.2595238095238095455, 0.2607142857142857317, 0.2619047619047619180, 0.2630952380952381042, 0.2642857142857142905, 0.2654761904761904767, 0.2666666666666666630, 0.2678571428571428492, 0.2690476190476190355, 0.2702380952380952217, 0.2714285714285714080, 0.2726190476190475942, 0.2738095238095238360, 0.2750000000000000222, 0.2761904761904762085, 0.2773809523809523947, 0.2785714285714285809, 0.2797619047619047672, 0.2809523809523809534, 0.2821428571428571397, 0.2833333333333333259, 0.2845238095238095122, 0.2857142857142856984, 0.2869047619047618847, 0.2880952380952380709, 0.2892857142857143127, 0.2904761904761904989, 0.2916666666666666852, 0.2928571428571428714, 0.2940476190476190577, 0.2952380952380952439, 0.2964285714285714302, 0.2976190476190476164, 0.2988095238095238027, 0.2999999999999999889, 0.3011904761904761751, 0.3023809523809523614, 0.3035714285714285476, 0.3047619047619047894, 0.3059523809523809756, 0.3071428571428571619, 0.3083333333333333481, 0.3095238095238095344, 0.3107142857142857206, 0.3119047619047619069, 0.3130952380952380931, 0.3142857142857142794, 0.3154761904761904656, 0.3166666666666666519, 0.3178571428571428381, 0.3190476190476190244, 0.3202380952380952106, 0.3214285714285714524, 0.3226190476190476386, 0.3238095238095238249, 0.3250000000000000111, 0.3261904761904761973, 0.3273809523809523836, 0.3285714285714285698, 0.3297619047619047561, 0.3309523809523809423, 0.3321428571428571286, 0.3333333333333333148, 0.3345238095238095011, 0.3357142857142856873, 0.3369047619047619291, 0.3380952380952381153, 0.3392857142857143016, 0.3404761904761904878, 0.3416666666666666741, 0.3428571428571428603, 0.3440476190476190466, 0.3452380952380952328, 0.3464285714285714191, 0.3476190476190476053, 0.3488095238095237915, 0.3499999999999999778, 0.3511904761904761640, 0.3523809523809524058, 0.3535714285714285920, 0.3547619047619047783, 0.3559523809523809645, 0.3571428571428571508, 0.3583333333333333370, 0.3595238095238095233, 0.3607142857142857095, 0.3619047619047618958, 0.3630952380952380820, 0.3642857142857142683, 0.3654761904761904545, 0.3666666666666666408, 0.3678571428571428825, 0.3690476190476190688, 0.3702380952380952550, 0.3714285714285714413, 0.3726190476190476275, 0.3738095238095238138, 0.3750000000000000000, 0.3761904761904761862, 0.3773809523809523725, 0.3785714285714285587, 0.3797619047619047450, 0.3809523809523809312, 0.3821428571428571175, 0.3833333333333333592, 0.3845238095238095455, 0.3857142857142857317, 0.3869047619047619180, 0.3880952380952381042, 0.3892857142857142905, 0.3904761904761904767, 0.3916666666666666630, 0.3928571428571428492, 0.3940476190476190355, 0.3952380952380952217, 0.3964285714285714080, 0.3976190476190475942, 0.3988095238095238360, 0.4000000000000000222, 0.4011904761904762085, 0.4023809523809523947, 0.4035714285714285809, 0.4047619047619047672, 0.4059523809523809534, 0.4071428571428571397, 0.4083333333333333259, 0.4095238095238095122, 0.4107142857142856984, 0.4119047619047618847, 0.4130952380952380709, 0.4142857142857143127, 0.4154761904761904989, 0.4166666666666666852, 0.4178571428571428714, 0.4190476190476190577, 0.4202380952380952439, 0.4214285714285714302, 0.4226190476190476164, 0.4238095238095238027, 0.4249999999999999889, 0.4261904761904761751, 0.4273809523809523614, 0.4285714285714285476, 0.4297619047619047894, 0.4309523809523809756, 0.4321428571428571619, 0.4333333333333333481, 0.4345238095238095344, 0.4357142857142857206, 0.4369047619047619069, 0.4380952380952380931, 0.4392857142857142794, 0.4404761904761904656, 0.4416666666666666519, 0.4428571428571428381, 0.4440476190476190244, 0.4452380952380952106, 0.4464285714285714524, 0.4476190476190476386, 0.4488095238095238249, 0.4500000000000000111, 0.4511904761904761973, 0.4523809523809523836, 0.4535714285714285698, 0.4547619047619047561, 0.4559523809523809423, 0.4571428571428571286, 0.4583333333333333148, 0.4595238095238095011, 0.4607142857142856873, 0.4619047619047619291, 0.4630952380952381153, 0.4642857142857143016, 0.4654761904761904878, 0.4666666666666666741, 0.4678571428571428603, 0.4690476190476190466, 0.4702380952380952328, 0.4714285714285714191, 0.4726190476190476053, 0.4738095238095237915, 0.4749999999999999778, 0.4761904761904761640, 0.4773809523809524058, 0.4785714285714285920, 0.4797619047619047783, 0.4809523809523809645, 0.4821428571428571508, 0.4833333333333333370, 0.4845238095238095233, 0.4857142857142857095, 0.4869047619047618958, 0.4880952380952380820, 0.4892857142857142683, 0.4904761904761904545, 0.4916666666666666408, 0.4928571428571428825, 0.4940476190476190688, 0.4952380952380952550, 0.4964285714285714413, 0.4976190476190476275, 0.4988095238095238138, 0.5000000000000000000, 0.5011904761904761862, 0.5023809523809523725, 0.5035714285714285587, 0.5047619047619047450, 0.5059523809523809312, 0.5071428571428571175, 0.5083333333333333037, 0.5095238095238094900, 0.5107142857142856762, 0.5119047619047618625, 0.5130952380952380487, 0.5142857142857142350, 0.5154761904761904212, 0.5166666666666667185, 0.5178571428571429047, 0.5190476190476190910, 0.5202380952380952772, 0.5214285714285714635, 0.5226190476190476497, 0.5238095238095238360, 0.5250000000000000222, 0.5261904761904762085, 0.5273809523809523947, 0.5285714285714285809, 0.5297619047619047672, 0.5309523809523809534, 0.5321428571428571397, 0.5333333333333333259, 0.5345238095238095122, 0.5357142857142856984, 0.5369047619047618847, 0.5380952380952380709, 0.5392857142857142572, 0.5404761904761904434, 0.5416666666666666297, 0.5428571428571428159, 0.5440476190476190022, 0.5452380952380951884, 0.5464285714285713746, 0.5476190476190476719, 0.5488095238095238582, 0.5500000000000000444, 0.5511904761904762307, 0.5523809523809524169, 0.5535714285714286031, 0.5547619047619047894, 0.5559523809523809756, 0.5571428571428571619, 0.5583333333333333481, 0.5595238095238095344, 0.5607142857142857206, 0.5619047619047619069, 0.5630952380952380931, 0.5642857142857142794, 0.5654761904761904656, 0.5666666666666666519, 0.5678571428571428381, 0.5690476190476190244, 0.5702380952380952106, 0.5714285714285713969, 0.5726190476190475831, 0.5738095238095237693, 0.5749999999999999556, 0.5761904761904761418, 0.5773809523809523281, 0.5785714285714286254, 0.5797619047619048116, 0.5809523809523809978, 0.5821428571428571841, 0.5833333333333333703, 0.5845238095238095566, 0.5857142857142857428, 0.5869047619047619291, 0.5880952380952381153, 0.5892857142857143016, 0.5904761904761904878, 0.5916666666666666741, 0.5928571428571428603, 0.5940476190476190466, 0.5952380952380952328, 0.5964285714285714191, 0.5976190476190476053, 0.5988095238095237915, 0.5999999999999999778, 0.6011904761904761640, 0.6023809523809523503, 0.6035714285714285365, 0.6047619047619047228, 0.6059523809523809090, 0.6071428571428570953, 0.6083333333333332815, 0.6095238095238095788, 0.6107142857142857650, 0.6119047619047619513, 0.6130952380952381375, 0.6142857142857143238, 0.6154761904761905100, 0.6166666666666666963, 0.6178571428571428825, 0.6190476190476190688, 0.6202380952380952550, 0.6214285714285714413, 0.6226190476190476275, 0.6238095238095238138, 0.6250000000000000000, 0.6261904761904761862, 0.6273809523809523725, 0.6285714285714285587, 0.6297619047619047450, 0.6309523809523809312, 0.6321428571428571175, 0.6333333333333333037, 0.6345238095238094900, 0.6357142857142856762, 0.6369047619047618625, 0.6380952380952380487, 0.6392857142857142350, 0.6404761904761904212, 0.6416666666666667185, 0.6428571428571429047, 0.6440476190476190910, 0.6452380952380952772, 0.6464285714285714635, 0.6476190476190476497, 0.6488095238095238360, 0.6500000000000000222, 0.6511904761904762085, 0.6523809523809523947, 0.6535714285714285809, 0.6547619047619047672, 0.6559523809523809534, 0.6571428571428571397, 0.6583333333333333259, 0.6595238095238095122, 0.6607142857142856984, 0.6619047619047618847, 0.6630952380952380709, 0.6642857142857142572, 0.6654761904761904434, 0.6666666666666666297, 0.6678571428571428159, 0.6690476190476190022, 0.6702380952380951884, 0.6714285714285713746, 0.6726190476190476719, 0.6738095238095238582, 0.6750000000000000444, 0.6761904761904762307, 0.6773809523809524169, 0.6785714285714286031, 0.6797619047619047894, 0.6809523809523809756, 0.6821428571428571619, 0.6833333333333333481, 0.6845238095238095344, 0.6857142857142857206, 0.6869047619047619069, 0.6880952380952380931, 0.6892857142857142794, 0.6904761904761904656, 0.6916666666666666519, 0.6928571428571428381, 0.6940476190476190244, 0.6952380952380952106, 0.6964285714285713969, 0.6976190476190475831, 0.6988095238095237693, 0.6999999999999999556, 0.7011904761904761418, 0.7023809523809523281, 0.7035714285714286254, 0.7047619047619048116, 0.7059523809523809978, 0.7071428571428571841, 0.7083333333333333703, 0.7095238095238095566, 0.7107142857142857428, 0.7119047619047619291, 0.7130952380952381153, 0.7142857142857143016, 0.7154761904761904878, 0.7166666666666666741, 0.7178571428571428603, 0.7190476190476190466, 0.7202380952380952328, 0.7214285714285714191, 0.7226190476190476053, 0.7238095238095237915, 0.7249999999999999778, 0.7261904761904761640, 0.7273809523809523503, 0.7285714285714285365, 0.7297619047619047228, 0.7309523809523809090, 0.7321428571428570953, 0.7333333333333332815, 0.7345238095238095788, 0.7357142857142857650, 0.7369047619047619513, 0.7380952380952381375, 0.7392857142857143238, 0.7404761904761905100, 0.7416666666666666963, 0.7428571428571428825, 0.7440476190476190688, 0.7452380952380952550, 0.7464285714285714413, 0.7476190476190476275, 0.7488095238095238138, 0.7500000000000000000, 0.7511904761904761862, 0.7523809523809523725, 0.7535714285714285587, 0.7547619047619047450, 0.7559523809523809312, 0.7571428571428571175, 0.7583333333333333037, 0.7595238095238094900, 0.7607142857142856762, 0.7619047619047618625, 0.7630952380952380487, 0.7642857142857142350, 0.7654761904761904212, 0.7666666666666667185, 0.7678571428571429047, 0.7690476190476190910, 0.7702380952380952772, 0.7714285714285714635, 0.7726190476190476497, 0.7738095238095238360, 0.7750000000000000222, 0.7761904761904762085, 0.7773809523809523947, 0.7785714285714285809, 0.7797619047619047672, 0.7809523809523809534, 0.7821428571428571397, 0.7833333333333333259, 0.7845238095238095122, 0.7857142857142856984, 0.7869047619047618847, 0.7880952380952380709, 0.7892857142857142572, 0.7904761904761904434, 0.7916666666666666297, 0.7928571428571428159, 0.7940476190476190022, 0.7952380952380951884, 0.7964285714285713746, 0.7976190476190476719, 0.7988095238095238582, 0.8000000000000000444, 0.8011904761904762307, 0.8023809523809524169, 0.8035714285714286031, 0.8047619047619047894, 0.8059523809523809756, 0.8071428571428571619, 0.8083333333333333481, 0.8095238095238095344, 0.8107142857142857206, 0.8119047619047619069, 0.8130952380952380931, 0.8142857142857142794, 0.8154761904761904656, 0.8166666666666666519, 0.8178571428571428381, 0.8190476190476190244, 0.8202380952380952106, 0.8214285714285713969, 0.8226190476190475831, 0.8238095238095237693, 0.8249999999999999556, 0.8261904761904761418, 0.8273809523809523281, 0.8285714285714286254, 0.8297619047619048116, 0.8309523809523809978, 0.8321428571428571841, 0.8333333333333333703, 0.8345238095238095566, 0.8357142857142857428, 0.8369047619047619291, 0.8380952380952381153, 0.8392857142857143016, 0.8404761904761904878, 0.8416666666666666741, 0.8428571428571428603, 0.8440476190476190466, 0.8452380952380952328, 0.8464285714285714191, 0.8476190476190476053, 0.8488095238095237915, 0.8499999999999999778, 0.8511904761904761640, 0.8523809523809523503, 0.8535714285714285365, 0.8547619047619047228, 0.8559523809523809090, 0.8571428571428570953, 0.8583333333333332815, 0.8595238095238095788, 0.8607142857142857650, 0.8619047619047619513, 0.8630952380952381375, 0.8642857142857143238, 0.8654761904761905100, 0.8666666666666666963, 0.8678571428571428825, 0.8690476190476190688, 0.8702380952380952550, 0.8714285714285714413, 0.8726190476190476275, 0.8738095238095238138, 0.8750000000000000000, 0.8761904761904761862, 0.8773809523809523725, 0.8785714285714285587, 0.8797619047619047450, 0.8809523809523809312, 0.8821428571428571175, 0.8833333333333333037, 0.8845238095238094900, 0.8857142857142856762, 0.8869047619047618625, 0.8880952380952380487, 0.8892857142857142350, 0.8904761904761904212, 0.8916666666666667185, 0.8928571428571429047, 0.8940476190476190910, 0.8952380952380952772, 0.8964285714285714635, 0.8976190476190476497, 0.8988095238095238360, 0.9000000000000000222, 0.9011904761904762085, 0.9023809523809523947, 0.9035714285714285809, 0.9047619047619047672, 0.9059523809523809534, 0.9071428571428571397, 0.9083333333333333259, 0.9095238095238095122, 0.9107142857142856984, 0.9119047619047618847, 0.9130952380952380709, 0.9142857142857142572, 0.9154761904761904434, 0.9166666666666666297, 0.9178571428571428159, 0.9190476190476190022, 0.9202380952380951884, 0.9214285714285713746, 0.9226190476190476719, 0.9238095238095238582, 0.9250000000000000444, 0.9261904761904762307, 0.9273809523809524169, 0.9285714285714286031, 0.9297619047619047894, 0.9309523809523809756, 0.9321428571428571619, 0.9333333333333333481, 0.9345238095238095344, 0.9357142857142857206, 0.9369047619047619069, 0.9380952380952380931, 0.9392857142857142794, 0.9404761904761904656, 0.9416666666666666519, 0.9428571428571428381, 0.9440476190476190244, 0.9452380952380952106, 0.9464285714285713969, 0.9476190476190475831, 0.9488095238095237693, 0.9499999999999999556, 0.9511904761904761418, 0.9523809523809523281, 0.9535714285714286254, 0.9547619047619048116, 0.9559523809523809978, 0.9571428571428571841, 0.9583333333333333703, 0.9595238095238095566, 0.9607142857142857428, 0.9619047619047619291, 0.9630952380952381153, 0.9642857142857143016, 0.9654761904761904878, 0.9666666666666666741, 0.9678571428571428603, 0.9690476190476190466, 0.9702380952380952328, 0.9714285714285714191, 0.9726190476190476053, 0.9738095238095237915, 0.9749999999999999778, 0.9761904761904761640, 0.9773809523809523503, 0.9785714285714285365, 0.9797619047619047228, 0.9809523809523809090, 0.9821428571428570953, 0.9833333333333332815, 0.9845238095238095788, 0.9857142857142857650, 0.9869047619047619513, 0.9880952380952381375, 0.9892857142857143238, 0.9904761904761905100, 0.9916666666666666963, 0.9928571428571428825, 0.9940476190476190688, 0.9952380952380952550, 0.9964285714285714413, 0.9976190476190476275, 0.9988095238095238138, 1.000000000000000000 ),
 .UNSPECIFIED. ) 
 GEOMETRIC_REPRESENTATION_ITEM ( )  RATIONAL_B_SPLINE_SURFACE ( (
 ( 1.000000000000000000, 0.8660254037844387076, 1.000000000000000000, 0.8660254037844387076, 1.000000000000000000, 0.8660254037844387076, 1.000000000000000000, 0.8660254037844387076, 1.000000000000000000, 0.8660254037844387076, 1.000000000000000000, 0.8660254037844387076, 1.000000000000000000, 0.8660254037844387076, 1.000000000000000000, 0.8660254037844387076, 1.000000000000000000, 0.8660254037844387076, 1.000000000000000000, 0.8660254037844387076, 1.000000000000000000, 0.8660254037844387076, 1.000000000000000000, 0.8660254037844387076, 1.000000000000000000, 0.8660254037844387076, 1.000000000000000000, 0.8660254037844387076, 1.000000000000000000, 0.8660254037844387076, 1.000000000000000000, 0.8660254037844387076, 1.000000000000000000, 0.8660254037844387076, 1.000000000000000000, 0.8660254037844387076, 1.000000000000000000, 0.8660254037844387076, 1.000000000000000000, 0.8660254037844387076, 1.000000000000000000, 0.8660254037844387076, 1.000000000000000000, 0.8660254037844387076, 1.000000000000000000, 0.8660254037844387076, 1.000000000000000000, 0.8660254037844387076, 1.000000000000000000, 0.8660254037844387076, 1.000000000000000000, 0.8660254037844387076, 1.000000000000000000, 0.8660254037844387076, 1.000000000000000000, 0.8660254037844387076, 1.000000000000000000, 0.8660254037844387076, 1.000000000000000000, 0.8660254037844387076, 1.000000000000000000, 0.8660254037844387076, 1.000000000000000000, 0.8660254037844387076, 1.000000000000000000, 0.8660254037844387076, 1.000000000000000000, 0.8660254037844387076, 1.000000000000000000, 0.8660254037844387076, 1.000000000000000000, 0.8660254037844387076, 1.000000000000000000, 0.8660254037844387076, 1.000000000000000000, 0.8660254037844387076, 1.000000000000000000, 0.8660254037844387076, 1.000000000000000000, 0.8660254037844387076, 1.000000000000000000, 0.8660254037844387076, 1.000000000000000000, 0.8660254037844387076, 1.000000000000000000, 0.8660254037844387076, 1.000000000000000000, 0.8660254037844387076, 1.000000000000000000, 0.8660254037844387076, 1.000000000000000000, 0.8660254037844387076, 1.000000000000000000, 0.8660254037844387076, 1.000000000000000000, 0.8660254037844387076, 1.000000000000000000, 0.8660254037844387076, 1.000000000000000000, 0.8660254037844387076, 1.000000000000000000, 0.8660254037844387076, 1.000000000000000000, 0.8660254037844387076, 1.000000000000000000, 0.8660254037844387076, 1.000000000000000000, 0.8660254037844387076, 1.000000000000000000, 0.8660254037844387076, 1.000000000000000000, 0.8660254037844387076, 1.000000000000000000, 0.8660254037844387076, 1.000000000000000000, 0.8660254037844387076, 1.000000000000000000, 0.8660254037844387076, 1.000000000000000000, 0.8660254037844387076, 1.000000000000000000, 0.8660254037844387076, 1.000000000000000000, 0.8660254037844387076, 1.000000000000000000, 0.8660254037844387076, 1.000000000000000000, 0.8660254037844387076, 1.000000000000000000, 0.8660254037844387076, 1.000000000000000000, 0.8660254037844387076, 1.000000000000000000, 0.8660254037844387076, 1.000000000000000000, 0.8660254037844387076, 1.000000000000000000, 0.8660254037844387076, 1.000000000000000000, 0.8660254037844387076, 1.000000000000000000, 0.8660254037844387076, 1.000000000000000000, 0.8660254037844387076, 1.000000000000000000, 0.8660254037844387076, 1.000000000000000000, 0.8660254037844387076, 1.000000000000000000, 0.8660254037844387076, 1.000000000000000000, 0.8660254037844387076, 1.000000000000000000, 0.8660254037844387076, 1.000000000000000000, 0.8660254037844387076, 1.000000000000000000, 0.8660254037844387076, 1.000000000000000000, 0.8660254037844387076, 1.000000000000000000, 0.8660254037844387076, 1.000000000000000000, 0.8660254037844387076, 1.000000000000000000, 0.8660254037844387076, 1.000000000000000000, 0.8660254037844387076, 1.000000000000000000, 0.8660254037844387076, 1.000000000000000000, 0.8660254037844387076, 1.000000000000000000, 0.8660254037844387076, 1.000000000000000000, 0.8660254037844387076, 1.000000000000000000, 0.8660254037844387076, 1.000000000000000000, 0.8660254037844387076, 1.000000000000000000, 0.8660254037844387076, 1.000000000000000000, 0.8660254037844387076, 1.000000000000000000, 0.8660254037844387076, 1.000000000000000000, 0.8660254037844387076, 1.000000000000000000, 0.8660254037844387076, 1.000000000000000000, 0.8660254037844387076, 1.000000000000000000, 0.8660254037844387076, 1.000000000000000000, 0.8660254037844387076, 1.000000000000000000, 0.8660254037844387076, 1.000000000000000000, 0.8660254037844387076, 1.000000000000000000, 0.8660254037844387076, 1.000000000000000000, 0.8660254037844387076, 1.000000000000000000, 0.8660254037844387076, 1.000000000000000000, 0.8660254037844387076, 1.000000000000000000, 0.8660254037844387076, 1.000000000000000000, 0.8660254037844387076, 1.000000000000000000, 0.8660254037844387076, 1.000000000000000000, 0.8660254037844387076, 1.000000000000000000, 0.8660254037844387076, 1.000000000000000000, 0.8660254037844387076, 1.000000000000000000, 0.8660254037844387076, 1.000000000000000000, 0.8660254037844387076, 1.000000000000000000, 0.8660254037844387076, 1.000000000000000000, 0.8660254037844387076, 1.000000000000000000, 0.8660254037844387076, 1.000000000000000000, 0.8660254037844387076, 1.000000000000000000, 0.8660254037844387076, 1.000000000000000000, 0.8660254037844387076, 1.000000000000000000, 0.8660254037844387076, 1.000000000000000000, 0.8660254037844387076, 1.000000000000000000, 0.8660254037844387076, 1.000000000000000000, 0.8660254037844387076, 1.000000000000000000, 0.8660254037844387076, 1.000000000000000000, 0.8660254037844387076, 1.000000000000000000, 0.8660254037844387076, 1.000000000000000000, 0.8660254037844387076, 1.000000000000000000, 0.8660254037844387076, 1.000000000000000000, 0.8660254037844387076, 1.000000000000000000, 0.8660254037844387076, 1.000000000000000000, 0.8660254037844387076, 1.000000000000000000, 0.8660254037844387076, 1.000000000000000000, 0.8660254037844387076, 1.000000000000000000, 0.8660254037844387076, 1.000000000000000000, 0.8660254037844387076, 1.000000000000000000, 0.8660254037844387076, 1.000000000000000000, 0.8660254037844387076, 1.000000000000000000, 0.8660254037844387076, 1.000000000000000000, 0.8660254037844387076, 1.000000000000000000, 0.8660254037844387076, 1.000000000000000000, 0.8660254037844387076, 1.000000000000000000, 0.8660254037844387076, 1.000000000000000000, 0.8660254037844387076, 1.000000000000000000, 0.8660254037844387076, 1.000000000000000000, 0.8660254037844387076, 1.000000000000000000, 0.8660254037844387076, 1.000000000000000000, 0.8660254037844387076, 1.000000000000000000, 0.8660254037844387076, 1.000000000000000000, 0.8660254037844387076, 1.000000000000000000, 0.8660254037844387076, 1.000000000000000000, 0.8660254037844387076, 1.000000000000000000, 0.8660254037844387076, 1.000000000000000000, 0.8660254037844387076, 1.000000000000000000, 0.8660254037844387076, 1.000000000000000000, 0.8660254037844387076, 1.000000000000000000, 0.8660254037844387076, 1.000000000000000000, 0.8660254037844387076, 1.000000000000000000, 0.8660254037844387076, 1.000000000000000000, 0.8660254037844387076, 1.000000000000000000, 0.8660254037844387076, 1.000000000000000000, 0.8660254037844387076, 1.000000000000000000, 0.8660254037844387076, 1.000000000000000000, 0.8660254037844387076, 1.000000000000000000, 0.8660254037844387076, 1.000000000000000000, 0.8660254037844387076, 1.000000000000000000, 0.8660254037844387076, 1.000000000000000000, 0.8660254037844387076, 1.000000000000000000, 0.8660254037844387076, 1.000000000000000000, 0.8660254037844387076, 1.000000000000000000, 0.8660254037844387076, 1.000000000000000000, 0.8660254037844387076, 1.000000000000000000, 0.8660254037844387076, 1.000000000000000000, 0.8660254037844387076, 1.000000000000000000, 0.8660254037844387076, 1.000000000000000000, 0.8660254037844387076, 1.000000000000000000, 0.8660254037844387076, 1.000000000000000000, 0.8660254037844387076, 1.000000000000000000, 0.8660254037844387076, 1.000000000000000000, 0.8660254037844387076, 1.000000000000000000, 0.8660254037844387076, 1.000000000000000000, 0.8660254037844387076, 1.000000000000000000, 0.8660254037844387076, 1.000000000000000000, 0.8660254037844387076, 1.000000000000000000, 0.8660254037844387076, 1.000000000000000000, 0.8660254037844387076, 1.000000000000000000, 0.8660254037844387076, 1.000000000000000000, 0.8660254037844387076, 1.000000000000000000, 0.8660254037844387076, 1.000000000000000000, 0.8660254037844387076, 1.000000000000000000, 0.8660254037844387076, 1.000000000000000000, 0.8660254037844387076, 1.000000000000000000, 0.8660254037844387076, 1.000000000000000000, 0.8660254037844387076, 1.000000000000000000, 0.8660254037844387076, 1.000000000000000000, 0.8660254037844387076, 1.000000000000000000, 0.8660254037844387076, 1.000000000000000000, 0.8660254037844387076, 1.000000000000000000, 0.8660254037844387076, 1.000000000000000000, 0.8660254037844387076, 1.000000000000000000, 0.8660254037844387076, 1.000000000000000000, 0.8660254037844387076, 1.000000000000000000, 0.8660254037844387076, 1.000000000000000000, 0.8660254037844387076, 1.000000000000000000, 0.8660254037844387076, 1.000000000000000000, 0.8660254037844387076, 1.000000000000000000, 0.8660254037844387076, 1.000000000000000000, 0.8660254037844387076, 1.000000000000000000, 0.8660254037844387076, 1.000000000000000000, 0.8660254037844387076, 1.000000000000000000, 0.8660254037844387076, 1.000000000000000000, 0.8660254037844387076, 1.000000000000000000, 0.8660254037844387076, 1.000000000000000000, 0.8660254037844387076, 1.000000000000000000, 0.8660254037844387076, 1.000000000000000000, 0.8660254037844387076, 1.000000000000000000, 0.8660254037844387076, 1.000000000000000000, 0.8660254037844387076, 1.000000000000000000, 0.8660254037844387076, 1.000000000000000000, 0.8660254037844387076, 1.000000000000000000, 0.8660254037844387076, 1.000000000000000000, 0.8660254037844387076, 1.000000000000000000, 0.8660254037844387076, 1.000000000000000000, 0.8660254037844387076, 1.000000000000000000, 0.8660254037844387076, 1.000000000000000000, 0.8660254037844387076, 1.000000000000000000, 0.8660254037844387076, 1.000000000000000000, 0.8660254037844387076, 1.000000000000000000, 0.8660254037844387076, 1.000000000000000000, 0.8660254037844387076, 1.000000000000000000, 0.8660254037844387076, 1.000000000000000000, 0.8660254037844387076, 1.000000000000000000, 0.8660254037844387076, 1.000000000000000000, 0.8660254037844387076, 1.000000000000000000, 0.8660254037844387076, 1.000000000000000000, 0.8660254037844387076, 1.000000000000000000, 0.8660254037844387076, 1.000000000000000000, 0.8660254037844387076, 1.000000000000000000, 0.8660254037844387076, 1.000000000000000000, 0.8660254037844387076, 1.000000000000000000, 0.8660254037844387076, 1.000000000000000000, 0.8660254037844387076, 1.000000000000000000, 0.8660254037844387076, 1.000000000000000000, 0.8660254037844387076, 1.000000000000000000, 0.8660254037844387076, 1.000000000000000000, 0.8660254037844387076, 1.000000000000000000, 0.8660254037844387076, 1.000000000000000000, 0.8660254037844387076, 1.000000000000000000, 0.8660254037844387076, 1.000000000000000000, 0.8660254037844387076, 1.000000000000000000, 0.8660254037844387076, 1.000000000000000000, 0.8660254037844387076, 1.000000000000000000, 0.8660254037844387076, 1.000000000000000000, 0.8660254037844387076, 1.000000000000000000, 0.8660254037844387076, 1.000000000000000000, 0.8660254037844387076, 1.000000000000000000, 0.8660254037844387076, 1.000000000000000000, 0.8660254037844387076, 1.000000000000000000, 0.8660254037844387076, 1.000000000000000000, 0.8660254037844387076, 1.000000000000000000, 0.8660254037844387076, 1.000000000000000000, 0.8660254037844387076, 1.000000000000000000, 0.8660254037844387076, 1.000000000000000000, 0.8660254037844387076, 1.000000000000000000, 0.8660254037844387076, 1.000000000000000000, 0.8660254037844387076, 1.000000000000000000, 0.8660254037844387076, 1.000000000000000000, 0.8660254037844387076, 1.000000000000000000, 0.8660254037844387076, 1.000000000000000000, 0.8660254037844387076, 1.000000000000000000, 0.8660254037844387076, 1.000000000000000000, 0.8660254037844387076, 1.000000000000000000, 0.8660254037844387076, 1.000000000000000000, 0.8660254037844387076, 1.000000000000000000, 0.8660254037844387076, 1.000000000000000000, 0.8660254037844387076, 1.000000000000000000, 0.8660254037844387076, 1.000000000000000000, 0.8660254037844387076, 1.000000000000000000, 0.8660254037844387076, 1.000000000000000000, 0.8660254037844387076, 1.000000000000000000, 0.8660254037844387076, 1.000000000000000000, 0.8660254037844387076, 1.000000000000000000, 0.8660254037844387076, 1.000000000000000000, 0.8660254037844387076, 1.000000000000000000, 0.8660254037844387076, 1.000000000000000000, 0.8660254037844387076, 1.000000000000000000, 0.8660254037844387076, 1.000000000000000000, 0.8660254037844387076, 1.000000000000000000, 0.8660254037844387076, 1.000000000000000000, 0.8660254037844387076, 1.000000000000000000, 0.8660254037844387076, 1.000000000000000000, 0.8660254037844387076, 1.000000000000000000, 0.8660254037844387076, 1.000000000000000000, 0.8660254037844387076, 1.000000000000000000, 0.8660254037844387076, 1.000000000000000000, 0.8660254037844387076, 1.000000000000000000, 0.8660254037844387076, 1.000000000000000000, 0.8660254037844387076, 1.000000000000000000, 0.8660254037844387076, 1.000000000000000000, 0.8660254037844387076, 1.000000000000000000, 0.8660254037844387076, 1.000000000000000000, 0.8660254037844387076, 1.000000000000000000, 0.8660254037844387076, 1.000000000000000000, 0.8660254037844387076, 1.000000000000000000, 0.8660254037844387076, 1.000000000000000000, 0.8660254037844387076, 1.000000000000000000, 0.8660254037844387076, 1.000000000000000000, 0.8660254037844387076, 1.000000000000000000, 0.8660254037844387076, 1.000000000000000000, 0.8660254037844387076, 1.000000000000000000, 0.8660254037844387076, 1.000000000000000000, 0.8660254037844387076, 1.000000000000000000, 0.8660254037844387076, 1.000000000000000000, 0.8660254037844387076, 1.000000000000000000, 0.8660254037844387076, 1.000000000000000000, 0.8660254037844387076, 1.000000000000000000, 0.8660254037844387076, 1.000000000000000000, 0.8660254037844387076, 1.000000000000000000, 0.8660254037844387076, 1.000000000000000000, 0.8660254037844387076, 1.000000000000000000, 0.8660254037844387076, 1.000000000000000000, 0.8660254037844387076, 1.000000000000000000, 0.8660254037844387076, 1.000000000000000000, 0.8660254037844387076, 1.000000000000000000, 0.8660254037844387076, 1.000000000000000000, 0.8660254037844387076, 1.000000000000000000, 0.8660254037844387076, 1.000000000000000000, 0.8660254037844387076, 1.000000000000000000, 0.8660254037844387076, 1.000000000000000000, 0.8660254037844387076, 1.000000000000000000, 0.8660254037844387076, 1.000000000000000000, 0.8660254037844387076, 1.000000000000000000, 0.8660254037844387076, 1.000000000000000000, 0.8660254037844387076, 1.000000000000000000, 0.8660254037844387076, 1.000000000000000000, 0.8660254037844387076, 1.000000000000000000, 0.8660254037844387076, 1.000000000000000000, 0.8660254037844387076, 1.000000000000000000, 0.8660254037844387076, 1.000000000000000000, 0.8660254037844387076, 1.000000000000000000, 0.8660254037844387076, 1.000000000000000000, 0.8660254037844387076, 1.000000000000000000, 0.8660254037844387076, 1.000000000000000000, 0.8660254037844387076, 1.000000000000000000, 0.8660254037844387076, 1.000000000000000000, 0.8660254037844387076, 1.000000000000000000, 0.8660254037844387076, 1.000000000000000000, 0.8660254037844387076, 1.000000000000000000, 0.8660254037844387076, 1.000000000000000000, 0.8660254037844387076, 1.000000000000000000, 0.8660254037844387076, 1.000000000000000000, 0.8660254037844387076, 1.000000000000000000, 0.8660254037844387076, 1.000000000000000000, 0.8660254037844387076, 1.000000000000000000, 0.8660254037844387076, 1.000000000000000000, 0.8660254037844387076, 1.000000000000000000, 0.8660254037844387076, 1.000000000000000000, 0.8660254037844387076, 1.000000000000000000, 0.8660254037844387076, 1.000000000000000000, 0.8660254037844387076, 1.000000000000000000, 0.8660254037844387076, 1.000000000000000000, 0.8660254037844387076, 1.000000000000000000, 0.8660254037844387076, 1.000000000000000000, 0.8660254037844387076, 1.000000000000000000, 0.8660254037844387076, 1.000000000000000000, 0.8660254037844387076, 1.000000000000000000, 0.8660254037844387076, 1.000000000000000000, 0.8660254037844387076, 1.000000000000000000, 0.8660254037844387076, 1.000000000000000000, 0.8660254037844387076, 1.000000000000000000, 0.8660254037844387076, 1.000000000000000000, 0.8660254037844387076, 1.000000000000000000, 0.8660254037844387076, 1.000000000000000000, 0.8660254037844387076, 1.000000000000000000, 0.8660254037844387076, 1.000000000000000000, 0.8660254037844387076, 1.000000000000000000, 0.8660254037844387076, 1.000000000000000000, 0.8660254037844387076, 1.000000000000000000, 0.8660254037844387076, 1.000000000000000000, 0.8660254037844387076, 1.000000000000000000, 0.8660254037844387076, 1.000000000000000000, 0.8660254037844387076, 1.000000000000000000, 0.8660254037844387076, 1.000000000000000000, 0.8660254037844387076, 1.000000000000000000, 0.8660254037844387076, 1.000000000000000000, 0.8660254037844387076, 1.000000000000000000, 0.8660254037844387076, 1.000000000000000000, 0.8660254037844387076, 1.000000000000000000, 0.8660254037844387076, 1.000000000000000000, 0.8660254037844387076, 1.000000000000000000, 0.8660254037844387076, 1.000000000000000000, 0.8660254037844387076, 1.000000000000000000, 0.8660254037844387076, 1.000000000000000000, 0.8660254037844387076, 1.000000000000000000, 0.8660254037844387076, 1.000000000000000000, 0.8660254037844387076, 1.000000000000000000, 0.8660254037844387076, 1.000000000000000000, 0.8660254037844387076, 1.000000000000000000, 0.8660254037844387076, 1.000000000000000000, 0.8660254037844387076, 1.000000000000000000, 0.8660254037844387076, 1.000000000000000000, 0.8660254037844387076, 1.000000000000000000, 0.8660254037844387076, 1.000000000000000000, 0.8660254037844387076, 1.000000000000000000, 0.8660254037844387076, 1.000000000000000000, 0.8660254037844387076, 1.000000000000000000, 0.8660254037844387076, 1.000000000000000000, 0.8660254037844387076, 1.000000000000000000, 0.8660254037844387076, 1.000000000000000000, 0.8660254037844387076, 1.000000000000000000, 0.8660254037844387076, 1.000000000000000000, 0.8660254037844387076, 1.000000000000000000, 0.8660254037844387076, 1.000000000000000000, 0.8660254037844387076, 1.000000000000000000, 0.8660254037844387076, 1.000000000000000000, 0.8660254037844387076, 1.000000000000000000, 0.8660254037844387076, 1.000000000000000000, 0.8660254037844387076, 1.000000000000000000, 0.8660254037844387076, 1.000000000000000000, 0.8660254037844387076, 1.000000000000000000, 0.8660254037844387076, 1.000000000000000000, 0.8660254037844387076, 1.000000000000000000, 0.8660254037844387076, 1.000000000000000000, 0.8660254037844387076, 1.000000000000000000, 0.8660254037844387076, 1.000000000000000000, 0.8660254037844387076, 1.000000000000000000, 0.8660254037844387076, 1.000000000000000000, 0.8660254037844387076, 1.000000000000000000, 0.8660254037844387076, 1.000000000000000000, 0.8660254037844387076, 1.000000000000000000, 0.8660254037844387076, 1.000000000000000000, 0.8660254037844387076, 1.000000000000000000, 0.8660254037844387076, 1.000000000000000000, 0.8660254037844387076, 1.000000000000000000, 0.8660254037844387076, 1.000000000000000000, 0.8660254037844387076, 1.000000000000000000, 0.8660254037844387076, 1.000000000000000000, 0.8660254037844387076, 1.000000000000000000, 0.8660254037844387076, 1.000000000000000000, 0.8660254037844387076, 1.000000000000000000, 0.8660254037844387076, 1.000000000000000000, 0.8660254037844387076, 1.000000000000000000, 0.8660254037844387076, 1.000000000000000000, 0.8660254037844387076, 1.000000000000000000, 0.8660254037844387076, 1.000000000000000000, 0.8660254037844387076, 1.000000000000000000, 0.8660254037844387076, 1.000000000000000000, 0.8660254037844387076, 1.000000000000000000, 0.8660254037844387076, 1.000000000000000000, 0.8660254037844387076, 1.000000000000000000, 0.8660254037844387076, 1.000000000000000000, 0.8660254037844387076, 1.000000000000000000, 0.8660254037844387076, 1.000000000000000000, 0.8660254037844387076, 1.000000000000000000, 0.8660254037844387076, 1.000000000000000000, 0.8660254037844387076, 1.000000000000000000, 0.8660254037844387076, 1.000000000000000000, 0.8660254037844387076, 1.000000000000000000, 0.8660254037844387076, 1.000000000000000000, 0.8660254037844387076, 1.000000000000000000, 0.8660254037844387076, 1.000000000000000000, 0.8660254037844387076, 1.000000000000000000, 0.8660254037844387076, 1.000000000000000000, 0.8660254037844387076, 1.000000000000000000, 0.8660254037844387076, 1.000000000000000000, 0.8660254037844387076, 1.000000000000000000, 0.8660254037844387076, 1.000000000000000000, 0.8660254037844387076, 1.000000000000000000, 0.8660254037844387076, 1.000000000000000000, 0.8660254037844387076, 1.000000000000000000, 0.8660254037844387076, 1.000000000000000000, 0.8660254037844387076, 1.000000000000000000, 0.8660254037844387076, 1.000000000000000000, 0.8660254037844387076, 1.000000000000000000, 0.8660254037844387076, 1.000000000000000000, 0.8660254037844387076, 1.000000000000000000, 0.8660254037844387076, 1.000000000000000000, 0.8660254037844387076, 1.000000000000000000, 0.8660254037844387076, 1.000000000000000000, 0.8660254037844387076, 1.000000000000000000, 0.8660254037844387076, 1.000000000000000000, 0.8660254037844387076, 1.000000000000000000, 0.8660254037844387076, 1.000000000000000000, 0.8660254037844387076, 1.000000000000000000, 0.8660254037844387076, 1.000000000000000000, 0.8660254037844387076, 1.000000000000000000, 0.8660254037844387076, 1.000000000000000000, 0.8660254037844387076, 1.000000000000000000, 0.8660254037844387076, 1.000000000000000000, 0.8660254037844387076, 1.000000000000000000, 0.8660254037844387076, 1.000000000000000000, 0.8660254037844387076, 1.000000000000000000, 0.8660254037844387076, 1.000000000000000000, 0.8660254037844387076, 1.000000000000000000, 0.8660254037844387076, 1.000000000000000000, 0.8660254037844387076, 1.000000000000000000, 0.8660254037844387076, 1.000000000000000000, 0.8660254037844387076, 1.000000000000000000, 0.8660254037844387076, 1.000000000000000000, 0.8660254037844387076, 1.000000000000000000, 0.8660254037844387076, 1.000000000000000000, 0.8660254037844387076, 1.000000000000000000, 0.8660254037844387076, 1.000000000000000000, 0.8660254037844387076, 1.000000000000000000, 0.8660254037844387076, 1.000000000000000000, 0.8660254037844387076, 1.000000000000000000, 0.8660254037844387076, 1.000000000000000000, 0.8660254037844387076, 1.000000000000000000, 0.8660254037844387076, 1.000000000000000000, 0.8660254037844387076, 1.000000000000000000, 0.8660254037844387076, 1.000000000000000000, 0.8660254037844387076, 1.000000000000000000, 0.8660254037844387076, 1.000000000000000000, 0.8660254037844387076, 1.000000000000000000, 0.8660254037844387076, 1.000000000000000000, 0.8660254037844387076, 1.000000000000000000, 0.8660254037844387076, 1.000000000000000000, 0.8660254037844387076, 1.000000000000000000, 0.8660254037844387076, 1.000000000000000000, 0.8660254037844387076, 1.000000000000000000, 0.8660254037844387076, 1.000000000000000000, 0.8660254037844387076, 1.000000000000000000, 0.8660254037844387076, 1.000000000000000000, 0.8660254037844387076, 1.000000000000000000, 0.8660254037844387076, 1.000000000000000000, 0.8660254037844387076, 1.000000000000000000, 0.8660254037844387076, 1.000000000000000000, 0.8660254037844387076, 1.000000000000000000, 0.8660254037844387076, 1.000000000000000000, 0.8660254037844387076, 1.000000000000000000, 0.8660254037844387076, 1.000000000000000000, 0.8660254037844387076, 1.000000000000000000, 0.8660254037844387076, 1.000000000000000000, 0.8660254037844387076, 1.000000000000000000, 0.8660254037844387076, 1.000000000000000000, 0.8660254037844387076, 1.000000000000000000, 0.8660254037844387076, 1.000000000000000000, 0.8660254037844387076, 1.000000000000000000, 0.8660254037844387076, 1.000000000000000000, 0.8660254037844387076, 1.000000000000000000, 0.8660254037844387076, 1.000000000000000000, 0.8660254037844387076, 1.000000000000000000, 0.8660254037844387076, 1.000000000000000000, 0.8660254037844387076, 1.000000000000000000, 0.8660254037844387076, 1.000000000000000000, 0.8660254037844387076, 1.000000000000000000, 0.8660254037844387076, 1.000000000000000000, 0.8660254037844387076, 1.000000000000000000, 0.8660254037844387076, 1.000000000000000000, 0.8660254037844387076, 1.000000000000000000, 0.8660254037844387076, 1.000000000000000000, 0.8660254037844387076, 1.000000000000000000, 0.8660254037844387076, 1.000000000000000000, 0.8660254037844387076, 1.000000000000000000, 0.8660254037844387076, 1.000000000000000000, 0.8660254037844387076, 1.000000000000000000, 0.8660254037844387076, 1.000000000000000000, 0.8660254037844387076, 1.000000000000000000, 0.8660254037844387076, 1.000000000000000000, 0.8660254037844387076, 1.000000000000000000, 0.8660254037844387076, 1.000000000000000000, 0.8660254037844387076, 1.000000000000000000, 0.8660254037844387076, 1.000000000000000000, 0.8660254037844387076, 1.000000000000000000, 0.8660254037844387076, 1.000000000000000000, 0.8660254037844387076, 1.000000000000000000, 0.8660254037844387076, 1.000000000000000000, 0.8660254037844387076, 1.000000000000000000, 0.8660254037844387076, 1.000000000000000000, 0.8660254037844387076, 1.000000000000000000, 0.8660254037844387076, 1.000000000000000000, 0.8660254037844387076, 1.000000000000000000, 0.8660254037844387076, 1.000000000000000000, 0.8660254037844387076, 1.000000000000000000, 0.8660254037844387076, 1.000000000000000000, 0.8660254037844387076, 1.000000000000000000, 0.8660254037844387076, 1.000000000000000000, 0.8660254037844387076, 1.000000000000000000, 0.8660254037844387076, 1.000000000000000000, 0.8660254037844387076, 1.000000000000000000, 0.8660254037844387076, 1.000000000000000000, 0.8660254037844387076, 1.000000000000000000, 0.8660254037844387076, 1.000000000000000000, 0.8660254037844387076, 1.000000000000000000, 0.8660254037844387076, 1.000000000000000000, 0.8660254037844387076, 1.000000000000000000, 0.8660254037844387076, 1.000000000000000000, 0.8660254037844387076, 1.000000000000000000, 0.8660254037844387076, 1.000000000000000000, 0.8660254037844387076, 1.000000000000000000, 0.8660254037844387076, 1.000000000000000000, 0.8660254037844387076, 1.000000000000000000, 0.8660254037844387076, 1.000000000000000000, 0.8660254037844387076, 1.000000000000000000, 0.8660254037844387076, 1.000000000000000000, 0.8660254037844387076, 1.000000000000000000, 0.8660254037844387076, 1.000000000000000000, 0.8660254037844387076, 1.000000000000000000, 0.8660254037844387076, 1.000000000000000000, 0.8660254037844387076, 1.000000000000000000, 0.8660254037844387076, 1.000000000000000000, 0.8660254037844387076, 1.000000000000000000, 0.8660254037844387076, 1.000000000000000000, 0.8660254037844387076, 1.000000000000000000, 0.8660254037844387076, 1.000000000000000000, 0.8660254037844387076, 1.000000000000000000, 0.8660254037844387076, 1.000000000000000000, 0.8660254037844387076, 1.000000000000000000, 0.8660254037844387076, 1.000000000000000000, 0.8660254037844387076, 1.000000000000000000, 0.8660254037844387076, 1.000000000000000000, 0.8660254037844387076, 1.000000000000000000, 0.8660254037844387076, 1.000000000000000000, 0.8660254037844387076, 1.000000000000000000, 0.8660254037844387076, 1.000000000000000000, 0.8660254037844387076, 1.000000000000000000, 0.8660254037844387076, 1.000000000000000000, 0.8660254037844387076, 1.000000000000000000, 0.8660254037844387076, 1.000000000000000000, 0.8660254037844387076, 1.000000000000000000, 0.8660254037844387076, 1.000000000000000000, 0.8660254037844387076, 1.000000000000000000, 0.8660254037844387076, 1.000000000000000000, 0.8660254037844387076, 1.000000000000000000, 0.8660254037844387076, 1.000000000000000000, 0.8660254037844387076, 1.000000000000000000, 0.8660254037844387076, 1.000000000000000000, 0.8660254037844387076, 1.000000000000000000, 0.8660254037844387076, 1.000000000000000000, 0.8660254037844387076, 1.000000000000000000, 0.8660254037844387076, 1.000000000000000000, 0.8660254037844387076, 1.000000000000000000, 0.8660254037844387076, 1.000000000000000000, 0.8660254037844387076, 1.000000000000000000, 0.8660254037844387076, 1.000000000000000000, 0.8660254037844387076, 1.000000000000000000, 0.8660254037844387076, 1.000000000000000000, 0.8660254037844387076, 1.000000000000000000, 0.8660254037844387076, 1.000000000000000000, 0.8660254037844387076, 1.000000000000000000, 0.8660254037844387076, 1.000000000000000000, 0.8660254037844387076, 1.000000000000000000, 0.8660254037844387076, 1.000000000000000000, 0.8660254037844387076, 1.000000000000000000, 0.8660254037844387076, 1.000000000000000000, 0.8660254037844387076, 1.000000000000000000, 0.8660254037844387076, 1.000000000000000000, 0.8660254037844387076, 1.000000000000000000, 0.8660254037844387076, 1.000000000000000000, 0.8660254037844387076, 1.000000000000000000, 0.8660254037844387076, 1.000000000000000000, 0.8660254037844387076, 1.000000000000000000, 0.8660254037844387076, 1.000000000000000000, 0.8660254037844387076, 1.000000000000000000, 0.8660254037844387076, 1.000000000000000000, 0.8660254037844387076, 1.000000000000000000, 0.8660254037844387076, 1.000000000000000000, 0.8660254037844387076, 1.000000000000000000, 0.8660254037844387076, 1.000000000000000000, 0.8660254037844387076, 1.000000000000000000, 0.8660254037844387076, 1.000000000000000000, 0.8660254037844387076, 1.000000000000000000, 0.8660254037844387076, 1.000000000000000000, 0.8660254037844387076, 1.000000000000000000, 0.8660254037844387076, 1.000000000000000000, 0.8660254037844387076, 1.000000000000000000, 0.8660254037844387076, 1.000000000000000000, 0.8660254037844387076, 1.000000000000000000, 0.8660254037844387076, 1.000000000000000000, 0.8660254037844387076, 1.000000000000000000, 0.8660254037844387076, 1.000000000000000000, 0.8660254037844387076, 1.000000000000000000, 0.8660254037844387076, 1.000000000000000000, 0.8660254037844387076, 1.000000000000000000, 0.8660254037844387076, 1.000000000000000000, 0.8660254037844387076, 1.000000000000000000, 0.8660254037844387076, 1.000000000000000000, 0.8660254037844387076, 1.000000000000000000, 0.8660254037844387076, 1.000000000000000000, 0.8660254037844387076, 1.000000000000000000, 0.8660254037844387076, 1.000000000000000000, 0.8660254037844387076, 1.000000000000000000, 0.8660254037844387076, 1.000000000000000000, 0.8660254037844387076, 1.000000000000000000, 0.8660254037844387076, 1.000000000000000000, 0.8660254037844387076, 1.000000000000000000, 0.8660254037844387076, 1.000000000000000000, 0.8660254037844387076, 1.000000000000000000, 0.8660254037844387076, 1.000000000000000000, 0.8660254037844387076, 1.000000000000000000, 0.8660254037844387076, 1.000000000000000000, 0.8660254037844387076, 1.000000000000000000, 0.8660254037844387076, 1.000000000000000000, 0.8660254037844387076, 1.000000000000000000, 0.8660254037844387076, 1.000000000000000000, 0.8660254037844387076, 1.000000000000000000, 0.8660254037844387076, 1.000000000000000000, 0.8660254037844387076, 1.000000000000000000, 0.8660254037844387076, 1.000000000000000000, 0.8660254037844387076, 1.000000000000000000, 0.8660254037844387076, 1.000000000000000000, 0.8660254037844387076, 1.000000000000000000, 0.8660254037844387076, 1.000000000000000000, 0.8660254037844387076, 1.000000000000000000, 0.8660254037844387076, 1.000000000000000000, 0.8660254037844387076, 1.000000000000000000, 0.8660254037844387076, 1.000000000000000000, 0.8660254037844387076, 1.000000000000000000, 0.8660254037844387076, 1.000000000000000000, 0.8660254037844387076, 1.000000000000000000, 0.8660254037844387076, 1.000000000000000000, 0.8660254037844387076, 1.000000000000000000, 0.8660254037844387076, 1.000000000000000000, 0.8660254037844387076, 1.000000000000000000, 0.8660254037844387076, 1.000000000000000000, 0.8660254037844387076, 1.000000000000000000, 0.8660254037844387076, 1.000000000000000000, 0.8660254037844387076, 1.000000000000000000, 0.8660254037844387076, 1.000000000000000000, 0.8660254037844387076, 1.000000000000000000, 0.8660254037844387076, 1.000000000000000000, 0.8660254037844387076, 1.000000000000000000, 0.8660254037844387076, 1.000000000000000000, 0.8660254037844387076, 1.000000000000000000, 0.8660254037844387076, 1.000000000000000000, 0.8660254037844387076, 1.000000000000000000, 0.8660254037844387076, 1.000000000000000000, 0.8660254037844387076, 1.000000000000000000, 0.8660254037844387076, 1.000000000000000000, 0.8660254037844387076, 1.000000000000000000, 0.8660254037844387076, 1.000000000000000000, 0.8660254037844387076, 1.000000000000000000, 0.8660254037844387076, 1.000000000000000000, 0.8660254037844387076, 1.000000000000000000, 0.8660254037844387076, 1.000000000000000000, 0.8660254037844387076, 1.000000000000000000, 0.8660254037844387076, 1.000000000000000000, 0.8660254037844387076, 1.000000000000000000, 0.8660254037844387076, 1.000000000000000000, 0.8660254037844387076, 1.000000000000000000, 0.8660254037844387076, 1.000000000000000000, 0.8660254037844387076, 1.000000000000000000, 0.8660254037844387076, 1.000000000000000000, 0.8660254037844387076, 1.000000000000000000, 0.8660254037844387076, 1.000000000000000000, 0.8660254037844387076, 1.000000000000000000, 0.8660254037844387076, 1.000000000000000000, 0.8660254037844387076, 1.000000000000000000, 0.8660254037844387076, 1.000000000000000000, 0.8660254037844387076, 1.000000000000000000, 0.8660254037844387076, 1.000000000000000000, 0.8660254037844387076, 1.000000000000000000, 0.8660254037844387076, 1.000000000000000000, 0.8660254037844387076, 1.000000000000000000, 0.8660254037844387076, 1.000000000000000000, 0.8660254037844387076, 1.000000000000000000, 0.8660254037844387076, 1.000000000000000000, 0.8660254037844387076, 1.000000000000000000, 0.8660254037844387076, 1.000000000000000000, 0.8660254037844387076, 1.000000000000000000, 0.8660254037844387076, 1.000000000000000000, 0.8660254037844387076, 1.000000000000000000, 0.8660254037844387076, 1.000000000000000000, 0.8660254037844387076, 1.000000000000000000, 0.8660254037844387076, 1.000000000000000000, 0.8660254037844387076, 1.000000000000000000, 0.8660254037844387076, 1.000000000000000000, 0.8660254037844387076, 1.000000000000000000, 0.8660254037844387076, 1.000000000000000000, 0.8660254037844387076, 1.000000000000000000, 0.8660254037844387076, 1.000000000000000000, 0.8660254037844387076, 1.000000000000000000, 0.8660254037844387076, 1.000000000000000000, 0.8660254037844387076, 1.000000000000000000, 0.8660254037844387076, 1.000000000000000000, 0.8660254037844387076, 1.000000000000000000, 0.8660254037844387076, 1.000000000000000000, 0.8660254037844387076, 1.000000000000000000, 0.8660254037844387076, 1.000000000000000000, 0.8660254037844387076, 1.000000000000000000, 0.8660254037844387076, 1.000000000000000000, 0.8660254037844387076, 1.000000000000000000, 0.8660254037844387076, 1.000000000000000000, 0.8660254037844387076, 1.000000000000000000, 0.8660254037844387076, 1.000000000000000000, 0.8660254037844387076, 1.000000000000000000, 0.8660254037844387076, 1.000000000000000000, 0.8660254037844387076, 1.000000000000000000, 0.8660254037844387076, 1.000000000000000000, 0.8660254037844387076, 1.000000000000000000, 0.8660254037844387076, 1.000000000000000000, 0.8660254037844387076, 1.000000000000000000, 0.8660254037844387076, 1.000000000000000000, 0.8660254037844387076, 1.000000000000000000, 0.8660254037844387076, 1.000000000000000000, 0.8660254037844387076, 1.000000000000000000, 0.8660254037844387076, 1.000000000000000000, 0.8660254037844387076, 1.000000000000000000, 0.8660254037844387076, 1.000000000000000000, 0.8660254037844387076, 1.000000000000000000, 0.8660254037844387076, 1.000000000000000000, 0.8660254037844387076, 1.000000000000000000, 0.8660254037844387076, 1.000000000000000000, 0.8660254037844387076, 1.000000000000000000, 0.8660254037844387076, 1.000000000000000000, 0.8660254037844387076, 1.000000000000000000, 0.8660254037844387076, 1.000000000000000000, 0.8660254037844387076, 1.000000000000000000, 0.8660254037844387076, 1.000000000000000000, 0.8660254037844387076, 1.000000000000000000, 0.8660254037844387076, 1.000000000000000000, 0.8660254037844387076, 1.000000000000000000, 0.8660254037844387076, 1.000000000000000000, 0.8660254037844387076, 1.000000000000000000, 0.8660254037844387076, 1.000000000000000000, 0.8660254037844387076, 1.000000000000000000, 0.8660254037844387076, 1.000000000000000000, 0.8660254037844387076, 1.000000000000000000, 0.8660254037844387076, 1.000000000000000000, 0.8660254037844387076, 1.000000000000000000, 0.8660254037844387076, 1.000000000000000000, 0.8660254037844387076, 1.000000000000000000, 0.8660254037844387076, 1.000000000000000000, 0.8660254037844387076, 1.000000000000000000, 0.8660254037844387076, 1.000000000000000000, 0.8660254037844387076, 1.000000000000000000, 0.8660254037844387076, 1.000000000000000000, 0.8660254037844387076, 1.000000000000000000, 0.8660254037844387076, 1.000000000000000000, 0.8660254037844387076, 1.000000000000000000, 0.8660254037844387076, 1.000000000000000000, 0.8660254037844387076, 1.000000000000000000, 0.8660254037844387076, 1.000000000000000000, 0.8660254037844387076, 1.000000000000000000, 0.8660254037844387076, 1.000000000000000000, 0.8660254037844387076, 1.000000000000000000, 0.8660254037844387076, 1.000000000000000000, 0.8660254037844387076, 1.000000000000000000, 0.8660254037844387076, 1.000000000000000000, 0.8660254037844387076, 1.000000000000000000, 0.8660254037844387076, 1.000000000000000000, 0.8660254037844387076, 1.000000000000000000),
 ( 1.000000000000000000, 0.8660254037844387076, 1.000000000000000000, 0.8660254037844387076, 1.000000000000000000, 0.8660254037844387076, 1.000000000000000000, 0.8660254037844387076, 1.000000000000000000, 0.8660254037844387076, 1.000000000000000000, 0.8660254037844387076, 1.000000000000000000, 0.8660254037844387076, 1.000000000000000000, 0.8660254037844387076, 1.000000000000000000, 0.8660254037844387076, 1.000000000000000000, 0.8660254037844387076, 1.000000000000000000, 0.8660254037844387076, 1.000000000000000000, 0.8660254037844387076, 1.000000000000000000, 0.8660254037844387076, 1.000000000000000000, 0.8660254037844387076, 1.000000000000000000, 0.8660254037844387076, 1.000000000000000000, 0.8660254037844387076, 1.000000000000000000, 0.8660254037844387076, 1.000000000000000000, 0.8660254037844387076, 1.000000000000000000, 0.8660254037844387076, 1.000000000000000000, 0.8660254037844387076, 1.000000000000000000, 0.8660254037844387076, 1.000000000000000000, 0.8660254037844387076, 1.000000000000000000, 0.8660254037844387076, 1.000000000000000000, 0.8660254037844387076, 1.000000000000000000, 0.8660254037844387076, 1.000000000000000000, 0.8660254037844387076, 1.000000000000000000, 0.8660254037844387076, 1.000000000000000000, 0.8660254037844387076, 1.000000000000000000, 0.8660254037844387076, 1.000000000000000000, 0.8660254037844387076, 1.000000000000000000, 0.8660254037844387076, 1.000000000000000000, 0.8660254037844387076, 1.000000000000000000, 0.8660254037844387076, 1.000000000000000000, 0.8660254037844387076, 1.000000000000000000, 0.8660254037844387076, 1.000000000000000000, 0.8660254037844387076, 1.000000000000000000, 0.8660254037844387076, 1.000000000000000000, 0.8660254037844387076, 1.000000000000000000, 0.8660254037844387076, 1.000000000000000000, 0.8660254037844387076, 1.000000000000000000, 0.8660254037844387076, 1.000000000000000000, 0.8660254037844387076, 1.000000000000000000, 0.8660254037844387076, 1.000000000000000000, 0.8660254037844387076, 1.000000000000000000, 0.8660254037844387076, 1.000000000000000000, 0.8660254037844387076, 1.000000000000000000, 0.8660254037844387076, 1.000000000000000000, 0.8660254037844387076, 1.000000000000000000, 0.8660254037844387076, 1.000000000000000000, 0.8660254037844387076, 1.000000000000000000, 0.8660254037844387076, 1.000000000000000000, 0.8660254037844387076, 1.000000000000000000, 0.8660254037844387076, 1.000000000000000000, 0.8660254037844387076, 1.000000000000000000, 0.8660254037844387076, 1.000000000000000000, 0.8660254037844387076, 1.000000000000000000, 0.8660254037844387076, 1.000000000000000000, 0.8660254037844387076, 1.000000000000000000, 0.8660254037844387076, 1.000000000000000000, 0.8660254037844387076, 1.000000000000000000, 0.8660254037844387076, 1.000000000000000000, 0.8660254037844387076, 1.000000000000000000, 0.8660254037844387076, 1.000000000000000000, 0.8660254037844387076, 1.000000000000000000, 0.8660254037844387076, 1.000000000000000000, 0.8660254037844387076, 1.000000000000000000, 0.8660254037844387076, 1.000000000000000000, 0.8660254037844387076, 1.000000000000000000, 0.8660254037844387076, 1.000000000000000000, 0.8660254037844387076, 1.000000000000000000, 0.8660254037844387076, 1.000000000000000000, 0.8660254037844387076, 1.000000000000000000, 0.8660254037844387076, 1.000000000000000000, 0.8660254037844387076, 1.000000000000000000, 0.8660254037844387076, 1.000000000000000000, 0.8660254037844387076, 1.000000000000000000, 0.8660254037844387076, 1.000000000000000000, 0.8660254037844387076, 1.000000000000000000, 0.8660254037844387076, 1.000000000000000000, 0.8660254037844387076, 1.000000000000000000, 0.8660254037844387076, 1.000000000000000000, 0.8660254037844387076, 1.000000000000000000, 0.8660254037844387076, 1.000000000000000000, 0.8660254037844387076, 1.000000000000000000, 0.8660254037844387076, 1.000000000000000000, 0.8660254037844387076, 1.000000000000000000, 0.8660254037844387076, 1.000000000000000000, 0.8660254037844387076, 1.000000000000000000, 0.8660254037844387076, 1.000000000000000000, 0.8660254037844387076, 1.000000000000000000, 0.8660254037844387076, 1.000000000000000000, 0.8660254037844387076, 1.000000000000000000, 0.8660254037844387076, 1.000000000000000000, 0.8660254037844387076, 1.000000000000000000, 0.8660254037844387076, 1.000000000000000000, 0.8660254037844387076, 1.000000000000000000, 0.8660254037844387076, 1.000000000000000000, 0.8660254037844387076, 1.000000000000000000, 0.8660254037844387076, 1.000000000000000000, 0.8660254037844387076, 1.000000000000000000, 0.8660254037844387076, 1.000000000000000000, 0.8660254037844387076, 1.000000000000000000, 0.8660254037844387076, 1.000000000000000000, 0.8660254037844387076, 1.000000000000000000, 0.8660254037844387076, 1.000000000000000000, 0.8660254037844387076, 1.000000000000000000, 0.8660254037844387076, 1.000000000000000000, 0.8660254037844387076, 1.000000000000000000, 0.8660254037844387076, 1.000000000000000000, 0.8660254037844387076, 1.000000000000000000, 0.8660254037844387076, 1.000000000000000000, 0.8660254037844387076, 1.000000000000000000, 0.8660254037844387076, 1.000000000000000000, 0.8660254037844387076, 1.000000000000000000, 0.8660254037844387076, 1.000000000000000000, 0.8660254037844387076, 1.000000000000000000, 0.8660254037844387076, 1.000000000000000000, 0.8660254037844387076, 1.000000000000000000, 0.8660254037844387076, 1.000000000000000000, 0.8660254037844387076, 1.000000000000000000, 0.8660254037844387076, 1.000000000000000000, 0.8660254037844387076, 1.000000000000000000, 0.8660254037844387076, 1.000000000000000000, 0.8660254037844387076, 1.000000000000000000, 0.8660254037844387076, 1.000000000000000000, 0.8660254037844387076, 1.000000000000000000, 0.8660254037844387076, 1.000000000000000000, 0.8660254037844387076, 1.000000000000000000, 0.8660254037844387076, 1.000000000000000000, 0.8660254037844387076, 1.000000000000000000, 0.8660254037844387076, 1.000000000000000000, 0.8660254037844387076, 1.000000000000000000, 0.8660254037844387076, 1.000000000000000000, 0.8660254037844387076, 1.000000000000000000, 0.8660254037844387076, 1.000000000000000000, 0.8660254037844387076, 1.000000000000000000, 0.8660254037844387076, 1.000000000000000000, 0.8660254037844387076, 1.000000000000000000, 0.8660254037844387076, 1.000000000000000000, 0.8660254037844387076, 1.000000000000000000, 0.8660254037844387076, 1.000000000000000000, 0.8660254037844387076, 1.000000000000000000, 0.8660254037844387076, 1.000000000000000000, 0.8660254037844387076, 1.000000000000000000, 0.8660254037844387076, 1.000000000000000000, 0.8660254037844387076, 1.000000000000000000, 0.8660254037844387076, 1.000000000000000000, 0.8660254037844387076, 1.000000000000000000, 0.8660254037844387076, 1.000000000000000000, 0.8660254037844387076, 1.000000000000000000, 0.8660254037844387076, 1.000000000000000000, 0.8660254037844387076, 1.000000000000000000, 0.8660254037844387076, 1.000000000000000000, 0.8660254037844387076, 1.000000000000000000, 0.8660254037844387076, 1.000000000000000000, 0.8660254037844387076, 1.000000000000000000, 0.8660254037844387076, 1.000000000000000000, 0.8660254037844387076, 1.000000000000000000, 0.8660254037844387076, 1.000000000000000000, 0.8660254037844387076, 1.000000000000000000, 0.8660254037844387076, 1.000000000000000000, 0.8660254037844387076, 1.000000000000000000, 0.8660254037844387076, 1.000000000000000000, 0.8660254037844387076, 1.000000000000000000, 0.8660254037844387076, 1.000000000000000000, 0.8660254037844387076, 1.000000000000000000, 0.8660254037844387076, 1.000000000000000000, 0.8660254037844387076, 1.000000000000000000, 0.8660254037844387076, 1.000000000000000000, 0.8660254037844387076, 1.000000000000000000, 0.8660254037844387076, 1.000000000000000000, 0.8660254037844387076, 1.000000000000000000, 0.8660254037844387076, 1.000000000000000000, 0.8660254037844387076, 1.000000000000000000, 0.8660254037844387076, 1.000000000000000000, 0.8660254037844387076, 1.000000000000000000, 0.8660254037844387076, 1.000000000000000000, 0.8660254037844387076, 1.000000000000000000, 0.8660254037844387076, 1.000000000000000000, 0.8660254037844387076, 1.000000000000000000, 0.8660254037844387076, 1.000000000000000000, 0.8660254037844387076, 1.000000000000000000, 0.8660254037844387076, 1.000000000000000000, 0.8660254037844387076, 1.000000000000000000, 0.8660254037844387076, 1.000000000000000000, 0.8660254037844387076, 1.000000000000000000, 0.8660254037844387076, 1.000000000000000000, 0.8660254037844387076, 1.000000000000000000, 0.8660254037844387076, 1.000000000000000000, 0.8660254037844387076, 1.000000000000000000, 0.8660254037844387076, 1.000000000000000000, 0.8660254037844387076, 1.000000000000000000, 0.8660254037844387076, 1.000000000000000000, 0.8660254037844387076, 1.000000000000000000, 0.8660254037844387076, 1.000000000000000000, 0.8660254037844387076, 1.000000000000000000, 0.8660254037844387076, 1.000000000000000000, 0.8660254037844387076, 1.000000000000000000, 0.8660254037844387076, 1.000000000000000000, 0.8660254037844387076, 1.000000000000000000, 0.8660254037844387076, 1.000000000000000000, 0.8660254037844387076, 1.000000000000000000, 0.8660254037844387076, 1.000000000000000000, 0.8660254037844387076, 1.000000000000000000, 0.8660254037844387076, 1.000000000000000000, 0.8660254037844387076, 1.000000000000000000, 0.8660254037844387076, 1.000000000000000000, 0.8660254037844387076, 1.000000000000000000, 0.8660254037844387076, 1.000000000000000000, 0.8660254037844387076, 1.000000000000000000, 0.8660254037844387076, 1.000000000000000000, 0.8660254037844387076, 1.000000000000000000, 0.8660254037844387076, 1.000000000000000000, 0.8660254037844387076, 1.000000000000000000, 0.8660254037844387076, 1.000000000000000000, 0.8660254037844387076, 1.000000000000000000, 0.8660254037844387076, 1.000000000000000000, 0.8660254037844387076, 1.000000000000000000, 0.8660254037844387076, 1.000000000000000000, 0.8660254037844387076, 1.000000000000000000, 0.8660254037844387076, 1.000000000000000000, 0.8660254037844387076, 1.000000000000000000, 0.8660254037844387076, 1.000000000000000000, 0.8660254037844387076, 1.000000000000000000, 0.8660254037844387076, 1.000000000000000000, 0.8660254037844387076, 1.000000000000000000, 0.8660254037844387076, 1.000000000000000000, 0.8660254037844387076, 1.000000000000000000, 0.8660254037844387076, 1.000000000000000000, 0.8660254037844387076, 1.000000000000000000, 0.8660254037844387076, 1.000000000000000000, 0.8660254037844387076, 1.000000000000000000, 0.8660254037844387076, 1.000000000000000000, 0.8660254037844387076, 1.000000000000000000, 0.8660254037844387076, 1.000000000000000000, 0.8660254037844387076, 1.000000000000000000, 0.8660254037844387076, 1.000000000000000000, 0.8660254037844387076, 1.000000000000000000, 0.8660254037844387076, 1.000000000000000000, 0.8660254037844387076, 1.000000000000000000, 0.8660254037844387076, 1.000000000000000000, 0.8660254037844387076, 1.000000000000000000, 0.8660254037844387076, 1.000000000000000000, 0.8660254037844387076, 1.000000000000000000, 0.8660254037844387076, 1.000000000000000000, 0.8660254037844387076, 1.000000000000000000, 0.8660254037844387076, 1.000000000000000000, 0.8660254037844387076, 1.000000000000000000, 0.8660254037844387076, 1.000000000000000000, 0.8660254037844387076, 1.000000000000000000, 0.8660254037844387076, 1.000000000000000000, 0.8660254037844387076, 1.000000000000000000, 0.8660254037844387076, 1.000000000000000000, 0.8660254037844387076, 1.000000000000000000, 0.8660254037844387076, 1.000000000000000000, 0.8660254037844387076, 1.000000000000000000, 0.8660254037844387076, 1.000000000000000000, 0.8660254037844387076, 1.000000000000000000, 0.8660254037844387076, 1.000000000000000000, 0.8660254037844387076, 1.000000000000000000, 0.8660254037844387076, 1.000000000000000000, 0.8660254037844387076, 1.000000000000000000, 0.8660254037844387076, 1.000000000000000000, 0.8660254037844387076, 1.000000000000000000, 0.8660254037844387076, 1.000000000000000000, 0.8660254037844387076, 1.000000000000000000, 0.8660254037844387076, 1.000000000000000000, 0.8660254037844387076, 1.000000000000000000, 0.8660254037844387076, 1.000000000000000000, 0.8660254037844387076, 1.000000000000000000, 0.8660254037844387076, 1.000000000000000000, 0.8660254037844387076, 1.000000000000000000, 0.8660254037844387076, 1.000000000000000000, 0.8660254037844387076, 1.000000000000000000, 0.8660254037844387076, 1.000000000000000000, 0.8660254037844387076, 1.000000000000000000, 0.8660254037844387076, 1.000000000000000000, 0.8660254037844387076, 1.000000000000000000, 0.8660254037844387076, 1.000000000000000000, 0.8660254037844387076, 1.000000000000000000, 0.8660254037844387076, 1.000000000000000000, 0.8660254037844387076, 1.000000000000000000, 0.8660254037844387076, 1.000000000000000000, 0.8660254037844387076, 1.000000000000000000, 0.8660254037844387076, 1.000000000000000000, 0.8660254037844387076, 1.000000000000000000, 0.8660254037844387076, 1.000000000000000000, 0.8660254037844387076, 1.000000000000000000, 0.8660254037844387076, 1.000000000000000000, 0.8660254037844387076, 1.000000000000000000, 0.8660254037844387076, 1.000000000000000000, 0.8660254037844387076, 1.000000000000000000, 0.8660254037844387076, 1.000000000000000000, 0.8660254037844387076, 1.000000000000000000, 0.8660254037844387076, 1.000000000000000000, 0.8660254037844387076, 1.000000000000000000, 0.8660254037844387076, 1.000000000000000000, 0.8660254037844387076, 1.000000000000000000, 0.8660254037844387076, 1.000000000000000000, 0.8660254037844387076, 1.000000000000000000, 0.8660254037844387076, 1.000000000000000000, 0.8660254037844387076, 1.000000000000000000, 0.8660254037844387076, 1.000000000000000000, 0.8660254037844387076, 1.000000000000000000, 0.8660254037844387076, 1.000000000000000000, 0.8660254037844387076, 1.000000000000000000, 0.8660254037844387076, 1.000000000000000000, 0.8660254037844387076, 1.000000000000000000, 0.8660254037844387076, 1.000000000000000000, 0.8660254037844387076, 1.000000000000000000, 0.8660254037844387076, 1.000000000000000000, 0.8660254037844387076, 1.000000000000000000, 0.8660254037844387076, 1.000000000000000000, 0.8660254037844387076, 1.000000000000000000, 0.8660254037844387076, 1.000000000000000000, 0.8660254037844387076, 1.000000000000000000, 0.8660254037844387076, 1.000000000000000000, 0.8660254037844387076, 1.000000000000000000, 0.8660254037844387076, 1.000000000000000000, 0.8660254037844387076, 1.000000000000000000, 0.8660254037844387076, 1.000000000000000000, 0.8660254037844387076, 1.000000000000000000, 0.8660254037844387076, 1.000000000000000000, 0.8660254037844387076, 1.000000000000000000, 0.8660254037844387076, 1.000000000000000000, 0.8660254037844387076, 1.000000000000000000, 0.8660254037844387076, 1.000000000000000000, 0.8660254037844387076, 1.000000000000000000, 0.8660254037844387076, 1.000000000000000000, 0.8660254037844387076, 1.000000000000000000, 0.8660254037844387076, 1.000000000000000000, 0.8660254037844387076, 1.000000000000000000, 0.8660254037844387076, 1.000000000000000000, 0.8660254037844387076, 1.000000000000000000, 0.8660254037844387076, 1.000000000000000000, 0.8660254037844387076, 1.000000000000000000, 0.8660254037844387076, 1.000000000000000000, 0.8660254037844387076, 1.000000000000000000, 0.8660254037844387076, 1.000000000000000000, 0.8660254037844387076, 1.000000000000000000, 0.8660254037844387076, 1.000000000000000000, 0.8660254037844387076, 1.000000000000000000, 0.8660254037844387076, 1.000000000000000000, 0.8660254037844387076, 1.000000000000000000, 0.8660254037844387076, 1.000000000000000000, 0.8660254037844387076, 1.000000000000000000, 0.8660254037844387076, 1.000000000000000000, 0.8660254037844387076, 1.000000000000000000, 0.8660254037844387076, 1.000000000000000000, 0.8660254037844387076, 1.000000000000000000, 0.8660254037844387076, 1.000000000000000000, 0.8660254037844387076, 1.000000000000000000, 0.8660254037844387076, 1.000000000000000000, 0.8660254037844387076, 1.000000000000000000, 0.8660254037844387076, 1.000000000000000000, 0.8660254037844387076, 1.000000000000000000, 0.8660254037844387076, 1.000000000000000000, 0.8660254037844387076, 1.000000000000000000, 0.8660254037844387076, 1.000000000000000000, 0.8660254037844387076, 1.000000000000000000, 0.8660254037844387076, 1.000000000000000000, 0.8660254037844387076, 1.000000000000000000, 0.8660254037844387076, 1.000000000000000000, 0.8660254037844387076, 1.000000000000000000, 0.8660254037844387076, 1.000000000000000000, 0.8660254037844387076, 1.000000000000000000, 0.8660254037844387076, 1.000000000000000000, 0.8660254037844387076, 1.000000000000000000, 0.8660254037844387076, 1.000000000000000000, 0.8660254037844387076, 1.000000000000000000, 0.8660254037844387076, 1.000000000000000000, 0.8660254037844387076, 1.000000000000000000, 0.8660254037844387076, 1.000000000000000000, 0.8660254037844387076, 1.000000000000000000, 0.8660254037844387076, 1.000000000000000000, 0.8660254037844387076, 1.000000000000000000, 0.8660254037844387076, 1.000000000000000000, 0.8660254037844387076, 1.000000000000000000, 0.8660254037844387076, 1.000000000000000000, 0.8660254037844387076, 1.000000000000000000, 0.8660254037844387076, 1.000000000000000000, 0.8660254037844387076, 1.000000000000000000, 0.8660254037844387076, 1.000000000000000000, 0.8660254037844387076, 1.000000000000000000, 0.8660254037844387076, 1.000000000000000000, 0.8660254037844387076, 1.000000000000000000, 0.8660254037844387076, 1.000000000000000000, 0.8660254037844387076, 1.000000000000000000, 0.8660254037844387076, 1.000000000000000000, 0.8660254037844387076, 1.000000000000000000, 0.8660254037844387076, 1.000000000000000000, 0.8660254037844387076, 1.000000000000000000, 0.8660254037844387076, 1.000000000000000000, 0.8660254037844387076, 1.000000000000000000, 0.8660254037844387076, 1.000000000000000000, 0.8660254037844387076, 1.000000000000000000, 0.8660254037844387076, 1.000000000000000000, 0.8660254037844387076, 1.000000000000000000, 0.8660254037844387076, 1.000000000000000000, 0.8660254037844387076, 1.000000000000000000, 0.8660254037844387076, 1.000000000000000000, 0.8660254037844387076, 1.000000000000000000, 0.8660254037844387076, 1.000000000000000000, 0.8660254037844387076, 1.000000000000000000, 0.8660254037844387076, 1.000000000000000000, 0.8660254037844387076, 1.000000000000000000, 0.8660254037844387076, 1.000000000000000000, 0.8660254037844387076, 1.000000000000000000, 0.8660254037844387076, 1.000000000000000000, 0.8660254037844387076, 1.000000000000000000, 0.8660254037844387076, 1.000000000000000000, 0.8660254037844387076, 1.000000000000000000, 0.8660254037844387076, 1.000000000000000000, 0.8660254037844387076, 1.000000000000000000, 0.8660254037844387076, 1.000000000000000000, 0.8660254037844387076, 1.000000000000000000, 0.8660254037844387076, 1.000000000000000000, 0.8660254037844387076, 1.000000000000000000, 0.8660254037844387076, 1.000000000000000000, 0.8660254037844387076, 1.000000000000000000, 0.8660254037844387076, 1.000000000000000000, 0.8660254037844387076, 1.000000000000000000, 0.8660254037844387076, 1.000000000000000000, 0.8660254037844387076, 1.000000000000000000, 0.8660254037844387076, 1.000000000000000000, 0.8660254037844387076, 1.000000000000000000, 0.8660254037844387076, 1.000000000000000000, 0.8660254037844387076, 1.000000000000000000, 0.8660254037844387076, 1.000000000000000000, 0.8660254037844387076, 1.000000000000000000, 0.8660254037844387076, 1.000000000000000000, 0.8660254037844387076, 1.000000000000000000, 0.8660254037844387076, 1.000000000000000000, 0.8660254037844387076, 1.000000000000000000, 0.8660254037844387076, 1.000000000000000000, 0.8660254037844387076, 1.000000000000000000, 0.8660254037844387076, 1.000000000000000000, 0.8660254037844387076, 1.000000000000000000, 0.8660254037844387076, 1.000000000000000000, 0.8660254037844387076, 1.000000000000000000, 0.8660254037844387076, 1.000000000000000000, 0.8660254037844387076, 1.000000000000000000, 0.8660254037844387076, 1.000000000000000000, 0.8660254037844387076, 1.000000000000000000, 0.8660254037844387076, 1.000000000000000000, 0.8660254037844387076, 1.000000000000000000, 0.8660254037844387076, 1.000000000000000000, 0.8660254037844387076, 1.000000000000000000, 0.8660254037844387076, 1.000000000000000000, 0.8660254037844387076, 1.000000000000000000, 0.8660254037844387076, 1.000000000000000000, 0.8660254037844387076, 1.000000000000000000, 0.8660254037844387076, 1.000000000000000000, 0.8660254037844387076, 1.000000000000000000, 0.8660254037844387076, 1.000000000000000000, 0.8660254037844387076, 1.000000000000000000, 0.8660254037844387076, 1.000000000000000000, 0.8660254037844387076, 1.000000000000000000, 0.8660254037844387076, 1.000000000000000000, 0.8660254037844387076, 1.000000000000000000, 0.8660254037844387076, 1.000000000000000000, 0.8660254037844387076, 1.000000000000000000, 0.8660254037844387076, 1.000000000000000000, 0.8660254037844387076, 1.000000000000000000, 0.8660254037844387076, 1.000000000000000000, 0.8660254037844387076, 1.000000000000000000, 0.8660254037844387076, 1.000000000000000000, 0.8660254037844387076, 1.000000000000000000, 0.8660254037844387076, 1.000000000000000000, 0.8660254037844387076, 1.000000000000000000, 0.8660254037844387076, 1.000000000000000000, 0.8660254037844387076, 1.000000000000000000, 0.8660254037844387076, 1.000000000000000000, 0.8660254037844387076, 1.000000000000000000, 0.8660254037844387076, 1.000000000000000000, 0.8660254037844387076, 1.000000000000000000, 0.8660254037844387076, 1.000000000000000000, 0.8660254037844387076, 1.000000000000000000, 0.8660254037844387076, 1.000000000000000000, 0.8660254037844387076, 1.000000000000000000, 0.8660254037844387076, 1.000000000000000000, 0.8660254037844387076, 1.000000000000000000, 0.8660254037844387076, 1.000000000000000000, 0.8660254037844387076, 1.000000000000000000, 0.8660254037844387076, 1.000000000000000000, 0.8660254037844387076, 1.000000000000000000, 0.8660254037844387076, 1.000000000000000000, 0.8660254037844387076, 1.000000000000000000, 0.8660254037844387076, 1.000000000000000000, 0.8660254037844387076, 1.000000000000000000, 0.8660254037844387076, 1.000000000000000000, 0.8660254037844387076, 1.000000000000000000, 0.8660254037844387076, 1.000000000000000000, 0.8660254037844387076, 1.000000000000000000, 0.8660254037844387076, 1.000000000000000000, 0.8660254037844387076, 1.000000000000000000, 0.8660254037844387076, 1.000000000000000000, 0.8660254037844387076, 1.000000000000000000, 0.8660254037844387076, 1.000000000000000000, 0.8660254037844387076, 1.000000000000000000, 0.8660254037844387076, 1.000000000000000000, 0.8660254037844387076, 1.000000000000000000, 0.8660254037844387076, 1.000000000000000000, 0.8660254037844387076, 1.000000000000000000, 0.8660254037844387076, 1.000000000000000000, 0.8660254037844387076, 1.000000000000000000, 0.8660254037844387076, 1.000000000000000000, 0.8660254037844387076, 1.000000000000000000, 0.8660254037844387076, 1.000000000000000000, 0.8660254037844387076, 1.000000000000000000, 0.8660254037844387076, 1.000000000000000000, 0.8660254037844387076, 1.000000000000000000, 0.8660254037844387076, 1.000000000000000000, 0.8660254037844387076, 1.000000000000000000, 0.8660254037844387076, 1.000000000000000000, 0.8660254037844387076, 1.000000000000000000, 0.8660254037844387076, 1.000000000000000000, 0.8660254037844387076, 1.000000000000000000, 0.8660254037844387076, 1.000000000000000000, 0.8660254037844387076, 1.000000000000000000, 0.8660254037844387076, 1.000000000000000000, 0.8660254037844387076, 1.000000000000000000, 0.8660254037844387076, 1.000000000000000000, 0.8660254037844387076, 1.000000000000000000, 0.8660254037844387076, 1.000000000000000000, 0.8660254037844387076, 1.000000000000000000, 0.8660254037844387076, 1.000000000000000000, 0.8660254037844387076, 1.000000000000000000, 0.8660254037844387076, 1.000000000000000000, 0.8660254037844387076, 1.000000000000000000, 0.8660254037844387076, 1.000000000000000000, 0.8660254037844387076, 1.000000000000000000, 0.8660254037844387076, 1.000000000000000000, 0.8660254037844387076, 1.000000000000000000, 0.8660254037844387076, 1.000000000000000000, 0.8660254037844387076, 1.000000000000000000, 0.8660254037844387076, 1.000000000000000000, 0.8660254037844387076, 1.000000000000000000, 0.8660254037844387076, 1.000000000000000000, 0.8660254037844387076, 1.000000000000000000, 0.8660254037844387076, 1.000000000000000000, 0.8660254037844387076, 1.000000000000000000, 0.8660254037844387076, 1.000000000000000000, 0.8660254037844387076, 1.000000000000000000, 0.8660254037844387076, 1.000000000000000000, 0.8660254037844387076, 1.000000000000000000, 0.8660254037844387076, 1.000000000000000000, 0.8660254037844387076, 1.000000000000000000, 0.8660254037844387076, 1.000000000000000000, 0.8660254037844387076, 1.000000000000000000, 0.8660254037844387076, 1.000000000000000000, 0.8660254037844387076, 1.000000000000000000, 0.8660254037844387076, 1.000000000000000000, 0.8660254037844387076, 1.000000000000000000, 0.8660254037844387076, 1.000000000000000000, 0.8660254037844387076, 1.000000000000000000, 0.8660254037844387076, 1.000000000000000000, 0.8660254037844387076, 1.000000000000000000, 0.8660254037844387076, 1.000000000000000000, 0.8660254037844387076, 1.000000000000000000, 0.8660254037844387076, 1.000000000000000000, 0.8660254037844387076, 1.000000000000000000, 0.8660254037844387076, 1.000000000000000000, 0.8660254037844387076, 1.000000000000000000, 0.8660254037844387076, 1.000000000000000000, 0.8660254037844387076, 1.000000000000000000, 0.8660254037844387076, 1.000000000000000000, 0.8660254037844387076, 1.000000000000000000, 0.8660254037844387076, 1.000000000000000000, 0.8660254037844387076, 1.000000000000000000, 0.8660254037844387076, 1.000000000000000000, 0.8660254037844387076, 1.000000000000000000, 0.8660254037844387076, 1.000000000000000000, 0.8660254037844387076, 1.000000000000000000, 0.8660254037844387076, 1.000000000000000000, 0.8660254037844387076, 1.000000000000000000, 0.8660254037844387076, 1.000000000000000000, 0.8660254037844387076, 1.000000000000000000, 0.8660254037844387076, 1.000000000000000000, 0.8660254037844387076, 1.000000000000000000, 0.8660254037844387076, 1.000000000000000000, 0.8660254037844387076, 1.000000000000000000, 0.8660254037844387076, 1.000000000000000000, 0.8660254037844387076, 1.000000000000000000, 0.8660254037844387076, 1.000000000000000000, 0.8660254037844387076, 1.000000000000000000, 0.8660254037844387076, 1.000000000000000000, 0.8660254037844387076, 1.000000000000000000, 0.8660254037844387076, 1.000000000000000000, 0.8660254037844387076, 1.000000000000000000, 0.8660254037844387076, 1.000000000000000000, 0.8660254037844387076, 1.000000000000000000, 0.8660254037844387076, 1.000000000000000000, 0.8660254037844387076, 1.000000000000000000, 0.8660254037844387076, 1.000000000000000000, 0.8660254037844387076, 1.000000000000000000, 0.8660254037844387076, 1.000000000000000000, 0.8660254037844387076, 1.000000000000000000, 0.8660254037844387076, 1.000000000000000000, 0.8660254037844387076, 1.000000000000000000, 0.8660254037844387076, 1.000000000000000000, 0.8660254037844387076, 1.000000000000000000, 0.8660254037844387076, 1.000000000000000000, 0.8660254037844387076, 1.000000000000000000, 0.8660254037844387076, 1.000000000000000000, 0.8660254037844387076, 1.000000000000000000, 0.8660254037844387076, 1.000000000000000000, 0.8660254037844387076, 1.000000000000000000, 0.8660254037844387076, 1.000000000000000000, 0.8660254037844387076, 1.000000000000000000, 0.8660254037844387076, 1.000000000000000000, 0.8660254037844387076, 1.000000000000000000, 0.8660254037844387076, 1.000000000000000000, 0.8660254037844387076, 1.000000000000000000, 0.8660254037844387076, 1.000000000000000000, 0.8660254037844387076, 1.000000000000000000, 0.8660254037844387076, 1.000000000000000000, 0.8660254037844387076, 1.000000000000000000, 0.8660254037844387076, 1.000000000000000000, 0.8660254037844387076, 1.000000000000000000, 0.8660254037844387076, 1.000000000000000000, 0.8660254037844387076, 1.000000000000000000, 0.8660254037844387076, 1.000000000000000000, 0.8660254037844387076, 1.000000000000000000, 0.8660254037844387076, 1.000000000000000000, 0.8660254037844387076, 1.000000000000000000, 0.8660254037844387076, 1.000000000000000000, 0.8660254037844387076, 1.000000000000000000, 0.8660254037844387076, 1.000000000000000000, 0.8660254037844387076, 1.000000000000000000, 0.8660254037844387076, 1.000000000000000000, 0.8660254037844387076, 1.000000000000000000, 0.8660254037844387076, 1.000000000000000000, 0.8660254037844387076, 1.000000000000000000, 0.8660254037844387076, 1.000000000000000000, 0.8660254037844387076, 1.000000000000000000, 0.8660254037844387076, 1.000000000000000000, 0.8660254037844387076, 1.000000000000000000, 0.8660254037844387076, 1.000000000000000000, 0.8660254037844387076, 1.000000000000000000, 0.8660254037844387076, 1.000000000000000000, 0.8660254037844387076, 1.000000000000000000, 0.8660254037844387076, 1.000000000000000000, 0.8660254037844387076, 1.000000000000000000, 0.8660254037844387076, 1.000000000000000000, 0.8660254037844387076, 1.000000000000000000, 0.8660254037844387076, 1.000000000000000000, 0.8660254037844387076, 1.000000000000000000, 0.8660254037844387076, 1.000000000000000000, 0.8660254037844387076, 1.000000000000000000, 0.8660254037844387076, 1.000000000000000000, 0.8660254037844387076, 1.000000000000000000, 0.8660254037844387076, 1.000000000000000000, 0.8660254037844387076, 1.000000000000000000, 0.8660254037844387076, 1.000000000000000000, 0.8660254037844387076, 1.000000000000000000, 0.8660254037844387076, 1.000000000000000000, 0.8660254037844387076, 1.000000000000000000, 0.8660254037844387076, 1.000000000000000000, 0.8660254037844387076, 1.000000000000000000, 0.8660254037844387076, 1.000000000000000000, 0.8660254037844387076, 1.000000000000000000, 0.8660254037844387076, 1.000000000000000000, 0.8660254037844387076, 1.000000000000000000, 0.8660254037844387076, 1.000000000000000000, 0.8660254037844387076, 1.000000000000000000, 0.8660254037844387076, 1.000000000000000000, 0.8660254037844387076, 1.000000000000000000, 0.8660254037844387076, 1.000000000000000000, 0.8660254037844387076, 1.000000000000000000, 0.8660254037844387076, 1.000000000000000000, 0.8660254037844387076, 1.000000000000000000, 0.8660254037844387076, 1.000000000000000000, 0.8660254037844387076, 1.000000000000000000, 0.8660254037844387076, 1.000000000000000000, 0.8660254037844387076, 1.000000000000000000, 0.8660254037844387076, 1.000000000000000000, 0.8660254037844387076, 1.000000000000000000, 0.8660254037844387076, 1.000000000000000000, 0.8660254037844387076, 1.000000000000000000, 0.8660254037844387076, 1.000000000000000000, 0.8660254037844387076, 1.000000000000000000, 0.8660254037844387076, 1.000000000000000000, 0.8660254037844387076, 1.000000000000000000, 0.8660254037844387076, 1.000000000000000000, 0.8660254037844387076, 1.000000000000000000, 0.8660254037844387076, 1.000000000000000000, 0.8660254037844387076, 1.000000000000000000, 0.8660254037844387076, 1.000000000000000000, 0.8660254037844387076, 1.000000000000000000, 0.8660254037844387076, 1.000000000000000000, 0.8660254037844387076, 1.000000000000000000, 0.8660254037844387076, 1.000000000000000000, 0.8660254037844387076, 1.000000000000000000, 0.8660254037844387076, 1.000000000000000000, 0.8660254037844387076, 1.000000000000000000, 0.8660254037844387076, 1.000000000000000000, 0.8660254037844387076, 1.000000000000000000, 0.8660254037844387076, 1.000000000000000000, 0.8660254037844387076, 1.000000000000000000, 0.8660254037844387076, 1.000000000000000000, 0.8660254037844387076, 1.000000000000000000, 0.8660254037844387076, 1.000000000000000000, 0.8660254037844387076, 1.000000000000000000, 0.8660254037844387076, 1.000000000000000000, 0.8660254037844387076, 1.000000000000000000, 0.8660254037844387076, 1.000000000000000000, 0.8660254037844387076, 1.000000000000000000, 0.8660254037844387076, 1.000000000000000000, 0.8660254037844387076, 1.000000000000000000, 0.8660254037844387076, 1.000000000000000000, 0.8660254037844387076, 1.000000000000000000, 0.8660254037844387076, 1.000000000000000000, 0.8660254037844387076, 1.000000000000000000, 0.8660254037844387076, 1.000000000000000000, 0.8660254037844387076, 1.000000000000000000, 0.8660254037844387076, 1.000000000000000000, 0.8660254037844387076, 1.000000000000000000, 0.8660254037844387076, 1.000000000000000000, 0.8660254037844387076, 1.000000000000000000, 0.8660254037844387076, 1.000000000000000000, 0.8660254037844387076, 1.000000000000000000, 0.8660254037844387076, 1.000000000000000000, 0.8660254037844387076, 1.000000000000000000, 0.8660254037844387076, 1.000000000000000000, 0.8660254037844387076, 1.000000000000000000, 0.8660254037844387076, 1.000000000000000000, 0.8660254037844387076, 1.000000000000000000, 0.8660254037844387076, 1.000000000000000000, 0.8660254037844387076, 1.000000000000000000, 0.8660254037844387076, 1.000000000000000000, 0.8660254037844387076, 1.000000000000000000, 0.8660254037844387076, 1.000000000000000000, 0.8660254037844387076, 1.000000000000000000, 0.8660254037844387076, 1.000000000000000000, 0.8660254037844387076, 1.000000000000000000, 0.8660254037844387076, 1.000000000000000000, 0.8660254037844387076, 1.000000000000000000, 0.8660254037844387076, 1.000000000000000000, 0.8660254037844387076, 1.000000000000000000, 0.8660254037844387076, 1.000000000000000000, 0.8660254037844387076, 1.000000000000000000, 0.8660254037844387076, 1.000000000000000000, 0.8660254037844387076, 1.000000000000000000, 0.8660254037844387076, 1.000000000000000000, 0.8660254037844387076, 1.000000000000000000, 0.8660254037844387076, 1.000000000000000000, 0.8660254037844387076, 1.000000000000000000, 0.8660254037844387076, 1.000000000000000000, 0.8660254037844387076, 1.000000000000000000, 0.8660254037844387076, 1.000000000000000000, 0.8660254037844387076, 1.000000000000000000, 0.8660254037844387076, 1.000000000000000000, 0.8660254037844387076, 1.000000000000000000, 0.8660254037844387076, 1.000000000000000000, 0.8660254037844387076, 1.000000000000000000, 0.8660254037844387076, 1.000000000000000000, 0.8660254037844387076, 1.000000000000000000, 0.8660254037844387076, 1.000000000000000000, 0.8660254037844387076, 1.000000000000000000, 0.8660254037844387076, 1.000000000000000000, 0.8660254037844387076, 1.000000000000000000, 0.8660254037844387076, 1.000000000000000000, 0.8660254037844387076, 1.000000000000000000, 0.8660254037844387076, 1.000000000000000000, 0.8660254037844387076, 1.000000000000000000, 0.8660254037844387076, 1.000000000000000000, 0.8660254037844387076, 1.000000000000000000, 0.8660254037844387076, 1.000000000000000000, 0.8660254037844387076, 1.000000000000000000, 0.8660254037844387076, 1.000000000000000000, 0.8660254037844387076, 1.000000000000000000, 0.8660254037844387076, 1.000000000000000000, 0.8660254037844387076, 1.000000000000000000, 0.8660254037844387076, 1.000000000000000000, 0.8660254037844387076, 1.000000000000000000, 0.8660254037844387076, 1.000000000000000000, 0.8660254037844387076, 1.000000000000000000, 0.8660254037844387076, 1.000000000000000000, 0.8660254037844387076, 1.000000000000000000, 0.8660254037844387076, 1.000000000000000000, 0.8660254037844387076, 1.000000000000000000, 0.8660254037844387076, 1.000000000000000000, 0.8660254037844387076, 1.000000000000000000, 0.8660254037844387076, 1.000000000000000000, 0.8660254037844387076, 1.000000000000000000, 0.8660254037844387076, 1.000000000000000000, 0.8660254037844387076, 1.000000000000000000, 0.8660254037844387076, 1.000000000000000000, 0.8660254037844387076, 1.000000000000000000, 0.8660254037844387076, 1.000000000000000000, 0.8660254037844387076, 1.000000000000000000, 0.8660254037844387076, 1.000000000000000000, 0.8660254037844387076, 1.000000000000000000, 0.8660254037844387076, 1.000000000000000000, 0.8660254037844387076, 1.000000000000000000, 0.8660254037844387076, 1.000000000000000000, 0.8660254037844387076, 1.000000000000000000, 0.8660254037844387076, 1.000000000000000000, 0.8660254037844387076, 1.000000000000000000, 0.8660254037844387076, 1.000000000000000000, 0.8660254037844387076, 1.000000000000000000, 0.8660254037844387076, 1.000000000000000000, 0.8660254037844387076, 1.000000000000000000, 0.8660254037844387076, 1.000000000000000000, 0.8660254037844387076, 1.000000000000000000, 0.8660254037844387076, 1.000000000000000000, 0.8660254037844387076, 1.000000000000000000, 0.8660254037844387076, 1.000000000000000000, 0.8660254037844387076, 1.000000000000000000, 0.8660254037844387076, 1.000000000000000000, 0.8660254037844387076, 1.000000000000000000, 0.8660254037844387076, 1.000000000000000000, 0.8660254037844387076, 1.000000000000000000, 0.8660254037844387076, 1.000000000000000000, 0.8660254037844387076, 1.000000000000000000, 0.8660254037844387076, 1.000000000000000000, 0.8660254037844387076, 1.000000000000000000, 0.8660254037844387076, 1.000000000000000000, 0.8660254037844387076, 1.000000000000000000, 0.8660254037844387076, 1.000000000000000000, 0.8660254037844387076, 1.000000000000000000, 0.8660254037844387076, 1.000000000000000000, 0.8660254037844387076, 1.000000000000000000, 0.8660254037844387076, 1.000000000000000000, 0.8660254037844387076, 1.000000000000000000, 0.8660254037844387076, 1.000000000000000000, 0.8660254037844387076, 1.000000000000000000, 0.8660254037844387076, 1.000000000000000000, 0.8660254037844387076, 1.000000000000000000, 0.8660254037844387076, 1.000000000000000000, 0.8660254037844387076, 1.000000000000000000, 0.8660254037844387076, 1.000000000000000000, 0.8660254037844387076, 1.000000000000000000, 0.8660254037844387076, 1.000000000000000000, 0.8660254037844387076, 1.000000000000000000, 0.8660254037844387076, 1.000000000000000000, 0.8660254037844387076, 1.000000000000000000, 0.8660254037844387076, 1.000000000000000000, 0.8660254037844387076, 1.000000000000000000) ) ) 
 REPRESENTATION_ITEM ( '' )  SURFACE ( )  );
#30266=ADVANCED_FACE ( 'NONE', ( #43429 ), #52783, .T. ) ;
#30272=CARTESIAN_POINT ( 'NONE',  ( -1.339745962155613146, 28.33034180399266333, 5.000000000000000000 ) ) ;
#30274=CARTESIAN_POINT ( 'NONE',  ( -5.000000000000000000, -48.95833333060213732, -2.886751345948128211 ) ) ;
#30277=CARTESIAN_POINT ( 'NONE',  ( 4.458734124999998549, -28.97916666530107577, -2.574251347313721627 ) ) ;
#30283=EDGE_CURVE ( 'NONE', #61600, #22073, #63275, .T. ) ;
#30286=LINE ( 'NONE', #15182, #26920 ) ;
#30289=CARTESIAN_POINT ( 'NONE',  ( 4.458734125000001214, -75.14583333196775072, 2.574251347313718519 ) ) ;
#30294=CARTESIAN_POINT ( 'NONE',  ( -2.499999999999996447, 8.166666666666666075, 4.330127018922195425 ) ) ;
#30296=CARTESIAN_POINT ( 'NONE',  ( -2.229367062500000163, -1.729166665301071992, -3.861377020970580443 ) ) ;
#30298=CARTESIAN_POINT ( 'NONE',  ( -1.339745962155613812, -93.08034179853027013, -5.000000000000000000 ) ) ;
#30299=CARTESIAN_POINT ( 'NONE',  ( 5.000000000000000000, -27.41666666666666430, -2.886751345948130876 ) ) ;
#30304=FACE_OUTER_BOUND ( 'NONE', #2211, .T. ) ;
#30306=CARTESIAN_POINT ( 'NONE',  ( 4.458734124999998549, -78.72916666530106511, -2.574251347313721627 ) ) ;
#30307=CARTESIAN_POINT ( 'NONE',  ( 5.000000000000000888, -75.58333333333334281, 2.886751345948126879 ) ) ;
#30308=CARTESIAN_POINT ( 'NONE',  ( -3.152548672688508926E-16, 4.437500001365595637, -5.148502694627439702 ) ) ;
#30311=CARTESIAN_POINT ( 'NONE',  ( 2.229367062500001939, -69.22916666530107932, 3.861377020970579999 ) ) ;
#30312=CARTESIAN_POINT ( 'NONE',  ( 2.500000000000002220, -27.54166666393548013, 4.330127018922192761 ) ) ;
#30314=CARTESIAN_POINT ( 'NONE',  ( -2.499999999999996447, -40.83333333333333570, 4.330127018922195425 ) ) ;
#30315=CARTESIAN_POINT ( 'NONE',  ( -2.500000000000000444, -56.16666666666667140, -4.330127018922193649 ) ) ;
#30317=CARTESIAN_POINT ( 'NONE',  ( -3.152548672688508926E-16, -47.56249999863440792, -5.148502694627439702 ) ) ;
#30318=CARTESIAN_POINT ( 'NONE',  ( 2.229367062500001939, -31.22916666530107221, 3.861377020970579999 ) ) ;
#30321=CARTESIAN_POINT ( 'NONE',  ( -4.999999999999999112, 21.08333333333333215, 2.886751345948131764 ) ) ;
#30324=CARTESIAN_POINT ( 'NONE',  ( -4.458734124999998549, -37.22916666530107221, 2.574251347313722516 ) ) ;
#30325=CARTESIAN_POINT ( 'NONE',  ( 1.060575238724906964E-15, -75.62499999726880162, 5.773502691896257311 ) ) ;
#30327=CARTESIAN_POINT ( 'NONE',  ( 1.339745962155615144, -24.58034179853029499, 4.999999999999999112 ) ) ;
#30329=CARTESIAN_POINT ( 'NONE',  ( 4.458734124999999437, -82.06249999863440792, -5.460374474430324690E-16 ) ) ;
#30331=CARTESIAN_POINT ( 'NONE',  ( 1.339745962155615144, 18.41965820146970856, 4.999999999999999112 ) ) ;
#30333=CARTESIAN_POINT ( 'NONE',  ( 5.000000000000000888, -26.58333333333333570, 2.886751345948126879 ) ) ;
#30339=CARTESIAN_POINT ( 'NONE',  ( 5.000000000000000000, 21.62500000273118417, -6.123233995736766282E-16 ) ) ;
#30346=EDGE_CURVE ( 'NONE', #52846, #21770, #41854, .T. ) ;
#30348=CARTESIAN_POINT ( 'NONE',  ( -5.000000000000000000, -0.08333333333333454995, -2.886751345948128211 ) ) ;
#30349=CARTESIAN_POINT ( 'NONE',  ( 1.339745962155613146, 28.41965820146970501, 5.000000000000000888 ) ) ;
#30352=CARTESIAN_POINT ( 'NONE',  ( -4.458734124999998549, -20.22916666530107221, 2.574251347313722516 ) ) ;
#30354=CARTESIAN_POINT ( 'NONE',  ( -5.000000000000000000, -77.87499999726881583, 0.000000000000000000 ) ) ;
#30358=EDGE_CURVE ( 'NONE', #56173, #44977, #21775, .T. ) ;
#30360=ORIENTED_EDGE ( 'NONE', *, *, #48877, .F. ) ;
#30361=CARTESIAN_POINT ( 'NONE',  ( 6.123233995736766282E-16, -120.0000000000000000, -5.000000000000000000 ) ) ;
#30363=VERTEX_POINT ( 'NONE', #30870 ) ;
#30365=CARTESIAN_POINT ( 'NONE',  ( 1.243387493232115550E-13, -9.124999997268817609, -5.000000000000000000 ) ) ;
#30367=EDGE_CURVE ( 'NONE', #13643, #29768, #55012, .T. ) ;
#30368=ORIENTED_EDGE ( 'NONE', *, *, #52376, .F. ) ;
#30369=EDGE_CURVE ( 'NONE', #14857, #25665, #30218, .T. ) ;
#30370=CARTESIAN_POINT ( 'NONE',  ( -6.972266317189433020E-16, -99.24999999999998579, -5.000000000000000000 ) ) ;
#30373=EDGE_LOOP ( 'NONE', ( #54643, #38925, #43402, #545 ) ) ;
#30374=EDGE_CURVE ( 'NONE', #34229, #24623, #19684, .T. ) ;
#30376=CARTESIAN_POINT ( 'NONE',  ( 2.229367062499998831, 13.35416666803226171, -3.861377020970580887 ) ) ;
#30379=CARTESIAN_POINT ( 'NONE',  ( 0.000000000000000000, -120.0000000000000000, 0.000000000000000000 ) ) ;
#30382=CARTESIAN_POINT ( 'NONE',  ( 2.229367062499998831, -66.64583333196773651, -3.861377020970580887 ) ) ;
#30383=CARTESIAN_POINT ( 'NONE',  ( -5.000000000000000000, -49.95833333060213022, -2.886751345948128211 ) ) ;
#30384=CARTESIAN_POINT ( 'NONE',  ( -2.229367062499996610, 19.85416666803225993, 3.861377020970582219 ) ) ;
#30388=CARTESIAN_POINT ( 'NONE',  ( 4.458734124999999437, -47.06249999863440792, -5.460374474430324690E-16 ) ) ;
#30389=CARTESIAN_POINT ( 'NONE',  ( 1.060575238724906964E-15, -7.624999997268813168, 5.773502691896257311 ) ) ;
#30391=CARTESIAN_POINT ( 'NONE',  ( -1.339745962155613812, -66.08034179853028434, -5.000000000000000000 ) ) ;
#30394=CARTESIAN_POINT ( 'NONE',  ( -3.152548672688508926E-16, -14.81249999863440436, -5.148502694627439702 ) ) ;
#30397=CARTESIAN_POINT ( 'NONE',  ( -4.458734124999998549, -104.2291666653010651, 2.574251347313722516 ) ) ;
#30400=CARTESIAN_POINT ( 'NONE',  ( 2.229367062500001939, -99.22916666530105090, 3.861377020970579999 ) ) ;
#30402=CARTESIAN_POINT ( 'NONE',  ( -5.000000000000000000, -57.87499999726880873, 0.000000000000000000 ) ) ;
#30406=CARTESIAN_POINT ( 'NONE',  ( 9.457646018065525792E-16, -24.06249999863440436, 5.148502694627439702 ) ) ;
#30407=CARTESIAN_POINT ( 'NONE',  ( -3.152548672688508926E-16, 5.187500001365592972, -5.148502694627439702 ) ) ;
#30408=CARTESIAN_POINT ( 'NONE',  ( -2.229367062500000163, -62.72916666530106511, -3.861377020970580443 ) ) ;
#30411=CARTESIAN_POINT ( 'NONE',  ( -1.339745962155610925, -32.79465819873851729, 5.000000000000000000 ) ) ;
#30413=CARTESIAN_POINT ( 'NONE',  ( 5.000000000000000888, -12.58333333333333570, 2.886751345948126879 ) ) ;
#30415=ORIENTED_EDGE ( 'NONE', *, *, #54183, .T. ) ;
#30418=CARTESIAN_POINT ( 'NONE',  ( 2.499999999999998668, -90.33333333333332860, -4.330127018922193649 ) ) ;
#30421=CARTESIAN_POINT ( 'NONE',  ( 1.339745962155615144, -82.70534180126146850, 4.999999999999999112 ) ) ;
#30425=CARTESIAN_POINT ( 'NONE',  ( 2.500000000000002220, -77.66666666666665719, 4.330127018922192761 ) ) ;
#30428=CARTESIAN_POINT ( 'NONE',  ( 2.500000000000002220, -80.54166666393547303, 4.330127018922192761 ) ) ;
#30430=CARTESIAN_POINT ( 'NONE',  ( 1.339745962155612702, -85.29465819873851729, -5.000000000000000000 ) ) ;
#30440=( BOUNDED_CURVE ( )  B_SPLINE_CURVE ( 2, ( #30900, #50528, #36680, #1653, #56314, #6470, #7103, #40859, #16430 ),
 .UNSPECIFIED., .F., .F. ) 
 B_SPLINE_CURVE_WITH_KNOTS ( ( 3, 2, 2, 2, 3 ),
 ( 0.7839285714285714191, 0.7845238095238095122, 0.7857142857142856984, 0.7869047619047618847, 0.7874999999999999778 ),
 .UNSPECIFIED. ) 
 CURVE ( )  GEOMETRIC_REPRESENTATION_ITEM ( )  RATIONAL_B_SPLINE_CURVE ( ( 0.9330127018922194093, 0.9330127018922194093, 1.000000000000000000, 0.8660254037844387076, 1.000000000000000000, 0.8660254037844387076, 1.000000000000000000, 0.9330127018922194093, 0.9330127018922194093 ) ) 
 REPRESENTATION_ITEM ( '' )  );
#30443=ORIENTED_EDGE ( 'NONE', *, *, #29563, .T. ) ;
#30446=CARTESIAN_POINT ( 'NONE',  ( -2.499999999999996447, -83.83333333333332860, 4.330127018922195425 ) ) ;
#30448=EDGE_CURVE ( 'NONE', #29631, #27636, #50120, .T. ) ;
#30451=CARTESIAN_POINT ( 'NONE',  ( -4.458734124999999437, 27.60416666803226349, -2.574251347313719407 ) ) ;
#30453=ORIENTED_EDGE ( 'NONE', *, *, #12655, .T. ) ;
#30457=CARTESIAN_POINT ( 'NONE',  ( -4.458734124999999437, -41.39583333196773651, -2.574251347313719407 ) ) ;
#30460=CARTESIAN_POINT ( 'NONE',  ( -4.458734124999999437, -51.31249999863440792, 0.000000000000000000 ) ) ;
#30461=CARTESIAN_POINT ( 'NONE',  ( 5.000000000000000888, 2.541666669397851130, 2.886751345948126879 ) ) ;
#30462=CARTESIAN_POINT ( 'NONE',  ( -4.458734124999998549, -18.22916666530107221, 2.574251347313722516 ) ) ;
#30463=CARTESIAN_POINT ( 'NONE',  ( 2.499999999999998668, -103.3333333333333286, -4.330127018922193649 ) ) ;
#30465=CARTESIAN_POINT ( 'NONE',  ( -2.229367062500000163, -33.72916666530107221, -3.861377020970580443 ) ) ;
#30466=CARTESIAN_POINT ( 'NONE',  ( 5.000000000000000000, 8.708333336064518093, -2.886751345948129988 ) ) ;
#30472=CYLINDRICAL_SURFACE ( 'NONE', #57141, 5.000000000000000000 ) ;
#30473=CARTESIAN_POINT ( 'NONE',  ( 2.229367062500001939, -0.2291666653010705768, 3.861377020970579999 ) ) ;
#30475=AXIS2_PLACEMENT_3D ( 'NONE', #37868, #48452, #42997 ) ;
#30476=CARTESIAN_POINT ( 'NONE',  ( 2.500000000000002220, -30.66666666666666785, 4.330127018922192761 ) ) ;
#30478=CARTESIAN_POINT ( 'NONE',  ( 4.458734124999998549, -88.72916666530106511, -2.574251347313721627 ) ) ;
#30479=CARTESIAN_POINT ( 'NONE',  ( 4.458734124999999437, -37.81249999863440792, -5.460374474430324690E-16 ) ) ;
#30481=CARTESIAN_POINT ( 'NONE',  ( 4.458734124999998549, -83.97916666530107932, -2.574251347313721627 ) ) ;
#30487=CARTESIAN_POINT ( 'NONE',  ( -4.458734124999999437, -3.395833331967739177, -2.574251347313719407 ) ) ;
#30488=CARTESIAN_POINT ( 'NONE',  ( -3.152548672688508926E-16, 24.18750000136559564, -5.148502694627439702 ) ) ;
#30489=CARTESIAN_POINT ( 'NONE',  ( 4.458734124999998549, -46.97916666530106511, -2.574251347313721627 ) ) ;
#30497=CARTESIAN_POINT ( 'NONE',  ( -4.458734124999999437, -76.31249999863440792, 0.000000000000000000 ) ) ;
#30498=CARTESIAN_POINT ( 'NONE',  ( 2.229367062499998831, 29.10416666803225993, -3.861377020970580887 ) ) ;
#30501=CARTESIAN_POINT ( 'NONE',  ( 2.229367062499998831, -109.8958333319677365, -3.861377020970580887 ) ) ;
#30503=CARTESIAN_POINT ( 'NONE',  ( -5.000000000000000000, -57.99999999999999289, 0.000000000000000000 ) ) ;
#30507=CARTESIAN_POINT ( 'NONE',  ( -2.500000000000000444, -73.04166666393548724, -4.330127018922193649 ) ) ;
#30514=ORIENTED_EDGE ( 'NONE', *, *, #8142, .F. ) ;
#30515=DIRECTION ( 'NONE',  ( -0.000000000000000000, 1.000000000000000000, -0.000000000000000000 ) ) ;
#30516=CARTESIAN_POINT ( 'NONE',  ( -1.339745962155613812, 10.91965820146970678, -5.000000000000000000 ) ) ;
#30522=CARTESIAN_POINT ( 'NONE',  ( 4.458734124999999437, -46.06249999863440081, -5.460374474430324690E-16 ) ) ;
#30523=CARTESIAN_POINT ( 'NONE',  ( 6.123233995736766282E-16, -120.0000000000000000, -5.000000000000000000 ) ) ;
#30525=FACE_OUTER_BOUND ( 'NONE', #48923, .T. ) ;
#30532=AXIS2_PLACEMENT_3D ( 'NONE', #3043, #12986, #61262 ) ;
#30533=CARTESIAN_POINT ( 'NONE',  ( -2.229367062499996610, -95.39583333196773651, 3.861377020970582219 ) ) ;
#30534=CARTESIAN_POINT ( 'NONE',  ( 0.000000000000000000, -120.0000000000000000, 5.000000000000000000 ) ) ;
#30536=CARTESIAN_POINT ( 'NONE',  ( 1.975475456537005874E-15, -71.62499999726878741, 5.000000000000000000 ) ) ;
#30541=CARTESIAN_POINT ( 'NONE',  ( 4.458734124999999437, 0.1875000013655953035, -5.460374474430324690E-16 ) ) ;
#30542=CARTESIAN_POINT ( 'NONE',  ( 2.229367062499998831, -17.89583333196773651, -3.861377020970580887 ) ) ;
#30545=CARTESIAN_POINT ( 'NONE',  ( 1.975475456537005874E-15, -77.62499999726881583, 5.000000000000000000 ) ) ;
#30547=CARTESIAN_POINT ( 'NONE',  ( 4.458734125000000326, 16.85416666803225993, 2.574251347313718519 ) ) ;
#30551=CARTESIAN_POINT ( 'NONE',  ( 4.458734124999999437, -20.81249999863440081, -5.460374474430324690E-16 ) ) ;
#30553=CARTESIAN_POINT ( 'NONE',  ( -2.480964764533239819E-13, -73.62499999726883004, 5.000000000000000000 ) ) ;
#30556=CARTESIAN_POINT ( 'NONE',  ( -5.000000000000000000, -48.87499999726880873, 0.000000000000000000 ) ) ;
#30557=CARTESIAN_POINT ( 'NONE',  ( -2.499999999999996447, 21.29166666939785202, 4.330127018922195425 ) ) ;
#30558=CARTESIAN_POINT ( 'NONE',  ( 4.458734125000000326, 14.10416666803226349, 2.574251347313718519 ) ) ;
#30559=CARTESIAN_POINT ( 'NONE',  ( 1.339745962155612702, -35.29465819873851729, -5.000000000000000000 ) ) ;
#30562=CARTESIAN_POINT ( 'NONE',  ( -4.458734124999999437, -69.31249999863439371, 0.000000000000000000 ) ) ;
#30563=VERTEX_POINT ( 'NONE', #34738 ) ;
#30566=CARTESIAN_POINT ( 'NONE',  ( 5.000000000000000888, 4.416666666666666075, 2.886751345948126879 ) ) ;
#30569=CARTESIAN_POINT ( 'NONE',  ( 4.458734124999999437, -57.81249999863440081, -5.460374474430324690E-16 ) ) ;
#30570=CARTESIAN_POINT ( 'NONE',  ( 5.000000000000000000, -95.29166666393547303, -2.886751345948129988 ) ) ;
#30572=CARTESIAN_POINT ( 'NONE',  ( 2.229367062500001939, -35.97916666530107221, 3.861377020970579999 ) ) ;
#30578=EDGE_CURVE ( 'NONE', #7254, #60295, #16465, .T. ) ;
#30579=CARTESIAN_POINT ( 'NONE',  ( 5.000000000000000000, -16.37499999726881228, -6.123233995736766282E-16 ) ) ;
#30581=CARTESIAN_POINT ( 'NONE',  ( 2.499999999999998668, -45.33333333333333570, -4.330127018922193649 ) ) ;
#30582=CARTESIAN_POINT ( 'NONE',  ( 0.000000000000000000, -120.0000000000000000, 5.000000000000000000 ) ) ;
#30584=ORIENTED_EDGE ( 'NONE', *, *, #34941, .T. ) ;
#30585=CARTESIAN_POINT ( 'NONE',  ( -3.152548672688508926E-16, -104.5624999986343937, -5.148502694627439702 ) ) ;
#30586=CARTESIAN_POINT ( 'NONE',  ( 4.458734125000001214, 2.854166668032259491, 2.574251347313718519 ) ) ;
#30591=( BOUNDED_CURVE ( )  B_SPLINE_CURVE ( 2, ( #53759, #4255, #9073, #23870, #48930, #10338, #38647, #25129, #9693 ),
 .UNSPECIFIED., .F., .F. ) 
 B_SPLINE_CURVE_WITH_KNOTS ( ( 3, 2, 2, 2, 3 ),
 ( 0.1910714285714285865, 0.1916666666666666796, 0.1928571428571428659, 0.1940476190476190521, 0.1946428571428571452 ),
 .UNSPECIFIED. ) 
 CURVE ( )  GEOMETRIC_REPRESENTATION_ITEM ( )  RATIONAL_B_SPLINE_CURVE ( ( 0.9330127018922194093, 0.9330127018922209636, 1.000000000000000000, 0.8660254037844387076, 1.000000000000000000, 0.8660254037844387076, 1.000000000000000000, 0.9330127018922194093, 0.9330127018922194093 ) ) 
 REPRESENTATION_ITEM ( '' )  );
#30601=CARTESIAN_POINT ( 'NONE',  ( 9.457646018065525792E-16, -32.31249999863440792, 5.148502694627439702 ) ) ;
#30609=ADVANCED_FACE ( 'NONE', ( #55072 ), #51206, .T. ) ;
#30610=CARTESIAN_POINT ( 'NONE',  ( 5.000000000000000888, -20.45833333060214798, 2.886751345948126879 ) ) ;
#30612=CARTESIAN_POINT ( 'NONE',  ( -2.229367062500000163, -76.72916666530106511, -3.861377020970580443 ) ) ;
#30613=CARTESIAN_POINT ( 'NONE',  ( -4.999999999999998224, 13.20833333606451987, 2.886751345948131764 ) ) ;
#30614=ORIENTED_EDGE ( 'NONE', *, *, #2880, .F. ) ;
#30617=CARTESIAN_POINT ( 'NONE',  ( 1.975475456537005874E-15, -31.62499999726880873, 5.000000000000000000 ) ) ;
#30620=CARTESIAN_POINT ( 'NONE',  ( -2.229367062499996610, -4.395833331967740065, 3.861377020970582219 ) ) ;
#30622=LINE ( 'NONE', #1386, #27586 ) ;
#30629=ORIENTED_EDGE ( 'NONE', *, *, #20817, .F. ) ;
#30630=CARTESIAN_POINT ( 'NONE',  ( 4.458734125000000326, -79.89583333196773651, 2.574251347313718519 ) ) ;
#30631=CARTESIAN_POINT ( 'NONE',  ( -1.339745962155610925, -96.79465819873851729, 5.000000000000000000 ) ) ;
#30632=CARTESIAN_POINT ( 'NONE',  ( -2.229367062499996610, -5.145833331967740065, 3.861377020970582219 ) ) ;
#30633=ADVANCED_FACE ( 'NONE', ( #1060 ), #50881, .T. ) ;
#30636=CARTESIAN_POINT ( 'NONE',  ( 4.458734125000001214, -69.14583333196773651, 2.574251347313718519 ) ) ;
#30637=CARTESIAN_POINT ( 'NONE',  ( 2.499999999999998668, -33.20833333060215153, -4.330127018922193649 ) ) ;
#30639=CARTESIAN_POINT ( 'NONE',  ( -5.000000000000000000, -40.99999999999999289, 0.000000000000000000 ) ) ;
#30640=CARTESIAN_POINT ( 'NONE',  ( 1.339745962155615144, -104.7053418012614827, 4.999999999999999112 ) ) ;
#30642=CARTESIAN_POINT ( 'NONE',  ( 4.458734124999998549, -53.72916666530106511, -2.574251347313721627 ) ) ;
#30643=CARTESIAN_POINT ( 'NONE',  ( -4.458734124999997661, -32.47916666530106511, 2.574251347313722516 ) ) ;
#30645=( BOUNDED_CURVE ( )  B_SPLINE_CURVE ( 2, ( #59783, #58807, #54629, #53985, #15708, #50447, #5101, #10553, #24719 ),
 .UNSPECIFIED., .F., .F. ) 
 B_SPLINE_CURVE_WITH_KNOTS ( ( 3, 2, 2, 2, 3 ),
 ( 0.5339285714285714191, 0.5345238095238095122, 0.5357142857142856984, 0.5369047619047618847, 0.5374999999999999778 ),
 .UNSPECIFIED. ) 
 CURVE ( )  GEOMETRIC_REPRESENTATION_ITEM ( )  RATIONAL_B_SPLINE_CURVE ( ( 0.9330127018922194093, 0.9330127018922194093, 1.000000000000000000, 0.8660254037844387076, 1.000000000000000000, 0.8660254037844387076, 1.000000000000000000, 0.9330127018922194093, 0.9330127018922194093 ) ) 
 REPRESENTATION_ITEM ( '' )  );
#30647=CARTESIAN_POINT ( 'NONE',  ( -4.999999999999999112, 23.08333333333332860, 2.886751345948131764 ) ) ;
#30651=CARTESIAN_POINT ( 'NONE',  ( -4.458734124999998549, -40.22916666530107932, 2.574251347313722516 ) ) ;
#30652=CARTESIAN_POINT ( 'NONE',  ( -5.000000000000000000, -73.95833333060214443, -2.886751345948128211 ) ) ;
#30657=CARTESIAN_POINT ( 'NONE',  ( -4.458734124999997661, -78.47916666530106511, 2.574251347313722516 ) ) ;
#30660=DIRECTION ( 'NONE',  ( -0.000000000000000000, 1.000000000000000000, -0.000000000000000000 ) ) ;
#30661=CARTESIAN_POINT ( 'NONE',  ( -2.500000000000000444, -28.16666666666666785, -4.330127018922193649 ) ) ;
#30663=ORIENTED_EDGE ( 'NONE', *, *, #20453, .T. ) ;
#30666=EDGE_CURVE ( 'NONE', #15028, #2754, #2064, .T. ) ;
#30668=AXIS2_PLACEMENT_3D ( 'NONE', #49607, #44133, #48336 ) ;
#30669=CARTESIAN_POINT ( 'NONE',  ( 5.000000000000000000, 23.62500000273118417, -6.123233995736766282E-16 ) ) ;
#30672=AXIS2_PLACEMENT_3D ( 'NONE', #7910, #27515, #47145 ) ;
#30677=CARTESIAN_POINT ( 'NONE',  ( 1.339745962155615144, -1.705341801261478274, 4.999999999999999112 ) ) ;
#30678=CARTESIAN_POINT ( 'NONE',  ( -1.975475456537005874E-15, 28.37500000273118772, 5.000000000000000000 ) ) ;
#30682=CARTESIAN_POINT ( 'NONE',  ( -5.000000000000000000, -79.08333333333332860, -2.886751345948128211 ) ) ;
#30683=CARTESIAN_POINT ( 'NONE',  ( -4.458734124999999437, -13.64583333196774007, -2.574251347313719407 ) ) ;
#30687=ADVANCED_FACE ( 'NONE', ( #16146 ), #6188, .T. ) ;
#30691=CARTESIAN_POINT ( 'NONE',  ( 1.975475456537005874E-15, 13.37500000273118417, 5.000000000000000000 ) ) ;
#30694=CARTESIAN_POINT ( 'NONE',  ( -2.499999999999996447, -85.83333333333332860, 4.330127018922195425 ) ) ;
#30700=ORIENTED_EDGE ( 'NONE', *, *, #62327, .T. ) ;
#30702=CARTESIAN_POINT ( 'NONE',  ( 9.457646018065525792E-16, 11.93750000136559386, 5.148502694627439702 ) ) ;
#30707=CARTESIAN_POINT ( 'NONE',  ( 2.229367062500001939, -62.97916666530106511, 3.861377020970579999 ) ) ;
#30709=CARTESIAN_POINT ( 'NONE',  ( -4.458734124999999437, 14.60416666803226171, -2.574251347313719407 ) ) ;
#30710=AXIS2_PLACEMENT_3D ( 'NONE', #29970, #60541, #16463 ) ;
#30714=EDGE_CURVE ( 'NONE', #14857, #32214, #32848, .T. ) ;
#30715=CARTESIAN_POINT ( 'NONE',  ( -3.152548672688508926E-16, -55.81249999863440081, -5.148502694627439702 ) ) ;
#30716=CARTESIAN_POINT ( 'NONE',  ( -5.000000000000000000, -13.87499999726881228, 0.000000000000000000 ) ) ;
#30719=EDGE_CURVE ( 'NONE', #9561, #46354, #40582, .T. ) ;
#30720=CARTESIAN_POINT ( 'NONE',  ( 5.000000000000000888, -104.4583333306021586, 2.886751345948126879 ) ) ;
#30721=CARTESIAN_POINT ( 'NONE',  ( -2.229367062500000163, -16.72916666530107577, -3.861377020970580443 ) ) ;
#30722=EDGE_LOOP ( 'NONE', ( #38092, #61473, #53550, #59329 ) ) ;
#30723=CARTESIAN_POINT ( 'NONE',  ( 5.000000000000000000, 23.58333333333333215, -2.886751345948130876 ) ) ;
#30724=CARTESIAN_POINT ( 'NONE',  ( -4.458734124999999437, -106.3958333319677507, -2.574251347313719407 ) ) ;
#30727=CARTESIAN_POINT ( 'NONE',  ( -2.229367062499996610, -100.3958333319677365, 3.861377020970582219 ) ) ;
#30728=CARTESIAN_POINT ( 'NONE',  ( -4.458734124999998549, -27.22916666530107221, 2.574251347313722516 ) ) ;
#30729=CARTESIAN_POINT ( 'NONE',  ( 5.000000000000000888, -59.45833333060214443, 2.886751345948126879 ) ) ;
#30733=CARTESIAN_POINT ( 'NONE',  ( 4.458734124999999437, -23.81249999863440436, -5.460374474430324690E-16 ) ) ;
#30735=CARTESIAN_POINT ( 'NONE',  ( 4.458734124999998549, -61.97916666530106511, -2.574251347313721627 ) ) ;
#30736=CARTESIAN_POINT ( 'NONE',  ( 0.000000000000000000, -120.0000000000000000, 0.000000000000000000 ) ) ;
#30740=CARTESIAN_POINT ( 'NONE',  ( 5.000000000000000000, -11.41666666666666607, -2.886751345948129988 ) ) ;
#30745=CARTESIAN_POINT ( 'NONE',  ( -5.000000000000000000, -37.99999999999999289, 0.000000000000000000 ) ) ;
#30747=EDGE_CURVE ( 'NONE', #54588, #22588, #47938, .T. ) ;
#30750=CARTESIAN_POINT ( 'NONE',  ( -6.972266317189433020E-16, -57.12499999726880162, -5.000000000000000000 ) ) ;
#30754=CARTESIAN_POINT ( 'NONE',  ( -3.535250795749689387E-16, -78.25000000000001421, -5.773502691896257311 ) ) ;
#30759=LINE ( 'NONE', #50380, #17318 ) ;
#30769=CARTESIAN_POINT ( 'NONE',  ( 2.493747252781420335E-13, -55.24999999999999289, -5.000000000000000000 ) ) ;
#30770=VERTEX_POINT ( 'NONE', #27374 ) ;
#30774=ORIENTED_EDGE ( 'NONE', *, *, #23952, .F. ) ;
#30777=CARTESIAN_POINT ( 'NONE',  ( 4.458734125000001214, -74.89583333196773651, 2.574251347313718519 ) ) ;
#30778=CARTESIAN_POINT ( 'NONE',  ( 9.457646018065525792E-16, -109.3124999986343937, 5.148502694627439702 ) ) ;
#30780=ORIENTED_EDGE ( 'NONE', *, *, #48712, .F. ) ;
#30785=CARTESIAN_POINT ( 'NONE',  ( 2.229367062499998831, -42.64583333196773651, -3.861377020970580887 ) ) ;
#30788=CARTESIAN_POINT ( 'NONE',  ( -4.458734124999999437, -48.31249999863440792, 0.000000000000000000 ) ) ;
#30790=FACE_OUTER_BOUND ( 'NONE', #22373, .T. ) ;
#30791=CARTESIAN_POINT ( 'NONE',  ( 4.458734124999998549, -18.72916666530106866, -2.574251347313721627 ) ) ;
#30792=CARTESIAN_POINT ( 'NONE',  ( 5.000000000000000000, -103.5000000000000142, -6.123233995736766282E-16 ) ) ;
#30794=CARTESIAN_POINT ( 'NONE',  ( -4.458734124999998549, -37.47916666530107221, 2.574251347313722516 ) ) ;
#30795=CARTESIAN_POINT ( 'NONE',  ( -2.500000000000000444, 6.958333336064520758, -4.330127018922193649 ) ) ;
#30800=CARTESIAN_POINT ( 'NONE',  ( 5.000000000000000000, -30.29166666393547658, -2.886751345948130876 ) ) ;
#30801=CARTESIAN_POINT ( 'NONE',  ( 2.229367062499998831, 1.104166668032261711, -3.861377020970580887 ) ) ;
#30803=CARTESIAN_POINT ( 'NONE',  ( 5.000000000000000000, -30.41666666666666785, -2.886751345948130876 ) ) ;
#30804=CARTESIAN_POINT ( 'NONE',  ( 4.458734125000001214, -89.89583333196775072, 2.574251347313718519 ) ) ;
#30805=CARTESIAN_POINT ( 'NONE',  ( 4.458734124999999437, -32.81249999863440792, -5.460374474430324690E-16 ) ) ;
#30806=CYLINDRICAL_SURFACE ( 'NONE', #57277, 5.000000000000000000 ) ;
#30807=CARTESIAN_POINT ( 'NONE',  ( -4.458734124999999437, -80.64583333196773651, -2.574251347313719407 ) ) ;
#30812=CARTESIAN_POINT ( 'NONE',  ( -2.229367062500000163, -8.479166665301073991, -3.861377020970580443 ) ) ;
#30813=CARTESIAN_POINT ( 'NONE',  ( -4.458734124999998549, 21.52083333469893134, 2.574251347313722516 ) ) ;
#30814=CARTESIAN_POINT ( 'NONE',  ( -4.458734124999997661, -49.47916666530107221, 2.574251347313722516 ) ) ;
#30820=ORIENTED_EDGE ( 'NONE', *, *, #23259, .F. ) ;
#30823=EDGE_CURVE ( 'NONE', #6601, #45642, #4470, .T. ) ;
#30824=CARTESIAN_POINT ( 'NONE',  ( 4.458734125000001214, -72.89583333196775072, 2.574251347313718519 ) ) ;
#30825=CARTESIAN_POINT ( 'NONE',  ( -3.152548672688508926E-16, 29.18750000136559208, -5.148502694627439702 ) ) ;
#30831=CARTESIAN_POINT ( 'NONE',  ( 1.060575238724906964E-15, -60.75000000000000000, 5.773502691896257311 ) ) ;
#30835=( BOUNDED_CURVE ( )  B_SPLINE_CURVE ( 2, ( #31531, #22214, #41811, #61457, #50843, #35734, #51485, #27341, #51795 ),
 .UNSPECIFIED., .F., .F. ) 
 B_SPLINE_CURVE_WITH_KNOTS ( ( 3, 2, 2, 2, 3 ),
 ( 0.1660714285714285643, 0.1666666666666666574, 0.1678571428571428437, 0.1690476190476190577, 0.1696428571428571508 ),
 .UNSPECIFIED. ) 
 CURVE ( )  GEOMETRIC_REPRESENTATION_ITEM ( )  RATIONAL_B_SPLINE_CURVE ( ( 0.9330127018922194093, 0.9330127018922194093, 1.000000000000000000, 0.8660254037844387076, 1.000000000000000000, 0.8660254037844387076, 1.000000000000000000, 0.9330127018922194093, 0.9330127018922194093 ) ) 
 REPRESENTATION_ITEM ( '' )  );
#30836=CARTESIAN_POINT ( 'NONE',  ( 1.339745962155612702, -67.29465819873851729, -5.000000000000000000 ) ) ;
#30837=CARTESIAN_POINT ( 'NONE',  ( -2.500000000000000444, -107.0416666639354730, -4.330127018922193649 ) ) ;
#30843=ORIENTED_EDGE ( 'NONE', *, *, #61479, .F. ) ;
#30846=ORIENTED_EDGE ( 'NONE', *, *, #33485, .T. ) ;
#30849=VECTOR ( 'NONE', #12765, 1000.000000000000000 ) ;
#30850=CARTESIAN_POINT ( 'NONE',  ( 2.229367062500001939, -47.22916666530106511, 3.861377020970579999 ) ) ;
#30851=CARTESIAN_POINT ( 'NONE',  ( -5.000000000000000000, -15.95833333060214443, -2.886751345948128211 ) ) ;
#30853=CARTESIAN_POINT ( 'NONE',  ( -6.972266317189433020E-16, -38.12499999726880873, -5.000000000000000000 ) ) ;
#30858=CARTESIAN_POINT ( 'NONE',  ( -1.336351044127974539E-14, 22.24999999999999645, 5.000000000000000000 ) ) ;
#30860=CARTESIAN_POINT ( 'NONE',  ( 4.458734125000001214, -97.14583333196773651, 2.574251347313718519 ) ) ;
#30861=CARTESIAN_POINT ( 'NONE',  ( -1.339745962155613812, -107.2053418012614543, -5.000000000000000000 ) ) ;
#30863=CARTESIAN_POINT ( 'NONE',  ( -5.000000000000000000, 14.12500000273118594, 0.000000000000000000 ) ) ;
#30868=CARTESIAN_POINT ( 'NONE',  ( -4.458734124999998549, -3.229166665301069994, 2.574251347313722516 ) ) ;
#30870=CARTESIAN_POINT ( 'NONE',  ( -6.972266317189433020E-16, 22.87500000273118417, -5.000000000000000000 ) ) ;
#30871=CARTESIAN_POINT ( 'NONE',  ( 2.229367062500001939, -16.22916666530107577, 3.861377020970579999 ) ) ;
#30872=CARTESIAN_POINT ( 'NONE',  ( -1.339745962155613812, -101.0803417985302843, -5.000000000000000000 ) ) ;
#30876=( BOUNDED_CURVE ( )  B_SPLINE_CURVE ( 2, ( #1591, #16685, #36305, #31462, #62339, #47225, #56883, #47528, #24583 ),
 .UNSPECIFIED., .F., .F. ) 
 B_SPLINE_CURVE_WITH_KNOTS ( ( 3, 2, 2, 2, 3 ),
 ( 0.6589285714285714191, 0.6595238095238095122, 0.6607142857142856984, 0.6619047619047618847, 0.6624999999999999778 ),
 .UNSPECIFIED. ) 
 CURVE ( )  GEOMETRIC_REPRESENTATION_ITEM ( )  RATIONAL_B_SPLINE_CURVE ( ( 0.9330127018922194093, 0.9330127018922194093, 1.000000000000000000, 0.8660254037844387076, 1.000000000000000000, 0.8660254037844387076, 1.000000000000000000, 0.9330127018922194093, 0.9330127018922194093 ) ) 
 REPRESENTATION_ITEM ( '' )  );
#30877=CARTESIAN_POINT ( 'NONE',  ( -3.152548672688508926E-16, 16.18750000136559564, -5.148502694627439702 ) ) ;
#30879=CARTESIAN_POINT ( 'NONE',  ( 0.000000000000000000, -120.0000000000000000, 0.000000000000000000 ) ) ;
#30880=CARTESIAN_POINT ( 'NONE',  ( -6.972266317189433020E-16, -13.25000000000000000, -5.000000000000000000 ) ) ;
#30881=CARTESIAN_POINT ( 'NONE',  ( 4.458734124999998549, -19.72916666530107221, -2.574251347313721627 ) ) ;
#30884=CARTESIAN_POINT ( 'NONE',  ( 5.000000000000000000, -45.37499999726880873, -6.123233995736766282E-16 ) ) ;
#30886=CARTESIAN_POINT ( 'NONE',  ( -3.152548672688508926E-16, 7.437500001365594748, -5.148502694627439702 ) ) ;
#30887=CARTESIAN_POINT ( 'NONE',  ( 2.500000000000002220, -35.66666666666666430, 4.330127018922192761 ) ) ;
#30888=CARTESIAN_POINT ( 'NONE',  ( 1.975475456537005874E-15, -10.75000000000000000, 5.000000000000000000 ) ) ;
#30890=CARTESIAN_POINT ( 'NONE',  ( 4.458734125000001214, -65.89583333196772230, 2.574251347313718519 ) ) ;
#30893=CARTESIAN_POINT ( 'NONE',  ( -2.499999999999996447, 2.166666666666667407, 4.330127018922195425 ) ) ;
#30896=CIRCLE ( 'NONE', #29866, 5.000000000000000000 ) ;
#30897=CARTESIAN_POINT ( 'NONE',  ( 4.458734125000001214, -60.89583333196774362, 2.574251347313718519 ) ) ;
#30898=CARTESIAN_POINT ( 'NONE',  ( 5.000000000000000000, -96.29166666393547303, -2.886751345948129988 ) ) ;
#30900=CARTESIAN_POINT ( 'NONE',  ( 1.975475456537005874E-15, -79.74999999999998579, 5.000000000000000000 ) ) ;
#30904=CARTESIAN_POINT ( 'NONE',  ( 5.000000000000000000, -41.49999999999999289, -6.123233995736766282E-16 ) ) ;
#30905=CARTESIAN_POINT ( 'NONE',  ( 1.339745962155612702, -13.29465819873852084, -5.000000000000000000 ) ) ;
#30906=CARTESIAN_POINT ( 'NONE',  ( 2.500000000000002220, -6.541666663935481019, 4.330127018922192761 ) ) ;
#30908=CARTESIAN_POINT ( 'NONE',  ( -3.152548672688508926E-16, -107.5624999986343795, -5.148502694627439702 ) ) ;
#30909=CARTESIAN_POINT ( 'NONE',  ( -2.229367062499996610, -0.3958333319677397322, 3.861377020970582219 ) ) ;
#30910=CARTESIAN_POINT ( 'NONE',  ( -6.972266317189433020E-16, -73.12499999726878741, -5.000000000000000000 ) ) ;
#30913=LINE ( 'NONE', #45070, #8229 ) ;
#30916=ORIENTED_EDGE ( 'NONE', *, *, #38902, .T. ) ;
#30919=ORIENTED_EDGE ( 'NONE', *, *, #43708, .T. ) ;
#30921=CARTESIAN_POINT ( 'NONE',  ( -2.229367062499996610, -30.39583333196773651, 3.861377020970582219 ) ) ;
#30926=ADVANCED_FACE ( 'NONE', ( #57479 ), #61982, .T. ) ;
#30931=ORIENTED_EDGE ( 'NONE', *, *, #40797, .T. ) ;
#30932=CARTESIAN_POINT ( 'NONE',  ( 9.457646018065525792E-16, -76.31249999863439371, 5.148502694627439702 ) ) ;
#30936=FACE_OUTER_BOUND ( 'NONE', #11475, .T. ) ;
#30939=CARTESIAN_POINT ( 'NONE',  ( 4.458734124999999437, -5.062499998634402587, -5.460374474430324690E-16 ) ) ;
#30941=CARTESIAN_POINT ( 'NONE',  ( -1.339745962155610925, -9.669658196007334894, 5.000000000000000000 ) ) ;
#30943=ORIENTED_EDGE ( 'NONE', *, *, #15730, .F. ) ;
#30944=CARTESIAN_POINT ( 'NONE',  ( 0.000000000000000000, -120.0000000000000000, 5.000000000000000000 ) ) ;
#30946=CARTESIAN_POINT ( 'NONE',  ( 2.500000000000002220, -64.66666666666665719, 4.330127018922192761 ) ) ;
#30949=VERTEX_POINT ( 'NONE', #17901 ) ;
#30950=CARTESIAN_POINT ( 'NONE',  ( -4.458734124999999437, -81.39583333196773651, -2.574251347313719407 ) ) ;
#30951=CARTESIAN_POINT ( 'NONE',  ( 1.339745962155612702, -75.29465819873853150, -5.000000000000000000 ) ) ;
#30952=CARTESIAN_POINT ( 'NONE',  ( 2.229367062500001939, -3.979166665301070438, 3.861377020970579999 ) ) ;
#30956=CARTESIAN_POINT ( 'NONE',  ( -2.229367062500000163, -68.72916666530107932, -3.861377020970580443 ) ) ;
#30957=CARTESIAN_POINT ( 'NONE',  ( 5.000000000000000000, -29.29166666393547658, -2.886751345948129988 ) ) ;
#30959=CARTESIAN_POINT ( 'NONE',  ( -4.458734124999997661, 28.77083333469892779, 2.574251347313722516 ) ) ;
#30960=CARTESIAN_POINT ( 'NONE',  ( -1.339745962155669101, -37.66965819600733312, 4.999999999999966249 ) ) ;
#30962=CARTESIAN_POINT ( 'NONE',  ( -4.458734124999999437, -52.39583333196773651, -2.574251347313719407 ) ) ;
#30963=CARTESIAN_POINT ( 'NONE',  ( 2.229367062499998831, -29.89583333196773296, -3.861377020970580887 ) ) ;
#30966=CARTESIAN_POINT ( 'NONE',  ( -2.500000000000000444, 22.83333333333333215, -4.330127018922193649 ) ) ;
#30969=CARTESIAN_POINT ( 'NONE',  ( 4.458734125000001214, -41.89583333196773651, 2.574251347313718519 ) ) ;
#30970=CARTESIAN_POINT ( 'NONE',  ( 5.000000000000000000, -77.37499999726881583, -6.123233995736766282E-16 ) ) ;
#30974=CARTESIAN_POINT ( 'NONE',  ( -4.458734124999997661, -80.47916666530105090, 2.574251347313722516 ) ) ;
#30976=CARTESIAN_POINT ( 'NONE',  ( 2.500000000000002220, 13.45833333606451987, 4.330127018922192761 ) ) ;
#30977=CARTESIAN_POINT ( 'NONE',  ( -2.500000000000000444, -25.16666666666666430, -4.330127018922193649 ) ) ;
#30982=CARTESIAN_POINT ( 'NONE',  ( -3.152548672688508926E-16, 13.18750000136559208, -5.148502694627439702 ) ) ;
#30983=CARTESIAN_POINT ( 'NONE',  ( 5.000000000000000000, 16.70833333606451987, -2.886751345948129988 ) ) ;
#30984=CARTESIAN_POINT ( 'NONE',  ( -4.999999999999998224, -60.79166666393547303, 2.886751345948131764 ) ) ;
#30991=CARTESIAN_POINT ( 'NONE',  ( 1.339745962155615144, -89.58034179853028434, 4.999999999999999112 ) ) ;
#30992=CARTESIAN_POINT ( 'NONE',  ( 1.975475456537005874E-15, -61.74999999999999289, 5.000000000000000000 ) ) ;
#30996=CARTESIAN_POINT ( 'NONE',  ( -2.229367062500000163, -15.72916666530107399, -3.861377020970580443 ) ) ;
#31004=ORIENTED_EDGE ( 'NONE', *, *, #35811, .T. ) ;
#31005=CARTESIAN_POINT ( 'NONE',  ( 5.000000000000000000, -21.41666666666666430, -2.886751345948130876 ) ) ;
#31006=CARTESIAN_POINT ( 'NONE',  ( 1.243387493232115550E-13, -8.250000000000003553, -5.000000000000000000 ) ) ;
#31008=EDGE_LOOP ( 'NONE', ( #3243, #24839, #43191, #50039 ) ) ;
#31011=CARTESIAN_POINT ( 'NONE',  ( 2.500000000000002220, 15.33333333333333215, 4.330127018922192761 ) ) ;
#31014=LINE ( 'NONE', #50964, #58355 ) ;
#31016=CARTESIAN_POINT ( 'NONE',  ( 2.229367062500001939, 16.02083333469892779, 3.861377020970579999 ) ) ;
#31019=CARTESIAN_POINT ( 'NONE',  ( 2.500000000000002220, -78.54166666393547303, 4.330127018922192761 ) ) ;
#31023=CARTESIAN_POINT ( 'NONE',  ( -3.152548672688508926E-16, -66.56249999863440792, -5.148502694627439702 ) ) ;
#31024=CARTESIAN_POINT ( 'NONE',  ( 6.123233995736766282E-16, -120.0000000000000000, -5.000000000000000000 ) ) ;
#31025=CARTESIAN_POINT ( 'NONE',  ( -4.458734124999999437, 10.68750000136559386, 0.000000000000000000 ) ) ;
#31027=CARTESIAN_POINT ( 'NONE',  ( -5.000000000000000000, -69.95833333060214443, -2.886751345948128211 ) ) ;
#31029=CARTESIAN_POINT ( 'NONE',  ( -4.458734124999999437, -52.64583333196773651, -2.574251347313719407 ) ) ;
#31030=CARTESIAN_POINT ( 'NONE',  ( -4.999999999999999112, -14.79166666393548368, 2.886751345948131764 ) ) ;
#31033=DIRECTION ( 'NONE',  ( -0.5000000000000009992, 0.000000000000000000, -0.8660254037844380415 ) ) ;
#31035=CARTESIAN_POINT ( 'NONE',  ( 2.229367062499998831, -15.89583333196773651, -3.861377020970580887 ) ) ;
#31038=CARTESIAN_POINT ( 'NONE',  ( -3.152548672688508926E-16, -105.5624999986344079, -5.148502694627439702 ) ) ;
#31041=CARTESIAN_POINT ( 'NONE',  ( 9.457646018065525792E-16, -103.3124999986344079, 5.148502694627439702 ) ) ;
#31042=CARTESIAN_POINT ( 'NONE',  ( 4.458734125000001214, -25.89583333196774007, 2.574251347313718519 ) ) ;
#31043=CARTESIAN_POINT ( 'NONE',  ( 2.500000000000002220, -61.54166666393547303, 4.330127018922192761 ) ) ;
#31046=EDGE_CURVE ( 'NONE', #38768, #10267, #13196, .T. ) ;
#31047=CARTESIAN_POINT ( 'NONE',  ( 2.229367062499998831, -21.64583333196774007, -3.861377020970580887 ) ) ;
#31048=CARTESIAN_POINT ( 'NONE',  ( 2.229367062499998831, -63.89583333196772941, -3.861377020970580887 ) ) ;
#31049=CARTESIAN_POINT ( 'NONE',  ( -5.926426369611017623E-15, 25.37500000273118062, 5.000000000000000000 ) ) ;
#31053=CARTESIAN_POINT ( 'NONE',  ( -5.000000000000000000, -14.08333333333333037, -2.886751345948128211 ) ) ;
#31057=( BOUNDED_CURVE ( )  B_SPLINE_CURVE ( 2, ( #47789, #14008, #13699, #8876, #28803, #3434, #42969, #33321, #28490 ),
 .UNSPECIFIED., .F., .F. ) 
 B_SPLINE_CURVE_WITH_KNOTS ( ( 3, 2, 2, 2, 3 ),
 ( 0.9089285714285714191, 0.9095238095238095122, 0.9107142857142856984, 0.9119047619047618847, 0.9124999999999999778 ),
 .UNSPECIFIED. ) 
 CURVE ( )  GEOMETRIC_REPRESENTATION_ITEM ( )  RATIONAL_B_SPLINE_CURVE ( ( 0.9330127018922194093, 0.9330127018922194093, 1.000000000000000000, 0.8660254037844387076, 1.000000000000000000, 0.8660254037844387076, 1.000000000000000000, 0.9330127018922194093, 0.9330127018922194093 ) ) 
 REPRESENTATION_ITEM ( '' )  );
#31058=CARTESIAN_POINT ( 'NONE',  ( 2.499999999999998668, 21.79166666939785202, -4.330127018922193649 ) ) ;
#31059=CARTESIAN_POINT ( 'NONE',  ( 5.000000000000000000, -90.50000000000000000, -6.123233995736766282E-16 ) ) ;
#31064=PLANE ( 'NONE',  #13952 ) ;
#31066=CARTESIAN_POINT ( 'NONE',  ( 2.499999999999998668, -81.33333333333332860, -4.330127018922193649 ) ) ;
#31074=ADVANCED_FACE ( 'NONE', ( #18836 ), #18540, .T. ) ;
#31075=ADVANCED_FACE ( 'NONE', ( #34570 ), #29109, .T. ) ;
#31078=ORIENTED_EDGE ( 'NONE', *, *, #16562, .T. ) ;
#31080=ORIENTED_EDGE ( 'NONE', *, *, #34729, .T. ) ;
#31085=ORIENTED_EDGE ( 'NONE', *, *, #46502, .T. ) ;
#31091=CARTESIAN_POINT ( 'NONE',  ( 4.458734124999998549, -74.72916666530106511, -2.574251347313721627 ) ) ;
#31093=CARTESIAN_POINT ( 'NONE',  ( 4.458734125000001214, -108.1458333319677365, 2.574251347313718519 ) ) ;
#31094=CARTESIAN_POINT ( 'NONE',  ( -6.972266317189433020E-16, -108.1249999972688016, -5.000000000000000000 ) ) ;
#31100=CARTESIAN_POINT ( 'NONE',  ( -2.229367062500000163, -45.47916666530106511, -3.861377020970580443 ) ) ;
#31103=CARTESIAN_POINT ( 'NONE',  ( 2.229367062499998831, -50.64583333196772941, -3.861377020970580887 ) ) ;
#31105=CARTESIAN_POINT ( 'NONE',  ( -4.458734124999999437, 26.68750000136559564, 0.000000000000000000 ) ) ;
#31106=CARTESIAN_POINT ( 'NONE',  ( -4.458734124999999437, -17.39583333196773651, -2.574251347313719407 ) ) ;
#31107=CARTESIAN_POINT ( 'NONE',  ( 2.500000000000002220, -103.6666666666666572, 4.330127018922192761 ) ) ;
#31108=CARTESIAN_POINT ( 'NONE',  ( 4.458734124999998549, -39.97916666530107221, -2.574251347313721627 ) ) ;
#31109=CARTESIAN_POINT ( 'NONE',  ( -5.000000000000000000, 3.041666669397851130, -2.886751345948128211 ) ) ;
#31114=CARTESIAN_POINT ( 'NONE',  ( 4.458734125000000326, -97.89583333196773651, 2.574251347313718519 ) ) ;
#31116=CARTESIAN_POINT ( 'NONE',  ( -4.458734124999999437, -2.645833331967738289, -2.574251347313719407 ) ) ;
#31117=VERTEX_POINT ( 'NONE', #14013 ) ;
#31119=CARTESIAN_POINT ( 'NONE',  ( 1.975475456537005874E-15, -75.74999999999998579, 5.000000000000000000 ) ) ;
#31120=CARTESIAN_POINT ( 'NONE',  ( 4.458734124999999437, -85.81249999863439371, -5.460374474430324690E-16 ) ) ;
#31122=CARTESIAN_POINT ( 'NONE',  ( 4.458734124999999437, -86.06249999863439371, -5.460374474430324690E-16 ) ) ;
#31126=CARTESIAN_POINT ( 'NONE',  ( -4.458734124999999437, -5.312499998634402587, 0.000000000000000000 ) ) ;
#31127=CARTESIAN_POINT ( 'NONE',  ( -4.458734124999998549, 16.52083333469892779, 2.574251347313722516 ) ) ;
#31128=CARTESIAN_POINT ( 'NONE',  ( -3.152548672688508926E-16, -49.81249999863440081, -5.148502694627439702 ) ) ;
#31135=CARTESIAN_POINT ( 'NONE',  ( 4.458734124999999437, -74.81249999863440792, -5.460374474430324690E-16 ) ) ;
#31136=CARTESIAN_POINT ( 'NONE',  ( -4.458734124999998549, 27.52083333469892779, 2.574251347313722516 ) ) ;
#31137=( BOUNDED_CURVE ( )  B_SPLINE_CURVE ( 2, ( #53662, #18627, #53032, #63323, #44318, #38250, #24085, #9596, #23773 ),
 .UNSPECIFIED., .F., .F. ) 
 B_SPLINE_CURVE_WITH_KNOTS ( ( 3, 2, 2, 2, 3 ),
 ( 0.9339285714285714413, 0.9345238095238095344, 0.9357142857142857206, 0.9369047619047619069, 0.9375000000000000000 ),
 .UNSPECIFIED. ) 
 CURVE ( )  GEOMETRIC_REPRESENTATION_ITEM ( )  RATIONAL_B_SPLINE_CURVE ( ( 0.9330127018922194093, 0.9330127018922194093, 1.000000000000000000, 0.8660254037844387076, 1.000000000000000000, 0.8660254037844387076, 1.000000000000000000, 0.9330127018922194093, 0.9330127018922194093 ) ) 
 REPRESENTATION_ITEM ( '' )  );
#31142=CARTESIAN_POINT ( 'NONE',  ( -2.499999999999996447, -63.83333333333332860, 4.330127018922195425 ) ) ;
#31145=ORIENTED_EDGE ( 'NONE', *, *, #22740, .T. ) ;
#31146=CARTESIAN_POINT ( 'NONE',  ( 5.000000000000000000, 7.500000000000000000, -6.123233995736766282E-16 ) ) ;
#31151=( BOUNDED_CURVE ( )  B_SPLINE_CURVE ( 2, ( #7330, #3131, #26941, #16968, #46557, #56848, #41708, #56211, #61357 ),
 .UNSPECIFIED., .F., .F. ) 
 B_SPLINE_CURVE_WITH_KNOTS ( ( 3, 2, 2, 2, 3 ),
 ( 0.4625000000000000222, 0.4630952380952381153, 0.4642857142857143016, 0.4654761904761904878, 0.4660714285714285809 ),
 .UNSPECIFIED. ) 
 CURVE ( )  GEOMETRIC_REPRESENTATION_ITEM ( )  RATIONAL_B_SPLINE_CURVE ( ( 0.9330127018922194093, 0.9330127018922194093, 1.000000000000000000, 0.8660254037844387076, 1.000000000000000000, 0.8660254037844387076, 1.000000000000000000, 0.9330127018922194093, 0.9330127018922194093 ) ) 
 REPRESENTATION_ITEM ( '' )  );
#31155=ORIENTED_EDGE ( 'NONE', *, *, #33485, .F. ) ;
#31156=CARTESIAN_POINT ( 'NONE',  ( -6.972266317189433020E-16, -105.1249999972688016, -5.000000000000000000 ) ) ;
#31159=ORIENTED_EDGE ( 'NONE', *, *, #51152, .F. ) ;
#31162=CARTESIAN_POINT ( 'NONE',  ( -2.229367062499996610, -45.39583333196774362, 3.861377020970582219 ) ) ;
#31166=CARTESIAN_POINT ( 'NONE',  ( 0.000000000000000000, -120.0000000000000000, 0.000000000000000000 ) ) ;
#31168=EDGE_CURVE ( 'NONE', #37025, #19133, #29419, .T. ) ;
#31171=CARTESIAN_POINT ( 'NONE',  ( -5.000000000000000000, -58.95833333060213732, -2.886751345948128211 ) ) ;
#31173=CARTESIAN_POINT ( 'NONE',  ( -3.152548672688508926E-16, -93.81249999863440792, -5.148502694627439702 ) ) ;
#31174=LINE ( 'NONE', #327, #60534 ) ;
#31176=EDGE_CURVE ( 'NONE', #12980, #22037, #43591, .T. ) ;
#31182=CARTESIAN_POINT ( 'NONE',  ( -4.458734124999999437, -1.395833331967737179, -2.574251347313719407 ) ) ;
#31185=CARTESIAN_POINT ( 'NONE',  ( 2.229367062499998831, -23.89583333196773651, -3.861377020970580887 ) ) ;
#31186=CARTESIAN_POINT ( 'NONE',  ( 1.339745962155499015, -72.70534180126148271, 5.000000000000065725 ) ) ;
#31188=CARTESIAN_POINT ( 'NONE',  ( 1.464175926609780648E-14, 23.87500000273118417, -5.000000000000000000 ) ) ;
#31190=CARTESIAN_POINT ( 'NONE',  ( 4.458734124999999437, 14.93750000136559386, -5.460374474430324690E-16 ) ) ;
#31193=CARTESIAN_POINT ( 'NONE',  ( 1.339745962155612702, -57.16965819600733312, -5.000000000000000000 ) ) ;
#31194=CARTESIAN_POINT ( 'NONE',  ( -4.999999999999999112, -87.91666666666667140, 2.886751345948131764 ) ) ;
#31195=CARTESIAN_POINT ( 'NONE',  ( -2.229367062500000163, -21.47916666530107221, -3.861377020970580443 ) ) ;
#31196=LINE ( 'NONE', #21560, #41681 ) ;
#31199=CARTESIAN_POINT ( 'NONE',  ( 2.499999999999998668, -45.20833333060214443, -4.330127018922193649 ) ) ;
#31200=CARTESIAN_POINT ( 'NONE',  ( -4.999999999999998224, -1.791666663935480353, 2.886751345948131764 ) ) ;
#31201=CARTESIAN_POINT ( 'NONE',  ( -2.229367062499996610, 5.854166668032262599, 3.861377020970582219 ) ) ;
#31202=DIRECTION ( 'NONE',  ( -0.000000000000000000, 1.000000000000000000, -0.000000000000000000 ) ) ;
#31203=CARTESIAN_POINT ( 'NONE',  ( 0.000000000000000000, -120.0000000000000000, 0.000000000000000000 ) ) ;
#31205=CARTESIAN_POINT ( 'NONE',  ( 4.458734125000001214, -69.89583333196773651, 2.574251347313718519 ) ) ;
#31208=CARTESIAN_POINT ( 'NONE',  ( 5.000000000000000888, -2.583333333333333481, 2.886751345948126879 ) ) ;
#31210=CARTESIAN_POINT ( 'NONE',  ( 6.123233995736766282E-16, -120.0000000000000000, -5.000000000000000000 ) ) ;
#31211=CARTESIAN_POINT ( 'NONE',  ( 9.457646018065525792E-16, -61.06249999863440081, 5.148502694627439702 ) ) ;
#31212=CARTESIAN_POINT ( 'NONE',  ( -4.999999999999999112, -96.79166666393545881, 2.886751345948131764 ) ) ;
#31213=CARTESIAN_POINT ( 'NONE',  ( -6.972266317189433020E-16, -70.25000000000000000, -5.000000000000000000 ) ) ;
#31216=CARTESIAN_POINT ( 'NONE',  ( -2.500000000000000444, -91.04166666393547303, -4.330127018922193649 ) ) ;
#31217=CARTESIAN_POINT ( 'NONE',  ( -2.499999999999996447, -46.83333333333333570, 4.330127018922195425 ) ) ;
#31219=ORIENTED_EDGE ( 'NONE', *, *, #37856, .F. ) ;
#31220=CARTESIAN_POINT ( 'NONE',  ( -2.229367062499996610, -104.1458333319677365, 3.861377020970582219 ) ) ;
#31221=CARTESIAN_POINT ( 'NONE',  ( -2.229367062500000163, -1.729166665301071992, -3.861377020970580443 ) ) ;
#31225=EDGE_CURVE ( 'NONE', #35143, #62889, #6181, .T. ) ;
#31229=ORIENTED_EDGE ( 'NONE', *, *, #62998, .F. ) ;
#31230=CARTESIAN_POINT ( 'NONE',  ( -2.499999999999996447, -16.70833333060214443, 4.330127018922195425 ) ) ;
#31232=ORIENTED_EDGE ( 'NONE', *, *, #59043, .T. ) ;
#31233=CARTESIAN_POINT ( 'NONE',  ( -1.339745962155613812, -49.08034179853029144, -5.000000000000000000 ) ) ;
#31235=CARTESIAN_POINT ( 'NONE',  ( -4.458734124999999437, -28.64583333196774007, -2.574251347313719407 ) ) ;
#31236=CARTESIAN_POINT ( 'NONE',  ( -6.972266317189433020E-16, -10.12499999726881406, -5.000000000000000000 ) ) ;
#31243=ORIENTED_EDGE ( 'NONE', *, *, #3156, .F. ) ;
#31244=CARTESIAN_POINT ( 'NONE',  ( -4.458734124999999437, -79.56249999863440792, 0.000000000000000000 ) ) ;
#31246=ORIENTED_EDGE ( 'NONE', *, *, #21146, .T. ) ;
#31250=CARTESIAN_POINT ( 'NONE',  ( -4.458734124999998549, -8.479166665301073991, 2.574251347313722516 ) ) ;
#31251=ORIENTED_EDGE ( 'NONE', *, *, #43417, .F. ) ;
#31254=ORIENTED_EDGE ( 'NONE', *, *, #49262, .T. ) ;
#31255=CARTESIAN_POINT ( 'NONE',  ( 2.229367062500001939, -7.229166665301073103, 3.861377020970579999 ) ) ;
#31258=CARTESIAN_POINT ( 'NONE',  ( -2.499999999999996447, -11.70833333060214798, 4.330127018922195425 ) ) ;
#31260=CARTESIAN_POINT ( 'NONE',  ( -4.458734124999999437, 29.35416666803225993, -2.574251347313719407 ) ) ;
#31262=CARTESIAN_POINT ( 'NONE',  ( -4.458734124999999437, -84.31249999863439371, 0.000000000000000000 ) ) ;
#31263=CARTESIAN_POINT ( 'NONE',  ( -4.458734124999999437, -2.312499998634407028, 0.000000000000000000 ) ) ;
#31265=VECTOR ( 'NONE', #28703, 1000.000000000000000 ) ;
#31266=CARTESIAN_POINT ( 'NONE',  ( 2.500000000000002220, -29.54166666393548013, 4.330127018922192761 ) ) ;
#31268=CARTESIAN_POINT ( 'NONE',  ( -2.229367062500000163, 24.52083333469892779, -3.861377020970580443 ) ) ;
#31271=CARTESIAN_POINT ( 'NONE',  ( 4.458734124999998549, -49.72916666530106511, -2.574251347313721627 ) ) ;
#31272=CARTESIAN_POINT ( 'NONE',  ( -2.229367062499996610, -37.39583333196773651, 3.861377020970582219 ) ) ;
#31275=CARTESIAN_POINT ( 'NONE',  ( 2.500000000000002220, 17.33333333333333215, 4.330127018922192761 ) ) ;
#31277=LINE ( 'NONE', #16811, #18182 ) ;
#31278=CARTESIAN_POINT ( 'NONE',  ( 4.458734124999999437, -44.81249999863440081, -5.460374474430324690E-16 ) ) ;
#31279=CARTESIAN_POINT ( 'NONE',  ( -2.500000000000000444, -79.04166666393547303, -4.330127018922193649 ) ) ;
#31283=CARTESIAN_POINT ( 'NONE',  ( -2.229367062499996610, -86.39583333196773651, 3.861377020970582219 ) ) ;
#31286=CARTESIAN_POINT ( 'NONE',  ( 5.000000000000000888, -25.58333333333333215, 2.886751345948126879 ) ) ;
#31290=ORIENTED_EDGE ( 'NONE', *, *, #46703, .F. ) ;
#31291=CARTESIAN_POINT ( 'NONE',  ( -3.152548672688508926E-16, -91.56249999863440792, -5.148502694627439702 ) ) ;
#31292=CARTESIAN_POINT ( 'NONE',  ( 4.458734124999998549, 15.02083333469892601, -2.574251347313721627 ) ) ;
#31293=CARTESIAN_POINT ( 'NONE',  ( -3.535250795749689387E-16, 18.87500000273118772, -5.773502691896257311 ) ) ;
#31301=CARTESIAN_POINT ( 'NONE',  ( 2.499999999999998668, -33.20833333060215153, -4.330127018922193649 ) ) ;
#31302=CARTESIAN_POINT ( 'NONE',  ( 2.499999999999998668, -11.20833333060214798, -4.330127018922193649 ) ) ;
#31306=CARTESIAN_POINT ( 'NONE',  ( -1.339745962155610925, -42.79465819873851729, 5.000000000000000000 ) ) ;
#31307=CARTESIAN_POINT ( 'NONE',  ( -4.458734124999998549, -14.47916666530107221, 2.574251347313722516 ) ) ;
#31319=CARTESIAN_POINT ( 'NONE',  ( 4.458734124999999437, -64.06249999863440792, -5.460374474430324690E-16 ) ) ;
#31321=CARTESIAN_POINT ( 'NONE',  ( 2.500000000000002220, 11.45833333606451809, 4.330127018922192761 ) ) ;
#31330=CARTESIAN_POINT ( 'NONE',  ( 2.229367062500001939, 11.02083333469892956, 3.861377020970579999 ) ) ;
#31335=CARTESIAN_POINT ( 'NONE',  ( -4.458734124999999437, -71.39583333196773651, -2.574251347313719407 ) ) ;
#31337=CARTESIAN_POINT ( 'NONE',  ( -4.458734124999999437, 12.68750000136559564, 0.000000000000000000 ) ) ;
#31338=CARTESIAN_POINT ( 'NONE',  ( 2.500000000000002220, 7.458333336064517205, 4.330127018922192761 ) ) ;
#31340=CARTESIAN_POINT ( 'NONE',  ( -4.458734124999999437, -52.56249999863440792, 0.000000000000000000 ) ) ;
#31341=CARTESIAN_POINT ( 'NONE',  ( -5.000000000000000000, -12.87499999726881050, 0.000000000000000000 ) ) ;
#31343=CARTESIAN_POINT ( 'NONE',  ( 4.458734125000000326, -20.14583333196774007, 2.574251347313718519 ) ) ;
#31344=ORIENTED_EDGE ( 'NONE', *, *, #787, .T. ) ;
#31346=CARTESIAN_POINT ( 'NONE',  ( 4.458734125000001214, -102.8958333319677365, 2.574251347313718519 ) ) ;
#31349=CARTESIAN_POINT ( 'NONE',  ( -3.152548672688508926E-16, -104.8124999986344079, -5.148502694627439702 ) ) ;
#31351=CARTESIAN_POINT ( 'NONE',  ( 2.229367062500001939, -27.97916666530107221, 3.861377020970579999 ) ) ;
#31352=CARTESIAN_POINT ( 'NONE',  ( -5.000000000000000000, -64.87499999726881583, 0.000000000000000000 ) ) ;
#31353=VECTOR ( 'NONE', #44368, 1000.000000000000000 ) ;
#31356=CARTESIAN_POINT ( 'NONE',  ( 2.229367062500001939, -24.97916666530106866, 3.861377020970579999 ) ) ;
#31357=CARTESIAN_POINT ( 'NONE',  ( -4.458734124999999437, -64.64583333196773651, -2.574251347313719407 ) ) ;
#31360=CARTESIAN_POINT ( 'NONE',  ( 4.330127018922258486, 45.00000000000000000, 7.499999999999910294 ) ) ;
#31362=CARTESIAN_POINT ( 'NONE',  ( 5.000000000000000000, -10.41666666666666430, -2.886751345948129988 ) ) ;
#31366=CARTESIAN_POINT ( 'NONE',  ( 1.975475456537005874E-15, -86.62499999726880162, 5.000000000000000000 ) ) ;
#31374=CARTESIAN_POINT ( 'NONE',  ( 5.000000000000000000, -95.37499999726881583, -6.123233995736766282E-16 ) ) ;
#31375=CYLINDRICAL_SURFACE ( 'NONE', #2681, 5.000000000000000000 ) ;
#31380=CARTESIAN_POINT ( 'NONE',  ( -6.972266317189433020E-16, -23.12499999726880873, -5.000000000000000000 ) ) ;
#31387=ORIENTED_EDGE ( 'NONE', *, *, #62040, .T. ) ;
#31396=CARTESIAN_POINT ( 'NONE',  ( -6.972266317189433020E-16, 20.74999999999999645, -5.000000000000000000 ) ) ;
#31397=VERTEX_POINT ( 'NONE', #44547 ) ;
#31398=EDGE_CURVE ( 'NONE', #18523, #1698, #20756, .T. ) ;
#31399=CARTESIAN_POINT ( 'NONE',  ( -4.458734124999999437, -76.31249999863440792, 0.000000000000000000 ) ) ;
#31400=CARTESIAN_POINT ( 'NONE',  ( 4.458734124999999437, 28.18750000136559208, -5.460374474430324690E-16 ) ) ;
#31401=CARTESIAN_POINT ( 'NONE',  ( -6.972266317189433020E-16, -54.24999999999999289, -5.000000000000000000 ) ) ;
#31403=CARTESIAN_POINT ( 'NONE',  ( 1.975475456537005874E-15, 5.375000002731185944, 5.000000000000000000 ) ) ;
#31410=CARTESIAN_POINT ( 'NONE',  ( 2.229367062499998831, -48.64583333196772941, -3.861377020970580887 ) ) ;
#31412=CARTESIAN_POINT ( 'NONE',  ( 9.457646018065525792E-16, 26.93750000136559564, 5.148502694627439702 ) ) ;
#31413=CARTESIAN_POINT ( 'NONE',  ( -2.500000000000000444, -108.1666666666666572, -4.330127018922193649 ) ) ;
#31414=LINE ( 'NONE', #61664, #5277 ) ;
#31415=CARTESIAN_POINT ( 'NONE',  ( -4.458734124999999437, -38.64583333196772941, -2.574251347313719407 ) ) ;
#31416=CARTESIAN_POINT ( 'NONE',  ( -4.999999999999999112, 3.208333336064520758, 2.886751345948131764 ) ) ;
#31420=CARTESIAN_POINT ( 'NONE',  ( 5.000000000000000888, -71.58333333333332860, 2.886751345948126879 ) ) ;
#31421=CARTESIAN_POINT ( 'NONE',  ( -4.458734124999997661, -98.22916666530103669, 2.574251347313722516 ) ) ;
#31423=CARTESIAN_POINT ( 'NONE',  ( 9.457646018065525792E-16, -5.312499998634401699, 5.148502694627439702 ) ) ;
#31424=EDGE_LOOP ( 'NONE', ( #27987, #60364, #14436, #4520 ) ) ;
#31425=CARTESIAN_POINT ( 'NONE',  ( -6.972266317189433020E-16, -68.12499999726881583, -5.000000000000000000 ) ) ;
#31426=CARTESIAN_POINT ( 'NONE',  ( -1.339745962155610925, -85.66965819600731891, 5.000000000000000000 ) ) ;
#31427=CARTESIAN_POINT ( 'NONE',  ( 9.457646018065525792E-16, -88.06249999863439371, 5.148502694627439702 ) ) ;
#31429=CARTESIAN_POINT ( 'NONE',  ( 2.229367062499998831, -87.89583333196773651, -3.861377020970580887 ) ) ;
#31432=LINE ( 'NONE', #40454, #27410 ) ;
#31434=CARTESIAN_POINT ( 'NONE',  ( 2.229367062499998831, -6.645833331967741842, -3.861377020970580887 ) ) ;
#31435=CARTESIAN_POINT ( 'NONE',  ( -2.229367062499996610, 17.60416666803225993, 3.861377020970582219 ) ) ;
#31436=CARTESIAN_POINT ( 'NONE',  ( -4.458734124999999437, -50.56249999863440792, 0.000000000000000000 ) ) ;
#31440=EDGE_LOOP ( 'NONE', ( #8319, #27262, #2954, #16464 ) ) ;
#31444=CARTESIAN_POINT ( 'NONE',  ( -4.458734124999999437, -72.31249999863439371, 0.000000000000000000 ) ) ;
#31445=CARTESIAN_POINT ( 'NONE',  ( -2.500000000000000444, -109.0416666639354730, -4.330127018922193649 ) ) ;
#31449=CARTESIAN_POINT ( 'NONE',  ( -4.999999999999998224, -93.91666666666665719, 2.886751345948131764 ) ) ;
#31453=CARTESIAN_POINT ( 'NONE',  ( -2.499999999999996447, -66.83333333333332860, 4.330127018922195425 ) ) ;
#31456=ORIENTED_EDGE ( 'NONE', *, *, #30003, .T. ) ;
#31458=CARTESIAN_POINT ( 'NONE',  ( -1.339745962155610925, 9.205341801261479162, 5.000000000000000000 ) ) ;
#31462=CARTESIAN_POINT ( 'NONE',  ( 5.000000000000000000, -62.41666666666666430, -2.886751345948130876 ) ) ;
#31465=VERTEX_POINT ( 'NONE', #12374 ) ;
#31467=CARTESIAN_POINT ( 'NONE',  ( 5.000000000000000000, -59.37499999726880873, -6.123233995736766282E-16 ) ) ;
#31469=ORIENTED_EDGE ( 'NONE', *, *, #15773, .T. ) ;
#31472=CARTESIAN_POINT ( 'NONE',  ( 2.229367062499998831, -47.89583333196774362, -3.861377020970580887 ) ) ;
#31475=CARTESIAN_POINT ( 'NONE',  ( -1.339745962155613812, -82.08034179853031276, -5.000000000000000000 ) ) ;
#31479=CARTESIAN_POINT ( 'NONE',  ( 1.339745962155608039, 22.29465819873851729, 5.000000000000003553 ) ) ;
#31481=CARTESIAN_POINT ( 'NONE',  ( 4.458734124999999437, -93.06249999863440792, -5.460374474430324690E-16 ) ) ;
#31482=CARTESIAN_POINT ( 'NONE',  ( 5.000000000000000888, -2.583333333333333481, 2.886751345948126879 ) ) ;
#31484=CARTESIAN_POINT ( 'NONE',  ( -6.972266317189433020E-16, -29.25000000000000000, -5.000000000000000000 ) ) ;
#31489=CARTESIAN_POINT ( 'NONE',  ( -4.458734124999999437, -0.3958333319677397322, -2.574251347313719407 ) ) ;
#31490=AXIS2_PLACEMENT_3D ( 'NONE', #35642, #21163, #59776 ) ;
#31491=CARTESIAN_POINT ( 'NONE',  ( 4.458734124999998549, -93.97916666530106511, -2.574251347313721627 ) ) ;
#31493=CARTESIAN_POINT ( 'NONE',  ( -2.229367062500000163, -24.72916666530106866, -3.861377020970580443 ) ) ;
#31498=CARTESIAN_POINT ( 'NONE',  ( -6.972266317189433020E-16, -98.24999999999998579, -5.000000000000000000 ) ) ;
#31500=CARTESIAN_POINT ( 'NONE',  ( 4.458734124999999437, 13.93750000136559386, -5.460374474430324690E-16 ) ) ;
#31501=EDGE_LOOP ( 'NONE', ( #59101, #47390, #25884, #12353, #11253, #52513 ) ) ;
#31504=CARTESIAN_POINT ( 'NONE',  ( -5.000000000000000000, -83.99999999999998579, 0.000000000000000000 ) ) ;
#31505=CARTESIAN_POINT ( 'NONE',  ( -3.152548672688508926E-16, -18.56249999863440792, -5.148502694627439702 ) ) ;
#31508=( BOUNDED_CURVE ( )  B_SPLINE_CURVE ( 2, ( #31654, #50638, #45810, #1771, #1452, #15906, #21053, #40660, #21372 ),
 .UNSPECIFIED., .F., .F. ) 
 B_SPLINE_CURVE_WITH_KNOTS ( ( 3, 2, 2, 2, 3 ),
 ( 0.2839285714285714191, 0.2845238095238095122, 0.2857142857142856984, 0.2869047619047618847, 0.2874999999999999778 ),
 .UNSPECIFIED. ) 
 CURVE ( )  GEOMETRIC_REPRESENTATION_ITEM ( )  RATIONAL_B_SPLINE_CURVE ( ( 0.9330127018922194093, 0.9330127018922194093, 1.000000000000000000, 0.8660254037844387076, 1.000000000000000000, 0.8660254037844387076, 1.000000000000000000, 0.9330127018922194093, 0.9330127018922194093 ) ) 
 REPRESENTATION_ITEM ( '' )  );
#31510=EDGE_CURVE ( 'NONE', #12052, #34023, #37144, .T. ) ;
#31512=CARTESIAN_POINT ( 'NONE',  ( 5.000000000000000000, -47.29166666393547303, -2.886751345948129988 ) ) ;
#31513=CARTESIAN_POINT ( 'NONE',  ( 5.000000000000000000, -41.29166666393548013, -2.886751345948130876 ) ) ;
#31514=CARTESIAN_POINT ( 'NONE',  ( 4.458734124999998549, 7.270833334698930450, -2.574251347313721627 ) ) ;
#31517=EDGE_CURVE ( 'NONE', #4102, #14760, #59141, .T. ) ;
#31519=CARTESIAN_POINT ( 'NONE',  ( -3.152548672688508926E-16, -65.56249999863440792, -5.148502694627439702 ) ) ;
#31521=EDGE_CURVE ( 'NONE', #37461, #42937, #12740, .T. ) ;
#31522=CARTESIAN_POINT ( 'NONE',  ( 2.499999999999998668, -0.3333333333333348136, -4.330127018922193649 ) ) ;
#31525=CARTESIAN_POINT ( 'NONE',  ( -4.458734124999999437, -56.31249999863440081, 0.000000000000000000 ) ) ;
#31526=CARTESIAN_POINT ( 'NONE',  ( 2.499999999999998668, -92.20833333060214443, -4.330127018922193649 ) ) ;
#31527=EDGE_CURVE ( 'NONE', #30039, #34132, #52941, .T. ) ;
#31529=( BOUNDED_CURVE ( )  B_SPLINE_CURVE ( 2, ( #41237, #7802, #60884, #6530, #2349, #35801, #50908, #47036, #56058 ),
 .UNSPECIFIED., .F., .F. ) 
 B_SPLINE_CURVE_WITH_KNOTS ( ( 3, 2, 2, 2, 3 ),
 ( 0.3410714285714285809, 0.3416666666666666741, 0.3428571428571428603, 0.3440476190476190466, 0.3446428571428571397 ),
 .UNSPECIFIED. ) 
 CURVE ( )  GEOMETRIC_REPRESENTATION_ITEM ( )  RATIONAL_B_SPLINE_CURVE ( ( 0.9330127018922194093, 0.9330127018922194093, 1.000000000000000000, 0.8660254037844387076, 1.000000000000000000, 0.8660254037844387076, 1.000000000000000000, 0.9330127018922194093, 0.9330127018922194093 ) ) 
 REPRESENTATION_ITEM ( '' )  );
#31531=CARTESIAN_POINT ( 'NONE',  ( -6.972266317189433020E-16, 5.875000002731184168, -5.000000000000000000 ) ) ;
#31534=CARTESIAN_POINT ( 'NONE',  ( 2.500000000000002220, -50.66666666666666430, 4.330127018922192761 ) ) ;
#31536=EDGE_CURVE ( 'NONE', #51626, #14365, #17194, .T. ) ;
#31539=CARTESIAN_POINT ( 'NONE',  ( -3.152548672688508926E-16, -108.5624999986343937, -5.148502694627439702 ) ) ;
#31540=CARTESIAN_POINT ( 'NONE',  ( 2.229367062500001939, -1.229166665301071548, 3.861377020970579999 ) ) ;
#31545=ADVANCED_FACE ( 'NONE', ( #56452 ), #56125, .T. ) ;
#31561=CARTESIAN_POINT ( 'NONE',  ( -2.229367062500000163, -31.72916666530107577, -3.861377020970580443 ) ) ;
#31562=CARTESIAN_POINT ( 'NONE',  ( -6.972266317189433020E-16, -106.2500000000000000, -5.000000000000000000 ) ) ;
#31568=CARTESIAN_POINT ( 'NONE',  ( 2.499999999999998668, -83.20833333060214443, -4.330127018922193649 ) ) ;
#31570=CARTESIAN_POINT ( 'NONE',  ( 4.458734124999998549, -79.97916666530107932, -2.574251347313721627 ) ) ;
#31573=DIRECTION ( 'NONE',  ( 0.000000000000000000, 0.000000000000000000, 1.000000000000000000 ) ) ;
#31576=CARTESIAN_POINT ( 'NONE',  ( -4.458734124999998549, -7.479166665301073991, 2.574251347313722516 ) ) ;
#31579=CARTESIAN_POINT ( 'NONE',  ( -5.000000000000000000, 3.041666669397851130, -2.886751345948128211 ) ) ;
#31580=EDGE_LOOP ( 'NONE', ( #36640, #43905, #50174, #10499 ) ) ;
#31581=CARTESIAN_POINT ( 'NONE',  ( -2.229367062499996610, -7.395833331967735624, 3.861377020970582219 ) ) ;
#31582=CARTESIAN_POINT ( 'NONE',  ( 0.000000000000000000, -120.0000000000000000, 0.000000000000000000 ) ) ;
#31589=CARTESIAN_POINT ( 'NONE',  ( 4.458734124999999437, -84.81249999863439371, -5.460374474430324690E-16 ) ) ;
#31591=CARTESIAN_POINT ( 'NONE',  ( -3.152548672688508926E-16, -2.562499998634407028, -5.148502694627439702 ) ) ;
#31592=AXIS2_PLACEMENT_3D ( 'NONE', #2843, #22463, #62013 ) ;
#31594=AXIS2_PLACEMENT_3D ( 'NONE', #757, #23917, #48979 ) ;
#31595=CARTESIAN_POINT ( 'NONE',  ( -5.000000000000000000, -28.95833333060215153, -2.886751345948128211 ) ) ;
#31597=CARTESIAN_POINT ( 'NONE',  ( 2.229367062499998831, 22.35416666803225993, -3.861377020970580887 ) ) ;
#31598=DIRECTION ( 'NONE',  ( -0.000000000000000000, 1.000000000000000000, -0.000000000000000000 ) ) ;
#31600=CARTESIAN_POINT ( 'NONE',  ( 2.229367062499998831, -49.64583333196772941, -3.861377020970580887 ) ) ;
#31601=CARTESIAN_POINT ( 'NONE',  ( 9.457646018065525792E-16, -39.31249999863439371, 5.148502694627439702 ) ) ;
#31604=CARTESIAN_POINT ( 'NONE',  ( 5.000000000000000888, 16.41666666666666785, 2.886751345948126879 ) ) ;
#31607=CARTESIAN_POINT ( 'NONE',  ( -2.229367062499996610, -43.14583333196773651, 3.861377020970582219 ) ) ;
#31608=CARTESIAN_POINT ( 'NONE',  ( -2.499999999999996447, -79.70833333060213022, 4.330127018922195425 ) ) ;
#31611=CARTESIAN_POINT ( 'NONE',  ( 1.339745962155612702, -36.29465819873852439, -5.000000000000000000 ) ) ;
#31612=CARTESIAN_POINT ( 'NONE',  ( -3.152548672688508926E-16, -87.81249999863437949, -5.148502694627439702 ) ) ;
#31614=CARTESIAN_POINT ( 'NONE',  ( 1.975475456537005874E-15, 13.37500000273118417, 5.000000000000000000 ) ) ;
#31615=CARTESIAN_POINT ( 'NONE',  ( 2.500000000000002220, -31.66666666666666075, 4.330127018922192761 ) ) ;
#31617=ORIENTED_EDGE ( 'NONE', *, *, #13286, .F. ) ;
#31618=ADVANCED_FACE ( 'NONE', ( #46154 ), #31672, .T. ) ;
#31620=ORIENTED_EDGE ( 'NONE', *, *, #26473, .T. ) ;
#31621=CARTESIAN_POINT ( 'NONE',  ( -4.458734124999999437, -89.39583333196773651, -2.574251347313719407 ) ) ;
#31622=CARTESIAN_POINT ( 'NONE',  ( -2.229367062499996610, 11.60416666803225993, 3.861377020970582219 ) ) ;
#31623=CARTESIAN_POINT ( 'NONE',  ( 5.000000000000000888, 18.54166666939785202, 2.886751345948126879 ) ) ;
#31631=CARTESIAN_POINT ( 'NONE',  ( 1.339745962155612702, -33.16965819600733312, -5.000000000000000000 ) ) ;
#31632=CARTESIAN_POINT ( 'NONE',  ( -5.000000000000000000, 18.12500000273118417, 0.000000000000000000 ) ) ;
#31635=CARTESIAN_POINT ( 'NONE',  ( -4.458734124999998549, -15.47916666530107399, 2.574251347313722516 ) ) ;
#31647=CARTESIAN_POINT ( 'NONE',  ( 1.975475456537005874E-15, -68.74999999999998579, 5.000000000000000000 ) ) ;
#31648=EDGE_LOOP ( 'NONE', ( #14066, #49111, #51716, #49551 ) ) ;
#31649=CARTESIAN_POINT ( 'NONE',  ( -4.458734124999999437, -61.56249999863440081, 0.000000000000000000 ) ) ;
#31651=CARTESIAN_POINT ( 'NONE',  ( 5.000000000000000000, -8.500000000000000000, -6.123233995736766282E-16 ) ) ;
#31653=EDGE_LOOP ( 'NONE', ( #39351, #47150, #4790, #6945 ) ) ;
#31654=CARTESIAN_POINT ( 'NONE',  ( 1.975475456537005874E-15, -9.750000000000000000, 5.000000000000000000 ) ) ;
#31659=CARTESIAN_POINT ( 'NONE',  ( -4.458734124999999437, 7.604166668032259935, -2.574251347313719407 ) ) ;
#31662=CARTESIAN_POINT ( 'NONE',  ( -6.972266317189433020E-16, -24.12499999726881228, -5.000000000000000000 ) ) ;
#31665=CARTESIAN_POINT ( 'NONE',  ( -2.229367062500000163, -68.47916666530107932, -3.861377020970580443 ) ) ;
#31667=CARTESIAN_POINT ( 'NONE',  ( 9.457646018065525792E-16, 11.93750000136559386, 5.148502694627439702 ) ) ;
#31668=CARTESIAN_POINT ( 'NONE',  ( 0.000000000000000000, -120.0000000000000000, 0.000000000000000000 ) ) ;
#31670=CARTESIAN_POINT ( 'NONE',  ( -2.229367062499996610, -53.39583333196773651, 3.861377020970582219 ) ) ;
#31671=CARTESIAN_POINT ( 'NONE',  ( -3.535250795749689387E-16, -15.12499999726881406, -5.773502691896257311 ) ) ;
#31672=CYLINDRICAL_SURFACE ( 'NONE', #23486, 5.000000000000000000 ) ;
#31673=LINE ( 'NONE', #27169, #29540 ) ;
#31675=CARTESIAN_POINT ( 'NONE',  ( -4.458734124999997661, -23.47916666530107221, 2.574251347313722516 ) ) ;
#31677=VECTOR ( 'NONE', #30172, 1000.000000000000000 ) ;
#31678=CARTESIAN_POINT ( 'NONE',  ( -3.152548672688508926E-16, -107.5624999986343795, -5.148502694627439702 ) ) ;
#31681=CARTESIAN_POINT ( 'NONE',  ( 2.229367062500001939, -105.2291666653010651, 3.861377020970579999 ) ) ;
#31683=CARTESIAN_POINT ( 'NONE',  ( -4.458734124999999437, -27.39583333196773651, -2.574251347313719407 ) ) ;
#31684=CARTESIAN_POINT ( 'NONE',  ( -2.500000000000000444, -65.04166666393547303, -4.330127018922193649 ) ) ;
#31687=CARTESIAN_POINT ( 'NONE',  ( -2.229367062500000163, -21.47916666530107221, -3.861377020970580443 ) ) ;
#31688=CARTESIAN_POINT ( 'NONE',  ( 4.458734124999999437, -71.06249999863439371, -5.460374474430324690E-16 ) ) ;
#31693=CARTESIAN_POINT ( 'NONE',  ( 2.500000000000002220, -17.66666666666666430, 4.330127018922192761 ) ) ;
#31695=VERTEX_POINT ( 'NONE', #43514 ) ;
#31696=DIRECTION ( 'NONE',  ( -0.000000000000000000, 1.000000000000000000, -0.000000000000000000 ) ) ;
#31698=CARTESIAN_POINT ( 'NONE',  ( 5.000000000000000000, -84.37499999726880162, -6.123233995736766282E-16 ) ) ;
#31699=CARTESIAN_POINT ( 'NONE',  ( -6.972266317189433020E-16, -14.24999999999999822, -5.000000000000000000 ) ) ;
#31705=CARTESIAN_POINT ( 'NONE',  ( 2.499999999999998668, -95.20833333060213022, -4.330127018922193649 ) ) ;
#31706=DIRECTION ( 'NONE',  ( 0.000000000000000000, 0.000000000000000000, 1.000000000000000000 ) ) ;
#31712=FACE_OUTER_BOUND ( 'NONE', #1524, .T. ) ;
#31715=( BOUNDED_CURVE ( )  B_SPLINE_CURVE ( 2, ( #48953, #34812, #44450, #19694, #38671, #4903, #59257, #38988, #15519 ),
 .UNSPECIFIED., .F., .F. ) 
 B_SPLINE_CURVE_WITH_KNOTS ( ( 3, 2, 2, 2, 3 ),
 ( 0.1232142857142857206, 0.1238095238095238138, 0.1250000000000000000, 0.1261904761904761862, 0.1267857142857142794 ),
 .UNSPECIFIED. ) 
 CURVE ( )  GEOMETRIC_REPRESENTATION_ITEM ( )  RATIONAL_B_SPLINE_CURVE ( ( 0.9330127018922192983, 0.9330127018922200755, 1.000000000000000000, 0.8660254037844387076, 1.000000000000000000, 0.8660254037844387076, 1.000000000000000000, 0.9330127018922194093, 0.9330127018922194093 ) ) 
 REPRESENTATION_ITEM ( '' )  );
#31717=ORIENTED_EDGE ( 'NONE', *, *, #27621, .T. ) ;
#31719=VERTEX_POINT ( 'NONE', #14562 ) ;
#31727=VECTOR ( 'NONE', #1613, 1000.000000000000000 ) ;
#31729=LINE ( 'NONE', #57140, #5284 ) ;
#31731=CARTESIAN_POINT ( 'NONE',  ( 4.458734125000001214, -76.89583333196775072, 2.574251347313718519 ) ) ;
#31732=CARTESIAN_POINT ( 'NONE',  ( 4.458734125000001214, 27.10416666803225993, 2.574251347313718519 ) ) ;
#31735=CYLINDRICAL_SURFACE ( 'NONE', #6899, 5.000000000000000000 ) ;
#31741=CARTESIAN_POINT ( 'NONE',  ( -3.152548672688508926E-16, -56.56249999863439371, -5.148502694627439702 ) ) ;
#31743=CARTESIAN_POINT ( 'NONE',  ( 2.229367062499998831, 29.35416666803225993, -3.861377020970580887 ) ) ;
#31744=VECTOR ( 'NONE', #22047, 1000.000000000000000 ) ;
#31745=CARTESIAN_POINT ( 'NONE',  ( 2.500000000000002220, -104.6666666666666572, 4.330127018922192761 ) ) ;
#31747=CARTESIAN_POINT ( 'NONE',  ( 4.458734125000001214, -39.14583333196773651, 2.574251347313718519 ) ) ;
#31748=CARTESIAN_POINT ( 'NONE',  ( 2.500000000000002220, 1.458333336064519203, 4.330127018922192761 ) ) ;
#31751=CARTESIAN_POINT ( 'NONE',  ( -2.229367062499996610, -102.1458333319677365, 3.861377020970582219 ) ) ;
#31752=CARTESIAN_POINT ( 'NONE',  ( 2.229367062499998831, -4.895833331967740065, -3.861377020970580887 ) ) ;
#31753=ORIENTED_EDGE ( 'NONE', *, *, #49918, .T. ) ;
#31754=CYLINDRICAL_SURFACE ( 'NONE', #51120, 5.000000000000000000 ) ;
#31756=CARTESIAN_POINT ( 'NONE',  ( 4.458734124999999437, -91.81249999863440792, -5.460374474430324690E-16 ) ) ;
#31758=CARTESIAN_POINT ( 'NONE',  ( -2.229367062500000163, -88.72916666530106511, -3.861377020970580443 ) ) ;
#31760=CARTESIAN_POINT ( 'NONE',  ( 5.000000000000000000, -2.291666663935477466, -2.886751345948130876 ) ) ;
#31762=CARTESIAN_POINT ( 'NONE',  ( -4.458734124999999437, -8.395833331967736513, -2.574251347313719407 ) ) ;
#31763=CARTESIAN_POINT ( 'NONE',  ( 2.229367062500001939, 16.77083333469892779, 3.861377020970579999 ) ) ;
#31764=CARTESIAN_POINT ( 'NONE',  ( 4.458734124999998549, -53.97916666530107221, -2.574251347313721627 ) ) ;
#31765=( BOUNDED_CURVE ( )  B_SPLINE_CURVE ( 2, ( #2522, #55916, #11830, #31449, #7028, #26961, #46258, #61068, #16989 ),
 .UNSPECIFIED., .F., .F. ) 
 B_SPLINE_CURVE_WITH_KNOTS ( ( 3, 2, 2, 2, 3 ),
 ( 0.8839285714285713969, 0.8845238095238094900, 0.8857142857142856762, 0.8869047619047618625, 0.8874999999999999556 ),
 .UNSPECIFIED. ) 
 CURVE ( )  GEOMETRIC_REPRESENTATION_ITEM ( )  RATIONAL_B_SPLINE_CURVE ( ( 0.9330127018922194093, 0.9330127018922194093, 1.000000000000000000, 0.8660254037844387076, 1.000000000000000000, 0.8660254037844387076, 1.000000000000000000, 0.9330127018922194093, 0.9330127018922194093 ) ) 
 REPRESENTATION_ITEM ( '' )  );
#31766=CARTESIAN_POINT ( 'NONE',  ( 2.500000000000002220, -11.66666666666666607, 4.330127018922192761 ) ) ;
#31769=ORIENTED_EDGE ( 'NONE', *, *, #34251, .T. ) ;
#31772=CARTESIAN_POINT ( 'NONE',  ( 9.457646018065525792E-16, -82.06249999863442213, 5.148502694627439702 ) ) ;
#31773=CARTESIAN_POINT ( 'NONE',  ( -5.000000000000000000, -109.9583333306021444, -2.886751345948128211 ) ) ;
#31780=CARTESIAN_POINT ( 'NONE',  ( 2.499999999999998668, -67.33333333333332860, -4.330127018922193649 ) ) ;
#31783=VERTEX_POINT ( 'NONE', #19713 ) ;
#31784=CARTESIAN_POINT ( 'NONE',  ( -2.500000000000000444, -62.04166666393547303, -4.330127018922193649 ) ) ;
#31795=ORIENTED_EDGE ( 'NONE', *, *, #37856, .T. ) ;
#31798=CARTESIAN_POINT ( 'NONE',  ( -4.458734124999999437, -52.56249999863440792, 0.000000000000000000 ) ) ;
#31799=CARTESIAN_POINT ( 'NONE',  ( -4.999999999999998224, 0.2083333360645180099, 2.886751345948131764 ) ) ;
#31809=CARTESIAN_POINT ( 'NONE',  ( -4.458734124999999437, -101.5624999986344079, 0.000000000000000000 ) ) ;
#31811=ORIENTED_EDGE ( 'NONE', *, *, #18079, .F. ) ;
#31819=CARTESIAN_POINT ( 'NONE',  ( 2.229367062500001939, -0.9791666653010712151, 3.861377020970579999 ) ) ;
#31820=CARTESIAN_POINT ( 'NONE',  ( -2.229367062500000163, -97.72916666530105090, -3.861377020970580443 ) ) ;
#31822=CARTESIAN_POINT ( 'NONE',  ( 9.457646018065525792E-16, -25.31249999863440792, 5.148502694627439702 ) ) ;
#31823=ADVANCED_FACE ( 'NONE', ( #8496 ), #3988, .T. ) ;
#31827=CARTESIAN_POINT ( 'NONE',  ( 5.000000000000000000, -70.41666666666667140, -2.886751345948130876 ) ) ;
#31830=CARTESIAN_POINT ( 'NONE',  ( 2.229367062500001939, 8.770833334698927786, 3.861377020970579999 ) ) ;
#31832=CARTESIAN_POINT ( 'NONE',  ( -1.339745962155610925, -80.79465819873850307, 5.000000000000000000 ) ) ;
#31833=PLANE ( 'NONE',  #11321 ) ;
#31834=CARTESIAN_POINT ( 'NONE',  ( -3.535250795749689387E-16, -87.24999999999998579, -5.773502691896257311 ) ) ;
#31835=CARTESIAN_POINT ( 'NONE',  ( 9.457646018065525792E-16, -24.06249999863440436, 5.148502694627439702 ) ) ;
#31836=DIRECTION ( 'NONE',  ( -0.000000000000000000, 1.000000000000000000, -0.000000000000000000 ) ) ;
#31839=CARTESIAN_POINT ( 'NONE',  ( 5.000000000000000888, -50.45833333060213732, 2.886751345948126879 ) ) ;
#31840=CARTESIAN_POINT ( 'NONE',  ( 1.339745962155612702, -24.29465819873852084, -5.000000000000000000 ) ) ;
#31841=CARTESIAN_POINT ( 'NONE',  ( 4.458734124999999437, 10.18750000136559386, -5.460374474430324690E-16 ) ) ;
#31845=CARTESIAN_POINT ( 'NONE',  ( 9.457646018065525792E-16, -68.06249999863440792, 5.148502694627439702 ) ) ;
#31847=CARTESIAN_POINT ( 'NONE',  ( -3.535250795749689387E-16, 1.750000000000001554, -5.773502691896257311 ) ) ;
#31850=CARTESIAN_POINT ( 'NONE',  ( 2.229367062499998831, -61.64583333196774362, -3.861377020970580887 ) ) ;
#31851=CARTESIAN_POINT ( 'NONE',  ( -4.999999999999999112, -93.79166666393545881, 2.886751345948131764 ) ) ;
#31856=CARTESIAN_POINT ( 'NONE',  ( -5.000000000000000000, -48.08333333333332860, -2.886751345948128211 ) ) ;
#31857=CARTESIAN_POINT ( 'NONE',  ( -6.972266317189433020E-16, -23.24999999999999645, -5.000000000000000000 ) ) ;
#31860=CARTESIAN_POINT ( 'NONE',  ( -3.152548672688508926E-16, -106.5624999986343937, -5.148502694627439702 ) ) ;
#31861=CARTESIAN_POINT ( 'NONE',  ( -4.458734124999999437, -3.562499998634407916, 0.000000000000000000 ) ) ;
#31864=AXIS2_PLACEMENT_3D ( 'NONE', #15642, #35258, #40707 ) ;
#31866=CARTESIAN_POINT ( 'NONE',  ( -1.339745962155613812, -31.08034179853029144, -5.000000000000000000 ) ) ;
#31870=LINE ( 'NONE', #42459, #56956 ) ;
#31872=ORIENTED_EDGE ( 'NONE', *, *, #43360, .T. ) ;
#31876=CARTESIAN_POINT ( 'NONE',  ( -3.152548672688508926E-16, -34.81249999863440792, -5.148502694627439702 ) ) ;
#31877=CARTESIAN_POINT ( 'NONE',  ( 2.499999999999998668, -10.33333333333333393, -4.330127018922193649 ) ) ;
#31884=EDGE_CURVE ( 'NONE', #52286, #4881, #22151, .T. ) ;
#31887=CARTESIAN_POINT ( 'NONE',  ( 4.458734125000001214, -77.14583333196775072, 2.574251347313718519 ) ) ;
#31890=ORIENTED_EDGE ( 'NONE', *, *, #38208, .T. ) ;
#31892=CARTESIAN_POINT ( 'NONE',  ( 0.000000000000000000, -120.0000000000000000, 0.000000000000000000 ) ) ;
#31894=CARTESIAN_POINT ( 'NONE',  ( 2.229367062500001939, -11.22916666530107044, 3.861377020970579999 ) ) ;
#31895=ORIENTED_EDGE ( 'NONE', *, *, #48531, .T. ) ;
#31899=CARTESIAN_POINT ( 'NONE',  ( 9.457646018065525792E-16, -8.312499998634406140, 5.148502694627439702 ) ) ;
#31905=CARTESIAN_POINT ( 'NONE',  ( 4.458734125000000326, 26.85416666803225993, 2.574251347313718519 ) ) ;
#31907=CARTESIAN_POINT ( 'NONE',  ( -2.229367062500000163, -86.47916666530107932, -3.861377020970580443 ) ) ;
#31909=CARTESIAN_POINT ( 'NONE',  ( -5.000000000000000000, -31.00000000000000000, 0.000000000000000000 ) ) ;
#31910=CARTESIAN_POINT ( 'NONE',  ( 2.229367062499998831, -3.645833331967739177, -3.861377020970580887 ) ) ;
#31911=LINE ( 'NONE', #12916, #38555 ) ;
#31912=( BOUNDED_CURVE ( )  B_SPLINE_CURVE ( 2, ( #17606, #31426, #37222, #2197, #13085, #7955, #32388, #51064, #47189 ),
 .UNSPECIFIED., .F., .F. ) 
 B_SPLINE_CURVE_WITH_KNOTS ( ( 3, 2, 2, 2, 3 ),
 ( 0.8196428571428571175, 0.8202380952380952106, 0.8214285714285713969, 0.8226190476190475831, 0.8232142857142856762 ),
 .UNSPECIFIED. ) 
 CURVE ( )  GEOMETRIC_REPRESENTATION_ITEM ( )  RATIONAL_B_SPLINE_CURVE ( ( 0.9330127018922194093, 0.9330127018922194093, 1.000000000000000000, 0.8660254037844387076, 1.000000000000000000, 0.8660254037844387076, 1.000000000000000000, 0.9330127018922194093, 0.9330127018922194093 ) ) 
 REPRESENTATION_ITEM ( '' )  );
#31913=CARTESIAN_POINT ( 'NONE',  ( 1.060575238724906964E-15, -32.62499999726880873, 5.773502691896257311 ) ) ;
#31915=CARTESIAN_POINT ( 'NONE',  ( 2.229367062499998831, 25.35416666803225993, -3.861377020970580887 ) ) ;
#31916=CARTESIAN_POINT ( 'NONE',  ( 2.500000000000002220, -7.666666666666668739, 4.330127018922192761 ) ) ;
#31918=CARTESIAN_POINT ( 'NONE',  ( 4.458734125000001214, -50.89583333196772230, 2.574251347313718519 ) ) ;
#31919=CARTESIAN_POINT ( 'NONE',  ( 4.458734124999998549, -36.97916666530107221, -2.574251347313721627 ) ) ;
#31922=CARTESIAN_POINT ( 'NONE',  ( 5.000000000000000000, 14.49999999999999822, -6.123233995736766282E-16 ) ) ;
#31925=CARTESIAN_POINT ( 'NONE',  ( -3.152548672688508926E-16, -47.56249999863440792, -5.148502694627439702 ) ) ;
#31926=CARTESIAN_POINT ( 'NONE',  ( -2.500000000000000444, -77.04166666393547303, -4.330127018922193649 ) ) ;
#31930=CARTESIAN_POINT ( 'NONE',  ( 4.458734124999999437, -83.06249999863440792, -5.460374474430324690E-16 ) ) ;
#31932=CARTESIAN_POINT ( 'NONE',  ( -5.000000000000000000, -35.00000000000000000, 0.000000000000000000 ) ) ;
#31934=ORIENTED_EDGE ( 'NONE', *, *, #51847, .F. ) ;
#31936=ORIENTED_EDGE ( 'NONE', *, *, #8583, .F. ) ;
#31937=CARTESIAN_POINT ( 'NONE',  ( 4.458734125000001214, -92.89583333196775072, 2.574251347313718519 ) ) ;
#31938=CARTESIAN_POINT ( 'NONE',  ( -4.458734124999999437, 15.35416666803225993, -2.574251347313719407 ) ) ;
#31939=CARTESIAN_POINT ( 'NONE',  ( -5.000000000000000000, 18.12500000273118417, 0.000000000000000000 ) ) ;
#31946=CARTESIAN_POINT ( 'NONE',  ( 1.339745962155615144, -33.58034179853029144, 4.999999999999999112 ) ) ;
#31949=CARTESIAN_POINT ( 'NONE',  ( 0.000000000000000000, -120.0000000000000000, 0.000000000000000000 ) ) ;
#31950=CARTESIAN_POINT ( 'NONE',  ( 4.458734124999999437, -14.06249999863440436, -5.460374474430324690E-16 ) ) ;
#31951=CARTESIAN_POINT ( 'NONE',  ( -6.972266317189433020E-16, -107.1249999972687874, -5.000000000000000000 ) ) ;
#31958=EDGE_CURVE ( 'NONE', #60996, #37188, #43896, .T. ) ;
#31961=ORIENTED_EDGE ( 'NONE', *, *, #5968, .F. ) ;
#31962=CARTESIAN_POINT ( 'NONE',  ( -4.458734124999999437, -64.56249999863440792, 0.000000000000000000 ) ) ;
#31971=ORIENTED_EDGE ( 'NONE', *, *, #3527, .T. ) ;
#31972=CARTESIAN_POINT ( 'NONE',  ( -6.031010364368858512E-14, 2.375000002731183280, 5.000000000000000000 ) ) ;
#31973=CARTESIAN_POINT ( 'NONE',  ( 9.457646018065525792E-16, 8.937500001365597413, 5.148502694627439702 ) ) ;
#31977=CARTESIAN_POINT ( 'NONE',  ( 1.339745962155729053, -77.29465819873853150, -4.999999999999933387 ) ) ;
#31979=ORIENTED_EDGE ( 'NONE', *, *, #16484, .T. ) ;
#31980=ADVANCED_FACE ( 'NONE', ( #29673 ), #40919, .T. ) ;
#31981=CARTESIAN_POINT ( 'NONE',  ( -4.458734124999999437, -73.31249999863439371, 0.000000000000000000 ) ) ;
#31982=CARTESIAN_POINT ( 'NONE',  ( 5.000000000000000888, 14.54166666939785202, 2.886751345948126879 ) ) ;
#31983=CARTESIAN_POINT ( 'NONE',  ( -2.229367062500000163, 11.52083333469892601, -3.861377020970580443 ) ) ;
#31986=CARTESIAN_POINT ( 'NONE',  ( -4.458734124999998549, -55.47916666530107221, 2.574251347313722516 ) ) ;
#31987=CARTESIAN_POINT ( 'NONE',  ( -2.500000000000000444, -16.04166666393548368, -4.330127018922193649 ) ) ;
#31988=CARTESIAN_POINT ( 'NONE',  ( -5.000000000000000000, -19.08333333333333570, -2.886751345948128211 ) ) ;
#31989=CARTESIAN_POINT ( 'NONE',  ( -2.480964764533239819E-13, -60.62499999726880873, 5.000000000000000000 ) ) ;
#31990=CARTESIAN_POINT ( 'NONE',  ( 2.229367062500001939, -32.97916666530106511, 3.861377020970579999 ) ) ;
#31991=CARTESIAN_POINT ( 'NONE',  ( 4.458734124999999437, -22.06249999863440436, -5.460374474430324690E-16 ) ) ;
#31992=VERTEX_POINT ( 'NONE', #2652 ) ;
#31993=CARTESIAN_POINT ( 'NONE',  ( -5.000000000000000000, -61.08333333333333570, -2.886751345948128211 ) ) ;
#31994=CARTESIAN_POINT ( 'NONE',  ( 4.458734124999998549, -107.7291666653010509, -2.574251347313721627 ) ) ;
#31997=CARTESIAN_POINT ( 'NONE',  ( 4.458734125000001214, -103.1458333319677365, 2.574251347313718519 ) ) ;
#31998=VECTOR ( 'NONE', #44827, 1000.000000000000000 ) ;
#31999=CARTESIAN_POINT ( 'NONE',  ( 9.457646018065525792E-16, -25.06249999863440792, 5.148502694627439702 ) ) ;
#32000=CARTESIAN_POINT ( 'NONE',  ( 5.000000000000000000, -63.29166666393547303, -2.886751345948129988 ) ) ;
#32003=CARTESIAN_POINT ( 'NONE',  ( -3.152548672688508926E-16, -28.56249999863440081, -5.148502694627439702 ) ) ;
#32004=CARTESIAN_POINT ( 'NONE',  ( -4.458734124999999437, -69.56249999863439371, 0.000000000000000000 ) ) ;
#32007=CARTESIAN_POINT ( 'NONE',  ( 5.000000000000000000, -32.50000000000000000, -6.123233995736766282E-16 ) ) ;
#32008=CARTESIAN_POINT ( 'NONE',  ( 2.499999999999998668, -5.208333330602148870, -4.330127018922193649 ) ) ;
#32009=CARTESIAN_POINT ( 'NONE',  ( -5.000000000000000000, -15.00000000000000000, 0.000000000000000000 ) ) ;
#32015=DIRECTION ( 'NONE',  ( -0.000000000000000000, 1.000000000000000000, -0.000000000000000000 ) ) ;
#32019=CARTESIAN_POINT ( 'NONE',  ( 2.500000000000002220, 1.458333336064519203, 4.330127018922192761 ) ) ;
#32038=CARTESIAN_POINT ( 'NONE',  ( -2.499999999999996447, 21.16666666666666785, 4.330127018922195425 ) ) ;
#32040=CARTESIAN_POINT ( 'NONE',  ( -4.458734124999998549, -75.22916666530106511, 2.574251347313722516 ) ) ;
#32041=CARTESIAN_POINT ( 'NONE',  ( 4.458734124999998549, 22.27083333469893134, -2.574251347313721627 ) ) ;
#32042=CARTESIAN_POINT ( 'NONE',  ( 1.975475456537005874E-15, -87.62499999726880162, 5.000000000000000000 ) ) ;
#32043=VERTEX_POINT ( 'NONE', #26456 ) ;
#32048=CARTESIAN_POINT ( 'NONE',  ( 1.339745962155615144, -27.70534180126147561, 4.999999999999999112 ) ) ;
#32051=CARTESIAN_POINT ( 'NONE',  ( 4.458734124999998549, -54.72916666530107221, -2.574251347313721627 ) ) ;
#32053=CARTESIAN_POINT ( 'NONE',  ( 4.458734124999999437, 29.18750000136559208, -5.460374474430324690E-16 ) ) ;
#32054=CARTESIAN_POINT ( 'NONE',  ( -2.499999999999996447, -105.8333333333333286, 4.330127018922195425 ) ) ;
#32056=CARTESIAN_POINT ( 'NONE',  ( 4.458734125000001214, -40.14583333196772941, 2.574251347313718519 ) ) ;
#32057=CARTESIAN_POINT ( 'NONE',  ( 5.000000000000000000, 2.708333336064520314, -2.886751345948129988 ) ) ;
#32061=CARTESIAN_POINT ( 'NONE',  ( -4.999999999999998224, 6.083333333333333037, 2.886751345948131764 ) ) ;
#32062=CARTESIAN_POINT ( 'NONE',  ( 2.229367062499998831, -100.6458333319677365, -3.861377020970580887 ) ) ;
#32063=CARTESIAN_POINT ( 'NONE',  ( -3.152548672688508926E-16, -3.812499998634408360, -5.148502694627439702 ) ) ;
#32066=CARTESIAN_POINT ( 'NONE',  ( 9.457646018065525792E-16, -95.06249999863440792, 5.148502694627439702 ) ) ;
#32068=CARTESIAN_POINT ( 'NONE',  ( -2.229367062499996610, -88.39583333196773651, 3.861377020970582219 ) ) ;
#32070=DIRECTION ( 'NONE',  ( 0.000000000000000000, 0.000000000000000000, 1.000000000000000000 ) ) ;
#32072=CARTESIAN_POINT ( 'NONE',  ( 4.458734124999999437, -9.812499998634406140, -5.460374474430324690E-16 ) ) ;
#32073=CARTESIAN_POINT ( 'NONE',  ( 9.457646018065525792E-16, 18.68750000136559208, 5.148502694627439702 ) ) ;
#32074=CARTESIAN_POINT ( 'NONE',  ( 4.458734124999999437, -54.06249999863440081, -5.460374474430324690E-16 ) ) ;
#32076=CARTESIAN_POINT ( 'NONE',  ( -1.339745962155613812, -37.20534180126147561, -5.000000000000000000 ) ) ;
#32078=CARTESIAN_POINT ( 'NONE',  ( 1.339745962155615144, -109.5803417985302843, 4.999999999999999112 ) ) ;
#32082=CARTESIAN_POINT ( 'NONE',  ( -6.972266317189433020E-16, -68.24999999999998579, -5.000000000000000000 ) ) ;
#32083=CARTESIAN_POINT ( 'NONE',  ( 2.229367062499998831, -81.64583333196773651, -3.861377020970580887 ) ) ;
#32084=CARTESIAN_POINT ( 'NONE',  ( 9.457646018065525792E-16, 22.68750000136559564, 5.148502694627439702 ) ) ;
#32086=( BOUNDED_CURVE ( )  B_SPLINE_CURVE ( 2, ( #11778, #36550, #32038, #46837, #22081, #51359, #56505, #61329, #31396 ),
 .UNSPECIFIED., .F., .F. ) 
 B_SPLINE_CURVE_WITH_KNOTS ( ( 3, 2, 2, 2, 3 ),
 ( 0.06250000000000000000, 0.06309523809523809312, 0.06428571428571427937, 0.06547619047619047949, 0.06607142857142857262 ),
 .UNSPECIFIED. ) 
 CURVE ( )  GEOMETRIC_REPRESENTATION_ITEM ( )  RATIONAL_B_SPLINE_CURVE ( ( 0.9330127018922194093, 0.9330127018922194093, 1.000000000000000000, 0.8660254037844387076, 1.000000000000000000, 0.8660254037844387076, 1.000000000000000000, 0.9330127018922194093, 0.9330127018922194093 ) ) 
 REPRESENTATION_ITEM ( '' )  );
#32089=DIRECTION ( 'NONE',  ( -0.000000000000000000, 1.000000000000000000, -0.000000000000000000 ) ) ;
#32090=FACE_OUTER_BOUND ( 'NONE', #40562, .T. ) ;
#32092=CARTESIAN_POINT ( 'NONE',  ( 2.499999999999998668, -64.33333333333332860, -4.330127018922193649 ) ) ;
#32093=CARTESIAN_POINT ( 'NONE',  ( 0.000000000000000000, -120.0000000000000000, 0.000000000000000000 ) ) ;
#32096=CARTESIAN_POINT ( 'NONE',  ( 1.339745962155615144, -18.58034179853029499, 4.999999999999999112 ) ) ;
#32098=CARTESIAN_POINT ( 'NONE',  ( -1.339745962155613812, -72.20534180126148271, -5.000000000000000000 ) ) ;
#32105=CARTESIAN_POINT ( 'NONE',  ( 2.499999999999998668, -28.33333333333333570, -4.330127018922193649 ) ) ;
#32110=CARTESIAN_POINT ( 'NONE',  ( 4.458734125000001214, -52.14583333196772941, 2.574251347313718519 ) ) ;
#32113=ORIENTED_EDGE ( 'NONE', *, *, #22458, .F. ) ;
#32120=CARTESIAN_POINT ( 'NONE',  ( -2.229367062500000163, -99.72916666530106511, -3.861377020970580443 ) ) ;
#32122=VERTEX_POINT ( 'NONE', #55731 ) ;
#32126=CARTESIAN_POINT ( 'NONE',  ( 4.458734124999998549, -8.729166665301073991, -2.574251347313721627 ) ) ;
#32127=CARTESIAN_POINT ( 'NONE',  ( -4.458734124999997661, -93.47916666530106511, 2.574251347313722516 ) ) ;
#32129=CARTESIAN_POINT ( 'NONE',  ( 2.229367062499998831, -20.89583333196774007, -3.861377020970580887 ) ) ;
#32134=CARTESIAN_POINT ( 'NONE',  ( 5.000000000000000888, -70.58333333333332860, 2.886751345948126879 ) ) ;
#32135=CARTESIAN_POINT ( 'NONE',  ( -6.972266317189433020E-16, 16.74999999999999645, -5.000000000000000000 ) ) ;
#32137=CARTESIAN_POINT ( 'NONE',  ( 9.457646018065525792E-16, 12.68750000136559208, 5.148502694627439702 ) ) ;
#32139=CARTESIAN_POINT ( 'NONE',  ( 1.975475456537005874E-15, -18.62499999726881228, 5.000000000000000000 ) ) ;
#32141=CARTESIAN_POINT ( 'NONE',  ( -2.500000000000000444, -90.16666666666665719, -4.330127018922193649 ) ) ;
#32142=CARTESIAN_POINT ( 'NONE',  ( -4.458734124999999437, -22.39583333196773651, -2.574251347313719407 ) ) ;
#32144=CARTESIAN_POINT ( 'NONE',  ( -4.458734124999999437, -69.56249999863439371, 0.000000000000000000 ) ) ;
#32148=CARTESIAN_POINT ( 'NONE',  ( 4.458734124999999437, 8.187500001365595637, -5.460374474430324690E-16 ) ) ;
#32149=CARTESIAN_POINT ( 'NONE',  ( -1.339745962155613812, -63.08034179853028434, -5.000000000000000000 ) ) ;
#32152=CARTESIAN_POINT ( 'NONE',  ( -2.229367062500000163, -72.47916666530107932, -3.861377020970580443 ) ) ;
#32154=CARTESIAN_POINT ( 'NONE',  ( 1.060575238724906964E-15, -1.750000000000001554, 5.773502691896257311 ) ) ;
#32157=CARTESIAN_POINT ( 'NONE',  ( -4.458734124999999437, -66.31249999863440792, 0.000000000000000000 ) ) ;
#32158=CARTESIAN_POINT ( 'NONE',  ( 5.000000000000000000, -100.2916666639354730, -2.886751345948129988 ) ) ;
#32165=CARTESIAN_POINT ( 'NONE',  ( -2.499999999999996447, -50.83333333333332860, 4.330127018922195425 ) ) ;
#32169=CARTESIAN_POINT ( 'NONE',  ( 2.229367062499998831, -109.6458333319677365, -3.861377020970580887 ) ) ;
#32170=CARTESIAN_POINT ( 'NONE',  ( 5.000000000000000888, -73.45833333060214443, 2.886751345948126879 ) ) ;
#32173=DIRECTION ( 'NONE',  ( -0.000000000000000000, 1.000000000000000000, -0.000000000000000000 ) ) ;
#32178=DIRECTION ( 'NONE',  ( -0.000000000000000000, 1.000000000000000000, -0.000000000000000000 ) ) ;
#32179=ADVANCED_FACE ( 'NONE', ( #32222 ), #41546, .F. ) ;
#32181=VERTEX_POINT ( 'NONE', #12298 ) ;
#32185=CARTESIAN_POINT ( 'NONE',  ( -2.229367062500000163, -36.72916666530107221, -3.861377020970580443 ) ) ;
#32186=CARTESIAN_POINT ( 'NONE',  ( -6.972266317189433020E-16, -87.25000000000001421, -5.000000000000000000 ) ) ;
#32188=( BOUNDED_CURVE ( )  B_SPLINE_CURVE ( 2, ( #40617, #16179, #35804, #11345, #50593, #26147, #1722, #41240, #11657 ),
 .UNSPECIFIED., .F., .F. ) 
 B_SPLINE_CURVE_WITH_KNOTS ( ( 3, 2, 2, 2, 3 ),
 ( 0.3946428571428571286, 0.3952380952380952217, 0.3964285714285714080, 0.3976190476190475942, 0.3982142857142857428 ),
 .UNSPECIFIED. ) 
 CURVE ( )  GEOMETRIC_REPRESENTATION_ITEM ( )  RATIONAL_B_SPLINE_CURVE ( ( 0.9330127018922194093, 0.9330127018922194093, 1.000000000000000000, 0.8660254037844387076, 1.000000000000000000, 0.8660254037844387076, 1.000000000000000000, 0.9330127018922163007, 0.9330127018922194093 ) ) 
 REPRESENTATION_ITEM ( '' )  );
#32196=CYLINDRICAL_SURFACE ( 'NONE', #16369, 5.000000000000000000 ) ;
#32197=CARTESIAN_POINT ( 'NONE',  ( -4.458734124999998549, -84.47916666530107932, 2.574251347313722516 ) ) ;
#32203=CARTESIAN_POINT ( 'NONE',  ( -4.458734124999999437, -41.31249999863440081, 0.000000000000000000 ) ) ;
#32204=CARTESIAN_POINT ( 'NONE',  ( 2.229367062500001939, -10.22916666530106866, 3.861377020970579999 ) ) ;
#32205=EDGE_LOOP ( 'NONE', ( #63203, #53208, #39087, #12096 ) ) ;
#32206=CARTESIAN_POINT ( 'NONE',  ( 0.000000000000000000, -120.0000000000000000, 5.000000000000000000 ) ) ;
#32208=EDGE_CURVE ( 'NONE', #24763, #12275, #41230, .T. ) ;
#32209=CARTESIAN_POINT ( 'NONE',  ( -4.458734124999999437, -4.645833331967739177, -2.574251347313719407 ) ) ;
#32213=CARTESIAN_POINT ( 'NONE',  ( -2.229367062499996610, 28.60416666803226349, 3.861377020970582219 ) ) ;
#32214=VERTEX_POINT ( 'NONE', #7796 ) ;
#32215=CARTESIAN_POINT ( 'NONE',  ( 2.229367062499998831, -86.64583333196773651, -3.861377020970580887 ) ) ;
#32217=CARTESIAN_POINT ( 'NONE',  ( -3.152548672688508926E-16, -10.56249999863440792, -5.148502694627439702 ) ) ;
#32221=CARTESIAN_POINT ( 'NONE',  ( -4.999999999999999112, -33.79166666393547303, 2.886751345948131764 ) ) ;
#32222=FACE_OUTER_BOUND ( 'NONE', #10822, .T. ) ;
#32223=CARTESIAN_POINT ( 'NONE',  ( 4.458734124999999437, 26.18750000136559564, -5.460374474430324690E-16 ) ) ;
#32224=CARTESIAN_POINT ( 'NONE',  ( -4.999999999999998224, -3.916666666666665630, 2.886751345948131764 ) ) ;
#32226=CARTESIAN_POINT ( 'NONE',  ( 4.458734124999999437, -57.81249999863440081, -5.460374474430324690E-16 ) ) ;
#32228=CARTESIAN_POINT ( 'NONE',  ( 1.975475456537005874E-15, 9.375000002731185944, 5.000000000000000000 ) ) ;
#32229=CARTESIAN_POINT ( 'NONE',  ( -3.535250795749689387E-16, 15.75000000000000178, -5.773502691896257311 ) ) ;
#32232=CARTESIAN_POINT ( 'NONE',  ( -4.458734124999998549, -47.22916666530106511, 2.574251347313722516 ) ) ;
#32233=CARTESIAN_POINT ( 'NONE',  ( 5.000000000000000000, -79.29166666393548724, -2.886751345948129988 ) ) ;
#32236=VECTOR ( 'NONE', #54610, 1000.000000000000000 ) ;
#32237=CARTESIAN_POINT ( 'NONE',  ( 1.339745962155612702, -37.16965819600733312, -5.000000000000000000 ) ) ;
#32238=EDGE_CURVE ( 'NONE', #4573, #31397, #56693, .T. ) ;
#32239=CARTESIAN_POINT ( 'NONE',  ( 5.000000000000000000, -36.50000000000000711, -6.123233995736766282E-16 ) ) ;
#32240=ADVANCED_FACE ( 'NONE', ( #52169 ), #16802, .T. ) ;
#32241=CARTESIAN_POINT ( 'NONE',  ( -2.229367062500000163, -83.72916666530106511, -3.861377020970580443 ) ) ;
#32243=CARTESIAN_POINT ( 'NONE',  ( -5.000000000000000000, -31.00000000000000000, 0.000000000000000000 ) ) ;
#32244=CARTESIAN_POINT ( 'NONE',  ( -5.000000000000000000, 23.91666666666666785, -2.886751345948128211 ) ) ;
#32248=CARTESIAN_POINT ( 'NONE',  ( 4.458734125000001214, -93.89583333196772230, 2.574251347313718519 ) ) ;
#32249=CARTESIAN_POINT ( 'NONE',  ( 4.458734124999999437, 13.93750000136559386, -5.460374474430324690E-16 ) ) ;
#32250=CARTESIAN_POINT ( 'NONE',  ( 2.500000000000002220, 16.45833333606451987, 4.330127018922192761 ) ) ;
#32251=CARTESIAN_POINT ( 'NONE',  ( -4.999999999999998224, -28.79166666393548013, 2.886751345948131764 ) ) ;
#32255=CARTESIAN_POINT ( 'NONE',  ( 2.500000000000002220, -79.66666666666665719, 4.330127018922192761 ) ) ;
#32257=CARTESIAN_POINT ( 'NONE',  ( 2.500000000000002220, -40.54166666393548013, 4.330127018922192761 ) ) ;
#32262=CARTESIAN_POINT ( 'NONE',  ( 1.339745962155615144, -96.70534180126146850, 4.999999999999999112 ) ) ;
#32263=CARTESIAN_POINT ( 'NONE',  ( -4.999999999999998224, 14.08333333333333393, 2.886751345948131764 ) ) ;
#32264=CARTESIAN_POINT ( 'NONE',  ( -2.229367062500000163, -18.72916666530106866, -3.861377020970580443 ) ) ;
#32275=CARTESIAN_POINT ( 'NONE',  ( 5.000000000000000888, -85.45833333060213022, 2.886751345948126879 ) ) ;
#32276=EDGE_LOOP ( 'NONE', ( #11040, #17806, #37456, #10203 ) ) ;
#32277=CARTESIAN_POINT ( 'NONE',  ( 4.458734124999999437, -69.06249999863439371, -5.460374474430324690E-16 ) ) ;
#32285=ORIENTED_EDGE ( 'NONE', *, *, #5248, .F. ) ;
#32289=CARTESIAN_POINT ( 'NONE',  ( -2.229367062499996610, 5.854166668032262599, 3.861377020970582219 ) ) ;
#32292=CARTESIAN_POINT ( 'NONE',  ( 5.000000000000000888, -77.58333333333334281, 2.886751345948126879 ) ) ;
#32295=CARTESIAN_POINT ( 'NONE',  ( -2.229367062499996610, -69.14583333196773651, 3.861377020970582219 ) ) ;
#32297=CARTESIAN_POINT ( 'NONE',  ( 9.457646018065525792E-16, 6.937500001365594748, 5.148502694627439702 ) ) ;
#32298=CARTESIAN_POINT ( 'NONE',  ( 2.229367062500001939, -61.22916666530106511, 3.861377020970579999 ) ) ;
#32299=CARTESIAN_POINT ( 'NONE',  ( 5.000000000000000888, -17.45833333060214443, 2.886751345948126879 ) ) ;
#32300=CARTESIAN_POINT ( 'NONE',  ( -1.339745962155613812, -33.08034179853029144, -5.000000000000000000 ) ) ;
#32304=CARTESIAN_POINT ( 'NONE',  ( -2.229367062499996610, -34.14583333196772941, 3.861377020970582219 ) ) ;
#32305=CARTESIAN_POINT ( 'NONE',  ( 9.457646018065525792E-16, -23.31249999863440436, 5.148502694627439702 ) ) ;
#32306=ORIENTED_EDGE ( 'NONE', *, *, #55869, .F. ) ;
#32307=CARTESIAN_POINT ( 'NONE',  ( -5.000000000000000000, -102.0000000000000142, 0.000000000000000000 ) ) ;
#32308=CARTESIAN_POINT ( 'NONE',  ( 2.229367062499998831, -109.6458333319677365, -3.861377020970580887 ) ) ;
#32311=CARTESIAN_POINT ( 'NONE',  ( -4.458734124999998549, -108.4791666653010793, 2.574251347313722516 ) ) ;
#32312=CARTESIAN_POINT ( 'NONE',  ( 2.229367062500001939, -31.97916666530106866, 3.861377020970579999 ) ) ;
#32313=CARTESIAN_POINT ( 'NONE',  ( 2.499999999999998668, -63.20833333060215153, -4.330127018922193649 ) ) ;
#32316=EDGE_CURVE ( 'NONE', #43365, #22249, #61229, .T. ) ;
#32317=CARTESIAN_POINT ( 'NONE',  ( 9.457646018065525792E-16, -30.06249999863440436, 5.148502694627439702 ) ) ;
#32318=CARTESIAN_POINT ( 'NONE',  ( -4.458734124999997661, -71.47916666530107932, 2.574251347313722516 ) ) ;
#32323=FACE_OUTER_BOUND ( 'NONE', #60027, .T. ) ;
#32324=CARTESIAN_POINT ( 'NONE',  ( 5.000000000000000888, -16.58333333333333215, 2.886751345948126879 ) ) ;
#32326=ORIENTED_EDGE ( 'NONE', *, *, #21676, .F. ) ;
#32331=CARTESIAN_POINT ( 'NONE',  ( -1.339745962155585168, -1.205341801261480716, -5.000000000000015987 ) ) ;
#32333=ADVANCED_FACE ( 'NONE', ( #18062 ), #53732, .T. ) ;
#32334=ADVANCED_FACE ( 'NONE', ( #48272 ), #28656, .T. ) ;
#32339=CARTESIAN_POINT ( 'NONE',  ( -2.499999999999996447, -80.70833333060213022, 4.330127018922195425 ) ) ;
#32342=EDGE_CURVE ( 'NONE', #29555, #57839, #45233, .T. ) ;
#32346=( BOUNDED_CURVE ( )  B_SPLINE_CURVE ( 2, ( #54007, #59160, #5441, #15093, #10268, #29872, #25059, #21195, #45317 ),
 .UNSPECIFIED., .F., .F. ) 
 B_SPLINE_CURVE_WITH_KNOTS ( ( 3, 2, 2, 2, 3 ),
 ( 0.4589285714285714080, 0.4595238095238095011, 0.4607142857142856873, 0.4619047619047619291, 0.4625000000000000222 ),
 .UNSPECIFIED. ) 
 CURVE ( )  GEOMETRIC_REPRESENTATION_ITEM ( )  RATIONAL_B_SPLINE_CURVE ( ( 0.9330127018922194093, 0.9330127018922194093, 1.000000000000000000, 0.8660254037844387076, 1.000000000000000000, 0.8660254037844387076, 1.000000000000000000, 0.9330127018922194093, 0.9330127018922194093 ) ) 
 REPRESENTATION_ITEM ( '' )  );
#32353=ORIENTED_EDGE ( 'NONE', *, *, #36239, .T. ) ;
#32356=CARTESIAN_POINT ( 'NONE',  ( -5.000000000000000000, -11.99999999999999645, 0.000000000000000000 ) ) ;
#32362=CARTESIAN_POINT ( 'NONE',  ( -2.229367062500000163, -83.47916666530106511, -3.861377020970580443 ) ) ;
#32363=CARTESIAN_POINT ( 'NONE',  ( 9.457646018065525792E-16, 24.93750000136559564, 5.148502694627439702 ) ) ;
#32365=ORIENTED_EDGE ( 'NONE', *, *, #54526, .T. ) ;
#32374=CARTESIAN_POINT ( 'NONE',  ( -2.229367062499996610, -54.14583333196773651, 3.861377020970582219 ) ) ;
#32376=CARTESIAN_POINT ( 'NONE',  ( -4.458734124999999437, 25.68750000136559208, 0.000000000000000000 ) ) ;
#32377=CARTESIAN_POINT ( 'NONE',  ( -2.500000000000000444, -104.1666666666666572, -4.330127018922193649 ) ) ;
#32378=AXIS2_PLACEMENT_3D ( 'NONE', #41543, #2649, #22268 ) ;
#32380=CARTESIAN_POINT ( 'NONE',  ( 2.229367062500001939, -42.22916666530107932, 3.861377020970579999 ) ) ;
#32381=CARTESIAN_POINT ( 'NONE',  ( -5.000000000000000000, 1.041666669397853129, -2.886751345948128211 ) ) ;
#32385=CARTESIAN_POINT ( 'NONE',  ( -4.458734124999999437, -103.3958333319677223, -2.574251347313719407 ) ) ;
#32386=CARTESIAN_POINT ( 'NONE',  ( -4.458734124999997661, -4.479166665301070438, 2.574251347313722516 ) ) ;
#32387=VERTEX_POINT ( 'NONE', #38934 ) ;
#32388=CARTESIAN_POINT ( 'NONE',  ( -2.500000000000000444, -86.04166666393547303, -4.330127018922193649 ) ) ;
#32389=CARTESIAN_POINT ( 'NONE',  ( -4.458734124999998549, -95.22916666530106511, 2.574251347313722516 ) ) ;
#32391=CARTESIAN_POINT ( 'NONE',  ( -4.458734124999998549, -85.47916666530106511, 2.574251347313722516 ) ) ;
#32395=CARTESIAN_POINT ( 'NONE',  ( 2.229367062499998831, -12.64583333196774007, -3.861377020970580887 ) ) ;
#32396=CARTESIAN_POINT ( 'NONE',  ( -2.229367062500000163, 15.27083333469892779, -3.861377020970580443 ) ) ;
#32397=CARTESIAN_POINT ( 'NONE',  ( -4.458734124999999437, -53.64583333196773651, -2.574251347313719407 ) ) ;
#32401=CARTESIAN_POINT ( 'NONE',  ( -2.499999999999996447, -38.83333333333332860, 4.330127018922195425 ) ) ;
#32405=CARTESIAN_POINT ( 'NONE',  ( 0.000000000000000000, -120.0000000000000000, 0.000000000000000000 ) ) ;
#32406=CARTESIAN_POINT ( 'NONE',  ( -4.458734124999998549, -79.22916666530107932, 2.574251347313722516 ) ) ;
#32407=CARTESIAN_POINT ( 'NONE',  ( 2.229367062499998831, 22.10416666803225993, -3.861377020970580887 ) ) ;
#32410=CYLINDRICAL_SURFACE ( 'NONE', #48241, 5.000000000000000000 ) ;
#32411=DIRECTION ( 'NONE',  ( -0.000000000000000000, 1.000000000000000000, -0.000000000000000000 ) ) ;
#32413=CARTESIAN_POINT ( 'NONE',  ( 2.500000000000002220, -65.66666666666667140, 4.330127018922192761 ) ) ;
#32414=CYLINDRICAL_SURFACE ( 'NONE', #31592, 5.000000000000000000 ) ;
#32416=ORIENTED_EDGE ( 'NONE', *, *, #31536, .F. ) ;
#32419=CARTESIAN_POINT ( 'NONE',  ( -2.499999999999996447, -71.83333333333332860, 4.330127018922195425 ) ) ;
#32430=ORIENTED_EDGE ( 'NONE', *, *, #57897, .T. ) ;
#32433=CARTESIAN_POINT ( 'NONE',  ( 2.229367062499998831, -51.89583333196773651, -3.861377020970580887 ) ) ;
#32436=ORIENTED_EDGE ( 'NONE', *, *, #46061, .F. ) ;
#32442=CARTESIAN_POINT ( 'NONE',  ( 2.229367062500001939, -98.22916666530105090, 3.861377020970579999 ) ) ;
#32447=DIRECTION ( 'NONE',  ( -0.000000000000000000, 1.000000000000000000, -0.000000000000000000 ) ) ;
#32448=CARTESIAN_POINT ( 'NONE',  ( -3.152548672688508926E-16, -6.562499998634404363, -5.148502694627439702 ) ) ;
#32449=CARTESIAN_POINT ( 'NONE',  ( -4.458734124999997661, -96.47916666530105090, 2.574251347313722516 ) ) ;
#32451=CARTESIAN_POINT ( 'NONE',  ( 4.458734124999999437, -22.06249999863440436, -5.460374474430324690E-16 ) ) ;
#32455=CARTESIAN_POINT ( 'NONE',  ( -2.480964764533239819E-13, -72.75000000000000000, 5.000000000000000000 ) ) ;
#32456=CARTESIAN_POINT ( 'NONE',  ( -5.000000000000000000, 17.00000000000000000, 0.000000000000000000 ) ) ;
#32458=CARTESIAN_POINT ( 'NONE',  ( 4.458734125000000326, 8.854166668032261711, 2.574251347313718519 ) ) ;
#32459=ORIENTED_EDGE ( 'NONE', *, *, #34267, .F. ) ;
#32460=CARTESIAN_POINT ( 'NONE',  ( -5.000000000000000000, -81.00000000000000000, 0.000000000000000000 ) ) ;
#32461=CARTESIAN_POINT ( 'NONE',  ( -6.972266317189433020E-16, -66.12499999726881583, -5.000000000000000000 ) ) ;
#32462=CARTESIAN_POINT ( 'NONE',  ( 5.000000000000000000, -90.41666666666664298, -2.886751345948129988 ) ) ;
#32463=CARTESIAN_POINT ( 'NONE',  ( 2.229367062499998831, -26.64583333196774007, -3.861377020970580887 ) ) ;
#32464=CARTESIAN_POINT ( 'NONE',  ( -2.500000000000000444, 6.958333336064520758, -4.330127018922193649 ) ) ;
#32465=CARTESIAN_POINT ( 'NONE',  ( 2.229367062499998831, -69.89583333196773651, -3.861377020970580887 ) ) ;
#32471=CARTESIAN_POINT ( 'NONE',  ( 4.458734124999999437, 4.187500001365595637, -5.460374474430324690E-16 ) ) ;
#32475=CARTESIAN_POINT ( 'NONE',  ( -3.152548672688508926E-16, -73.56249999863440792, -5.148502694627439702 ) ) ;
#32477=CARTESIAN_POINT ( 'NONE',  ( -4.999999999999999112, 1.083333333333331927, 2.886751345948131764 ) ) ;
#32480=CARTESIAN_POINT ( 'NONE',  ( -2.229367062499996610, -63.14583333196774362, 3.861377020970582219 ) ) ;
#32481=CARTESIAN_POINT ( 'NONE',  ( 5.000000000000000000, -101.3749999972688158, -6.123233995736766282E-16 ) ) ;
#32482=LINE ( 'NONE', #32805, #52214 ) ;
#32484=CARTESIAN_POINT ( 'NONE',  ( -4.458734124999997661, -108.4791666653010509, 2.574251347313722516 ) ) ;
#32486=CARTESIAN_POINT ( 'NONE',  ( 1.060575238724906964E-15, -50.75000000000000000, 5.773502691896257311 ) ) ;
#32490=CARTESIAN_POINT ( 'NONE',  ( 4.458734124999998549, -109.7291666653010793, -2.574251347313721627 ) ) ;
#32495=CARTESIAN_POINT ( 'NONE',  ( -2.500000000000000444, -6.166666666666667851, -4.330127018922193649 ) ) ;
#32498=ORIENTED_EDGE ( 'NONE', *, *, #7139, .F. ) ;
#32499=CARTESIAN_POINT ( 'NONE',  ( 1.339745962155615144, -100.5803417985302843, 4.999999999999999112 ) ) ;
#32501=ORIENTED_EDGE ( 'NONE', *, *, #53079, .T. ) ;
#32502=DIRECTION ( 'NONE',  ( 0.000000000000000000, 0.000000000000000000, 1.000000000000000000 ) ) ;
#32505=CARTESIAN_POINT ( 'NONE',  ( 9.457646018065525792E-16, -35.31249999863440792, 5.148502694627439702 ) ) ;
#32506=CARTESIAN_POINT ( 'NONE',  ( -2.500000000000000444, -11.04166666393547835, -4.330127018922193649 ) ) ;
#32509=CARTESIAN_POINT ( 'NONE',  ( -2.500000000000000444, -30.16666666666666785, -4.330127018922193649 ) ) ;
#32514=CARTESIAN_POINT ( 'NONE',  ( 1.339745962155615144, -83.58034179853031276, 4.999999999999999112 ) ) ;
#32515=CARTESIAN_POINT ( 'NONE',  ( -4.458734124999999437, -84.64583333196773651, -2.574251347313719407 ) ) ;
#32517=( BOUNDED_CURVE ( )  B_SPLINE_CURVE ( 2, ( #62751, #18672, #38295, #57923, #63064, #58223, #33778, #53396, #9327 ),
 .UNSPECIFIED., .F., .F. ) 
 B_SPLINE_CURVE_WITH_KNOTS ( ( 3, 2, 2, 2, 3 ),
 ( 0.4517857142857142905, 0.4523809523809523836, 0.4535714285714285698, 0.4547619047619047561, 0.4553571428571428492 ),
 .UNSPECIFIED. ) 
 CURVE ( )  GEOMETRIC_REPRESENTATION_ITEM ( )  RATIONAL_B_SPLINE_CURVE ( ( 0.9330127018922194093, 0.9330127018922194093, 1.000000000000000000, 0.8660254037844387076, 1.000000000000000000, 0.8660254037844387076, 1.000000000000000000, 0.9330127018922194093, 0.9330127018922194093 ) ) 
 REPRESENTATION_ITEM ( '' )  );
#32518=EDGE_LOOP ( 'NONE', ( #18264, #60839, #53920, #58550 ) ) ;
#32524=CARTESIAN_POINT ( 'NONE',  ( -2.229367062499996610, -11.39583333196773829, 3.861377020970582219 ) ) ;
#32527=CARTESIAN_POINT ( 'NONE',  ( -6.972266317189433020E-16, 2.875000002731185500, -5.000000000000000000 ) ) ;
#32528=CARTESIAN_POINT ( 'NONE',  ( 9.457646018065525792E-16, -6.312499998634404363, 5.148502694627439702 ) ) ;
#32529=DIRECTION ( 'NONE',  ( -0.000000000000000000, 1.000000000000000000, -0.000000000000000000 ) ) ;
#32532=CARTESIAN_POINT ( 'NONE',  ( 4.458734124999998549, 27.02083333469892068, -2.574251347313721627 ) ) ;
#32534=CARTESIAN_POINT ( 'NONE',  ( 2.229367062499998831, -87.64583333196773651, -3.861377020970580887 ) ) ;
#32535=CARTESIAN_POINT ( 'NONE',  ( -6.972266317189433020E-16, 15.75000000000000000, -5.000000000000000000 ) ) ;
#32536=CARTESIAN_POINT ( 'NONE',  ( 4.458734124999999437, -6.812499998634404363, -5.460374474430324690E-16 ) ) ;
#32539=EDGE_CURVE ( 'NONE', #60194, #30770, #16094, .T. ) ;
#32541=CARTESIAN_POINT ( 'NONE',  ( -2.500000000000000444, -37.04166666393548013, -4.330127018922193649 ) ) ;
#32542=DIRECTION ( 'NONE',  ( -0.000000000000000000, 1.000000000000000000, -0.000000000000000000 ) ) ;
#32543=CARTESIAN_POINT ( 'NONE',  ( -3.152548672688508926E-16, 24.43750000136559564, -5.148502694627439702 ) ) ;
#32544=CARTESIAN_POINT ( 'NONE',  ( -5.000000000000000000, -95.08333333333332860, -2.886751345948128211 ) ) ;
#32545=( BOUNDED_CURVE ( )  B_SPLINE_CURVE ( 2, ( #40950, #16519, #36141, #7825, #23241, #12637, #33212, #8457, #51571 ),
 .UNSPECIFIED., .F., .F. ) 
 B_SPLINE_CURVE_WITH_KNOTS ( ( 3, 2, 2, 2, 3 ),
 ( 0.6446428571428571841, 0.6452380952380952772, 0.6464285714285714635, 0.6476190476190476497, 0.6482142857142857428 ),
 .UNSPECIFIED. ) 
 CURVE ( )  GEOMETRIC_REPRESENTATION_ITEM ( )  RATIONAL_B_SPLINE_CURVE ( ( 0.9330127018922194093, 0.9330127018922194093, 1.000000000000000000, 0.8660254037844387076, 1.000000000000000000, 0.8660254037844387076, 1.000000000000000000, 0.9330127018922194093, 0.9330127018922194093 ) ) 
 REPRESENTATION_ITEM ( '' )  );
#32547=CARTESIAN_POINT ( 'NONE',  ( 2.229367062500001939, -56.97916666530107932, 3.861377020970579999 ) ) ;
#32549=AXIS2_PLACEMENT_3D ( 'NONE', #40928, #26785, #17131 ) ;
#32551=CARTESIAN_POINT ( 'NONE',  ( -4.999999999999999112, 13.08333333333333037, 2.886751345948131764 ) ) ;
#32553=CARTESIAN_POINT ( 'NONE',  ( 1.975475456537005874E-15, -45.74999999999999289, 5.000000000000000000 ) ) ;
#32554=CARTESIAN_POINT ( 'NONE',  ( -3.152548672688508926E-16, -45.56249999863439371, -5.148502694627439702 ) ) ;
#32555=CARTESIAN_POINT ( 'NONE',  ( 5.000000000000000888, -85.45833333060213022, 2.886751345948126879 ) ) ;
#32556=VECTOR ( 'NONE', #22948, 1000.000000000000000 ) ;
#32560=CARTESIAN_POINT ( 'NONE',  ( -6.972266317189433020E-16, -92.24999999999998579, -5.000000000000000000 ) ) ;
#32562=CARTESIAN_POINT ( 'NONE',  ( -4.458734124999999437, -84.64583333196773651, -2.574251347313719407 ) ) ;
#32564=CARTESIAN_POINT ( 'NONE',  ( 5.000000000000000000, -31.41666666666667140, -2.886751345948129988 ) ) ;
#32565=CARTESIAN_POINT ( 'NONE',  ( -1.339745962155610925, 24.20534180126147206, 5.000000000000000000 ) ) ;
#32566=ORIENTED_EDGE ( 'NONE', *, *, #26111, .F. ) ;
#32569=CARTESIAN_POINT ( 'NONE',  ( 4.458734124999999437, -96.81249999863440792, -5.460374474430324690E-16 ) ) ;
#32570=CARTESIAN_POINT ( 'NONE',  ( -2.229367062499996610, 8.604166668032261711, 3.861377020970582219 ) ) ;
#32571=CARTESIAN_POINT ( 'NONE',  ( -2.499999999999996447, 12.29166666939785202, 4.330127018922195425 ) ) ;
#32572=( BOUNDED_CURVE ( )  B_SPLINE_CURVE ( 2, ( #36, #29271, #23531, #19952, #48901, #4846, #350, #43755, #24465 ),
 .UNSPECIFIED., .F., .F. ) 
 B_SPLINE_CURVE_WITH_KNOTS ( ( 3, 2, 2, 2, 3 ),
 ( 0.8410714285714285809, 0.8416666666666666741, 0.8428571428571428603, 0.8440476190476190466, 0.8446428571428571397 ),
 .UNSPECIFIED. ) 
 CURVE ( )  GEOMETRIC_REPRESENTATION_ITEM ( )  RATIONAL_B_SPLINE_CURVE ( ( 0.9330127018922194093, 0.9330127018922194093, 1.000000000000000000, 0.8660254037844387076, 1.000000000000000000, 0.8660254037844387076, 1.000000000000000000, 0.9330127018922194093, 0.9330127018922194093 ) ) 
 REPRESENTATION_ITEM ( '' )  );
#32573=CARTESIAN_POINT ( 'NONE',  ( -5.000000000000000000, -28.95833333060214443, -2.886751345948128211 ) ) ;
#32576=CARTESIAN_POINT ( 'NONE',  ( -1.339745962155610925, 15.33034180399266511, 5.000000000000000000 ) ) ;
#32577=CARTESIAN_POINT ( 'NONE',  ( -4.999999999999999112, -79.91666666666667140, 2.886751345948131764 ) ) ;
#32580=CARTESIAN_POINT ( 'NONE',  ( -5.000000000000000000, -12.87499999726881050, 0.000000000000000000 ) ) ;
#32583=LINE ( 'NONE', #11686, #32556 ) ;
#32585=CARTESIAN_POINT ( 'NONE',  ( 2.229367062500001939, -22.22916666530107221, 3.861377020970579999 ) ) ;
#32595=CARTESIAN_POINT ( 'NONE',  ( -4.458734124999999437, -65.64583333196773651, -2.574251347313719407 ) ) ;
#32596=CARTESIAN_POINT ( 'NONE',  ( 5.000000000000000000, -7.291666663935481907, -2.886751345948130876 ) ) ;
#32604=AXIS2_PLACEMENT_3D ( 'NONE', #49249, #63110, #24172 ) ;
#32607=CARTESIAN_POINT ( 'NONE',  ( 2.229367062500001939, 9.020833334698927786, 3.861377020970579999 ) ) ;
#32611=EDGE_LOOP ( 'NONE', ( #53235, #35119, #27814, #9230 ) ) ;
#32612=CARTESIAN_POINT ( 'NONE',  ( 4.458734124999999437, -69.81249999863439371, -5.460374474430324690E-16 ) ) ;
#32614=CARTESIAN_POINT ( 'NONE',  ( 2.499999999999998668, -10.20833333060214621, -4.330127018922193649 ) ) ;
#32615=CARTESIAN_POINT ( 'NONE',  ( -3.152548672688508926E-16, 8.437500001365595637, -5.148502694627439702 ) ) ;
#32617=CARTESIAN_POINT ( 'NONE',  ( 4.458734124999999437, -62.06249999863440792, -5.460374474430324690E-16 ) ) ;
#32618=CARTESIAN_POINT ( 'NONE',  ( 2.500000000000002220, -19.54166666393548013, 4.330127018922192761 ) ) ;
#32620=CARTESIAN_POINT ( 'NONE',  ( -5.000000000000000000, -18.99999999999999645, 0.000000000000000000 ) ) ;
#32622=CARTESIAN_POINT ( 'NONE',  ( 5.000000000000000888, 19.54166666939785202, 2.886751345948126879 ) ) ;
#32624=CARTESIAN_POINT ( 'NONE',  ( -2.229367062500000163, -38.47916666530107221, -3.861377020970580443 ) ) ;
#32625=CARTESIAN_POINT ( 'NONE',  ( 2.229367062499998831, -21.89583333196774007, -3.861377020970580887 ) ) ;
#32628=CARTESIAN_POINT ( 'NONE',  ( 4.458734124999999437, -106.8124999986343937, -5.460374474430324690E-16 ) ) ;
#32631=CARTESIAN_POINT ( 'NONE',  ( -4.458734124999999437, -107.5624999986343937, 0.000000000000000000 ) ) ;
#32632=CARTESIAN_POINT ( 'NONE',  ( 4.458734125000001214, -30.89583333196773296, 2.574251347313718519 ) ) ;
#32633=CARTESIAN_POINT ( 'NONE',  ( -5.000000000000000000, -67.87499999726881583, 0.000000000000000000 ) ) ;
#32636=CARTESIAN_POINT ( 'NONE',  ( 4.458734125000000326, -29.89583333196773651, 2.574251347313718519 ) ) ;
#32637=CARTESIAN_POINT ( 'NONE',  ( -3.152548672688508926E-16, -69.81249999863439371, -5.148502694627439702 ) ) ;
#32641=CARTESIAN_POINT ( 'NONE',  ( -5.000000000000000000, -17.08333333333333215, -2.886751345948128211 ) ) ;
#32647=CARTESIAN_POINT ( 'NONE',  ( -6.972266317189433020E-16, -84.12499999726880162, -5.000000000000000000 ) ) ;
#32648=CARTESIAN_POINT ( 'NONE',  ( 2.500000000000002220, -81.54166666393547303, 4.330127018922192761 ) ) ;
#32650=EDGE_CURVE ( 'NONE', #23818, #44517, #25511, .T. ) ;
#32652=CARTESIAN_POINT ( 'NONE',  ( 2.500000000000002220, -76.54166666393547303, 4.330127018922192761 ) ) ;
#32658=ORIENTED_EDGE ( 'NONE', *, *, #22111, .F. ) ;
#32671=CARTESIAN_POINT ( 'NONE',  ( -4.999999999999998224, -38.79166666393548013, 2.886751345948131764 ) ) ;
#32675=ORIENTED_EDGE ( 'NONE', *, *, #21760, .T. ) ;
#32678=CARTESIAN_POINT ( 'NONE',  ( -4.458734124999999437, -81.39583333196773651, -2.574251347313719407 ) ) ;
#32679=CARTESIAN_POINT ( 'NONE',  ( -4.458734124999998549, 25.77083333469892779, 2.574251347313722516 ) ) ;
#32681=EDGE_CURVE ( 'NONE', #30563, #57684, #47680, .T. ) ;
#32682=ORIENTED_EDGE ( 'NONE', *, *, #30747, .T. ) ;
#32687=CARTESIAN_POINT ( 'NONE',  ( 5.000000000000000000, 0.7083333360645185373, -2.886751345948130876 ) ) ;
#32689=CARTESIAN_POINT ( 'NONE',  ( 4.458734124999998549, -55.72916666530107221, -2.574251347313721627 ) ) ;
#32690=CARTESIAN_POINT ( 'NONE',  ( 1.339745962155615144, 21.29465819873852084, 4.999999999999999112 ) ) ;
#32691=CARTESIAN_POINT ( 'NONE',  ( -4.458734124999999437, 23.68750000136559564, 0.000000000000000000 ) ) ;
#32692=AXIS2_PLACEMENT_3D ( 'NONE', #41045, #4340, #52917 ) ;
#32694=CARTESIAN_POINT ( 'NONE',  ( 5.000000000000000000, -107.4166666666666572, -2.886751345948129988 ) ) ;
#32696=CARTESIAN_POINT ( 'NONE',  ( -4.458734124999999437, -41.56249999863440081, 0.000000000000000000 ) ) ;
#32697=CARTESIAN_POINT ( 'NONE',  ( -3.535250795749689387E-16, -2.124999997268814944, -5.773502691896257311 ) ) ;
#32701=ADVANCED_FACE ( 'NONE', ( #51472 ), #36350, .T. ) ;
#32702=CARTESIAN_POINT ( 'NONE',  ( -2.229367062500000163, -102.4791666653010651, -3.861377020970580443 ) ) ;
#32703=CARTESIAN_POINT ( 'NONE',  ( -3.152548672688508926E-16, -6.812499998634404363, -5.148502694627439702 ) ) ;
#32704=EDGE_LOOP ( 'NONE', ( #45839, #19832, #35520, #29026 ) ) ;
#32705=CARTESIAN_POINT ( 'NONE',  ( 0.000000000000000000, -120.0000000000000000, 0.000000000000000000 ) ) ;
#32706=CARTESIAN_POINT ( 'NONE',  ( -2.229367062500000163, -94.47916666530106511, -3.861377020970580443 ) ) ;
#32707=EDGE_CURVE ( 'NONE', #44977, #35740, #7866, .T. ) ;
#32709=CARTESIAN_POINT ( 'NONE',  ( -4.458734124999999437, -91.56249999863440792, 0.000000000000000000 ) ) ;
#32713=CARTESIAN_POINT ( 'NONE',  ( 9.457646018065525792E-16, -12.06249999863440081, 5.148502694627439702 ) ) ;
#32714=CARTESIAN_POINT ( 'NONE',  ( 4.458734125000001214, 11.85416666803225993, 2.574251347313718519 ) ) ;
#32715=CARTESIAN_POINT ( 'NONE',  ( -4.458734124999999437, -55.56249999863440081, 0.000000000000000000 ) ) ;
#32718=CARTESIAN_POINT ( 'NONE',  ( 2.500000000000002220, -109.5416666639354730, 4.330127018922192761 ) ) ;
#32723=CARTESIAN_POINT ( 'NONE',  ( 0.000000000000000000, -120.0000000000000000, 0.000000000000000000 ) ) ;
#32725=CARTESIAN_POINT ( 'NONE',  ( -2.229367062499996610, -81.14583333196773651, 3.861377020970582219 ) ) ;
#32726=CARTESIAN_POINT ( 'NONE',  ( 2.229367062499998831, 24.10416666803225993, -3.861377020970580887 ) ) ;
#32731=CARTESIAN_POINT ( 'NONE',  ( -2.500000000000000444, -72.16666666666667140, -4.330127018922193649 ) ) ;
#32732=CARTESIAN_POINT ( 'NONE',  ( 5.000000000000000000, -63.29166666393547303, -2.886751345948130876 ) ) ;
#32734=ORIENTED_EDGE ( 'NONE', *, *, #50321, .T. ) ;
#32736=AXIS2_PLACEMENT_3D ( 'NONE', #18097, #37721, #2376 ) ;
#32740=AXIS2_PLACEMENT_3D ( 'NONE', #1048, #11297, #20654 ) ;
#32741=DIRECTION ( 'NONE',  ( 0.000000000000000000, 0.000000000000000000, 1.000000000000000000 ) ) ;
#32751=CARTESIAN_POINT ( 'NONE',  ( 4.458734124999999437, -51.06249999863440792, -5.460374474430324690E-16 ) ) ;
#32752=( BOUNDED_CURVE ( )  B_SPLINE_CURVE ( 2, ( #8809, #28425, #53498, #18763, #23916, #38085, #14256, #48039, #3682 ),
 .UNSPECIFIED., .F., .F. ) 
 B_SPLINE_CURVE_WITH_KNOTS ( ( 3, 2, 2, 2, 3 ),
 ( 0.9625000000000000222, 0.9630952380952381153, 0.9642857142857143016, 0.9654761904761904878, 0.9660714285714285809 ),
 .UNSPECIFIED. ) 
 CURVE ( )  GEOMETRIC_REPRESENTATION_ITEM ( )  RATIONAL_B_SPLINE_CURVE ( ( 0.9330127018922194093, 0.9330127018922194093, 1.000000000000000000, 0.8660254037844387076, 1.000000000000000000, 0.8660254037844387076, 1.000000000000000000, 0.9330127018922194093, 0.9330127018922194093 ) ) 
 REPRESENTATION_ITEM ( '' )  );
#32754=CARTESIAN_POINT ( 'NONE',  ( 1.975475456537005874E-15, -54.62499999726880873, 5.000000000000000000 ) ) ;
#32762=CARTESIAN_POINT ( 'NONE',  ( -4.458734124999998549, -98.47916666530105090, 2.574251347313722516 ) ) ;
#32763=CARTESIAN_POINT ( 'NONE',  ( -5.000000000000000000, -26.87499999726881583, 0.000000000000000000 ) ) ;
#32767=CARTESIAN_POINT ( 'NONE',  ( -1.339745962155610925, 1.330341803992665106, 5.000000000000000000 ) ) ;
#32768=CARTESIAN_POINT ( 'NONE',  ( -4.458734124999999437, -7.395833331967734736, -2.574251347313719407 ) ) ;
#32769=CARTESIAN_POINT ( 'NONE',  ( -4.458734124999999437, -95.56249999863440792, 0.000000000000000000 ) ) ;
#32771=CARTESIAN_POINT ( 'NONE',  ( -2.229367062499996610, -29.39583333196774007, 3.861377020970582219 ) ) ;
#32772=CARTESIAN_POINT ( 'NONE',  ( -2.500000000000000444, -67.16666666666667140, -4.330127018922193649 ) ) ;
#32776=CARTESIAN_POINT ( 'NONE',  ( -6.972266317189433020E-16, -91.24999999999998579, -5.000000000000000000 ) ) ;
#32779=VECTOR ( 'NONE', #13345, 1000.000000000000000 ) ;
#32780=CARTESIAN_POINT ( 'NONE',  ( -3.152548672688508926E-16, 8.187500001365595637, -5.148502694627439702 ) ) ;
#32785=CARTESIAN_POINT ( 'NONE',  ( -5.000000000000000000, -88.00000000000000000, 0.000000000000000000 ) ) ;
#32786=CARTESIAN_POINT ( 'NONE',  ( 4.458734125000001214, -23.89583333196774007, 2.574251347313718519 ) ) ;
#32787=CARTESIAN_POINT ( 'NONE',  ( -5.000000000000000000, 7.125000002731185944, 0.000000000000000000 ) ) ;
#32788=CARTESIAN_POINT ( 'NONE',  ( -4.458734124999999437, -76.64583333196775072, -2.574251347313719407 ) ) ;
#32791=CARTESIAN_POINT ( 'NONE',  ( 2.499999999999998668, -79.20833333060213022, -4.330127018922193649 ) ) ;
#32793=EDGE_CURVE ( 'NONE', #14226, #33683, #58384, .T. ) ;
#32794=CARTESIAN_POINT ( 'NONE',  ( 2.229367062500001939, 1.020833334698927120, 3.861377020970579999 ) ) ;
#32795=DIRECTION ( 'NONE',  ( -0.000000000000000000, 1.000000000000000000, -0.000000000000000000 ) ) ;
#32796=CARTESIAN_POINT ( 'NONE',  ( 1.975475456537005874E-15, -99.62499999726880162, 5.000000000000000000 ) ) ;
#32798=CARTESIAN_POINT ( 'NONE',  ( 4.458734124999998549, -72.72916666530106511, -2.574251347313721627 ) ) ;
#32800=CARTESIAN_POINT ( 'NONE',  ( -2.499999999999996447, -7.833333333333331261, 4.330127018922195425 ) ) ;
#32803=CARTESIAN_POINT ( 'NONE',  ( 4.458734124999999437, -63.81249999863440792, -5.460374474430324690E-16 ) ) ;
#32804=CARTESIAN_POINT ( 'NONE',  ( 5.000000000000000000, -101.2916666639354730, -2.886751345948129988 ) ) ;
#32805=CARTESIAN_POINT ( 'NONE',  ( 0.000000000000000000, -120.0000000000000000, 5.000000000000000000 ) ) ;
#32807=DIRECTION ( 'NONE',  ( -0.000000000000000000, 1.000000000000000000, -0.000000000000000000 ) ) ;
#32808=CARTESIAN_POINT ( 'NONE',  ( -4.458734124999999437, -103.6458333319677365, -2.574251347313719407 ) ) ;
#32810=CARTESIAN_POINT ( 'NONE',  ( -5.000000000000000000, -54.99999999999999289, 0.000000000000000000 ) ) ;
#32814=CARTESIAN_POINT ( 'NONE',  ( 5.000000000000000888, -94.58333333333332860, 2.886751345948126879 ) ) ;
#32823=CARTESIAN_POINT ( 'NONE',  ( 1.339745962155615144, -81.70534180126146850, 4.999999999999999112 ) ) ;
#32829=CARTESIAN_POINT ( 'NONE',  ( 2.229367062499998831, -33.89583333196772941, -3.861377020970580887 ) ) ;
#32837=ADVANCED_FACE ( 'NONE', ( #27330 ), #12225, .T. ) ;
#32838=CARTESIAN_POINT ( 'NONE',  ( 2.500000000000002220, -26.66666666666666430, 4.330127018922192761 ) ) ;
#32839=CARTESIAN_POINT ( 'NONE',  ( 4.458734124999998549, -81.97916666530106511, -2.574251347313721627 ) ) ;
#32840=LINE ( 'NONE', #21925, #13270 ) ;
#32841=ORIENTED_EDGE ( 'NONE', *, *, #31517, .F. ) ;
#32846=ORIENTED_EDGE ( 'NONE', *, *, #53511, .F. ) ;
#32848=( BOUNDED_CURVE ( )  B_SPLINE_CURVE ( 2, ( #46050, #1690, #49911, #45413, #1381, #36398, #20981, #2013, #5865 ),
 .UNSPECIFIED., .F., .F. ) 
 B_SPLINE_CURVE_WITH_KNOTS ( ( 3, 2, 2, 2, 3 ),
 ( 0.3303571428571428492, 0.3309523809523809423, 0.3321428571428571286, 0.3333333333333333148, 0.3339285714285714080 ),
 .UNSPECIFIED. ) 
 CURVE ( )  GEOMETRIC_REPRESENTATION_ITEM ( )  RATIONAL_B_SPLINE_CURVE ( ( 0.9330127018922194093, 0.9330127018922194093, 1.000000000000000000, 0.8660254037844387076, 1.000000000000000000, 0.8660254037844387076, 1.000000000000000000, 0.9330127018922194093, 0.9330127018922194093 ) ) 
 REPRESENTATION_ITEM ( '' )  );
#32849=CARTESIAN_POINT ( 'NONE',  ( 2.499999999999998668, 17.66666666666666430, -4.330127018922193649 ) ) ;
#32850=CARTESIAN_POINT ( 'NONE',  ( 2.229367062500001939, -14.22916666530107221, 3.861377020970579999 ) ) ;
#32851=CARTESIAN_POINT ( 'NONE',  ( 1.975475456537005874E-15, -34.75000000000000000, 5.000000000000000000 ) ) ;
#32855=CARTESIAN_POINT ( 'NONE',  ( -4.458734124999997661, 28.52083333469892423, 2.574251347313722516 ) ) ;
#32856=ORIENTED_EDGE ( 'NONE', *, *, #27440, .T. ) ;
#32857=CARTESIAN_POINT ( 'NONE',  ( 4.458734124999999437, -92.81249999863440792, -5.460374474430324690E-16 ) ) ;
#32858=CARTESIAN_POINT ( 'NONE',  ( -2.499999999999996447, -67.83333333333332860, 4.330127018922195425 ) ) ;
#32859=CARTESIAN_POINT ( 'NONE',  ( -5.000000000000000000, -63.08333333333331439, -2.886751345948128211 ) ) ;
#32860=CARTESIAN_POINT ( 'NONE',  ( -2.229367062499996610, -6.145833331967740953, 3.861377020970582219 ) ) ;
#32861=CARTESIAN_POINT ( 'NONE',  ( 1.339745962155615144, -51.70534180126148271, 4.999999999999999112 ) ) ;
#32862=FACE_OUTER_BOUND ( 'NONE', #49501, .T. ) ;
#32864=CARTESIAN_POINT ( 'NONE',  ( -3.535250795749689387E-16, -35.12499999726881583, -5.773502691896257311 ) ) ;
#32865=CARTESIAN_POINT ( 'NONE',  ( 0.000000000000000000, -120.0000000000000000, 0.000000000000000000 ) ) ;
#32866=CARTESIAN_POINT ( 'NONE',  ( -4.458734124999999437, 16.68750000136559564, 0.000000000000000000 ) ) ;
#32867=DIRECTION ( 'NONE',  ( 0.000000000000000000, 0.000000000000000000, 1.000000000000000000 ) ) ;
#32869=CARTESIAN_POINT ( 'NONE',  ( 4.458734124999998549, -58.72916666530106511, -2.574251347313721627 ) ) ;
#32872=CARTESIAN_POINT ( 'NONE',  ( 5.000000000000000888, 10.41666666666666607, 2.886751345948126879 ) ) ;
#32876=CARTESIAN_POINT ( 'NONE',  ( 4.458734125000001214, -46.89583333196773651, 2.574251347313718519 ) ) ;
#32877=CARTESIAN_POINT ( 'NONE',  ( 5.000000000000000888, -82.45833333060214443, 2.886751345948126879 ) ) ;
#32879=CARTESIAN_POINT ( 'NONE',  ( -1.339745962155613812, -17.20534180126147916, -5.000000000000000000 ) ) ;
#32881=CARTESIAN_POINT ( 'NONE',  ( 2.229367062500001939, -90.22916666530106511, 3.861377020970579999 ) ) ;
#32883=CARTESIAN_POINT ( 'NONE',  ( -2.500000000000000444, -33.16666666666666430, -4.330127018922193649 ) ) ;
#32885=ORIENTED_EDGE ( 'NONE', *, *, #31527, .T. ) ;
#32887=ORIENTED_EDGE ( 'NONE', *, *, #10339, .F. ) ;
#32888=CARTESIAN_POINT ( 'NONE',  ( -3.152548672688508926E-16, -96.56249999863439371, -5.148502694627439702 ) ) ;
#32889=CARTESIAN_POINT ( 'NONE',  ( -2.229367062499996610, 7.604166668032260823, 3.861377020970582219 ) ) ;
#32890=CARTESIAN_POINT ( 'NONE',  ( 2.500000000000002220, 10.45833333606451987, 4.330127018922192761 ) ) ;
#32891=DIRECTION ( 'NONE',  ( -0.000000000000000000, 1.000000000000000000, -0.000000000000000000 ) ) ;
#32893=EDGE_CURVE ( 'NONE', #55181, #32387, #44852, .T. ) ;
#32897=CARTESIAN_POINT ( 'NONE',  ( 5.000000000000000000, -81.41666666666667140, -2.886751345948129988 ) ) ;
#32902=CYLINDRICAL_SURFACE ( 'NONE', #8364, 5.000000000000000000 ) ;
#32905=CARTESIAN_POINT ( 'NONE',  ( 1.975475456537005874E-15, 6.375000002731185944, 5.000000000000000000 ) ) ;
#32906=( BOUNDED_CURVE ( )  B_SPLINE_CURVE ( 2, ( #36475, #46127, #16223, #50635, #6573, #35846, #60935, #60620, #51286 ),
 .UNSPECIFIED., .F., .F. ) 
 B_SPLINE_CURVE_WITH_KNOTS ( ( 3, 2, 2, 2, 3 ),
 ( 0.9517857142857142350, 0.9523809523809523281, 0.9535714285714286254, 0.9547619047619048116, 0.9553571428571429047 ),
 .UNSPECIFIED. ) 
 CURVE ( )  GEOMETRIC_REPRESENTATION_ITEM ( )  RATIONAL_B_SPLINE_CURVE ( ( 0.9330127018922194093, 0.9330127018922194093, 1.000000000000000000, 0.8660254037844387076, 1.000000000000000000, 0.8660254037844387076, 1.000000000000000000, 0.9330127018922194093, 0.9330127018922194093 ) ) 
 REPRESENTATION_ITEM ( '' )  );
#32907=CARTESIAN_POINT ( 'NONE',  ( -4.458734124999999437, -20.64583333196774007, -2.574251347313719407 ) ) ;
#32918=CARTESIAN_POINT ( 'NONE',  ( 2.229367062499998831, -67.89583333196773651, -3.861377020970580887 ) ) ;
#32919=FACE_OUTER_BOUND ( 'NONE', #60482, .T. ) ;
#32925=CARTESIAN_POINT ( 'NONE',  ( 4.458734124999999437, 0.9375000013655959696, -5.460374474430324690E-16 ) ) ;
#32927=CARTESIAN_POINT ( 'NONE',  ( -6.972266317189433020E-16, -45.24999999999999289, -5.000000000000000000 ) ) ;
#32928=CARTESIAN_POINT ( 'NONE',  ( -4.458734124999999437, 3.687500001365594748, 0.000000000000000000 ) ) ;
#32931=CARTESIAN_POINT ( 'NONE',  ( 1.339745962155612702, -92.16965819600733312, -5.000000000000000000 ) ) ;
#32934=CARTESIAN_POINT ( 'NONE',  ( -2.229367062499996610, -74.14583333196773651, 3.861377020970582219 ) ) ;
#32935=CARTESIAN_POINT ( 'NONE',  ( 0.000000000000000000, -120.0000000000000000, 5.000000000000000000 ) ) ;
#32936=CARTESIAN_POINT ( 'NONE',  ( 2.229367062500001939, 9.020833334698927786, 3.861377020970579999 ) ) ;
#32938=CARTESIAN_POINT ( 'NONE',  ( -4.458734124999999437, -62.64583333196774362, -2.574251347313719407 ) ) ;
#32939=CARTESIAN_POINT ( 'NONE',  ( 2.499999999999998668, -18.20833333060214798, -4.330127018922193649 ) ) ;
#32941=CARTESIAN_POINT ( 'NONE',  ( 1.975475456537005874E-15, -28.62499999726881583, 5.000000000000000000 ) ) ;
#32942=CARTESIAN_POINT ( 'NONE',  ( 2.500000000000002220, -65.66666666666667140, 4.330127018922192761 ) ) ;
#32943=CARTESIAN_POINT ( 'NONE',  ( 0.000000000000000000, -120.0000000000000000, 0.000000000000000000 ) ) ;
#32944=CARTESIAN_POINT ( 'NONE',  ( 2.229367062499998831, -39.64583333196773651, -3.861377020970580887 ) ) ;
#32945=CARTESIAN_POINT ( 'NONE',  ( 4.458734124999999437, -26.06249999863440792, -5.460374474430324690E-16 ) ) ;
#32946=( BOUNDED_CURVE ( )  B_SPLINE_CURVE ( 2, ( #57979, #18421, #43794, #48938, #19038, #3640, #33840, #13904, #8771 ),
 .UNSPECIFIED., .F., .F. ) 
 B_SPLINE_CURVE_WITH_KNOTS ( ( 3, 2, 2, 2, 3 ),
 ( 0.03392857142857143293, 0.03452380952380952606, 0.03571428571428571230, 0.03690476190476190549, 0.03750000000000000555 ),
 .UNSPECIFIED. ) 
 CURVE ( )  GEOMETRIC_REPRESENTATION_ITEM ( )  RATIONAL_B_SPLINE_CURVE ( ( 0.9330127018922194093, 0.9330127018922197424, 1.000000000000000000, 0.8660254037844387076, 1.000000000000000000, 0.8660254037844387076, 1.000000000000000000, 0.9330127018922189652, 0.9330127018922194093 ) ) 
 REPRESENTATION_ITEM ( '' )  );
#32948=CARTESIAN_POINT ( 'NONE',  ( 5.000000000000000000, 29.58333333333332860, -2.886751345948129988 ) ) ;
#32951=CARTESIAN_POINT ( 'NONE',  ( 2.229367062499998831, -107.8958333319677365, -3.861377020970580887 ) ) ;
#32952=CARTESIAN_POINT ( 'NONE',  ( -4.458734124999999437, -31.39583333196773296, -2.574251347313719407 ) ) ;
#32953=CARTESIAN_POINT ( 'NONE',  ( 2.499999999999998668, -66.20833333060213022, -4.330127018922193649 ) ) ;
#32956=CARTESIAN_POINT ( 'NONE',  ( -2.229367062499996610, -30.14583333196773651, 3.861377020970582219 ) ) ;
#32957=CARTESIAN_POINT ( 'NONE',  ( 2.229367062500001939, -70.22916666530107932, 3.861377020970579999 ) ) ;
#32961=CARTESIAN_POINT ( 'NONE',  ( 0.000000000000000000, -120.0000000000000000, 0.000000000000000000 ) ) ;
#32962=CARTESIAN_POINT ( 'NONE',  ( 5.000000000000000000, -16.41666666666667140, -2.886751345948129988 ) ) ;
#32964=VERTEX_POINT ( 'NONE', #10202 ) ;
#32968=CARTESIAN_POINT ( 'NONE',  ( 5.000000000000000888, 27.54166666939785557, 2.886751345948126879 ) ) ;
#32972=ADVANCED_FACE ( 'NONE', ( #40096 ), #45884, .T. ) ;
#32980=VERTEX_POINT ( 'NONE', #50073 ) ;
#32986=ORIENTED_EDGE ( 'NONE', *, *, #13712, .F. ) ;
#32989=EDGE_LOOP ( 'NONE', ( #58761, #35956, #15650, #34474 ) ) ;
#32990=CARTESIAN_POINT ( 'NONE',  ( -1.339745962155613812, -0.08034179853029406460, -5.000000000000000000 ) ) ;
#32991=CARTESIAN_POINT ( 'NONE',  ( -4.999999999999998224, -11.91666666666666607, 2.886751345948131764 ) ) ;
#32997=EDGE_CURVE ( 'NONE', #60061, #3585, #49360, .T. ) ;
#32998=CARTESIAN_POINT ( 'NONE',  ( 2.229367062500001939, -82.97916666530106511, 3.861377020970579999 ) ) ;
#32999=CARTESIAN_POINT ( 'NONE',  ( -4.458734124999998549, 22.77083333469892423, 2.574251347313722516 ) ) ;
#33005=CARTESIAN_POINT ( 'NONE',  ( 0.000000000000000000, -120.0000000000000000, 0.000000000000000000 ) ) ;
#33007=CARTESIAN_POINT ( 'NONE',  ( 1.339745962155586056, 4.294658198738518173, 5.000000000000015987 ) ) ;
#33008=CARTESIAN_POINT ( 'NONE',  ( 2.229367062499998831, -56.64583333196773651, -3.861377020970580887 ) ) ;
#33009=CARTESIAN_POINT ( 'NONE',  ( -6.972266317189433020E-16, 21.75000000000000000, -5.000000000000000000 ) ) ;
#33011=CARTESIAN_POINT ( 'NONE',  ( -2.229367062499996610, 21.85416666803226349, 3.861377020970582219 ) ) ;
#33012=CARTESIAN_POINT ( 'NONE',  ( 1.339745962155612702, -102.1696581960073331, -5.000000000000000000 ) ) ;
#33014=CARTESIAN_POINT ( 'NONE',  ( -4.458734124999999437, -45.56249999863440081, 0.000000000000000000 ) ) ;
#33016=CARTESIAN_POINT ( 'NONE',  ( 5.000000000000000000, -6.291666663935480130, -2.886751345948129988 ) ) ;
#33020=CARTESIAN_POINT ( 'NONE',  ( -2.229367062500000163, -104.4791666653010651, -3.861377020970580443 ) ) ;
#33021=CARTESIAN_POINT ( 'NONE',  ( -3.152548672688508926E-16, -11.81249999863440969, -5.148502694627439702 ) ) ;
#33024=CARTESIAN_POINT ( 'NONE',  ( -4.458734124999998549, -92.22916666530106511, 2.574251347313722516 ) ) ;
#33026=CARTESIAN_POINT ( 'NONE',  ( -4.458734124999998549, -94.47916666530106511, 2.574251347313722516 ) ) ;
#33027=CARTESIAN_POINT ( 'NONE',  ( -5.000000000000000000, -52.87499999726881583, 0.000000000000000000 ) ) ;
#33031=CARTESIAN_POINT ( 'NONE',  ( 4.458734125000000326, -14.89583333196773474, 2.574251347313718519 ) ) ;
#33032=CARTESIAN_POINT ( 'NONE',  ( -2.229367062499996610, 13.60416666803226171, 3.861377020970582219 ) ) ;
#33033=CARTESIAN_POINT ( 'NONE',  ( -3.152548672688508926E-16, -51.81249999863440081, -5.148502694627439702 ) ) ;
#33037=LINE ( 'NONE', #14658, #61719 ) ;
#33040=UNCERTAINTY_MEASURE_WITH_UNIT (LENGTH_MEASURE( 1.000000000000000082E-05 ), #13615, 'distance_accuracy_value', 'NONE');
#33042=CARTESIAN_POINT ( 'NONE',  ( 2.499999999999998668, 26.79166666939785202, -4.330127018922193649 ) ) ;
#33043=DIRECTION ( 'NONE',  ( 0.000000000000000000, 0.000000000000000000, 1.000000000000000000 ) ) ;
#33044=CARTESIAN_POINT ( 'NONE',  ( 9.457646018065525792E-16, -83.06249999863439371, 5.148502694627439702 ) ) ;
#33045=CARTESIAN_POINT ( 'NONE',  ( 9.457646018065525792E-16, 23.68750000136559564, 5.148502694627439702 ) ) ;
#33046=ADVANCED_FACE ( 'NONE', ( #10832 ), #59417, .T. ) ;
#33051=DIRECTION ( 'NONE',  ( 0.000000000000000000, 0.000000000000000000, 1.000000000000000000 ) ) ;
#33053=CARTESIAN_POINT ( 'NONE',  ( 5.000000000000000000, -67.50000000000000000, -6.123233995736766282E-16 ) ) ;
#33056=CARTESIAN_POINT ( 'NONE',  ( 2.499999999999998668, -18.20833333060214798, -4.330127018922193649 ) ) ;
#33058=CARTESIAN_POINT ( 'NONE',  ( 5.000000000000000000, -40.49999999999999289, -6.123233995736766282E-16 ) ) ;
#33061=DIRECTION ( 'NONE',  ( -0.000000000000000000, 1.000000000000000000, -0.000000000000000000 ) ) ;
#33062=EDGE_CURVE ( 'NONE', #25630, #55067, #31729, .T. ) ;
#33067=EDGE_CURVE ( 'NONE', #23303, #30363, #5413, .T. ) ;
#33072=CARTESIAN_POINT ( 'NONE',  ( -2.229367062499996610, -54.39583333196773651, 3.861377020970582219 ) ) ;
#33075=ORIENTED_EDGE ( 'NONE', *, *, #17013, .F. ) ;
#33081=CARTESIAN_POINT ( 'NONE',  ( 4.458734124999998549, -98.97916666530105090, -2.574251347313721627 ) ) ;
#33083=ORIENTED_EDGE ( 'NONE', *, *, #47502, .F. ) ;
#33086=CARTESIAN_POINT ( 'NONE',  ( 5.000000000000000888, -83.58333333333332860, 2.886751345948126879 ) ) ;
#33087=CARTESIAN_POINT ( 'NONE',  ( 2.229367062500001939, -8.979166665301075767, 3.861377020970579999 ) ) ;
#33088=CARTESIAN_POINT ( 'NONE',  ( 4.458734125000000326, -99.14583333196773651, 2.574251347313718519 ) ) ;
#33090=CARTESIAN_POINT ( 'NONE',  ( 4.458734125000001214, -26.14583333196774007, 2.574251347313718519 ) ) ;
#33094=CARTESIAN_POINT ( 'NONE',  ( 1.339745962155612702, -21.16965819600733312, -5.000000000000000000 ) ) ;
#33095=CARTESIAN_POINT ( 'NONE',  ( 2.499999999999998668, -88.20833333060214443, -4.330127018922193649 ) ) ;
#33097=CARTESIAN_POINT ( 'NONE',  ( 4.458734125000000326, 7.854166668032260823, 2.574251347313718519 ) ) ;
#33100=LINE ( 'NONE', #19873, #47973 ) ;
#33102=CARTESIAN_POINT ( 'NONE',  ( 2.500000000000002220, -90.66666666666665719, 4.330127018922192761 ) ) ;
#33103=CARTESIAN_POINT ( 'NONE',  ( 4.458734125000001214, -25.89583333196774007, 2.574251347313718519 ) ) ;
#33104=CARTESIAN_POINT ( 'NONE',  ( 0.000000000000000000, -120.0000000000000000, 5.000000000000000000 ) ) ;
#33105=CARTESIAN_POINT ( 'NONE',  ( -3.152548672688508926E-16, -77.81249999863440792, -5.148502694627439702 ) ) ;
#33109=CARTESIAN_POINT ( 'NONE',  ( -4.458734124999999437, 5.687500001365592972, 0.000000000000000000 ) ) ;
#33110=CARTESIAN_POINT ( 'NONE',  ( 2.229367062499998831, 26.10416666803225993, -3.861377020970580887 ) ) ;
#33111=CARTESIAN_POINT ( 'NONE',  ( 4.458734124999999437, -39.06249999863440081, -5.460374474430324690E-16 ) ) ;
#33114=CARTESIAN_POINT ( 'NONE',  ( -2.229367062499996610, -72.14583333196773651, 3.861377020970582219 ) ) ;
#33116=CARTESIAN_POINT ( 'NONE',  ( 1.060575238724906964E-15, -3.750000000000003553, 5.773502691896257311 ) ) ;
#33120=CARTESIAN_POINT ( 'NONE',  ( 4.458734125000001214, -65.89583333196772230, 2.574251347313718519 ) ) ;
#33121=CARTESIAN_POINT ( 'NONE',  ( -2.500000000000000444, -98.04166666393545881, -4.330127018922193649 ) ) ;
#33124=EDGE_CURVE ( 'NONE', #14229, #23523, #32086, .T. ) ;
#33126=CARTESIAN_POINT ( 'NONE',  ( -4.458734124999999437, -105.5624999986344221, 0.000000000000000000 ) ) ;
#33128=CARTESIAN_POINT ( 'NONE',  ( -3.535250795749689387E-16, -53.24999999999999289, -5.773502691896257311 ) ) ;
#33129=CARTESIAN_POINT ( 'NONE',  ( -4.999999999999998224, -22.91666666666666785, 2.886751345948131764 ) ) ;
#33132=CARTESIAN_POINT ( 'NONE',  ( 2.229367062500001939, -109.9791666653010651, 3.861377020970579999 ) ) ;
#33140=CARTESIAN_POINT ( 'NONE',  ( -4.999999999999998224, -4.791666663935479242, 2.886751345948131764 ) ) ;
#33151=CARTESIAN_POINT ( 'NONE',  ( 9.457646018065525792E-16, -38.31249999863441502, 5.148502694627439702 ) ) ;
#33159=CARTESIAN_POINT ( 'NONE',  ( 1.975475456537005874E-15, -83.62499999726878741, 5.000000000000000000 ) ) ;
#33161=CARTESIAN_POINT ( 'NONE',  ( -4.458734124999998549, -86.47916666530107932, 2.574251347313722516 ) ) ;
#33162=CARTESIAN_POINT ( 'NONE',  ( 5.000000000000000000, -108.4166666666666572, -2.886751345948130876 ) ) ;
#33165=DIRECTION ( 'NONE',  ( -0.000000000000000000, 1.000000000000000000, -0.000000000000000000 ) ) ;
#33168=ORIENTED_EDGE ( 'NONE', *, *, #8596, .T. ) ;
#33169=CARTESIAN_POINT ( 'NONE',  ( -2.499999999999996447, -70.70833333060214443, 4.330127018922195425 ) ) ;
#33170=CARTESIAN_POINT ( 'NONE',  ( -3.152548672688508926E-16, -11.81249999863440969, -5.148502694627439702 ) ) ;
#33174=CARTESIAN_POINT ( 'NONE',  ( -2.229367062500000163, 24.27083333469892779, -3.861377020970580443 ) ) ;
#33176=CARTESIAN_POINT ( 'NONE',  ( 4.458734124999999437, -89.81249999863440792, -5.460374474430324690E-16 ) ) ;
#33177=CARTESIAN_POINT ( 'NONE',  ( -6.972266317189433020E-16, -68.24999999999998579, -5.000000000000000000 ) ) ;
#33178=CARTESIAN_POINT ( 'NONE',  ( 2.499999999999998668, -60.20833333060214443, -4.330127018922193649 ) ) ;
#33179=CARTESIAN_POINT ( 'NONE',  ( 4.458734124999998549, -9.729166665301068662, -2.574251347313721627 ) ) ;
#33180=CARTESIAN_POINT ( 'NONE',  ( 1.975475456537005874E-15, -84.62499999726880162, 5.000000000000000000 ) ) ;
#33183=CARTESIAN_POINT ( 'NONE',  ( -2.500000000000000444, -35.04166666393547303, -4.330127018922193649 ) ) ;
#33184=CARTESIAN_POINT ( 'NONE',  ( 5.000000000000000888, -49.45833333060213732, 2.886751345948126879 ) ) ;
#33185=CARTESIAN_POINT ( 'NONE',  ( -4.458734124999999437, 19.68750000136559208, 0.000000000000000000 ) ) ;
#33188=CARTESIAN_POINT ( 'NONE',  ( 9.457646018065525792E-16, -54.06249999863440081, 5.148502694627439702 ) ) ;
#33191=CARTESIAN_POINT ( 'NONE',  ( -3.535250795749689387E-16, 7.749999999999999112, -5.773502691896257311 ) ) ;
#33194=CARTESIAN_POINT ( 'NONE',  ( -3.152548672688508926E-16, -49.56249999863440792, -5.148502694627439702 ) ) ;
#33195=CARTESIAN_POINT ( 'NONE',  ( -2.499999999999996447, -86.70833333060214443, 4.330127018922195425 ) ) ;
#33197=CARTESIAN_POINT ( 'NONE',  ( 5.000000000000000888, -14.45833333060214976, 2.886751345948126879 ) ) ;
#33198=CARTESIAN_POINT ( 'NONE',  ( 0.000000000000000000, -120.0000000000000000, 5.000000000000000000 ) ) ;
#33199=CARTESIAN_POINT ( 'NONE',  ( 2.229367062499998831, -89.89583333196773651, -3.861377020970580887 ) ) ;
#33201=CARTESIAN_POINT ( 'NONE',  ( 1.060575238724906964E-15, -37.75000000000000000, 5.773502691896257311 ) ) ;
#33202=DIRECTION ( 'NONE',  ( 0.000000000000000000, 0.000000000000000000, 1.000000000000000000 ) ) ;
#33203=ORIENTED_EDGE ( 'NONE', *, *, #53788, .F. ) ;
#33205=ORIENTED_EDGE ( 'NONE', *, *, #29558, .T. ) ;
#33206=CARTESIAN_POINT ( 'NONE',  ( 4.458734124999999437, -95.81249999863440792, -5.460374474430324690E-16 ) ) ;
#33207=CARTESIAN_POINT ( 'NONE',  ( 2.229367062499998831, 6.104166668032262599, -3.861377020970580887 ) ) ;
#33208=CARTESIAN_POINT ( 'NONE',  ( 5.000000000000000888, 10.54166666939785202, 2.886751345948126879 ) ) ;
#33212=CARTESIAN_POINT ( 'NONE',  ( 2.500000000000002220, -61.54166666393547303, 4.330127018922192761 ) ) ;
#33217=FACE_OUTER_BOUND ( 'NONE', #41371, .T. ) ;
#33220=CARTESIAN_POINT ( 'NONE',  ( 2.229367062500001939, -17.22916666530106866, 3.861377020970579999 ) ) ;
#33228=ORIENTED_EDGE ( 'NONE', *, *, #51213, .T. ) ;
#33230=VERTEX_POINT ( 'NONE', #14230 ) ;
#33231=CARTESIAN_POINT ( 'NONE',  ( 2.229367062499998831, -69.89583333196773651, -3.861377020970580887 ) ) ;
#33237=CARTESIAN_POINT ( 'NONE',  ( -2.229367062500000163, 3.270833334698929118, -3.861377020970580443 ) ) ;
#33238=ORIENTED_EDGE ( 'NONE', *, *, #45541, .T. ) ;
#33239=CARTESIAN_POINT ( 'NONE',  ( 1.339745962155612702, -45.29465819873851729, -5.000000000000000000 ) ) ;
#33240=CARTESIAN_POINT ( 'NONE',  ( -3.152548672688508926E-16, 2.437500001365594304, -5.148502694627439702 ) ) ;
#33245=ORIENTED_EDGE ( 'NONE', *, *, #42487, .T. ) ;
#33246=CARTESIAN_POINT ( 'NONE',  ( 4.458734125000000326, -77.89583333196773651, 2.574251347313718519 ) ) ;
#33248=CARTESIAN_POINT ( 'NONE',  ( 9.457646018065525792E-16, 8.937500001365597413, 5.148502694627439702 ) ) ;
#33251=CARTESIAN_POINT ( 'NONE',  ( 4.458734125000001214, -58.14583333196773651, 2.574251347313718519 ) ) ;
#33252=CARTESIAN_POINT ( 'NONE',  ( -4.999999999999999112, -17.79166666393547658, 2.886751345948131764 ) ) ;
#33253=CARTESIAN_POINT ( 'NONE',  ( 2.500000000000002220, -96.54166666393545881, 4.330127018922192761 ) ) ;
#33254=CARTESIAN_POINT ( 'NONE',  ( 1.339745962155615144, -42.58034179853029144, 4.999999999999999112 ) ) ;
#33258=CARTESIAN_POINT ( 'NONE',  ( 9.457646018065525792E-16, -40.06249999863439371, 5.148502694627439702 ) ) ;
#33260=CARTESIAN_POINT ( 'NONE',  ( -4.458734124999999437, -26.64583333196774007, -2.574251347313719407 ) ) ;
#33262=CARTESIAN_POINT ( 'NONE',  ( -5.000000000000000000, 27.91666666666666430, -2.886751345948128211 ) ) ;
#33264=ORIENTED_EDGE ( 'NONE', *, *, #18866, .T. ) ;
#33265=CARTESIAN_POINT ( 'NONE',  ( 9.457646018065525792E-16, -108.3124999986343937, 5.148502694627439702 ) ) ;
#33266=CARTESIAN_POINT ( 'NONE',  ( 4.458734124999998549, -29.72916666530107221, -2.574251347313721627 ) ) ;
#33267=CARTESIAN_POINT ( 'NONE',  ( -5.000000000000000000, -67.95833333060214443, -2.886751345948128211 ) ) ;
#33270=CARTESIAN_POINT ( 'NONE',  ( -4.458734124999997661, -27.22916666530107221, 2.574251347313722516 ) ) ;
#33271=CARTESIAN_POINT ( 'NONE',  ( 4.458734124999999437, -76.06249999863440792, -5.460374474430324690E-16 ) ) ;
#33275=DIRECTION ( 'NONE',  ( 0.000000000000000000, 0.000000000000000000, 1.000000000000000000 ) ) ;
#33276=CARTESIAN_POINT ( 'NONE',  ( -2.499999999999996447, -23.83333333333333215, 4.330127018922195425 ) ) ;
#33280=( BOUNDED_CURVE ( )  B_SPLINE_CURVE ( 2, ( #33412, #13164, #63017, #8652, #32787, #18924, #32464, #3214, #23456 ),
 .UNSPECIFIED., .F., .F. ) 
 B_SPLINE_CURVE_WITH_KNOTS ( ( 3, 2, 2, 2, 3 ),
 ( 0.1553571428571428603, 0.1559523809523809534, 0.1571428571428571397, 0.1583333333333333259, 0.1589285714285714191 ),
 .UNSPECIFIED. ) 
 CURVE ( )  GEOMETRIC_REPRESENTATION_ITEM ( )  RATIONAL_B_SPLINE_CURVE ( ( 0.9330127018922194093, 0.9330127018922194093, 1.000000000000000000, 0.8660254037844387076, 1.000000000000000000, 0.8660254037844387076, 1.000000000000000000, 0.9330127018922194093, 0.9330127018922194093 ) ) 
 REPRESENTATION_ITEM ( '' )  );
#33281=CARTESIAN_POINT ( 'NONE',  ( -5.000000000000000000, 26.12500000273118417, 0.000000000000000000 ) ) ;
#33282=CARTESIAN_POINT ( 'NONE',  ( -5.000000000000000000, -1.000000000000000888, 0.000000000000000000 ) ) ;
#33289=ORIENTED_EDGE ( 'NONE', *, *, #31884, .T. ) ;
#33293=VECTOR ( 'NONE', #6752, 1000.000000000000000 ) ;
#33295=ORIENTED_EDGE ( 'NONE', *, *, #37785, .F. ) ;
#33302=CARTESIAN_POINT ( 'NONE',  ( -6.972266317189433020E-16, -39.12499999726880162, -5.000000000000000000 ) ) ;
#33306=CARTESIAN_POINT ( 'NONE',  ( -3.152548672688508926E-16, -81.56249999863440792, -5.148502694627439702 ) ) ;
#33307=CARTESIAN_POINT ( 'NONE',  ( -2.229367062499996610, 17.85416666803225993, 3.861377020970582219 ) ) ;
#33313=CARTESIAN_POINT ( 'NONE',  ( 2.500000000000002220, -88.66666666666665719, 4.330127018922192761 ) ) ;
#33317=CARTESIAN_POINT ( 'NONE',  ( -4.458734124999999437, -58.31249999863440081, 0.000000000000000000 ) ) ;
#33318=CARTESIAN_POINT ( 'NONE',  ( 5.000000000000000000, 21.58333333333333215, -2.886751345948130876 ) ) ;
#33319=CARTESIAN_POINT ( 'NONE',  ( 9.457646018065525792E-16, 22.93750000136559919, 5.148502694627439702 ) ) ;
#33320=ADVANCED_FACE ( 'NONE', ( #53475 ), #43497, .T. ) ;
#33321=CARTESIAN_POINT ( 'NONE',  ( 1.339745962155615144, -97.70534180126145429, 4.999999999999999112 ) ) ;
#33323=CARTESIAN_POINT ( 'NONE',  ( -4.458734124999999437, -42.56249999863440081, 0.000000000000000000 ) ) ;
#33324=CARTESIAN_POINT ( 'NONE',  ( -2.499999999999996447, -5.708333330602148870, 4.330127018922195425 ) ) ;
#33325=CARTESIAN_POINT ( 'NONE',  ( -4.999999999999998224, -92.91666666666665719, 2.886751345948131764 ) ) ;
#33328=CARTESIAN_POINT ( 'NONE',  ( -4.458734124999999437, -108.3958333319677365, -2.574251347313719407 ) ) ;
#33329=CARTESIAN_POINT ( 'NONE',  ( -4.458734124999997661, -10.47916666530106866, 2.574251347313722516 ) ) ;
#33330=EDGE_LOOP ( 'NONE', ( #17426, #9163, #13482, #48409 ) ) ;
#33332=CARTESIAN_POINT ( 'NONE',  ( 9.457646018065525792E-16, -97.06249999863439371, 5.148502694627439702 ) ) ;
#33334=CARTESIAN_POINT ( 'NONE',  ( -4.458734124999999437, -94.64583333196773651, -2.574251347313719407 ) ) ;
#33335=CARTESIAN_POINT ( 'NONE',  ( -5.000000000000000000, -49.87499999726881583, 0.000000000000000000 ) ) ;
#33336=DIRECTION ( 'NONE',  ( -0.000000000000000000, 1.000000000000000000, -0.000000000000000000 ) ) ;
#33337=VECTOR ( 'NONE', #16763, 1000.000000000000000 ) ;
#33341=CARTESIAN_POINT ( 'NONE',  ( -3.152548672688508926E-16, -12.56249999863440259, -5.148502694627439702 ) ) ;
#33342=CARTESIAN_POINT ( 'NONE',  ( -4.458734124999999437, 11.43750000136559564, 0.000000000000000000 ) ) ;
#33344=CARTESIAN_POINT ( 'NONE',  ( 2.229367062499998831, -56.89583333196773651, -3.861377020970580887 ) ) ;
#33345=FACE_OUTER_BOUND ( 'NONE', #16295, .T. ) ;
#33346=CARTESIAN_POINT ( 'NONE',  ( -2.500000000000000444, -37.16666666666666430, -4.330127018922193649 ) ) ;
#33349=ORIENTED_EDGE ( 'NONE', *, *, #41385, .F. ) ;
#33352=CARTESIAN_POINT ( 'NONE',  ( 1.339745962155612702, -76.29465819873853150, -5.000000000000000000 ) ) ;
#33353=CARTESIAN_POINT ( 'NONE',  ( -4.458734124999999437, -83.39583333196772230, -2.574251347313719407 ) ) ;
#33354=CARTESIAN_POINT ( 'NONE',  ( -4.458734124999999437, 25.43750000136559208, 0.000000000000000000 ) ) ;
#33355=EDGE_CURVE ( 'NONE', #24536, #20419, #31715, .T. ) ;
#33358=CYLINDRICAL_SURFACE ( 'NONE', #21445, 5.000000000000000000 ) ;
#33360=CARTESIAN_POINT ( 'NONE',  ( -2.499999999999996447, -71.83333333333332860, 4.330127018922195425 ) ) ;
#33364=CARTESIAN_POINT ( 'NONE',  ( -6.972266317189433020E-16, -80.12499999726881583, -5.000000000000000000 ) ) ;
#33377=CARTESIAN_POINT ( 'NONE',  ( 4.458734125000001214, -58.14583333196773651, 2.574251347313718519 ) ) ;
#33387=CARTESIAN_POINT ( 'NONE',  ( 4.458734124999998549, -106.9791666653010509, -2.574251347313721627 ) ) ;
#33389=VERTEX_POINT ( 'NONE', #34470 ) ;
#33392=CARTESIAN_POINT ( 'NONE',  ( -2.229367062500000163, -37.47916666530107221, -3.861377020970580443 ) ) ;
#33393=CARTESIAN_POINT ( 'NONE',  ( -6.972266317189433020E-16, 0.8750000027311866102, -5.000000000000000000 ) ) ;
#33395=CARTESIAN_POINT ( 'NONE',  ( 2.229367062500001939, -7.979166665301073991, 3.861377020970579999 ) ) ;
#33396=( BOUNDED_CURVE ( )  B_SPLINE_CURVE ( 2, ( #32851, #24140, #13551, #52479, #28016, #47635, #52785, #29260, #33789 ),
 .UNSPECIFIED., .F., .F. ) 
 B_SPLINE_CURVE_WITH_KNOTS ( ( 3, 2, 2, 2, 3 ),
 ( 0.4625000000000000222, 0.4630952380952381153, 0.4642857142857143016, 0.4654761904761904878, 0.4660714285714285809 ),
 .UNSPECIFIED. ) 
 CURVE ( )  GEOMETRIC_REPRESENTATION_ITEM ( )  RATIONAL_B_SPLINE_CURVE ( ( 0.9330127018922194093, 0.9330127018922194093, 1.000000000000000000, 0.8660254037844387076, 1.000000000000000000, 0.8660254037844387076, 1.000000000000000000, 0.9330127018922194093, 0.9330127018922194093 ) ) 
 REPRESENTATION_ITEM ( '' )  );
#33397=CARTESIAN_POINT ( 'NONE',  ( -2.229367062499996610, -101.3958333319677365, 3.861377020970582219 ) ) ;
#33399=CARTESIAN_POINT ( 'NONE',  ( -3.152548672688508926E-16, -29.81249999863440436, -5.148502694627439702 ) ) ;
#33400=CARTESIAN_POINT ( 'NONE',  ( -2.500000000000000444, 11.83333333333333037, -4.330127018922193649 ) ) ;
#33403=CARTESIAN_POINT ( 'NONE',  ( -1.339745962155610925, -15.79465819873852261, 5.000000000000000000 ) ) ;
#33406=CARTESIAN_POINT ( 'NONE',  ( 4.458734124999999437, 5.937500001365593860, -5.460374474430324690E-16 ) ) ;
#33407=VERTEX_POINT ( 'NONE', #58625 ) ;
#33408=CARTESIAN_POINT ( 'NONE',  ( -6.972266317189433020E-16, -94.25000000000000000, -5.000000000000000000 ) ) ;
#33410=CARTESIAN_POINT ( 'NONE',  ( 2.500000000000002220, -95.66666666666664298, 4.330127018922192761 ) ) ;
#33411=CARTESIAN_POINT ( 'NONE',  ( 4.458734124999998549, -29.72916666530107221, -2.574251347313721627 ) ) ;
#33412=CARTESIAN_POINT ( 'NONE',  ( 1.975475456537005874E-15, 7.375000002731186832, 5.000000000000000000 ) ) ;
#33413=CARTESIAN_POINT ( 'NONE',  ( 9.457646018065525792E-16, -74.31249999863440792, 5.148502694627439702 ) ) ;
#33417=CARTESIAN_POINT ( 'NONE',  ( 4.458734125000000326, 4.104166668032260823, 2.574251347313718519 ) ) ;
#33418=CARTESIAN_POINT ( 'NONE',  ( -2.229367062499996610, 25.60416666803225993, 3.861377020970582219 ) ) ;
#33419=EDGE_CURVE ( 'NONE', #19133, #49359, #62901, .T. ) ;
#33420=CARTESIAN_POINT ( 'NONE',  ( -2.229367062500000163, -40.72916666530107221, -3.861377020970580443 ) ) ;
#33425=CARTESIAN_POINT ( 'NONE',  ( 4.458734125000001214, -68.89583333196773651, 2.574251347313718519 ) ) ;
#33426=CARTESIAN_POINT ( 'NONE',  ( -2.500000000000000444, -102.0416666639354588, -4.330127018922193649 ) ) ;
#33427=VECTOR ( 'NONE', #47341, 1000.000000000000000 ) ;
#33429=DIRECTION ( 'NONE',  ( -0.000000000000000000, 1.000000000000000000, -0.000000000000000000 ) ) ;
#33430=CARTESIAN_POINT ( 'NONE',  ( 4.458734124999998549, -104.9791666653010651, -2.574251347313721627 ) ) ;
#33432=CARTESIAN_POINT ( 'NONE',  ( 2.499999999999998668, -54.33333333333332860, -4.330127018922193649 ) ) ;
#33433=CARTESIAN_POINT ( 'NONE',  ( -5.000000000000000000, -66.08333333333332860, -2.886751345948128211 ) ) ;
#33435=ORIENTED_EDGE ( 'NONE', *, *, #30374, .T. ) ;
#33440=ADVANCED_FACE ( 'NONE', ( #10035 ), #59251, .T. ) ;
#33448=ORIENTED_EDGE ( 'NONE', *, *, #57812, .F. ) ;
#33452=CARTESIAN_POINT ( 'NONE',  ( -3.152548672688508926E-16, -41.81249999863440081, -5.148502694627439702 ) ) ;
#33459=CARTESIAN_POINT ( 'NONE',  ( -2.499999999999996447, -24.70833333060214443, 4.330127018922195425 ) ) ;
#33461=CARTESIAN_POINT ( 'NONE',  ( 4.458734124999998549, -85.97916666530107932, -2.574251347313721627 ) ) ;
#33463=CARTESIAN_POINT ( 'NONE',  ( 2.500000000000002220, -99.66666666666665719, 4.330127018922192761 ) ) ;
#33466=CARTESIAN_POINT ( 'NONE',  ( -2.500000000000000444, -105.1666666666666572, -4.330127018922193649 ) ) ;
#33470=EDGE_CURVE ( 'NONE', #63012, #59890, #55066, .T. ) ;
#33472=CARTESIAN_POINT ( 'NONE',  ( 2.229367062499998831, -11.89583333196774007, -3.861377020970580887 ) ) ;
#33478=EDGE_CURVE ( 'NONE', #17397, #51665, #40266, .T. ) ;
#33479=CARTESIAN_POINT ( 'NONE',  ( -2.229367062499996610, 21.60416666803226349, 3.861377020970582219 ) ) ;
#33480=VERTEX_POINT ( 'NONE', #44443 ) ;
#33481=CARTESIAN_POINT ( 'NONE',  ( -4.458734124999997661, -90.22916666530106511, 2.574251347313722516 ) ) ;
#33482=CARTESIAN_POINT ( 'NONE',  ( 2.500000000000002220, -47.66666666666666430, 4.330127018922192761 ) ) ;
#33483=CARTESIAN_POINT ( 'NONE',  ( -2.500000000000000444, -104.0416666639354730, -4.330127018922193649 ) ) ;
#33484=CARTESIAN_POINT ( 'NONE',  ( -2.229367062500000163, -11.47916666530107044, -3.861377020970580443 ) ) ;
#33485=EDGE_CURVE ( 'NONE', #49915, #25201, #27576, .T. ) ;
#33490=CARTESIAN_POINT ( 'NONE',  ( 2.499999999999998668, -34.20833333060213732, -4.330127018922193649 ) ) ;
#33492=CARTESIAN_POINT ( 'NONE',  ( -4.458734124999999437, 17.60416666803225993, -2.574251347313719407 ) ) ;
#33494=EDGE_CURVE ( 'NONE', #17397, #32122, #30286, .T. ) ;
#33497=CARTESIAN_POINT ( 'NONE',  ( -2.229367062499996610, -57.14583333196773651, 3.861377020970582219 ) ) ;
#33501=CARTESIAN_POINT ( 'NONE',  ( 2.500000000000002220, 7.333333333333333925, 4.330127018922192761 ) ) ;
#33502=EDGE_CURVE ( 'NONE', #10267, #2700, #24520, .T. ) ;
#33506=CARTESIAN_POINT ( 'NONE',  ( -3.152548672688508926E-16, -55.56249999863440081, -5.148502694627439702 ) ) ;
#33507=CARTESIAN_POINT ( 'NONE',  ( -2.500000000000000444, -84.04166666393547303, -4.330127018922193649 ) ) ;
#33509=CARTESIAN_POINT ( 'NONE',  ( -2.499999999999996447, -16.83333333333333215, 4.330127018922195425 ) ) ;
#33510=CARTESIAN_POINT ( 'NONE',  ( -2.500000000000000444, -92.16666666666665719, -4.330127018922193649 ) ) ;
#33511=CARTESIAN_POINT ( 'NONE',  ( -4.458734124999999437, -92.64583333196773651, -2.574251347313719407 ) ) ;
#33513=CARTESIAN_POINT ( 'NONE',  ( 1.060575238724906964E-15, -35.75000000000000711, 5.773502691896257311 ) ) ;
#33517=CARTESIAN_POINT ( 'NONE',  ( 2.229367062499998831, -97.64583333196773651, -3.861377020970580887 ) ) ;
#33518=CARTESIAN_POINT ( 'NONE',  ( 4.458734125000001214, 9.854166668032263487, 2.574251347313718519 ) ) ;
#33519=CARTESIAN_POINT ( 'NONE',  ( -2.499999999999996447, 13.29166666939785379, 4.330127018922195425 ) ) ;
#33524=AXIS2_PLACEMENT_3D ( 'NONE', #25015, #59760, #35306 ) ;
#33525=CARTESIAN_POINT ( 'NONE',  ( 0.000000000000000000, -114.9999999999999858, 0.000000000000000000 ) ) ;
#33529=CARTESIAN_POINT ( 'NONE',  ( 2.499999999999998668, 19.66666666666666430, -4.330127018922193649 ) ) ;
#33530=CARTESIAN_POINT ( 'NONE',  ( 1.975475456537005874E-15, 7.249999999999998224, 5.000000000000000000 ) ) ;
#33533=CARTESIAN_POINT ( 'NONE',  ( -2.229367062499996610, -18.39583333196774007, 3.861377020970582219 ) ) ;
#33541=ORIENTED_EDGE ( 'NONE', *, *, #46011, .F. ) ;
#33542=CARTESIAN_POINT ( 'NONE',  ( 1.975475456537005874E-15, -93.62499999726881583, 5.000000000000000000 ) ) ;
#33544=CARTESIAN_POINT ( 'NONE',  ( -4.458734124999998549, -69.47916666530107932, 2.574251347313722516 ) ) ;
#33546=ORIENTED_EDGE ( 'NONE', *, *, #31225, .T. ) ;
#33549=CARTESIAN_POINT ( 'NONE',  ( -4.458734124999998549, 3.520833334698929118, 2.574251347313722516 ) ) ;
#33556=ORIENTED_EDGE ( 'NONE', *, *, #24039, .T. ) ;
#33557=CARTESIAN_POINT ( 'NONE',  ( -4.458734124999997661, -76.22916666530107932, 2.574251347313722516 ) ) ;
#33559=CARTESIAN_POINT ( 'NONE',  ( 2.229367062499998831, 7.354166668032259935, -3.861377020970580887 ) ) ;
#33560=AXIS2_PLACEMENT_3D ( 'NONE', #24657, #44263, #227 ) ;
#33563=CARTESIAN_POINT ( 'NONE',  ( 9.457646018065525792E-16, -59.31249999863440081, 5.148502694627439702 ) ) ;
#33564=CARTESIAN_POINT ( 'NONE',  ( -3.535250795749689387E-16, -18.12499999726881228, -5.773502691896257311 ) ) ;
#33567=CARTESIAN_POINT ( 'NONE',  ( -2.499999999999996447, -58.83333333333333570, 4.330127018922195425 ) ) ;
#33571=CARTESIAN_POINT ( 'NONE',  ( -4.458734124999999437, -42.31249999863440081, 0.000000000000000000 ) ) ;
#33572=CARTESIAN_POINT ( 'NONE',  ( -2.229367062499996610, -29.39583333196774007, 3.861377020970582219 ) ) ;
#33573=CARTESIAN_POINT ( 'NONE',  ( -5.000000000000000000, 26.00000000000000000, 0.000000000000000000 ) ) ;
#33575=CARTESIAN_POINT ( 'NONE',  ( -4.458734124999999437, -105.5624999986344221, 0.000000000000000000 ) ) ;
#33576=CARTESIAN_POINT ( 'NONE',  ( 2.229367062499998831, -33.64583333196772941, -3.861377020970580887 ) ) ;
#33577=CARTESIAN_POINT ( 'NONE',  ( -5.000000000000000000, -68.95833333060214443, -2.886751345948128211 ) ) ;
#33582=CARTESIAN_POINT ( 'NONE',  ( 2.229367062500001939, -76.22916666530106511, 3.861377020970579999 ) ) ;
#33583=CARTESIAN_POINT ( 'NONE',  ( 1.975475456537005874E-15, -93.74999999999998579, 5.000000000000000000 ) ) ;
#33586=CARTESIAN_POINT ( 'NONE',  ( 1.339745962155608039, 22.41965820146970501, 5.000000000000003553 ) ) ;
#33587=CARTESIAN_POINT ( 'NONE',  ( 2.500000000000002220, -20.66666666666666785, 4.330127018922192761 ) ) ;
#33591=CARTESIAN_POINT ( 'NONE',  ( -2.499999999999996447, -48.83333333333332860, 4.330127018922195425 ) ) ;
#33593=CARTESIAN_POINT ( 'NONE',  ( -4.999999999999999112, 26.20833333606451632, 2.886751345948131764 ) ) ;
#33594=CARTESIAN_POINT ( 'NONE',  ( 2.499999999999998668, 4.791666669397852907, -4.330127018922193649 ) ) ;
#33600=CARTESIAN_POINT ( 'NONE',  ( -5.000000000000000000, -40.87499999726880162, 0.000000000000000000 ) ) ;
#33604=VECTOR ( 'NONE', #39023, 1000.000000000000000 ) ;
#33605=CARTESIAN_POINT ( 'NONE',  ( 5.000000000000000000, 10.70833333606451987, -2.886751345948130876 ) ) ;
#33610=ORIENTED_EDGE ( 'NONE', *, *, #23901, .F. ) ;
#33611=VECTOR ( 'NONE', #21064, 1000.000000000000000 ) ;
#33614=CARTESIAN_POINT ( 'NONE',  ( 2.500000000000002220, -4.666666666666666075, 4.330127018922192761 ) ) ;
#33617=ORIENTED_EDGE ( 'NONE', *, *, #14939, .F. ) ;
#33620=DIRECTION ( 'NONE',  ( 0.000000000000000000, 0.000000000000000000, 1.000000000000000000 ) ) ;
#33622=ORIENTED_EDGE ( 'NONE', *, *, #53167, .F. ) ;
#33624=CARTESIAN_POINT ( 'NONE',  ( -4.458734124999999437, -80.39583333196772230, -2.574251347313719407 ) ) ;
#33625=CARTESIAN_POINT ( 'NONE',  ( -4.458734124999999437, 16.68750000136559564, 0.000000000000000000 ) ) ;
#33626=ORIENTED_EDGE ( 'NONE', *, *, #39695, .T. ) ;
#33632=CARTESIAN_POINT ( 'NONE',  ( -2.229367062499996610, -60.14583333196774362, 3.861377020970582219 ) ) ;
#33633=CARTESIAN_POINT ( 'NONE',  ( 1.339745962155612702, 21.70534180126147916, -5.000000000000000000 ) ) ;
#33634=CARTESIAN_POINT ( 'NONE',  ( -2.229367062500000163, 23.52083333469892779, -3.861377020970580443 ) ) ;
#33635=CARTESIAN_POINT ( 'NONE',  ( 1.339745962155729053, -42.29465819873852439, -4.999999999999933387 ) ) ;
#33637=CARTESIAN_POINT ( 'NONE',  ( 2.229367062499998831, -45.89583333196774362, -3.861377020970580887 ) ) ;
#33638=CARTESIAN_POINT ( 'NONE',  ( 1.060575238724906964E-15, -2.624999997268815388, 5.773502691896257311 ) ) ;
#33642=CARTESIAN_POINT ( 'NONE',  ( -4.458734124999999437, -107.3958333319677649, -2.574251347313719407 ) ) ;
#33643=CARTESIAN_POINT ( 'NONE',  ( 4.458734124999998549, -11.97916666530107044, -2.574251347313721627 ) ) ;
#33646=DIRECTION ( 'NONE',  ( 0.000000000000000000, 1.000000000000000000, 0.000000000000000000 ) ) ;
#33647=CARTESIAN_POINT ( 'NONE',  ( -2.229367062499996610, -97.14583333196773651, 3.861377020970582219 ) ) ;
#33649=CARTESIAN_POINT ( 'NONE',  ( -3.152548672688508926E-16, -92.81249999863439371, -5.148502694627439702 ) ) ;
#33651=CARTESIAN_POINT ( 'NONE',  ( -2.499999999999996447, -54.70833333060213732, 4.330127018922195425 ) ) ;
#33652=CARTESIAN_POINT ( 'NONE',  ( 2.500000000000002220, -5.666666666666666963, 4.330127018922192761 ) ) ;
#33655=CARTESIAN_POINT ( 'NONE',  ( -2.229367062500000163, -15.47916666530107399, -3.861377020970580443 ) ) ;
#33656=CARTESIAN_POINT ( 'NONE',  ( 4.458734125000001214, 9.854166668032263487, 2.574251347313718519 ) ) ;
#33657=CARTESIAN_POINT ( 'NONE',  ( -4.458734124999999437, -60.56249999863440081, 0.000000000000000000 ) ) ;
#33658=CARTESIAN_POINT ( 'NONE',  ( 0.000000000000000000, -120.0000000000000000, 0.000000000000000000 ) ) ;
#33664=CARTESIAN_POINT ( 'NONE',  ( -4.999999999999998224, -24.91666666666666430, 2.886751345948131764 ) ) ;
#33665=CARTESIAN_POINT ( 'NONE',  ( 9.457646018065525792E-16, -84.06249999863439371, 5.148502694627439702 ) ) ;
#33666=CARTESIAN_POINT ( 'NONE',  ( -4.458734124999999437, 19.35416666803225993, -2.574251347313719407 ) ) ;
#33668=FACE_OUTER_BOUND ( 'NONE', #23732, .T. ) ;
#33671=CARTESIAN_POINT ( 'NONE',  ( -2.500000000000000444, -68.16666666666667140, -4.330127018922193649 ) ) ;
#33673=ORIENTED_EDGE ( 'NONE', *, *, #26905, .F. ) ;
#33674=CARTESIAN_POINT ( 'NONE',  ( 5.000000000000000000, -79.50000000000000000, -6.123233995736766282E-16 ) ) ;
#33677=CARTESIAN_POINT ( 'NONE',  ( -1.339745962155610925, -103.7946581987385173, 5.000000000000000000 ) ) ;
#33680=EDGE_CURVE ( 'NONE', #30949, #54038, #11982, .T. ) ;
#33683=VERTEX_POINT ( 'NONE', #41521 ) ;
#33689=CARTESIAN_POINT ( 'NONE',  ( 2.229367062500001939, -59.22916666530106511, 3.861377020970579999 ) ) ;
#33690=VECTOR ( 'NONE', #52566, 1000.000000000000000 ) ;
#33693=CARTESIAN_POINT ( 'NONE',  ( -1.339745962155610925, 10.33034180399266333, 5.000000000000000000 ) ) ;
#33694=ORIENTED_EDGE ( 'NONE', *, *, #13101, .F. ) ;
#33701=CARTESIAN_POINT ( 'NONE',  ( 4.458734125000001214, -105.1458333319677365, 2.574251347313718519 ) ) ;
#33703=ORIENTED_EDGE ( 'NONE', *, *, #29034, .T. ) ;
#33706=CARTESIAN_POINT ( 'NONE',  ( -2.229367062499996610, -36.14583333196773651, 3.861377020970582219 ) ) ;
#33707=CARTESIAN_POINT ( 'NONE',  ( 5.000000000000000000, -83.41666666666667140, -2.886751345948130876 ) ) ;
#33708=CARTESIAN_POINT ( 'NONE',  ( -4.458734124999999437, -15.31249999863440436, 0.000000000000000000 ) ) ;
#33710=CARTESIAN_POINT ( 'NONE',  ( 4.458734125000000326, -102.1458333319677365, 2.574251347313718519 ) ) ;
#33712=CARTESIAN_POINT ( 'NONE',  ( -4.458734124999998549, -27.47916666530106866, 2.574251347313722516 ) ) ;
#33713=CARTESIAN_POINT ( 'NONE',  ( 1.975475456537005874E-15, 12.24999999999999822, 5.000000000000000000 ) ) ;
#33716=CARTESIAN_POINT ( 'NONE',  ( -4.999999999999998224, -15.91666666666666963, 2.886751345948131764 ) ) ;
#33719=CARTESIAN_POINT ( 'NONE',  ( -4.458734124999999437, 6.437500001365593860, 0.000000000000000000 ) ) ;
#33722=CARTESIAN_POINT ( 'NONE',  ( -6.972266317189433020E-16, 0.7499999999999996669, -5.000000000000000000 ) ) ;
#33723=CARTESIAN_POINT ( 'NONE',  ( 2.499999999999998668, -93.33333333333332860, -4.330127018922193649 ) ) ;
#33724=CARTESIAN_POINT ( 'NONE',  ( 4.458734124999999437, -29.81249999863440436, -5.460374474430324690E-16 ) ) ;
#33726=CARTESIAN_POINT ( 'NONE',  ( 2.229367062499998831, -77.89583333196773651, -3.861377020970580887 ) ) ;
#33730=CARTESIAN_POINT ( 'NONE',  ( -3.152548672688508926E-16, 5.437500001365592084, -5.148502694627439702 ) ) ;
#33731=CARTESIAN_POINT ( 'NONE',  ( 2.229367062499998831, 28.10416666803225993, -3.861377020970580887 ) ) ;
#33732=CARTESIAN_POINT ( 'NONE',  ( 4.458734124999998549, -42.97916666530107932, -2.574251347313721627 ) ) ;
#33736=AXIS2_PLACEMENT_3D ( 'NONE', #43659, #22257, #8098 ) ;
#33738=CARTESIAN_POINT ( 'NONE',  ( 2.229367062500001939, -68.97916666530107932, 3.861377020970579999 ) ) ;
#33739=CARTESIAN_POINT ( 'NONE',  ( 5.000000000000000000, -107.3749999972687874, -6.123233995736766282E-16 ) ) ;
#33743=CARTESIAN_POINT ( 'NONE',  ( -4.458734124999999437, -104.6458333319677365, -2.574251347313719407 ) ) ;
#33745=CARTESIAN_POINT ( 'NONE',  ( -2.500000000000000444, -52.16666666666666430, -4.330127018922193649 ) ) ;
#33749=CYLINDRICAL_SURFACE ( 'NONE', #21221, 5.000000000000000000 ) ;
#33750=CARTESIAN_POINT ( 'NONE',  ( 1.339745962155615144, -27.58034179853028789, 4.999999999999999112 ) ) ;
#33753=ADVANCED_FACE ( 'NONE', ( #55389 ), #32196, .T. ) ;
#33759=CARTESIAN_POINT ( 'NONE',  ( -6.972266317189433020E-16, -45.12499999726880162, -5.000000000000000000 ) ) ;
#33765=CARTESIAN_POINT ( 'NONE',  ( 2.229367062499998831, -42.89583333196773651, -3.861377020970580887 ) ) ;
#33773=( BOUNDED_CURVE ( )  B_SPLINE_CURVE ( 2, ( #48888, #57623, #14161, #63076, #63387, #58554, #28642, #14474, #4833 ),
 .UNSPECIFIED., .F., .F. ) 
 B_SPLINE_CURVE_WITH_KNOTS ( ( 3, 2, 2, 2, 3 ),
 ( 0.9589285714285714635, 0.9595238095238095566, 0.9607142857142857428, 0.9619047619047619291, 0.9625000000000000222 ),
 .UNSPECIFIED. ) 
 CURVE ( )  GEOMETRIC_REPRESENTATION_ITEM ( )  RATIONAL_B_SPLINE_CURVE ( ( 0.9330127018922194093, 0.9330127018922194093, 1.000000000000000000, 0.8660254037844387076, 1.000000000000000000, 0.8660254037844387076, 1.000000000000000000, 0.9330127018922194093, 0.9330127018922194093 ) ) 
 REPRESENTATION_ITEM ( '' )  );
#33776=EDGE_CURVE ( 'NONE', #25237, #47640, #40721, .T. ) ;
#33777=CARTESIAN_POINT ( 'NONE',  ( -2.229367062499996610, -88.39583333196773651, 3.861377020970582219 ) ) ;
#33778=CARTESIAN_POINT ( 'NONE',  ( 2.500000000000002220, -34.54166666393547303, 4.330127018922192761 ) ) ;
#33780=CARTESIAN_POINT ( 'NONE',  ( -5.000000000000000000, -47.08333333333333570, -2.886751345948128211 ) ) ;
#33781=PRODUCT_DEFINITION_SHAPE ( 'NONE', 'NONE',  #50832 ) ;
#33784=FACE_OUTER_BOUND ( 'NONE', #26026, .T. ) ;
#33788=CARTESIAN_POINT ( 'NONE',  ( 2.229367062500001939, -10.22916666530106866, 3.861377020970579999 ) ) ;
#33789=CARTESIAN_POINT ( 'NONE',  ( -6.972266317189433020E-16, -35.25000000000000000, -5.000000000000000000 ) ) ;
#33793=CARTESIAN_POINT ( 'NONE',  ( -4.458734124999997661, 23.52083333469892779, 2.574251347313722516 ) ) ;
#33794=ORIENTED_EDGE ( 'NONE', *, *, #24697, .F. ) ;
#33795=CARTESIAN_POINT ( 'NONE',  ( -2.229367062500000163, -91.47916666530106511, -3.861377020970580443 ) ) ;
#33797=CARTESIAN_POINT ( 'NONE',  ( 9.457646018065525792E-16, -14.06249999863440259, 5.148502694627439702 ) ) ;
#33801=EDGE_CURVE ( 'NONE', #25201, #26022, #55960, .T. ) ;
#33802=CARTESIAN_POINT ( 'NONE',  ( 2.500000000000002220, -43.54166666393548013, 4.330127018922192761 ) ) ;
#33804=CARTESIAN_POINT ( 'NONE',  ( 4.458734125000000326, 17.10416666803225993, 2.574251347313718519 ) ) ;
#33805=CARTESIAN_POINT ( 'NONE',  ( -4.999999999999998224, 12.20833333606451632, 2.886751345948131764 ) ) ;
#33808=CARTESIAN_POINT ( 'NONE',  ( -2.229367062499996610, -61.14583333196774362, 3.861377020970582219 ) ) ;
#33810=DIRECTION ( 'NONE',  ( 0.000000000000000000, 0.000000000000000000, 1.000000000000000000 ) ) ;
#33811=CARTESIAN_POINT ( 'NONE',  ( -5.000000000000000000, 9.916666666666667851, -2.886751345948128211 ) ) ;
#33813=CARTESIAN_POINT ( 'NONE',  ( -2.229367062500000163, -53.47916666530107221, -3.861377020970580443 ) ) ;
#33814=CARTESIAN_POINT ( 'NONE',  ( -5.000000000000000000, -86.87499999726880162, 0.000000000000000000 ) ) ;
#33816=CARTESIAN_POINT ( 'NONE',  ( 0.000000000000000000, -120.0000000000000000, 0.000000000000000000 ) ) ;
#33817=CYLINDRICAL_SURFACE ( 'NONE', #40858, 5.000000000000000000 ) ;
#33818=CARTESIAN_POINT ( 'NONE',  ( -4.458734124999999437, -88.64583333196773651, -2.574251347313719407 ) ) ;
#33821=CARTESIAN_POINT ( 'NONE',  ( -3.535250795749689387E-16, -37.25000000000001421, -5.773502691896257311 ) ) ;
#33823=CARTESIAN_POINT ( 'NONE',  ( -6.972266317189433020E-16, -22.24999999999999645, -5.000000000000000000 ) ) ;
#33824=ORIENTED_EDGE ( 'NONE', *, *, #3224, .T. ) ;
#33825=CARTESIAN_POINT ( 'NONE',  ( 4.458734125000001214, -99.89583333196772230, 2.574251347313718519 ) ) ;
#33826=CARTESIAN_POINT ( 'NONE',  ( -3.152548672688508926E-16, 10.18750000136559564, -5.148502694627439702 ) ) ;
#33830=AXIS2_PLACEMENT_3D ( 'NONE', #14903, #54477, #15228 ) ;
#33832=DIRECTION ( 'NONE',  ( 0.000000000000000000, 0.000000000000000000, 1.000000000000000000 ) ) ;
#33833=EDGE_CURVE ( 'NONE', #58981, #50402, #5788, .T. ) ;
#33834=EDGE_CURVE ( 'NONE', #49482, #44442, #23461, .T. ) ;
#33838=CARTESIAN_POINT ( 'NONE',  ( 5.000000000000000888, -19.58333333333333215, 2.886751345948126879 ) ) ;
#33840=CARTESIAN_POINT ( 'NONE',  ( -2.500000000000000444, 23.95833333606451987, -4.330127018922193649 ) ) ;
#33841=CARTESIAN_POINT ( 'NONE',  ( -2.229367062500000163, -24.72916666530106866, -3.861377020970580443 ) ) ;
#33847=EDGE_CURVE ( 'NONE', #29077, #2195, #18566, .T. ) ;
#33854=CARTESIAN_POINT ( 'NONE',  ( 4.458734124999998549, -70.97916666530107932, -2.574251347313721627 ) ) ;
#33860=CARTESIAN_POINT ( 'NONE',  ( 9.457646018065525792E-16, 1.687500001365593194, 5.148502694627439702 ) ) ;
#33861=ORIENTED_EDGE ( 'NONE', *, *, #51246, .T. ) ;
#33862=CARTESIAN_POINT ( 'NONE',  ( -1.339745962155613812, -20.20534180126147916, -5.000000000000000000 ) ) ;
#33868=( BOUNDED_CURVE ( )  B_SPLINE_CURVE ( 2, ( #45747, #11637, #31258, #50892, #57934, #9339, #52159, #62450, #28953 ),
 .UNSPECIFIED., .F., .F. ) 
 B_SPLINE_CURVE_WITH_KNOTS ( ( 3, 2, 2, 2, 3 ),
 ( 0.2910714285714285920, 0.2916666666666666852, 0.2928571428571428714, 0.2940476190476190577, 0.2946428571428571508 ),
 .UNSPECIFIED. ) 
 CURVE ( )  GEOMETRIC_REPRESENTATION_ITEM ( )  RATIONAL_B_SPLINE_CURVE ( ( 0.9330127018922194093, 0.9330127018922194093, 1.000000000000000000, 0.8660254037844387076, 1.000000000000000000, 0.8660254037844387076, 1.000000000000000000, 0.9330127018922194093, 0.9330127018922194093 ) ) 
 REPRESENTATION_ITEM ( '' )  );
#33870=CARTESIAN_POINT ( 'NONE',  ( -4.458734124999997661, -74.22916666530106511, 2.574251347313722516 ) ) ;
#33872=CARTESIAN_POINT ( 'NONE',  ( -2.229367062500000163, 4.520833334698926897, -3.861377020970580443 ) ) ;
#33874=CARTESIAN_POINT ( 'NONE',  ( 2.229367062499998831, -64.89583333196773651, -3.861377020970580887 ) ) ;
#33875=CARTESIAN_POINT ( 'NONE',  ( -2.500000000000000444, -25.04166666393547658, -4.330127018922193649 ) ) ;
#33877=CARTESIAN_POINT ( 'NONE',  ( 1.975475456537005874E-15, -44.62499999726880162, 5.000000000000000000 ) ) ;
#33878=CARTESIAN_POINT ( 'NONE',  ( -1.339745962155613812, -59.20534180126148271, -5.000000000000000000 ) ) ;
#33880=CARTESIAN_POINT ( 'NONE',  ( 4.458734125000001214, -39.89583333196772941, 2.574251347313718519 ) ) ;
#33881=CARTESIAN_POINT ( 'NONE',  ( -4.458734124999997661, -25.47916666530106866, 2.574251347313722516 ) ) ;
#33883=CARTESIAN_POINT ( 'NONE',  ( 0.000000000000000000, -120.0000000000000000, 0.000000000000000000 ) ) ;
#33884=CARTESIAN_POINT ( 'NONE',  ( 2.500000000000002220, 23.33333333333333215, 4.330127018922192761 ) ) ;
#33887=CARTESIAN_POINT ( 'NONE',  ( 4.458734124999999437, -37.81249999863440792, -5.460374474430324690E-16 ) ) ;
#33888=CARTESIAN_POINT ( 'NONE',  ( -2.499999999999996447, -66.70833333060214443, 4.330127018922195425 ) ) ;
#33891=CARTESIAN_POINT ( 'NONE',  ( 2.229367062499998831, -75.89583333196773651, -3.861377020970580887 ) ) ;
#33894=CYLINDRICAL_SURFACE ( 'NONE', #48171, 5.000000000000000000 ) ;
#33895=CARTESIAN_POINT ( 'NONE',  ( -1.336351044127974539E-14, 22.37500000273118417, 5.000000000000000000 ) ) ;
#33896=CARTESIAN_POINT ( 'NONE',  ( 1.060575238724906964E-15, -20.74999999999999645, 5.773502691896257311 ) ) ;
#33900=CARTESIAN_POINT ( 'NONE',  ( 1.975475456537005874E-15, 8.249999999999998224, 5.000000000000000000 ) ) ;
#33902=CARTESIAN_POINT ( 'NONE',  ( -6.972266317189433020E-16, -27.12499999726881228, -5.000000000000000000 ) ) ;
#33905=LINE ( 'NONE', #48384, #50970 ) ;
#33907=CARTESIAN_POINT ( 'NONE',  ( -4.999999999999998224, 4.083333333333334814, 2.886751345948131764 ) ) ;
#33908=EDGE_CURVE ( 'NONE', #51679, #35740, #63061, .T. ) ;
#33912=CARTESIAN_POINT ( 'NONE',  ( -2.229367062499996610, -20.14583333196774007, 3.861377020970582219 ) ) ;
#33913=CARTESIAN_POINT ( 'NONE',  ( 2.500000000000002220, 0.3333333333333348136, 4.330127018922192761 ) ) ;
#33916=VECTOR ( 'NONE', #35489, 1000.000000000000000 ) ;
#33921=CARTESIAN_POINT ( 'NONE',  ( 1.975475456537005874E-15, -4.749999999999999112, 5.000000000000000000 ) ) ;
#33922=CARTESIAN_POINT ( 'NONE',  ( 1.339745962155670655, -9.169658196007338447, -4.999999999999966249 ) ) ;
#33928=CARTESIAN_POINT ( 'NONE',  ( 0.000000000000000000, -120.0000000000000000, 0.000000000000000000 ) ) ;
#33932=VERTEX_POINT ( 'NONE', #8087 ) ;
#33934=CARTESIAN_POINT ( 'NONE',  ( 1.339745962155612702, -103.1696581960073331, -5.000000000000000000 ) ) ;
#33935=CARTESIAN_POINT ( 'NONE',  ( 2.229367062500001939, 19.02083333469892779, 3.861377020970579999 ) ) ;
#33936=LINE ( 'NONE', #28164, #3007 ) ;
#33937=EDGE_LOOP ( 'NONE', ( #14279, #34001, #28557, #8268 ) ) ;
#33941=CARTESIAN_POINT ( 'NONE',  ( -6.972266317189433020E-16, -100.2499999999999858, -5.000000000000000000 ) ) ;
#33943=CARTESIAN_POINT ( 'NONE',  ( -4.458734124999999437, -61.31249999863440081, 0.000000000000000000 ) ) ;
#33945=CARTESIAN_POINT ( 'NONE',  ( 4.458734124999999437, 18.18750000136559564, -5.460374474430324690E-16 ) ) ;
#33946=( BOUNDED_CURVE ( )  B_SPLINE_CURVE ( 2, ( #12354, #9645, #63067, #38592, #53712, #33780, #37125, #63379, #48567 ),
 .UNSPECIFIED., .F., .F. ) 
 B_SPLINE_CURVE_WITH_KNOTS ( ( 3, 2, 2, 2, 3 ),
 ( 0.5482142857142857650, 0.5488095238095238582, 0.5500000000000000444, 0.5511904761904762307, 0.5517857142857143238 ),
 .UNSPECIFIED. ) 
 CURVE ( )  GEOMETRIC_REPRESENTATION_ITEM ( )  RATIONAL_B_SPLINE_CURVE ( ( 0.9330127018922194093, 0.9330127018922194093, 1.000000000000000000, 0.8660254037844387076, 1.000000000000000000, 0.8660254037844387076, 1.000000000000000000, 0.9330127018922194093, 0.9330127018922194093 ) ) 
 REPRESENTATION_ITEM ( '' )  );
#33947=CARTESIAN_POINT ( 'NONE',  ( 2.500000000000002220, -102.5416666639354588, 4.330127018922192761 ) ) ;
#33949=CARTESIAN_POINT ( 'NONE',  ( -4.458734124999999437, -50.64583333196773651, -2.574251347313719407 ) ) ;
#33950=CARTESIAN_POINT ( 'NONE',  ( -5.000000000000000000, -1.874999997268814944, 0.000000000000000000 ) ) ;
#33954=CARTESIAN_POINT ( 'NONE',  ( 9.457646018065525792E-16, -110.0624999986343937, 5.148502694627439702 ) ) ;
#33955=CARTESIAN_POINT ( 'NONE',  ( -4.458734124999999437, -10.56249999863440792, 0.000000000000000000 ) ) ;
#33956=EDGE_LOOP ( 'NONE', ( #43963, #30774, #37190, #11529 ) ) ;
#33958=CARTESIAN_POINT ( 'NONE',  ( 2.229367062500001939, -95.97916666530105090, 3.861377020970579999 ) ) ;
#33960=CARTESIAN_POINT ( 'NONE',  ( 4.458734124999998549, -90.97916666530106511, -2.574251347313721627 ) ) ;
#33962=CARTESIAN_POINT ( 'NONE',  ( -2.500000000000000444, -53.04166666393548013, -4.330127018922193649 ) ) ;
#33965=( BOUNDED_CURVE ( )  B_SPLINE_CURVE ( 2, ( #55805, #45827, #11721, #36492, #50653, #8726, #31338, #47643, #57631 ),
 .UNSPECIFIED., .F., .F. ) 
 B_SPLINE_CURVE_WITH_KNOTS ( ( 3, 2, 2, 2, 3 ),
 ( 0.1517857142857143016, 0.1523809523809523947, 0.1535714285714285809, 0.1547619047619047672, 0.1553571428571428603 ),
 .UNSPECIFIED. ) 
 CURVE ( )  GEOMETRIC_REPRESENTATION_ITEM ( )  RATIONAL_B_SPLINE_CURVE ( ( 0.9330127018922194093, 0.9330127018922209636, 1.000000000000000000, 0.8660254037844387076, 1.000000000000000000, 0.8660254037844387076, 1.000000000000000000, 0.9330127018922194093, 0.9330127018922194093 ) ) 
 REPRESENTATION_ITEM ( '' )  );
#33967=CARTESIAN_POINT ( 'NONE',  ( -3.152548672688508926E-16, -16.56249999863440436, -5.148502694627439702 ) ) ;
#33968=CARTESIAN_POINT ( 'NONE',  ( 2.229367062500001939, 13.77083333469892779, 3.861377020970579999 ) ) ;
#33969=CARTESIAN_POINT ( 'NONE',  ( -4.458734124999999437, -56.64583333196773651, -2.574251347313719407 ) ) ;
#33972=DIRECTION ( 'NONE',  ( 0.000000000000000000, 0.000000000000000000, 1.000000000000000000 ) ) ;
#33974=EDGE_LOOP ( 'NONE', ( #39938, #47942, #31004, #57829 ) ) ;
#33978=CARTESIAN_POINT ( 'NONE',  ( -6.972266317189433020E-16, -25.24999999999999645, -5.000000000000000000 ) ) ;
#33979=CARTESIAN_POINT ( 'NONE',  ( 4.458734125000001214, -85.89583333196773651, 2.574251347313718519 ) ) ;
#33980=CARTESIAN_POINT ( 'NONE',  ( 2.229367062499998831, 18.10416666803225993, -3.861377020970580887 ) ) ;
#33983=CARTESIAN_POINT ( 'NONE',  ( 6.123233995736766282E-16, -120.0000000000000000, -5.000000000000000000 ) ) ;
#33985=CARTESIAN_POINT ( 'NONE',  ( -6.972266317189433020E-16, 20.87500000273118062, -5.000000000000000000 ) ) ;
#33987=CARTESIAN_POINT ( 'NONE',  ( 5.000000000000000888, -72.58333333333334281, 2.886751345948126879 ) ) ;
#33989=VERTEX_POINT ( 'NONE', #54986 ) ;
#33990=CARTESIAN_POINT ( 'NONE',  ( 1.975475456537005874E-15, -102.7499999999999858, 5.000000000000000000 ) ) ;
#33991=ORIENTED_EDGE ( 'NONE', *, *, #43570, .F. ) ;
#33997=ORIENTED_EDGE ( 'NONE', *, *, #5436, .T. ) ;
#34001=ORIENTED_EDGE ( 'NONE', *, *, #41324, .T. ) ;
#34003=CARTESIAN_POINT ( 'NONE',  ( -6.972266317189433020E-16, -83.12499999726878741, -5.000000000000000000 ) ) ;
#34004=CARTESIAN_POINT ( 'NONE',  ( -4.458734124999999437, -55.56249999863440081, 0.000000000000000000 ) ) ;
#34006=DIRECTION ( 'NONE',  ( 0.000000000000000000, 0.000000000000000000, 1.000000000000000000 ) ) ;
#34012=CARTESIAN_POINT ( 'NONE',  ( 9.457646018065525792E-16, -107.3124999986343937, 5.148502694627439702 ) ) ;
#34017=CARTESIAN_POINT ( 'NONE',  ( -3.152548672688508926E-16, -38.56249999863440081, -5.148502694627439702 ) ) ;
#34018=( BOUNDED_CURVE ( )  B_SPLINE_CURVE ( 2, ( #22144, #57514, #56562, #12165, #13430, #7672, #31784, #47220, #12797 ),
 .UNSPECIFIED., .F., .F. ) 
 B_SPLINE_CURVE_WITH_KNOTS ( ( 3, 2, 2, 2, 3 ),
 ( 0.6482142857142857428, 0.6488095238095238360, 0.6500000000000000222, 0.6511904761904762085, 0.6517857142857143016 ),
 .UNSPECIFIED. ) 
 CURVE ( )  GEOMETRIC_REPRESENTATION_ITEM ( )  RATIONAL_B_SPLINE_CURVE ( ( 0.9330127018922194093, 0.9330127018922194093, 1.000000000000000000, 0.8660254037844387076, 1.000000000000000000, 0.8660254037844387076, 1.000000000000000000, 0.9330127018922194093, 0.9330127018922194093 ) ) 
 REPRESENTATION_ITEM ( '' )  );
#34020=CARTESIAN_POINT ( 'NONE',  ( -5.000000000000000000, -2.000000000000001776, 0.000000000000000000 ) ) ;
#34021=CARTESIAN_POINT ( 'NONE',  ( -4.458734124999999437, -12.31249999863440259, 0.000000000000000000 ) ) ;
#34022=CARTESIAN_POINT ( 'NONE',  ( -4.458734124999999437, -98.56249999863440792, 0.000000000000000000 ) ) ;
#34023=VERTEX_POINT ( 'NONE', #14462 ) ;
#34025=CARTESIAN_POINT ( 'NONE',  ( -4.458734124999999437, -29.64583333196773651, -2.574251347313719407 ) ) ;
#34029=CARTESIAN_POINT ( 'NONE',  ( -5.000000000000000000, -91.08333333333334281, -2.886751345948128211 ) ) ;
#34032=CARTESIAN_POINT ( 'NONE',  ( -4.458734124999997661, 2.520833334698928230, 2.574251347313722516 ) ) ;
#34033=EDGE_LOOP ( 'NONE', ( #56997, #3254, #57483, #648 ) ) ;
#34034=LINE ( 'NONE', #24707, #60353 ) ;
#34035=CARTESIAN_POINT ( 'NONE',  ( 1.975475456537005874E-15, 2.249999999999999556, 5.000000000000000000 ) ) ;
#34036=CARTESIAN_POINT ( 'NONE',  ( 5.000000000000000000, -97.41666666666665719, -2.886751345948129988 ) ) ;
#34037=CARTESIAN_POINT ( 'NONE',  ( 2.229367062499998831, -28.64583333196774007, -3.861377020970580887 ) ) ;
#34038=CARTESIAN_POINT ( 'NONE',  ( 5.000000000000000000, -9.500000000000001776, -6.123233995736766282E-16 ) ) ;
#34039=CARTESIAN_POINT ( 'NONE',  ( 4.458734125000001214, -77.14583333196775072, 2.574251347313718519 ) ) ;
#34043=CARTESIAN_POINT ( 'NONE',  ( -2.229367062499996610, -4.145833331967739177, 3.861377020970582219 ) ) ;
#34044=CARTESIAN_POINT ( 'NONE',  ( 2.229367062499998831, 25.10416666803225993, -3.861377020970580887 ) ) ;
#34045=CARTESIAN_POINT ( 'NONE',  ( -4.458734124999997661, -45.47916666530106511, 2.574251347313722516 ) ) ;
#34050=VECTOR ( 'NONE', #58795, 1000.000000000000000 ) ;
#34051=CARTESIAN_POINT ( 'NONE',  ( -4.458734124999998549, -67.22916666530106511, 2.574251347313722516 ) ) ;
#34052=CARTESIAN_POINT ( 'NONE',  ( -2.500000000000000444, -106.0416666639354730, -4.330127018922193649 ) ) ;
#34054=DIRECTION ( 'NONE',  ( 0.000000000000000000, 0.000000000000000000, 1.000000000000000000 ) ) ;
#34055=FACE_OUTER_BOUND ( 'NONE', #59058, .T. ) ;
#34057=CARTESIAN_POINT ( 'NONE',  ( 5.000000000000000888, -52.58333333333332860, 2.886751345948126879 ) ) ;
#34058=FACE_OUTER_BOUND ( 'NONE', #28161, .T. ) ;
#34060=ORIENTED_EDGE ( 'NONE', *, *, #28398, .F. ) ;
#34061=CARTESIAN_POINT ( 'NONE',  ( -2.500000000000000444, -27.16666666666666430, -4.330127018922193649 ) ) ;
#34069=VERTEX_POINT ( 'NONE', #44683 ) ;
#34070=CARTESIAN_POINT ( 'NONE',  ( 1.975475456537005874E-15, -23.75000000000000000, 5.000000000000000000 ) ) ;
#34073=ORIENTED_EDGE ( 'NONE', *, *, #42411, .T. ) ;
#34077=CARTESIAN_POINT ( 'NONE',  ( -4.458734124999998549, -43.47916666530106511, 2.574251347313722516 ) ) ;
#34084=CARTESIAN_POINT ( 'NONE',  ( 2.499999999999998668, -89.33333333333332860, -4.330127018922193649 ) ) ;
#34086=CARTESIAN_POINT ( 'NONE',  ( 4.458734125000001214, -89.14583333196775072, 2.574251347313718519 ) ) ;
#34091=CARTESIAN_POINT ( 'NONE',  ( 6.123233995736766282E-16, -120.0000000000000000, -5.000000000000000000 ) ) ;
#34092=ORIENTED_EDGE ( 'NONE', *, *, #22111, .T. ) ;
#34094=CARTESIAN_POINT ( 'NONE',  ( -2.229367062500000163, -13.72916666530107221, -3.861377020970580443 ) ) ;
#34097=CARTESIAN_POINT ( 'NONE',  ( 5.000000000000000000, -55.37499999726880162, -6.123233995736766282E-16 ) ) ;
#34099=CARTESIAN_POINT ( 'NONE',  ( -4.458734124999999437, 18.35416666803225993, -2.574251347313719407 ) ) ;
#34101=CARTESIAN_POINT ( 'NONE',  ( 9.457646018065525792E-16, -90.06249999863440792, 5.148502694627439702 ) ) ;
#34104=CARTESIAN_POINT ( 'NONE',  ( -2.229367062500000163, -15.47916666530107399, -3.861377020970580443 ) ) ;
#34105=EDGE_CURVE ( 'NONE', #3623, #22435, #47317, .T. ) ;
#34106=FACE_OUTER_BOUND ( 'NONE', #63468, .T. ) ;
#34107=CARTESIAN_POINT ( 'NONE',  ( -2.500000000000000444, -73.16666666666665719, -4.330127018922193649 ) ) ;
#34109=CARTESIAN_POINT ( 'NONE',  ( 1.060575238724906964E-15, -42.62499999726880162, 5.773502691896257311 ) ) ;
#34111=CARTESIAN_POINT ( 'NONE',  ( 2.229367062499998831, 16.35416666803225993, -3.861377020970580887 ) ) ;
#34114=ORIENTED_EDGE ( 'NONE', *, *, #35116, .T. ) ;
#34116=CARTESIAN_POINT ( 'NONE',  ( -4.458734124999999437, -63.39583333196772941, -2.574251347313719407 ) ) ;
#34118=CARTESIAN_POINT ( 'NONE',  ( -2.499999999999996447, 8.166666666666666075, 4.330127018922195425 ) ) ;
#34120=CARTESIAN_POINT ( 'NONE',  ( 0.000000000000000000, -120.0000000000000000, 0.000000000000000000 ) ) ;
#34121=CARTESIAN_POINT ( 'NONE',  ( 4.458734125000001214, -54.89583333196773651, 2.574251347313718519 ) ) ;
#34122=CARTESIAN_POINT ( 'NONE',  ( -3.535250795749689387E-16, -87.12499999726880162, -5.773502691896257311 ) ) ;
#34125=CARTESIAN_POINT ( 'NONE',  ( 5.000000000000000888, 25.54166666939784847, 2.886751345948126879 ) ) ;
#34129=CARTESIAN_POINT ( 'NONE',  ( -5.000000000000000000, -39.99999999999999289, 0.000000000000000000 ) ) ;
#34132=VERTEX_POINT ( 'NONE', #15437 ) ;
#34133=CARTESIAN_POINT ( 'NONE',  ( 9.457646018065525792E-16, -101.0624999986344079, 5.148502694627439702 ) ) ;
#34134=CARTESIAN_POINT ( 'NONE',  ( -4.458734124999998549, 2.520833334698928674, 2.574251347313722516 ) ) ;
#34147=CARTESIAN_POINT ( 'NONE',  ( 1.339745962155615144, 6.419658201469706782, 4.999999999999999112 ) ) ;
#34148=CARTESIAN_POINT ( 'NONE',  ( 4.458734124999999437, -26.06249999863440792, -5.460374474430324690E-16 ) ) ;
#34160=CARTESIAN_POINT ( 'NONE',  ( -2.229367062499996610, -75.39583333196773651, 3.861377020970582219 ) ) ;
#34161=CARTESIAN_POINT ( 'NONE',  ( -2.499999999999996447, 29.16666666666666785, 4.330127018922195425 ) ) ;
#34162=ORIENTED_EDGE ( 'NONE', *, *, #22058, .F. ) ;
#34166=CARTESIAN_POINT ( 'NONE',  ( -3.152548672688508926E-16, 2.187500001365593416, -5.148502694627439702 ) ) ;
#34169=CARTESIAN_POINT ( 'NONE',  ( -6.972266317189433020E-16, -69.12499999726880162, -5.000000000000000000 ) ) ;
#34175=CARTESIAN_POINT ( 'NONE',  ( -2.229367062500000163, -73.47916666530106511, -3.861377020970580443 ) ) ;
#34177=CARTESIAN_POINT ( 'NONE',  ( -4.458734124999999437, 2.687500001365593860, 0.000000000000000000 ) ) ;
#34178=EDGE_CURVE ( 'NONE', #4714, #6601, #54020, .T. ) ;
#34181=ADVANCED_FACE ( 'NONE', ( #35055 ), #49831, .T. ) ;
#34182=CARTESIAN_POINT ( 'NONE',  ( -4.458734124999998549, -65.47916666530107932, 2.574251347313722516 ) ) ;
#34183=CARTESIAN_POINT ( 'NONE',  ( 1.060575238724906964E-15, -26.62499999726881228, 5.773502691896257311 ) ) ;
#34185=CARTESIAN_POINT ( 'NONE',  ( 2.499999999999998668, -44.20833333060214443, -4.330127018922193649 ) ) ;
#34186=CARTESIAN_POINT ( 'NONE',  ( 1.975475456537005874E-15, -72.62499999726878741, 5.000000000000000000 ) ) ;
#34188=CARTESIAN_POINT ( 'NONE',  ( -4.458734124999998549, -47.22916666530106511, 2.574251347313722516 ) ) ;
#34189=CARTESIAN_POINT ( 'NONE',  ( -4.458734124999997661, -28.47916666530107221, 2.574251347313722516 ) ) ;
#34191=DIRECTION ( 'NONE',  ( 0.000000000000000000, 0.000000000000000000, 1.000000000000000000 ) ) ;
#34192=CARTESIAN_POINT ( 'NONE',  ( 5.000000000000000000, 26.50000000000000000, -6.123233995736766282E-16 ) ) ;
#34195=CARTESIAN_POINT ( 'NONE',  ( -4.458734124999999437, -39.39583333196773651, -2.574251347313719407 ) ) ;
#34196=CARTESIAN_POINT ( 'NONE',  ( 5.000000000000000000, -74.37499999726880162, -6.123233995736766282E-16 ) ) ;
#34199=EDGE_CURVE ( 'NONE', #7022, #26835, #10293, .T. ) ;
#34200=CARTESIAN_POINT ( 'NONE',  ( -4.458734124999999437, -76.64583333196775072, -2.574251347313719407 ) ) ;
#34203=LINE ( 'NONE', #24243, #34818 ) ;
#34204=CARTESIAN_POINT ( 'NONE',  ( 5.000000000000000000, -21.41666666666666430, -2.886751345948129988 ) ) ;
#34206=ORIENTED_EDGE ( 'NONE', *, *, #12848, .T. ) ;
#34209=CARTESIAN_POINT ( 'NONE',  ( -4.999999999999999112, 27.20833333606451987, 2.886751345948131764 ) ) ;
#34214=CARTESIAN_POINT ( 'NONE',  ( -6.972266317189433020E-16, 3.749999999999999556, -5.000000000000000000 ) ) ;
#34215=CARTESIAN_POINT ( 'NONE',  ( -5.000000000000000000, -40.95833333060215153, -2.886751345948128211 ) ) ;
#34216=CARTESIAN_POINT ( 'NONE',  ( -4.999999999999998224, 0.08333333333333454995, 2.886751345948131764 ) ) ;
#34219=CARTESIAN_POINT ( 'NONE',  ( -4.458734124999999437, -23.39583333196773296, -2.574251347313719407 ) ) ;
#34220=CARTESIAN_POINT ( 'NONE',  ( 5.000000000000000000, 0.5833333333333314830, -2.886751345948130876 ) ) ;
#34229=VERTEX_POINT ( 'NONE', #41447 ) ;
#34231=CARTESIAN_POINT ( 'NONE',  ( -6.972266317189433020E-16, -72.25000000000000000, -5.000000000000000000 ) ) ;
#34236=AXIS2_PLACEMENT_3D ( 'NONE', #9261, #32447, #38232 ) ;
#34238=CARTESIAN_POINT ( 'NONE',  ( 9.457646018065525792E-16, 18.93750000136559208, 5.148502694627439702 ) ) ;
#34243=CARTESIAN_POINT ( 'NONE',  ( -6.972266317189433020E-16, -4.124999997268814056, -5.000000000000000000 ) ) ;
#34245=CARTESIAN_POINT ( 'NONE',  ( -5.000000000000000000, -103.0000000000000142, 0.000000000000000000 ) ) ;
#34246=CARTESIAN_POINT ( 'NONE',  ( 4.458734124999998549, -60.72916666530106511, -2.574251347313721627 ) ) ;
#34247=DIRECTION ( 'NONE',  ( 0.000000000000000000, 0.000000000000000000, 1.000000000000000000 ) ) ;
#34248=CARTESIAN_POINT ( 'NONE',  ( -2.229367062500000163, 16.52083333469892779, -3.861377020970580443 ) ) ;
#34251=EDGE_CURVE ( 'NONE', #1553, #48706, #53863, .T. ) ;
#34252=CARTESIAN_POINT ( 'NONE',  ( -2.229367062499996610, -51.39583333196773651, 3.861377020970582219 ) ) ;
#34253=CARTESIAN_POINT ( 'NONE',  ( 1.060575238724906964E-15, -9.624999997268814056, 5.773502691896257311 ) ) ;
#34256=FACE_OUTER_BOUND ( 'NONE', #4697, .T. ) ;
#34258=CARTESIAN_POINT ( 'NONE',  ( 4.458734124999998549, -108.7291666653010651, -2.574251347313721627 ) ) ;
#34259=CARTESIAN_POINT ( 'NONE',  ( -3.152548672688508926E-16, -10.81249999863440792, -5.148502694627439702 ) ) ;
#34260=ORIENTED_EDGE ( 'NONE', *, *, #30358, .F. ) ;
#34262=CARTESIAN_POINT ( 'NONE',  ( 4.458734124999998549, -97.72916666530106511, -2.574251347313721627 ) ) ;
#34264=CARTESIAN_POINT ( 'NONE',  ( -3.152548672688508926E-16, -97.81249999863439371, -5.148502694627439702 ) ) ;
#34265=CARTESIAN_POINT ( 'NONE',  ( 1.975475456537005874E-15, -94.62499999726880162, 5.000000000000000000 ) ) ;
#34266=CARTESIAN_POINT ( 'NONE',  ( 2.500000000000002220, -56.54166666393548013, 4.330127018922192761 ) ) ;
#34267=EDGE_CURVE ( 'NONE', #41892, #9483, #60474, .T. ) ;
#34268=CARTESIAN_POINT ( 'NONE',  ( 2.499999999999998668, -5.333333333333335702, -4.330127018922193649 ) ) ;
#34269=ADVANCED_FACE ( 'NONE', ( #26671 ), #16388, .T. ) ;
#34272=CARTESIAN_POINT ( 'NONE',  ( -4.458734124999997661, -17.22916666530106866, 2.574251347313722516 ) ) ;
#34273=CARTESIAN_POINT ( 'NONE',  ( -2.229367062499996610, 4.604166668032261711, 3.861377020970582219 ) ) ;
#34274=CARTESIAN_POINT ( 'NONE',  ( 4.458734125000000326, -59.14583333196772230, 2.574251347313718519 ) ) ;
#34279=CARTESIAN_POINT ( 'NONE',  ( 2.500000000000002220, -5.666666666666666963, 4.330127018922192761 ) ) ;
#34280=ADVANCED_FACE ( 'NONE', ( #17336 ), #20898, .T. ) ;
#34285=CARTESIAN_POINT ( 'NONE',  ( -5.000000000000000000, -9.000000000000001776, 0.000000000000000000 ) ) ;
#34287=CARTESIAN_POINT ( 'NONE',  ( -4.458734124999999437, -85.39583333196773651, -2.574251347313719407 ) ) ;
#34288=CARTESIAN_POINT ( 'NONE',  ( -4.458734124999999437, 20.35416666803225993, -2.574251347313719407 ) ) ;
#34289=AXIS2_PLACEMENT_3D ( 'NONE', #31582, #47331, #17435 ) ;
#34295=CARTESIAN_POINT ( 'NONE',  ( -5.000000000000000000, -77.08333333333334281, -2.886751345948128211 ) ) ;
#34305=ORIENTED_EDGE ( 'NONE', *, *, #38902, .F. ) ;
#34309=VERTEX_POINT ( 'NONE', #4654 ) ;
#34312=CARTESIAN_POINT ( 'NONE',  ( 4.458734125000001214, -59.14583333196773651, 2.574251347313718519 ) ) ;
#34314=ORIENTED_EDGE ( 'NONE', *, *, #29028, .F. ) ;
#34321=CARTESIAN_POINT ( 'NONE',  ( 2.229367062499998831, -105.8958333319677365, -3.861377020970580887 ) ) ;
#34326=CARTESIAN_POINT ( 'NONE',  ( -4.458734124999999437, -37.39583333196773651, -2.574251347313719407 ) ) ;
#34329=CARTESIAN_POINT ( 'NONE',  ( 2.229367062499998831, -11.64583333196774007, -3.861377020970580887 ) ) ;
#34330=CARTESIAN_POINT ( 'NONE',  ( 2.229367062500001939, -101.2291666653010651, 3.861377020970579999 ) ) ;
#34333=( BOUNDED_CURVE ( )  B_SPLINE_CURVE ( 2, ( #20638, #40244, #59882, #15803, #10966, #50537, #25776, #11602, #20954 ),
 .UNSPECIFIED., .F., .F. ) 
 B_SPLINE_CURVE_WITH_KNOTS ( ( 3, 2, 2, 2, 3 ),
 ( 0.8982142857142857428, 0.8988095238095238360, 0.9000000000000000222, 0.9011904761904762085, 0.9017857142857143016 ),
 .UNSPECIFIED. ) 
 CURVE ( )  GEOMETRIC_REPRESENTATION_ITEM ( )  RATIONAL_B_SPLINE_CURVE ( ( 0.9330127018922194093, 0.9330127018922194093, 1.000000000000000000, 0.8660254037844387076, 1.000000000000000000, 0.8660254037844387076, 1.000000000000000000, 0.9330127018922194093, 0.9330127018922194093 ) ) 
 REPRESENTATION_ITEM ( '' )  );
#34335=CARTESIAN_POINT ( 'NONE',  ( -4.458734124999999437, -33.64583333196772941, -2.574251347313719407 ) ) ;
#34336=CARTESIAN_POINT ( 'NONE',  ( -3.535250795749689387E-16, 6.875000002731186832, -5.773502691896257311 ) ) ;
#34343=CARTESIAN_POINT ( 'NONE',  ( -4.458734124999997661, 6.520833334698930450, 2.574251347313722516 ) ) ;
#34346=CARTESIAN_POINT ( 'NONE',  ( -2.499999999999996447, -95.83333333333332860, 4.330127018922195425 ) ) ;
#34347=CARTESIAN_POINT ( 'NONE',  ( -4.458734124999999437, -30.39583333196773651, -2.574251347313719407 ) ) ;
#34348=CARTESIAN_POINT ( 'NONE',  ( 9.457646018065525792E-16, -80.31249999863440792, 5.148502694627439702 ) ) ;
#34352=CARTESIAN_POINT ( 'NONE',  ( -4.458734124999997661, -0.2291666653010705768, 2.574251347313722516 ) ) ;
#34353=DIRECTION ( 'NONE',  ( -0.000000000000000000, 1.000000000000000000, -0.000000000000000000 ) ) ;
#34354=CARTESIAN_POINT ( 'NONE',  ( -4.458734124999999437, -45.64583333196774362, -2.574251347313719407 ) ) ;
#34358=CARTESIAN_POINT ( 'NONE',  ( -2.229367062499996610, -70.14583333196773651, 3.861377020970582219 ) ) ;
#34359=CARTESIAN_POINT ( 'NONE',  ( 5.000000000000000888, -103.4583333306021444, 2.886751345948126879 ) ) ;
#34362=CARTESIAN_POINT ( 'NONE',  ( -5.000000000000000000, -65.08333333333332860, -2.886751345948128211 ) ) ;
#34363=DIRECTION ( 'NONE',  ( 0.000000000000000000, -0.000000000000000000, -1.000000000000000000 ) ) ;
#34365=CARTESIAN_POINT ( 'NONE',  ( -5.000000000000000000, -58.08333333333332860, -2.886751345948128211 ) ) ;
#34368=ORIENTED_EDGE ( 'NONE', *, *, #47833, .F. ) ;
#34379=CARTESIAN_POINT ( 'NONE',  ( 1.975475456537005874E-15, -91.62499999726878741, 5.000000000000000000 ) ) ;
#34380=CARTESIAN_POINT ( 'NONE',  ( -6.972266317189433020E-16, -62.24999999999999289, -5.000000000000000000 ) ) ;
#34382=EDGE_LOOP ( 'NONE', ( #46474, #50958, #22264, #194 ) ) ;
#34386=CARTESIAN_POINT ( 'NONE',  ( -2.229367062500000163, -40.72916666530107221, -3.861377020970580443 ) ) ;
#34387=CARTESIAN_POINT ( 'NONE',  ( 1.975475456537005874E-15, -68.62499999726881583, 5.000000000000000000 ) ) ;
#34395=CARTESIAN_POINT ( 'NONE',  ( 2.229367062499998831, -88.89583333196773651, -3.861377020970580887 ) ) ;
#34396=ORIENTED_EDGE ( 'NONE', *, *, #59883, .F. ) ;
#34397=CARTESIAN_POINT ( 'NONE',  ( 1.975475456537005874E-15, 14.37500000273118417, 5.000000000000000000 ) ) ;
#34401=CARTESIAN_POINT ( 'NONE',  ( 4.458734124999999437, 1.187500001365596081, -5.460374474430324690E-16 ) ) ;
#34402=DIRECTION ( 'NONE',  ( -0.000000000000000000, 1.000000000000000000, -0.000000000000000000 ) ) ;
#34403=CARTESIAN_POINT ( 'NONE',  ( 4.458734124999999437, -18.06249999863440792, -5.460374474430324690E-16 ) ) ;
#34408=CARTESIAN_POINT ( 'NONE',  ( -2.229367062499996610, 20.60416666803225993, 3.861377020970582219 ) ) ;
#34410=CARTESIAN_POINT ( 'NONE',  ( -2.229367062500000163, -99.47916666530106511, -3.861377020970580443 ) ) ;
#34411=CARTESIAN_POINT ( 'NONE',  ( -6.972266317189433020E-16, -26.25000000000000355, -5.000000000000000000 ) ) ;
#34413=CARTESIAN_POINT ( 'NONE',  ( -4.458734124999999437, -15.31249999863440436, 0.000000000000000000 ) ) ;
#34418=CARTESIAN_POINT ( 'NONE',  ( 5.000000000000000000, -39.37499999726880162, -6.123233995736766282E-16 ) ) ;
#34420=CARTESIAN_POINT ( 'NONE',  ( -4.458734124999997661, 15.77083333469892601, 2.574251347313722516 ) ) ;
#34421=CARTESIAN_POINT ( 'NONE',  ( 5.000000000000000000, -51.29166666393547303, -2.886751345948130876 ) ) ;
#34422=ORIENTED_EDGE ( 'NONE', *, *, #60151, .F. ) ;
#34424=CARTESIAN_POINT ( 'NONE',  ( -2.229367062499996610, -64.14583333196773651, 3.861377020970582219 ) ) ;
#34428=CARTESIAN_POINT ( 'NONE',  ( -3.535250795749689387E-16, 6.749999999999999112, -5.773502691896257311 ) ) ;
#34431=CARTESIAN_POINT ( 'NONE',  ( -4.458734124999999437, -52.39583333196773651, -2.574251347313719407 ) ) ;
#34432=CARTESIAN_POINT ( 'NONE',  ( 2.500000000000002220, -89.54166666393547303, 4.330127018922192761 ) ) ;
#34433=CARTESIAN_POINT ( 'NONE',  ( 2.229367062500001939, -34.97916666530107221, 3.861377020970579999 ) ) ;
#34435=CARTESIAN_POINT ( 'NONE',  ( 7.204675194429079505E-15, 25.87500000273118062, -5.000000000000000000 ) ) ;
#34436=CARTESIAN_POINT ( 'NONE',  ( 0.000000000000000000, -120.0000000000000000, 5.000000000000000000 ) ) ;
#34438=CARTESIAN_POINT ( 'NONE',  ( 5.000000000000000888, -40.58333333333333570, 2.886751345948126879 ) ) ;
#34439=CARTESIAN_POINT ( 'NONE',  ( 1.339745962155615144, -98.58034179853029855, 4.999999999999999112 ) ) ;
#34441=ORIENTED_EDGE ( 'NONE', *, *, #38398, .F. ) ;
#34442=CARTESIAN_POINT ( 'NONE',  ( -4.458734124999999437, -99.39583333196772230, -2.574251347313719407 ) ) ;
#34443=CARTESIAN_POINT ( 'NONE',  ( -2.229367062500000163, 1.270833334698927342, -3.861377020970580443 ) ) ;
#34450=ORIENTED_EDGE ( 'NONE', *, *, #36265, .F. ) ;
#34452=CARTESIAN_POINT ( 'NONE',  ( 1.339745962155615144, 19.29465819873852439, 4.999999999999999112 ) ) ;
#34453=CARTESIAN_POINT ( 'NONE',  ( 1.339745962155615144, -20.70534180126147916, 4.999999999999999112 ) ) ;
#34455=DIRECTION ( 'NONE',  ( 0.000000000000000000, 0.000000000000000000, 1.000000000000000000 ) ) ;
#34456=CARTESIAN_POINT ( 'NONE',  ( 4.458734125000001214, -26.14583333196774007, 2.574251347313718519 ) ) ;
#34461=EDGE_CURVE ( 'NONE', #55487, #19063, #25888, .T. ) ;
#34467=CARTESIAN_POINT ( 'NONE',  ( -3.152548672688508926E-16, -70.81249999863440792, -5.148502694627439702 ) ) ;
#34470=CARTESIAN_POINT ( 'NONE',  ( 1.975475456537005874E-15, -61.74999999999999289, 5.000000000000000000 ) ) ;
#34471=CARTESIAN_POINT ( 'NONE',  ( -1.339745962155610925, 8.205341801261479162, 5.000000000000000000 ) ) ;
#34473=CARTESIAN_POINT ( 'NONE',  ( 2.229367062500001939, -2.229166665301068662, 3.861377020970579999 ) ) ;
#34474=ORIENTED_EDGE ( 'NONE', *, *, #59883, .T. ) ;
#34476=DIRECTION ( 'NONE',  ( 0.000000000000000000, 0.000000000000000000, -1.000000000000000000 ) ) ;
#34481=VERTEX_POINT ( 'NONE', #9173 ) ;
#34482=CARTESIAN_POINT ( 'NONE',  ( 2.229367062499998831, -80.64583333196773651, -3.861377020970580887 ) ) ;
#34484=CARTESIAN_POINT ( 'NONE',  ( 9.457646018065525792E-16, 0.9375000013655959696, 5.148502694627439702 ) ) ;
#34485=CARTESIAN_POINT ( 'NONE',  ( -5.000000000000000000, -84.08333333333332860, -2.886751345948128211 ) ) ;
#34486=CARTESIAN_POINT ( 'NONE',  ( -2.500000000000000444, -43.04166666393548013, -4.330127018922193649 ) ) ;
#34487=CARTESIAN_POINT ( 'NONE',  ( 4.458734124999999437, -63.06249999863440792, -5.460374474430324690E-16 ) ) ;
#34488=CARTESIAN_POINT ( 'NONE',  ( 5.000000000000000000, -23.29166666393548368, -2.886751345948129988 ) ) ;
#34490=CARTESIAN_POINT ( 'NONE',  ( -4.458734124999997661, 27.77083333469892423, 2.574251347313722516 ) ) ;
#34492=CARTESIAN_POINT ( 'NONE',  ( -2.229367062500000163, -48.47916666530106511, -3.861377020970580443 ) ) ;
#34493=CARTESIAN_POINT ( 'NONE',  ( 2.229367062499998831, -31.89583333196773651, -3.861377020970580887 ) ) ;
#34495=VECTOR ( 'NONE', #23945, 1000.000000000000000 ) ;
#34496=CARTESIAN_POINT ( 'NONE',  ( 0.000000000000000000, -120.0000000000000000, 0.000000000000000000 ) ) ;
#34497=CARTESIAN_POINT ( 'NONE',  ( 5.000000000000000888, 21.41666666666666430, 2.886751345948126879 ) ) ;
#34500=CARTESIAN_POINT ( 'NONE',  ( 2.229367062500001939, -36.97916666530107221, 3.861377020970579999 ) ) ;
#34501=CARTESIAN_POINT ( 'NONE',  ( 5.000000000000000000, -73.29166666393548724, -2.886751345948129988 ) ) ;
#34502=VECTOR ( 'NONE', #46321, 1000.000000000000000 ) ;
#34503=VECTOR ( 'NONE', #4526, 1000.000000000000000 ) ;
#34508=CARTESIAN_POINT ( 'NONE',  ( -4.458734124999999437, -80.56249999863440792, 0.000000000000000000 ) ) ;
#34512=LINE ( 'NONE', #39033, #39973 ) ;
#34513=CARTESIAN_POINT ( 'NONE',  ( 1.060575238724906964E-15, -19.74999999999999645, 5.773502691896257311 ) ) ;
#34519=CARTESIAN_POINT ( 'NONE',  ( 2.499999999999998668, 22.79166666939785202, -4.330127018922193649 ) ) ;
#34525=CARTESIAN_POINT ( 'NONE',  ( -2.499999999999996447, -76.83333333333334281, 4.330127018922195425 ) ) ;
#34527=CARTESIAN_POINT ( 'NONE',  ( -2.499999999999996447, 5.166666666666666963, 4.330127018922195425 ) ) ;
#34528=CARTESIAN_POINT ( 'NONE',  ( -4.458734124999999437, -20.39583333196774362, -2.574251347313719407 ) ) ;
#34529=CARTESIAN_POINT ( 'NONE',  ( -6.972266317189433020E-16, 0.7499999999999996669, -5.000000000000000000 ) ) ;
#34535=CARTESIAN_POINT ( 'NONE',  ( -5.000000000000000000, 25.04166666939785202, -2.886751345948128211 ) ) ;
#34539=CARTESIAN_POINT ( 'NONE',  ( -6.972266317189433020E-16, -68.12499999726881583, -5.000000000000000000 ) ) ;
#34546=CARTESIAN_POINT ( 'NONE',  ( 5.000000000000000888, -53.45833333060213732, 2.886751345948126879 ) ) ;
#34548=VECTOR ( 'NONE', #61946, 1000.000000000000000 ) ;
#34553=CARTESIAN_POINT ( 'NONE',  ( 4.458734124999999437, 17.18750000136559564, -5.460374474430324690E-16 ) ) ;
#34554=CARTESIAN_POINT ( 'NONE',  ( -5.000000000000000000, -84.99999999999998579, 0.000000000000000000 ) ) ;
#34559=CYLINDRICAL_SURFACE ( 'NONE', #11059, 5.000000000000000000 ) ;
#34563=CARTESIAN_POINT ( 'NONE',  ( -2.229367062499996610, -66.14583333196773651, 3.861377020970582219 ) ) ;
#34565=CARTESIAN_POINT ( 'NONE',  ( -2.229367062500000163, 18.52083333469892779, -3.861377020970580443 ) ) ;
#34566=CYLINDRICAL_SURFACE ( 'NONE', #13398, 5.000000000000000000 ) ;
#34567=CARTESIAN_POINT ( 'NONE',  ( 4.458734125000001214, -52.14583333196772941, 2.574251347313718519 ) ) ;
#34568=CARTESIAN_POINT ( 'NONE',  ( -2.499999999999996447, -11.70833333060214798, 4.330127018922195425 ) ) ;
#34569=CARTESIAN_POINT ( 'NONE',  ( 1.975475456537005874E-15, -108.7499999999999858, 5.000000000000000000 ) ) ;
#34570=FACE_OUTER_BOUND ( 'NONE', #57701, .T. ) ;
#34572=CARTESIAN_POINT ( 'NONE',  ( -2.229367062499996610, -110.1458333319677365, 3.861377020970582219 ) ) ;
#34573=CARTESIAN_POINT ( 'NONE',  ( -4.458734124999997661, -16.47916666530107577, 2.574251347313722516 ) ) ;
#34574=VERTEX_POINT ( 'NONE', #29397 ) ;
#34575=DIRECTION ( 'NONE',  ( 0.000000000000000000, 0.000000000000000000, 1.000000000000000000 ) ) ;
#34576=CARTESIAN_POINT ( 'NONE',  ( -4.458734124999998549, -97.22916666530105090, 2.574251347313722516 ) ) ;
#34578=CARTESIAN_POINT ( 'NONE',  ( 4.458734124999999437, -100.0624999986344079, -5.460374474430324690E-16 ) ) ;
#34580=CARTESIAN_POINT ( 'NONE',  ( 0.000000000000000000, -120.0000000000000000, 0.000000000000000000 ) ) ;
#34581=CARTESIAN_POINT ( 'NONE',  ( 5.000000000000000000, -59.29166666393547303, -2.886751345948129988 ) ) ;
#34582=CARTESIAN_POINT ( 'NONE',  ( -2.500000000000000444, 18.95833333606451632, -4.330127018922193649 ) ) ;
#34585=CARTESIAN_POINT ( 'NONE',  ( -4.458734124999999437, -19.31249999863440081, 0.000000000000000000 ) ) ;
#34586=CARTESIAN_POINT ( 'NONE',  ( -4.458734124999999437, 8.354166668032261711, -2.574251347313719407 ) ) ;
#34588=CARTESIAN_POINT ( 'NONE',  ( -4.458734124999997661, -56.47916666530107221, 2.574251347313722516 ) ) ;
#34589=FACE_OUTER_BOUND ( 'NONE', #12745, .T. ) ;
#34593=CARTESIAN_POINT ( 'NONE',  ( -2.499999999999996447, -5.833333333333336590, 4.330127018922195425 ) ) ;
#34596=AXIS2_PLACEMENT_3D ( 'NONE', #46212, #21780, #36881 ) ;
#34600=CARTESIAN_POINT ( 'NONE',  ( -4.458734124999999437, -92.39583333196773651, -2.574251347313719407 ) ) ;
#34601=CARTESIAN_POINT ( 'NONE',  ( 4.458734124999998549, 19.02083333469892779, -2.574251347313721627 ) ) ;
#34603=VECTOR ( 'NONE', #27469, 1000.000000000000000 ) ;
#34605=CARTESIAN_POINT ( 'NONE',  ( 5.000000000000000000, -93.41666666666667140, -2.886751345948130876 ) ) ;
#34610=CARTESIAN_POINT ( 'NONE',  ( 2.500000000000002220, -74.66666666666665719, 4.330127018922192761 ) ) ;
#34613=CARTESIAN_POINT ( 'NONE',  ( 0.000000000000000000, -120.0000000000000000, 5.000000000000000000 ) ) ;
#34615=( BOUNDED_CURVE ( )  B_SPLINE_CURVE ( 2, ( #25433, #16426, #55675, #49867, #21248, #50839, #10949, #61138, #16103 ),
 .UNSPECIFIED., .F., .F. ) 
 B_SPLINE_CURVE_WITH_KNOTS ( ( 3, 2, 2, 2, 3 ),
 ( 0.01964285714285714593, 0.02023809523809523905, 0.02142857142857142877, 0.02261904761904761849, 0.02321428571428571508 ),
 .UNSPECIFIED. ) 
 CURVE ( )  GEOMETRIC_REPRESENTATION_ITEM ( )  RATIONAL_B_SPLINE_CURVE ( ( 0.9330127018922194093, 0.9330127018922195203, 1.000000000000000000, 0.8660254037844387076, 1.000000000000000000, 0.8660254037844387076, 1.000000000000000000, 0.9330127018922191873, 0.9330127018922194093 ) ) 
 REPRESENTATION_ITEM ( '' )  );
#34619=ADVANCED_FACE ( 'NONE', ( #3190 ), #52069, .T. ) ;
#34621=ADVANCED_FACE ( 'NONE', ( #45812 ), #59333, .T. ) ;
#34626=VERTEX_POINT ( 'NONE', #40662 ) ;
#34630=CARTESIAN_POINT ( 'NONE',  ( 4.458734124999998549, -55.97916666530107932, -2.574251347313721627 ) ) ;
#34632=FACE_OUTER_BOUND ( 'NONE', #54887, .T. ) ;
#34636=CARTESIAN_POINT ( 'NONE',  ( 5.000000000000000888, -41.45833333060214443, 2.886751345948126879 ) ) ;
#34641=EDGE_CURVE ( 'NONE', #36504, #50783, #39027, .T. ) ;
#34642=CARTESIAN_POINT ( 'NONE',  ( 4.458734124999999437, -106.0624999986344221, -5.460374474430324690E-16 ) ) ;
#34644=ORIENTED_EDGE ( 'NONE', *, *, #16228, .F. ) ;
#34648=CARTESIAN_POINT ( 'NONE',  ( -4.458734124999999437, -44.39583333196774362, -2.574251347313719407 ) ) ;
#34655=CARTESIAN_POINT ( 'NONE',  ( -4.458734124999998549, -11.22916666530106866, 2.574251347313722516 ) ) ;
#34656=AXIS2_PLACEMENT_3D ( 'NONE', #393, #5524, #34455 ) ;
#34657=CARTESIAN_POINT ( 'NONE',  ( 2.500000000000002220, -99.66666666666665719, 4.330127018922192761 ) ) ;
#34660=CARTESIAN_POINT ( 'NONE',  ( -4.458734124999999437, -35.64583333196772941, -2.574251347313719407 ) ) ;
#34661=AXIS2_PLACEMENT_3D ( 'NONE', #40380, #60021, #15944 ) ;
#34662=CARTESIAN_POINT ( 'NONE',  ( 1.060575238724906964E-15, 8.375000002731187720, 5.773502691896257311 ) ) ;
#34663=CARTESIAN_POINT ( 'NONE',  ( 6.123233995736766282E-16, -120.0000000000000000, -5.000000000000000000 ) ) ;
#34666=FACE_OUTER_BOUND ( 'NONE', #32205, .T. ) ;
#34667=DIRECTION ( 'NONE',  ( -0.000000000000000000, 1.000000000000000000, -0.000000000000000000 ) ) ;
#34669=CARTESIAN_POINT ( 'NONE',  ( -4.458734124999997661, 5.520833334698926009, 2.574251347313722516 ) ) ;
#34670=ORIENTED_EDGE ( 'NONE', *, *, #41385, .T. ) ;
#34671=CARTESIAN_POINT ( 'NONE',  ( 2.499999999999998668, -30.33333333333332860, -4.330127018922193649 ) ) ;
#34673=CARTESIAN_POINT ( 'NONE',  ( 5.000000000000000000, -93.50000000000000000, -6.123233995736766282E-16 ) ) ;
#34674=CARTESIAN_POINT ( 'NONE',  ( 4.458734125000001214, -29.89583333196773651, 2.574251347313718519 ) ) ;
#34675=CARTESIAN_POINT ( 'NONE',  ( -5.000000000000000000, -22.95833333060214798, -2.886751345948128211 ) ) ;
#34676=CARTESIAN_POINT ( 'NONE',  ( 4.458734124999999437, -79.06249999863440792, -5.460374474430324690E-16 ) ) ;
#34680=CARTESIAN_POINT ( 'NONE',  ( -2.229367062500000163, -3.479166665301069994, -3.861377020970580443 ) ) ;
#34681=CARTESIAN_POINT ( 'NONE',  ( 2.229367062499998831, 22.10416666803225993, -3.861377020970580887 ) ) ;
#34682=CARTESIAN_POINT ( 'NONE',  ( 4.458734125000000326, -43.14583333196773651, 2.574251347313718519 ) ) ;
#34683=CARTESIAN_POINT ( 'NONE',  ( 5.000000000000000000, -15.50000000000000000, -6.123233995736766282E-16 ) ) ;
#34686=CARTESIAN_POINT ( 'NONE',  ( -4.458734124999998549, -68.22916666530107932, 2.574251347313722516 ) ) ;
#34687=CARTESIAN_POINT ( 'NONE',  ( -2.500000000000000444, -103.0416666639354730, -4.330127018922193649 ) ) ;
#34690=CARTESIAN_POINT ( 'NONE',  ( -2.229367062500000163, -109.7291666653010651, -3.861377020970580443 ) ) ;
#34692=CARTESIAN_POINT ( 'NONE',  ( -5.000000000000000000, -59.00000000000000000, 0.000000000000000000 ) ) ;
#34694=CARTESIAN_POINT ( 'NONE',  ( -1.339745962155610925, -31.66965819600733312, 5.000000000000000000 ) ) ;
#34698=AXIS2_PLACEMENT_3D ( 'NONE', #63161, #43515, #14254 ) ;
#34699=CARTESIAN_POINT ( 'NONE',  ( -2.499999999999996447, -98.83333333333332860, 4.330127018922195425 ) ) ;
#34705=EDGE_CURVE ( 'NONE', #49354, #19379, #45620, .T. ) ;
#34716=CARTESIAN_POINT ( 'NONE',  ( 9.457646018065525792E-16, -41.31249999863440081, 5.148502694627439702 ) ) ;
#34717=CARTESIAN_POINT ( 'NONE',  ( 1.975475456537005874E-15, -23.75000000000000000, 5.000000000000000000 ) ) ;
#34719=CARTESIAN_POINT ( 'NONE',  ( -4.999999999999998224, -56.79166666393547303, 2.886751345948131764 ) ) ;
#34726=CARTESIAN_POINT ( 'NONE',  ( 4.458734124999999437, -91.06249999863440792, -5.460374474430324690E-16 ) ) ;
#34729=EDGE_CURVE ( 'NONE', #23099, #39107, #25875, .T. ) ;
#34730=FACE_OUTER_BOUND ( 'NONE', #20665, .T. ) ;
#34733=ADVANCED_FACE ( 'NONE', ( #50640 ), #45172, .T. ) ;
#34735=VERTEX_POINT ( 'NONE', #56434 ) ;
#34736=CARTESIAN_POINT ( 'NONE',  ( -2.229367062499996610, 2.854166668032259935, 3.861377020970582219 ) ) ;
#34738=CARTESIAN_POINT ( 'NONE',  ( -1.336351044127974539E-14, 21.37500000273118417, 5.000000000000000000 ) ) ;
#34739=CARTESIAN_POINT ( 'NONE',  ( 4.458734124999999437, -19.06249999863440792, -5.460374474430324690E-16 ) ) ;
#34740=DIRECTION ( 'NONE',  ( -0.000000000000000000, 1.000000000000000000, -0.000000000000000000 ) ) ;
#34742=CARTESIAN_POINT ( 'NONE',  ( 0.000000000000000000, -120.0000000000000000, 5.000000000000000000 ) ) ;
#34744=VECTOR ( 'NONE', #44654, 1000.000000000000000 ) ;
#34745=CARTESIAN_POINT ( 'NONE',  ( -4.458734124999999437, 20.43750000136559208, 0.000000000000000000 ) ) ;
#34747=CARTESIAN_POINT ( 'NONE',  ( 4.458734124999999437, -97.81249999863440792, -5.460374474430324690E-16 ) ) ;
#34749=CARTESIAN_POINT ( 'NONE',  ( -1.339745962155613812, -104.0803417985302701, -5.000000000000000000 ) ) ;
#34750=CARTESIAN_POINT ( 'NONE',  ( -4.458734124999998549, -14.22916666530107221, 2.574251347313722516 ) ) ;
#34751=AXIS2_PLACEMENT_3D ( 'NONE', #27281, #8303, #12800 ) ;
#34755=CARTESIAN_POINT ( 'NONE',  ( -2.500000000000000444, -41.04166666393548013, -4.330127018922193649 ) ) ;
#34757=CARTESIAN_POINT ( 'NONE',  ( -4.458734124999999437, 13.60416666803226171, -2.574251347313719407 ) ) ;
#34761=CARTESIAN_POINT ( 'NONE',  ( 4.458734124999999437, -63.81249999863440792, -5.460374474430324690E-16 ) ) ;
#34764=CARTESIAN_POINT ( 'NONE',  ( -5.000000000000000000, 1.916666666666667407, -2.886751345948128211 ) ) ;
#34767=CARTESIAN_POINT ( 'NONE',  ( 9.457646018065525792E-16, -51.06249999863440792, 5.148502694627439702 ) ) ;
#34768=CARTESIAN_POINT ( 'NONE',  ( 1.060575238724906964E-15, -91.62499999726880162, 5.773502691896257311 ) ) ;
#34769=CARTESIAN_POINT ( 'NONE',  ( 2.229367062499998831, -31.64583333196773651, -3.861377020970580887 ) ) ;
#34771=CARTESIAN_POINT ( 'NONE',  ( 0.000000000000000000, -120.0000000000000000, 0.000000000000000000 ) ) ;
#34772=CARTESIAN_POINT ( 'NONE',  ( 2.500000000000002220, -8.666666666666669627, 4.330127018922192761 ) ) ;
#34775=CARTESIAN_POINT ( 'NONE',  ( 2.499999999999998668, -43.33333333333333570, -4.330127018922193649 ) ) ;
#34779=CARTESIAN_POINT ( 'NONE',  ( 4.458734124999998549, -100.7291666653010651, -2.574251347313721627 ) ) ;
#34780=CARTESIAN_POINT ( 'NONE',  ( 4.458734124999998549, 1.020833334698927120, -2.574251347313721627 ) ) ;
#34785=ADVANCED_FACE ( 'NONE', ( #61573 ), #42251, .T. ) ;
#34790=ORIENTED_EDGE ( 'NONE', *, *, #2880, .T. ) ;
#34793=ORIENTED_EDGE ( 'NONE', *, *, #14068, .F. ) ;
#34794=CARTESIAN_POINT ( 'NONE',  ( 3.044556291839386294E-14, 12.75000000000000000, -5.000000000000000000 ) ) ;
#34796=FACE_OUTER_BOUND ( 'NONE', #23889, .T. ) ;
#34797=CARTESIAN_POINT ( 'NONE',  ( 2.229367062499998831, -25.89583333196773651, -3.861377020970580887 ) ) ;
#34802=VECTOR ( 'NONE', #14139, 1000.000000000000000 ) ;
#34806=ORIENTED_EDGE ( 'NONE', *, *, #57825, .T. ) ;
#34809=CARTESIAN_POINT ( 'NONE',  ( -3.152548672688508926E-16, -73.81249999863440792, -5.148502694627439702 ) ) ;
#34810=CARTESIAN_POINT ( 'NONE',  ( 0.000000000000000000, -120.0000000000000000, 0.000000000000000000 ) ) ;
#34812=CARTESIAN_POINT ( 'NONE',  ( 1.339745962155627135, 12.70534180126147739, -4.999999999999991118 ) ) ;
#34816=CARTESIAN_POINT ( 'NONE',  ( -2.229367062500000163, -3.729166665301070438, -3.861377020970580443 ) ) ;
#34818=VECTOR ( 'NONE', #19090, 1000.000000000000000 ) ;
#34819=CARTESIAN_POINT ( 'NONE',  ( 1.975475456537005874E-15, -19.75000000000000000, 5.000000000000000000 ) ) ;
#34820=CARTESIAN_POINT ( 'NONE',  ( 5.000000000000000000, -91.50000000000000000, -6.123233995736766282E-16 ) ) ;
#34826=CARTESIAN_POINT ( 'NONE',  ( 4.458734124999998549, -80.72916666530106511, -2.574251347313721627 ) ) ;
#34828=CARTESIAN_POINT ( 'NONE',  ( -4.458734124999999437, 1.687500001365593194, 0.000000000000000000 ) ) ;
#34829=CARTESIAN_POINT ( 'NONE',  ( 1.060575238724906964E-15, -86.75000000000000000, 5.773502691896257311 ) ) ;
#34830=CARTESIAN_POINT ( 'NONE',  ( -1.339745962155610925, -42.66965819600731891, 5.000000000000000000 ) ) ;
#34831=CARTESIAN_POINT ( 'NONE',  ( 2.229367062500001939, -63.22916666530106511, 3.861377020970579999 ) ) ;
#34832=CARTESIAN_POINT ( 'NONE',  ( 2.499999999999998668, -26.20833333060214798, -4.330127018922193649 ) ) ;
#34833=DIRECTION ( 'NONE',  ( -0.000000000000000000, 1.000000000000000000, -0.000000000000000000 ) ) ;
#34834=CARTESIAN_POINT ( 'NONE',  ( 1.975475456537005874E-15, -46.62499999726880873, 5.000000000000000000 ) ) ;
#34836=DIRECTION ( 'NONE',  ( 0.000000000000000000, 0.000000000000000000, 1.000000000000000000 ) ) ;
#34837=CARTESIAN_POINT ( 'NONE',  ( 2.229367062500001939, -45.97916666530106511, 3.861377020970579999 ) ) ;
#34839=CARTESIAN_POINT ( 'NONE',  ( -4.458734124999997661, -31.47916666530107577, 2.574251347313722516 ) ) ;
#34843=CARTESIAN_POINT ( 'NONE',  ( 5.000000000000000000, 20.49999999999999645, -6.123233995736766282E-16 ) ) ;
#34847=VECTOR ( 'NONE', #49909, 1000.000000000000000 ) ;
#34848=CARTESIAN_POINT ( 'NONE',  ( -4.458734124999999437, -35.39583333196773651, -2.574251347313719407 ) ) ;
#34849=CARTESIAN_POINT ( 'NONE',  ( -2.500000000000000444, -72.04166666393548724, -4.330127018922193649 ) ) ;
#34852=CARTESIAN_POINT ( 'NONE',  ( 5.000000000000000888, -37.58333333333332860, 2.886751345948126879 ) ) ;
#34853=CARTESIAN_POINT ( 'NONE',  ( 9.457646018065525792E-16, -82.31249999863440792, 5.148502694627439702 ) ) ;
#34857=CARTESIAN_POINT ( 'NONE',  ( -5.000000000000000000, -25.00000000000000000, 0.000000000000000000 ) ) ;
#34859=ORIENTED_EDGE ( 'NONE', *, *, #11469, .F. ) ;
#34863=CARTESIAN_POINT ( 'NONE',  ( 5.000000000000000000, 23.70833333606451632, -2.886751345948129988 ) ) ;
#34866=AXIS2_PLACEMENT_3D ( 'NONE', #35493, #55111, #10081 ) ;
#34871=DIRECTION ( 'NONE',  ( -0.000000000000000000, 1.000000000000000000, -0.000000000000000000 ) ) ;
#34875=CARTESIAN_POINT ( 'NONE',  ( 4.458734124999998549, -20.72916666530106866, -2.574251347313721627 ) ) ;
#34876=CARTESIAN_POINT ( 'NONE',  ( 2.500000000000002220, 17.45833333606451987, 4.330127018922192761 ) ) ;
#34881=CARTESIAN_POINT ( 'NONE',  ( 1.975475456537005874E-15, -47.62499999726880873, 5.000000000000000000 ) ) ;
#34883=VERTEX_POINT ( 'NONE', #46131 ) ;
#34885=DIRECTION ( 'NONE',  ( -0.000000000000000000, 1.000000000000000000, -0.000000000000000000 ) ) ;
#34887=ORIENTED_EDGE ( 'NONE', *, *, #17311, .F. ) ;
#34888=CARTESIAN_POINT ( 'NONE',  ( 5.000000000000000000, -23.37499999726881228, -6.123233995736766282E-16 ) ) ;
#34894=CARTESIAN_POINT ( 'NONE',  ( 2.499999999999998668, -103.2083333306021444, -4.330127018922193649 ) ) ;
#34895=CARTESIAN_POINT ( 'NONE',  ( 4.458734124999999437, 11.18750000136559386, -5.460374474430324690E-16 ) ) ;
#34898=DIRECTION ( 'NONE',  ( 0.000000000000000000, 0.000000000000000000, 1.000000000000000000 ) ) ;
#34901=CARTESIAN_POINT ( 'NONE',  ( -4.458734124999999437, -63.31249999863440792, 0.000000000000000000 ) ) ;
#34903=CARTESIAN_POINT ( 'NONE',  ( 2.229367062500001939, 18.02083333469892779, 3.861377020970579999 ) ) ;
#34906=CARTESIAN_POINT ( 'NONE',  ( -2.229367062499996610, -49.39583333196772941, 3.861377020970582219 ) ) ;
#34907=CARTESIAN_POINT ( 'NONE',  ( 2.499999999999998668, -7.208333330602150646, -4.330127018922193649 ) ) ;
#34912=CARTESIAN_POINT ( 'NONE',  ( -4.458734124999999437, -15.56249999863440436, 0.000000000000000000 ) ) ;
#34914=FACE_OUTER_BOUND ( 'NONE', #27191, .T. ) ;
#34915=CARTESIAN_POINT ( 'NONE',  ( 4.458734124999999437, -102.8124999986344079, -5.460374474430324690E-16 ) ) ;
#34917=CARTESIAN_POINT ( 'NONE',  ( -3.152548672688508926E-16, -95.81249999863440792, -5.148502694627439702 ) ) ;
#34919=CARTESIAN_POINT ( 'NONE',  ( -5.000000000000000000, -8.000000000000000000, 0.000000000000000000 ) ) ;
#34920=CARTESIAN_POINT ( 'NONE',  ( 5.000000000000000000, -56.37499999726880162, -6.123233995736766282E-16 ) ) ;
#34921=CARTESIAN_POINT ( 'NONE',  ( 5.000000000000000000, -62.29166666393547303, -2.886751345948130876 ) ) ;
#34924=CARTESIAN_POINT ( 'NONE',  ( 2.229367062499998831, -16.64583333196773651, -3.861377020970580887 ) ) ;
#34925=CARTESIAN_POINT ( 'NONE',  ( -4.458734124999999437, 7.437500001365594748, 0.000000000000000000 ) ) ;
#34926=CARTESIAN_POINT ( 'NONE',  ( 4.458734125000000326, -64.14583333196773651, 2.574251347313718519 ) ) ;
#34931=CARTESIAN_POINT ( 'NONE',  ( -5.000000000000000000, -6.999999999999999112, 0.000000000000000000 ) ) ;
#34933=EDGE_LOOP ( 'NONE', ( #30943, #23344, #30919, #22572 ) ) ;
#34936=CARTESIAN_POINT ( 'NONE',  ( -6.972266317189433020E-16, -66.24999999999998579, -5.000000000000000000 ) ) ;
#34938=CARTESIAN_POINT ( 'NONE',  ( -3.152548672688508926E-16, -90.56249999863440792, -5.148502694627439702 ) ) ;
#34939=CARTESIAN_POINT ( 'NONE',  ( 2.229367062500001939, 13.77083333469892779, 3.861377020970579999 ) ) ;
#34941=EDGE_CURVE ( 'NONE', #11847, #24623, #12027, .T. ) ;
#34942=CARTESIAN_POINT ( 'NONE',  ( 5.000000000000000000, -82.50000000000000000, -6.123233995736766282E-16 ) ) ;
#34945=CYLINDRICAL_SURFACE ( 'NONE', #53990, 5.000000000000000000 ) ;
#34947=CARTESIAN_POINT ( 'NONE',  ( 2.499999999999998668, -75.33333333333332860, -4.330127018922193649 ) ) ;
#34951=VERTEX_POINT ( 'NONE', #61892 ) ;
#34952=DIRECTION ( 'NONE',  ( 0.000000000000000000, 0.000000000000000000, 1.000000000000000000 ) ) ;
#34960=ORIENTED_EDGE ( 'NONE', *, *, #50629, .T. ) ;
#34964=CARTESIAN_POINT ( 'NONE',  ( 4.458734124999998549, -64.97916666530106511, -2.574251347313721627 ) ) ;
#34965=( BOUNDED_CURVE ( )  B_SPLINE_CURVE ( 2, ( #26246, #6015, #40079, #21112, #6326, #20798, #36223, #26574, #55215 ),
 .UNSPECIFIED., .F., .F. ) 
 B_SPLINE_CURVE_WITH_KNOTS ( ( 3, 2, 2, 2, 3 ),
 ( 0.5910714285714285809, 0.5916666666666666741, 0.5928571428571428603, 0.5940476190476190466, 0.5946428571428571397 ),
 .UNSPECIFIED. ) 
 CURVE ( )  GEOMETRIC_REPRESENTATION_ITEM ( )  RATIONAL_B_SPLINE_CURVE ( ( 0.9330127018922194093, 0.9330127018922194093, 1.000000000000000000, 0.8660254037844387076, 1.000000000000000000, 0.8660254037844387076, 1.000000000000000000, 0.9330127018922194093, 0.9330127018922194093 ) ) 
 REPRESENTATION_ITEM ( '' )  );
#34971=CARTESIAN_POINT ( 'NONE',  ( 1.339745962155615144, -41.58034179853029144, 4.999999999999999112 ) ) ;
#34972=ORIENTED_EDGE ( 'NONE', *, *, #14939, .T. ) ;
#34975=CARTESIAN_POINT ( 'NONE',  ( -3.152548672688508926E-16, -109.8124999986343795, -5.148502694627439702 ) ) ;
#34982=CARTESIAN_POINT ( 'NONE',  ( 4.458734124999999437, -42.81249999863440081, -5.460374474430324690E-16 ) ) ;
#34985=CARTESIAN_POINT ( 'NONE',  ( -4.458734124999999437, -49.31249999863440792, 0.000000000000000000 ) ) ;
#34987=CARTESIAN_POINT ( 'NONE',  ( -3.152548672688508926E-16, -14.56249999863440436, -5.148502694627439702 ) ) ;
#34988=CARTESIAN_POINT ( 'NONE',  ( 5.000000000000000888, -100.5833333333333144, 2.886751345948126879 ) ) ;
#34990=CARTESIAN_POINT ( 'NONE',  ( -4.458734124999999437, -31.56249999863440436, 0.000000000000000000 ) ) ;
#34991=CARTESIAN_POINT ( 'NONE',  ( 5.000000000000000000, 4.625000002731187720, -6.123233995736766282E-16 ) ) ;
#34995=CARTESIAN_POINT ( 'NONE',  ( 0.000000000000000000, -120.0000000000000000, 0.000000000000000000 ) ) ;
#34996=CARTESIAN_POINT ( 'NONE',  ( 0.000000000000000000, -120.0000000000000000, 5.000000000000000000 ) ) ;
#34998=CARTESIAN_POINT ( 'NONE',  ( -4.458734124999999437, 0.3541666680322609340, -2.574251347313719407 ) ) ;
#35001=LINE ( 'NONE', #10230, #14393 ) ;
#35002=CARTESIAN_POINT ( 'NONE',  ( -4.458734124999999437, -86.31249999863439371, 0.000000000000000000 ) ) ;
#35003=CARTESIAN_POINT ( 'NONE',  ( -2.229367062499996610, -36.14583333196773651, 3.861377020970582219 ) ) ;
#35005=CARTESIAN_POINT ( 'NONE',  ( 2.229367062499998831, -81.89583333196773651, -3.861377020970580887 ) ) ;
#35012=CARTESIAN_POINT ( 'NONE',  ( -3.152548672688508926E-16, 0.4375000013655955255, -5.148502694627439702 ) ) ;
#35013=CARTESIAN_POINT ( 'NONE',  ( -4.458734124999999437, 21.35416666803225993, -2.574251347313719407 ) ) ;
#35014=CARTESIAN_POINT ( 'NONE',  ( 2.229367062500001939, -48.22916666530106511, 3.861377020970579999 ) ) ;
#35015=CARTESIAN_POINT ( 'NONE',  ( 0.000000000000000000, -120.0000000000000000, 0.000000000000000000 ) ) ;
#35018=( BOUNDED_CURVE ( )  B_SPLINE_CURVE ( 2, ( #16409, #50175, #40521, #11884, #5797, #6127, #35710, #11572, #36026 ),
 .UNSPECIFIED., .F., .F. ) 
 B_SPLINE_CURVE_WITH_KNOTS ( ( 3, 2, 2, 2, 3 ),
 ( 0.3053571428571428825, 0.3059523809523809756, 0.3071428571428571619, 0.3083333333333333481, 0.3089285714285714413 ),
 .UNSPECIFIED. ) 
 CURVE ( )  GEOMETRIC_REPRESENTATION_ITEM ( )  RATIONAL_B_SPLINE_CURVE ( ( 0.9330127018922194093, 0.9330127018922194093, 1.000000000000000000, 0.8660254037844387076, 1.000000000000000000, 0.8660254037844387076, 1.000000000000000000, 0.9330127018922194093, 0.9330127018922194093 ) ) 
 REPRESENTATION_ITEM ( '' )  );
#35020=CARTESIAN_POINT ( 'NONE',  ( 4.458734125000001214, -73.89583333196773651, 2.574251347313718519 ) ) ;
#35021=CARTESIAN_POINT ( 'NONE',  ( -4.999999999999999112, -104.7916666639354730, 2.886751345948131764 ) ) ;
#35026=DIRECTION ( 'NONE',  ( -0.000000000000000000, 1.000000000000000000, -0.000000000000000000 ) ) ;
#35028=CARTESIAN_POINT ( 'NONE',  ( -4.999999999999999112, -60.91666666666666430, 2.886751345948131764 ) ) ;
#35029=CARTESIAN_POINT ( 'NONE',  ( 1.339745962155612702, -36.16965819600732601, -5.000000000000000000 ) ) ;
#35031=ORIENTED_EDGE ( 'NONE', *, *, #23550, .F. ) ;
#35040=ORIENTED_EDGE ( 'NONE', *, *, #62642, .F. ) ;
#35041=CARTESIAN_POINT ( 'NONE',  ( -4.999999999999998224, -75.79166666393547303, 2.886751345948131764 ) ) ;
#35042=CARTESIAN_POINT ( 'NONE',  ( 5.000000000000000000, 27.70833333606451987, -2.886751345948130876 ) ) ;
#35044=ORIENTED_EDGE ( 'NONE', *, *, #46061, .T. ) ;
#35048=CARTESIAN_POINT ( 'NONE',  ( 2.229367062500001939, -46.22916666530106511, 3.861377020970579999 ) ) ;
#35051=DIRECTION ( 'NONE',  ( -0.000000000000000000, 1.000000000000000000, -0.000000000000000000 ) ) ;
#35055=FACE_OUTER_BOUND ( 'NONE', #33956, .T. ) ;
#35057=CARTESIAN_POINT ( 'NONE',  ( 9.457646018065525792E-16, -89.31249999863440792, 5.148502694627439702 ) ) ;
#35061=DIRECTION ( 'NONE',  ( 0.4999999999999951150, 0.000000000000000000, -0.8660254037844414832 ) ) ;
#35064=ORIENTED_EDGE ( 'NONE', *, *, #8612, .T. ) ;
#35065=CARTESIAN_POINT ( 'NONE',  ( 4.458734125000001214, 3.104166668032260379, 2.574251347313718519 ) ) ;
#35067=CARTESIAN_POINT ( 'NONE',  ( 4.458734125000001214, -20.14583333196774007, 2.574251347313718519 ) ) ;
#35071=CARTESIAN_POINT ( 'NONE',  ( -2.229367062500000163, 17.27083333469892779, -3.861377020970580443 ) ) ;
#35073=CARTESIAN_POINT ( 'NONE',  ( 2.229367062500001939, -95.97916666530105090, 3.861377020970579999 ) ) ;
#35074=CARTESIAN_POINT ( 'NONE',  ( 2.499999999999998668, -71.20833333060214443, -4.330127018922193649 ) ) ;
#35075=CARTESIAN_POINT ( 'NONE',  ( -4.458734124999999437, -21.31249999863440436, 0.000000000000000000 ) ) ;
#35077=CARTESIAN_POINT ( 'NONE',  ( 1.339745962155612702, -3.294658198738522170, -5.000000000000000000 ) ) ;
#35080=CARTESIAN_POINT ( 'NONE',  ( -5.000000000000000000, -43.87499999726880873, 0.000000000000000000 ) ) ;
#35082=CARTESIAN_POINT ( 'NONE',  ( -4.458734124999999437, 14.60416666803226171, -2.574251347313719407 ) ) ;
#35083=CARTESIAN_POINT ( 'NONE',  ( -4.999999999999998224, -8.791666663935483683, 2.886751345948131764 ) ) ;
#35086=CARTESIAN_POINT ( 'NONE',  ( -3.152548672688508926E-16, -61.56249999863440792, -5.148502694627439702 ) ) ;
#35090=CARTESIAN_POINT ( 'NONE',  ( -2.500000000000000444, 5.833333333333333037, -4.330127018922193649 ) ) ;
#35092=CARTESIAN_POINT ( 'NONE',  ( 4.458734124999998549, -57.72916666530107221, -2.574251347313721627 ) ) ;
#35093=CARTESIAN_POINT ( 'NONE',  ( -3.535250795749689387E-16, -89.12499999726880162, -5.773502691896257311 ) ) ;
#35094=CARTESIAN_POINT ( 'NONE',  ( 2.229367062499998831, -33.64583333196772941, -3.861377020970580887 ) ) ;
#35098=CYLINDRICAL_SURFACE ( 'NONE', #36003, 5.000000000000000000 ) ;
#35100=CARTESIAN_POINT ( 'NONE',  ( -1.339745962155610925, -107.6696581960073189, 5.000000000000000000 ) ) ;
#35101=CARTESIAN_POINT ( 'NONE',  ( 1.339745962155615144, -16.58034179853029499, 4.999999999999999112 ) ) ;
#35103=CARTESIAN_POINT ( 'NONE',  ( 5.000000000000000000, -44.50000000000000000, -6.123233995736766282E-16 ) ) ;
#35104=DIRECTION ( 'NONE',  ( -0.000000000000000000, 1.000000000000000000, -0.000000000000000000 ) ) ;
#35105=EDGE_CURVE ( 'NONE', #27768, #35769, #23895, .T. ) ;
#35106=CARTESIAN_POINT ( 'NONE',  ( -6.031010364368858512E-14, 2.375000002731183280, 5.000000000000000000 ) ) ;
#35108=CARTESIAN_POINT ( 'NONE',  ( 4.458734124999999437, -98.81249999863440792, -5.460374474430324690E-16 ) ) ;
#35109=CARTESIAN_POINT ( 'NONE',  ( 9.457646018065525792E-16, 0.6875000013655957476, 5.148502694627439702 ) ) ;
#35114=( BOUNDED_CURVE ( )  B_SPLINE_CURVE ( 2, ( #45055, #1022, #50197, #6148, #60185, #25764, #20942, #45376, #35732 ),
 .UNSPECIFIED., .F., .F. ) 
 B_SPLINE_CURVE_WITH_KNOTS ( ( 3, 2, 2, 2, 3 ),
 ( 0.5053571428571428381, 0.5059523809523809312, 0.5071428571428571175, 0.5083333333333333037, 0.5089285714285713969 ),
 .UNSPECIFIED. ) 
 CURVE ( )  GEOMETRIC_REPRESENTATION_ITEM ( )  RATIONAL_B_SPLINE_CURVE ( ( 0.9330127018922194093, 0.9330127018922194093, 1.000000000000000000, 0.8660254037844387076, 1.000000000000000000, 0.8660254037844387076, 1.000000000000000000, 0.9330127018922194093, 0.9330127018922194093 ) ) 
 REPRESENTATION_ITEM ( '' )  );
#35116=EDGE_CURVE ( 'NONE', #63012, #19213, #27953, .T. ) ;
#35119=ORIENTED_EDGE ( 'NONE', *, *, #17017, .T. ) ;
#35120=CARTESIAN_POINT ( 'NONE',  ( 3.253724281355068545E-15, 27.87500000273118417, -5.000000000000000000 ) ) ;
#35121=ORIENTED_EDGE ( 'NONE', *, *, #22380, .T. ) ;
#35122=CARTESIAN_POINT ( 'NONE',  ( -6.972266317189433020E-16, -49.12499999726880162, -5.000000000000000000 ) ) ;
#35124=CARTESIAN_POINT ( 'NONE',  ( 0.000000000000000000, -120.0000000000000000, 0.000000000000000000 ) ) ;
#35125=CARTESIAN_POINT ( 'NONE',  ( 4.458734124999999437, -30.06249999863440436, -5.460374474430324690E-16 ) ) ;
#35134=DIRECTION ( 'NONE',  ( 0.000000000000000000, -1.000000000000000000, 0.000000000000000000 ) ) ;
#35135=VERTEX_POINT ( 'NONE', #44769 ) ;
#35136=CARTESIAN_POINT ( 'NONE',  ( -4.458734124999999437, -74.56249999863440792, 0.000000000000000000 ) ) ;
#35142=CARTESIAN_POINT ( 'NONE',  ( 2.229367062499998831, -4.895833331967740065, -3.861377020970580887 ) ) ;
#35143=VERTEX_POINT ( 'NONE', #39940 ) ;
#35150=CARTESIAN_POINT ( 'NONE',  ( 5.000000000000000000, -109.4999999999999858, -6.123233995736766282E-16 ) ) ;
#35152=CARTESIAN_POINT ( 'NONE',  ( -4.458734124999997661, -79.22916666530106511, 2.574251347313722516 ) ) ;
#35154=CARTESIAN_POINT ( 'NONE',  ( 4.458734124999999437, 2.187500001365593416, -5.460374474430324690E-16 ) ) ;
#35155=DIRECTION ( 'NONE',  ( 0.000000000000000000, 0.000000000000000000, 1.000000000000000000 ) ) ;
#35157=CARTESIAN_POINT ( 'NONE',  ( -3.152548672688508926E-16, -67.81249999863440792, -5.148502694627439702 ) ) ;
#35158=CARTESIAN_POINT ( 'NONE',  ( 1.060575238724906964E-15, -25.62499999726881583, 5.773502691896257311 ) ) ;
#35160=CARTESIAN_POINT ( 'NONE',  ( 4.458734125000000326, 29.10416666803226349, 2.574251347313718519 ) ) ;
#35161=CARTESIAN_POINT ( 'NONE',  ( 2.500000000000002220, -110.5416666639354730, 4.330127018922192761 ) ) ;
#35162=CARTESIAN_POINT ( 'NONE',  ( -6.972266317189433020E-16, 25.74999999999999645, -5.000000000000000000 ) ) ;
#35163=CARTESIAN_POINT ( 'NONE',  ( -4.458734124999999437, -47.31249999863440792, 0.000000000000000000 ) ) ;
#35164=CARTESIAN_POINT ( 'NONE',  ( -2.229367062500000163, -29.72916666530107221, -3.861377020970580443 ) ) ;
#35168=CARTESIAN_POINT ( 'NONE',  ( 5.000000000000000000, 22.58333333333333570, -2.886751345948129988 ) ) ;
#35171=CARTESIAN_POINT ( 'NONE',  ( 2.229367062499998831, -38.64583333196773651, -3.861377020970580887 ) ) ;
#35172=CARTESIAN_POINT ( 'NONE',  ( -5.000000000000000000, -71.95833333060214443, -2.886751345948128211 ) ) ;
#35176=CARTESIAN_POINT ( 'NONE',  ( -2.229367062499996610, -79.39583333196773651, 3.861377020970582219 ) ) ;
#35178=CARTESIAN_POINT ( 'NONE',  ( 5.000000000000000000, 18.62500000273118772, -6.123233995736766282E-16 ) ) ;
#35179=LINE ( 'NONE', #50281, #21545 ) ;
#35180=CARTESIAN_POINT ( 'NONE',  ( 2.500000000000002220, -29.66666666666666785, 4.330127018922192761 ) ) ;
#35186=CARTESIAN_POINT ( 'NONE',  ( -2.499999999999996447, 19.29166666939785202, 4.330127018922195425 ) ) ;
#35191=CARTESIAN_POINT ( 'NONE',  ( -5.000000000000000000, 3.916666666666665630, -2.886751345948128211 ) ) ;
#35192=CARTESIAN_POINT ( 'NONE',  ( -6.972266317189433020E-16, -44.12499999726880162, -5.000000000000000000 ) ) ;
#35194=CARTESIAN_POINT ( 'NONE',  ( 5.000000000000000000, 28.62500000273118417, -6.123233995736766282E-16 ) ) ;
#35197=CARTESIAN_POINT ( 'NONE',  ( -1.339745962155610925, -78.79465819873851729, 5.000000000000000000 ) ) ;
#35198=CARTESIAN_POINT ( 'NONE',  ( -2.229367062499996610, -22.14583333196773651, 3.861377020970582219 ) ) ;
#35206=CARTESIAN_POINT ( 'NONE',  ( 2.499999999999998668, -21.33333333333333570, -4.330127018922193649 ) ) ;
#35213=EDGE_LOOP ( 'NONE', ( #20732, #45954, #53717, #50700 ) ) ;
#35215=CARTESIAN_POINT ( 'NONE',  ( 4.458734124999999437, 16.18750000136559564, -5.460374474430324690E-16 ) ) ;
#35220=DIRECTION ( 'NONE',  ( -0.000000000000000000, 1.000000000000000000, -0.000000000000000000 ) ) ;
#35221=CARTESIAN_POINT ( 'NONE',  ( 4.458734125000000326, -67.89583333196773651, 2.574251347313718519 ) ) ;
#35222=DIRECTION ( 'NONE',  ( -0.000000000000000000, 1.000000000000000000, -0.000000000000000000 ) ) ;
#35223=CARTESIAN_POINT ( 'NONE',  ( -4.458734124999999437, 20.60416666803225993, -2.574251347313719407 ) ) ;
#35226=CARTESIAN_POINT ( 'NONE',  ( -4.458734124999999437, -47.56249999863440792, 0.000000000000000000 ) ) ;
#35227=CARTESIAN_POINT ( 'NONE',  ( -5.000000000000000000, -9.874999997268815832, 0.000000000000000000 ) ) ;
#35229=CARTESIAN_POINT ( 'NONE',  ( -5.000000000000000000, -65.95833333060213022, -2.886751345948128211 ) ) ;
#35231=LINE ( 'NONE', #1159, #4905 ) ;
#35232=CARTESIAN_POINT ( 'NONE',  ( -4.458734124999997661, -17.47916666530106866, 2.574251347313722516 ) ) ;
#35234=CARTESIAN_POINT ( 'NONE',  ( -2.500000000000000444, -47.04166666393547303, -4.330127018922193649 ) ) ;
#35235=CARTESIAN_POINT ( 'NONE',  ( 9.457646018065525792E-16, -103.0624999986344221, 5.148502694627439702 ) ) ;
#35237=ORIENTED_EDGE ( 'NONE', *, *, #24754, .T. ) ;
#35238=CARTESIAN_POINT ( 'NONE',  ( 4.458734124999998549, -98.97916666530105090, -2.574251347313721627 ) ) ;
#35240=CARTESIAN_POINT ( 'NONE',  ( 5.000000000000000000, -55.29166666393548013, -2.886751345948129988 ) ) ;
#35241=CARTESIAN_POINT ( 'NONE',  ( -6.972266317189433020E-16, 18.87500000273119127, -5.000000000000000000 ) ) ;
#35244=CARTESIAN_POINT ( 'NONE',  ( -3.152548672688508926E-16, -21.56249999863440792, -5.148502694627439702 ) ) ;
#35245=CARTESIAN_POINT ( 'NONE',  ( 2.229367062500001939, 5.770833334698927786, 3.861377020970579999 ) ) ;
#35246=CARTESIAN_POINT ( 'NONE',  ( 4.458734124999998549, -62.97916666530106511, -2.574251347313721627 ) ) ;
#35250=CARTESIAN_POINT ( 'NONE',  ( 5.000000000000000000, -13.49999999999999822, -6.123233995736766282E-16 ) ) ;
#35252=ORIENTED_EDGE ( 'NONE', *, *, #56601, .T. ) ;
#35254=CARTESIAN_POINT ( 'NONE',  ( 5.000000000000000000, 21.62500000273118417, -6.123233995736766282E-16 ) ) ;
#35255=CARTESIAN_POINT ( 'NONE',  ( 5.000000000000000888, -38.45833333060213732, 2.886751345948126879 ) ) ;
#35258=DIRECTION ( 'NONE',  ( -0.000000000000000000, 1.000000000000000000, -0.000000000000000000 ) ) ;
#35262=CARTESIAN_POINT ( 'NONE',  ( -2.499999999999996447, -76.83333333333334281, 4.330127018922195425 ) ) ;
#35264=ORIENTED_EDGE ( 'NONE', *, *, #20959, .T. ) ;
#35265=CARTESIAN_POINT ( 'NONE',  ( 0.000000000000000000, -120.0000000000000000, 5.000000000000000000 ) ) ;
#35266=ORIENTED_EDGE ( 'NONE', *, *, #36996, .F. ) ;
#35267=LINE ( 'NONE', #15965, #24515 ) ;
#35271=ORIENTED_EDGE ( 'NONE', *, *, #15773, .F. ) ;
#35273=ORIENTED_EDGE ( 'NONE', *, *, #4031, .F. ) ;
#35276=CARTESIAN_POINT ( 'NONE',  ( 4.458734125000001214, -62.14583333196774362, 2.574251347313718519 ) ) ;
#35284=ORIENTED_EDGE ( 'NONE', *, *, #47992, .F. ) ;
#35288=CARTESIAN_POINT ( 'NONE',  ( -2.229367062499996610, 27.85416666803225993, 3.861377020970582219 ) ) ;
#35294=CARTESIAN_POINT ( 'NONE',  ( 4.458734124999999437, -43.81249999863440081, -5.460374474430324690E-16 ) ) ;
#35297=CARTESIAN_POINT ( 'NONE',  ( 9.457646018065525792E-16, -49.06249999863440792, 5.148502694627439702 ) ) ;
#35298=CARTESIAN_POINT ( 'NONE',  ( -1.975475456537005874E-15, 29.25000000000000000, 5.000000000000000000 ) ) ;
#35299=CARTESIAN_POINT ( 'NONE',  ( -3.152548672688508926E-16, -16.56249999863440792, -5.148502694627439702 ) ) ;
#35300=CARTESIAN_POINT ( 'NONE',  ( 5.000000000000000000, -102.5000000000000142, -6.123233995736766282E-16 ) ) ;
#35301=EDGE_CURVE ( 'NONE', #8786, #15905, #60849, .T. ) ;
#35303=CARTESIAN_POINT ( 'NONE',  ( -2.229367062499996610, -31.39583333196773651, 3.861377020970582219 ) ) ;
#35305=CARTESIAN_POINT ( 'NONE',  ( -2.499999999999996447, 5.291666669397853795, 4.330127018922195425 ) ) ;
#35306=DIRECTION ( 'NONE',  ( 1.000000000000000000, 0.000000000000000000, -0.000000000000000000 ) ) ;
#35309=DIRECTION ( 'NONE',  ( -0.000000000000000000, 1.000000000000000000, -0.000000000000000000 ) ) ;
#35310=CARTESIAN_POINT ( 'NONE',  ( 0.000000000000000000, -120.0000000000000000, 5.000000000000000000 ) ) ;
#35312=CARTESIAN_POINT ( 'NONE',  ( 4.458734124999999437, 0.9375000013655959696, -5.460374474430324690E-16 ) ) ;
#35314=CARTESIAN_POINT ( 'NONE',  ( 1.339745962155615144, 16.41965820146970501, 4.999999999999999112 ) ) ;
#35316=CARTESIAN_POINT ( 'NONE',  ( -4.458734124999999437, -90.31249999863440792, 0.000000000000000000 ) ) ;
#35317=CARTESIAN_POINT ( 'NONE',  ( 4.458734124999998549, -32.72916666530107221, -2.574251347313721627 ) ) ;
#35318=CARTESIAN_POINT ( 'NONE',  ( -5.000000000000000000, -36.00000000000000711, 0.000000000000000000 ) ) ;
#35319=CARTESIAN_POINT ( 'NONE',  ( -4.458734124999999437, -82.56249999863440792, 0.000000000000000000 ) ) ;
#35322=CARTESIAN_POINT ( 'NONE',  ( -4.458734124999997661, -2.229166665301068662, 2.574251347313722516 ) ) ;
#35323=CARTESIAN_POINT ( 'NONE',  ( -2.229367062499996610, 21.60416666803226349, 3.861377020970582219 ) ) ;
#35324=CARTESIAN_POINT ( 'NONE',  ( -4.458734124999997661, -46.47916666530106511, 2.574251347313722516 ) ) ;
#35325=CARTESIAN_POINT ( 'NONE',  ( 2.499999999999998668, -11.33333333333333393, -4.330127018922193649 ) ) ;
#35328=EDGE_LOOP ( 'NONE', ( #26012, #20179, #57308, #56103 ) ) ;
#35331=CARTESIAN_POINT ( 'NONE',  ( 2.229367062500001939, -72.97916666530107932, 3.861377020970579999 ) ) ;
#35332=CARTESIAN_POINT ( 'NONE',  ( -5.000000000000000000, -109.8749999972688016, 0.000000000000000000 ) ) ;
#35335=ADVANCED_FACE ( 'NONE', ( #30936 ), #15189, .T. ) ;
#35338=CARTESIAN_POINT ( 'NONE',  ( 2.500000000000002220, -59.66666666666665719, 4.330127018922192761 ) ) ;
#35339=CARTESIAN_POINT ( 'NONE',  ( 2.499999999999998668, -90.20833333060214443, -4.330127018922193649 ) ) ;
#35341=VERTEX_POINT ( 'NONE', #54103 ) ;
#35350=ORIENTED_EDGE ( 'NONE', *, *, #40797, .F. ) ;
#35351=CARTESIAN_POINT ( 'NONE',  ( 1.339745962155615144, -59.58034179853028434, 4.999999999999999112 ) ) ;
#35357=CARTESIAN_POINT ( 'NONE',  ( -2.229367062499996610, -47.39583333196774362, 3.861377020970582219 ) ) ;
#35363=AXIS2_PLACEMENT_3D ( 'NONE', #50952, #12970, #7215 ) ;
#35366=CARTESIAN_POINT ( 'NONE',  ( 4.458734124999998549, -93.97916666530106511, -2.574251347313721627 ) ) ;
#35369=CARTESIAN_POINT ( 'NONE',  ( 2.500000000000002220, -19.54166666393548013, 4.330127018922192761 ) ) ;
#35375=CARTESIAN_POINT ( 'NONE',  ( 4.458734124999998549, -3.729166665301070438, -2.574251347313721627 ) ) ;
#35376=CARTESIAN_POINT ( 'NONE',  ( 1.339745962155612702, -1.169658196007335338, -5.000000000000000000 ) ) ;
#35377=CARTESIAN_POINT ( 'NONE',  ( -4.458734124999999437, -18.56249999863440792, 0.000000000000000000 ) ) ;
#35378=EDGE_CURVE ( 'NONE', #19379, #52091, #40274, .T. ) ;
#35381=ADVANCED_FACE ( 'NONE', ( #7461 ), #17734, .T. ) ;
#35382=CARTESIAN_POINT ( 'NONE',  ( -5.000000000000000000, -73.95833333060214443, -2.886751345948128211 ) ) ;
#35384=( BOUNDED_CURVE ( )  B_SPLINE_CURVE ( 2, ( #61709, #19750, #34527, #37563, #47834, #62022, #17638, #58676, #37255 ),
 .UNSPECIFIED., .F., .F. ) 
 B_SPLINE_CURVE_WITH_KNOTS ( ( 3, 2, 2, 2, 3 ),
 ( 0.1767857142857142960, 0.1773809523809523891, 0.1785714285714285754, 0.1797619047619047616, 0.1803571428571428548 ),
 .UNSPECIFIED. ) 
 CURVE ( )  GEOMETRIC_REPRESENTATION_ITEM ( )  RATIONAL_B_SPLINE_CURVE ( ( 0.9330127018922194093, 0.9330127018922194093, 1.000000000000000000, 0.8660254037844387076, 1.000000000000000000, 0.8660254037844387076, 1.000000000000000000, 0.9330127018922194093, 0.9330127018922194093 ) ) 
 REPRESENTATION_ITEM ( '' )  );
#35385=CARTESIAN_POINT ( 'NONE',  ( 2.229367062500001939, 13.77083333469892779, 3.861377020970579999 ) ) ;
#35387=CARTESIAN_POINT ( 'NONE',  ( -6.972266317189433020E-16, -19.12499999726880873, -5.000000000000000000 ) ) ;
#35388=CARTESIAN_POINT ( 'NONE',  ( 1.975475456537005874E-15, -3.750000000000001776, 5.000000000000000000 ) ) ;
#35389=CARTESIAN_POINT ( 'NONE',  ( 9.457646018065525792E-16, -17.06249999863440792, 5.148502694627439702 ) ) ;
#35391=LINE ( 'NONE', #5802, #21177 ) ;
#35393=CARTESIAN_POINT ( 'NONE',  ( -4.999999999999999112, -45.79166666393547303, 2.886751345948131764 ) ) ;
#35395=CARTESIAN_POINT ( 'NONE',  ( 9.457646018065525792E-16, 15.93750000136559564, 5.148502694627439702 ) ) ;
#35399=CARTESIAN_POINT ( 'NONE',  ( -4.458734124999999437, -66.39583333196773651, -2.574251347313719407 ) ) ;
#35402=CARTESIAN_POINT ( 'NONE',  ( 5.000000000000000000, 3.499999999999999556, -6.123233995736766282E-16 ) ) ;
#35405=CARTESIAN_POINT ( 'NONE',  ( 4.458734125000001214, -57.89583333196773651, 2.574251347313718519 ) ) ;
#35406=CARTESIAN_POINT ( 'NONE',  ( 1.060575238724906964E-15, -92.62499999726881583, 5.773502691896257311 ) ) ;
#35408=CARTESIAN_POINT ( 'NONE',  ( 2.229367062499998831, -32.64583333196773651, -3.861377020970580887 ) ) ;
#35412=CARTESIAN_POINT ( 'NONE',  ( -2.500000000000000444, -79.04166666393547303, -4.330127018922193649 ) ) ;
#35414=CARTESIAN_POINT ( 'NONE',  ( -5.000000000000000000, -44.08333333333334281, -2.886751345948128211 ) ) ;
#35416=CARTESIAN_POINT ( 'NONE',  ( 5.000000000000000000, -6.291666663935481019, -2.886751345948130876 ) ) ;
#35418=CARTESIAN_POINT ( 'NONE',  ( 4.458734125000001214, -106.8958333319677649, 2.574251347313718519 ) ) ;
#35419=CARTESIAN_POINT ( 'NONE',  ( -4.458734124999999437, 0.3541666680322609340, -2.574251347313719407 ) ) ;
#35423=CARTESIAN_POINT ( 'NONE',  ( -1.339745962155669101, -25.79465819873852084, 4.999999999999966249 ) ) ;
#35428=CARTESIAN_POINT ( 'NONE',  ( 2.499999999999998668, -81.33333333333332860, -4.330127018922193649 ) ) ;
#35432=CARTESIAN_POINT ( 'NONE',  ( -4.458734124999999437, -31.64583333196773651, -2.574251347313719407 ) ) ;
#35440=EDGE_CURVE ( 'NONE', #35972, #35143, #1691, .T. ) ;
#35441=DIRECTION ( 'NONE',  ( 0.000000000000000000, 0.000000000000000000, 1.000000000000000000 ) ) ;
#35442=ORIENTED_EDGE ( 'NONE', *, *, #4022, .T. ) ;
#35443=CARTESIAN_POINT ( 'NONE',  ( -4.458734124999999437, -76.56249999863440792, 0.000000000000000000 ) ) ;
#35444=FACE_OUTER_BOUND ( 'NONE', #52988, .T. ) ;
#35446=ORIENTED_EDGE ( 'NONE', *, *, #18517, .F. ) ;
#35450=ADVANCED_FACE ( 'NONE', ( #47008 ), #40899, .T. ) ;
#35451=CARTESIAN_POINT ( 'NONE',  ( 2.229367062500001939, -1.229166665301071548, 3.861377020970579999 ) ) ;
#35456=CARTESIAN_POINT ( 'NONE',  ( -4.729367062499999719, -110.1562499993171969, 0.000000000000000000 ) ) ;
#35463=CARTESIAN_POINT ( 'NONE',  ( -6.972266317189433020E-16, -75.12499999726880162, -5.000000000000000000 ) ) ;
#35466=CARTESIAN_POINT ( 'NONE',  ( 2.229367062500001939, -81.97916666530106511, 3.861377020970579999 ) ) ;
#35468=CARTESIAN_POINT ( 'NONE',  ( 1.975475456537005874E-15, -29.62499999726881228, 5.000000000000000000 ) ) ;
#35469=CARTESIAN_POINT ( 'NONE',  ( 2.229367062499998831, -2.645833331967738289, -3.861377020970580887 ) ) ;
#35471=( BOUNDED_CURVE ( )  B_SPLINE_CURVE ( 2, ( #4209, #52779, #57304, #23821, #47626, #19297, #33466, #8708, #23512 ),
 .UNSPECIFIED., .F., .F. ) 
 B_SPLINE_CURVE_WITH_KNOTS ( ( 3, 2, 2, 2, 3 ),
 ( 0.9625000000000000222, 0.9630952380952381153, 0.9642857142857143016, 0.9654761904761904878, 0.9660714285714285809 ),
 .UNSPECIFIED. ) 
 CURVE ( )  GEOMETRIC_REPRESENTATION_ITEM ( )  RATIONAL_B_SPLINE_CURVE ( ( 0.9330127018922194093, 0.9330127018922194093, 1.000000000000000000, 0.8660254037844387076, 1.000000000000000000, 0.8660254037844387076, 1.000000000000000000, 0.9330127018922194093, 0.9330127018922194093 ) ) 
 REPRESENTATION_ITEM ( '' )  );
#35472=CARTESIAN_POINT ( 'NONE',  ( 1.975475456537005874E-15, 1.250000000000000000, 5.000000000000000000 ) ) ;
#35473=CARTESIAN_POINT ( 'NONE',  ( 9.457646018065525792E-16, -69.31249999863440792, 5.148502694627439702 ) ) ;
#35474=CARTESIAN_POINT ( 'NONE',  ( -2.500000000000000444, -30.04166666393548013, -4.330127018922193649 ) ) ;
#35475=CARTESIAN_POINT ( 'NONE',  ( -2.500000000000000444, -15.16666666666666785, -4.330127018922193649 ) ) ;
#35476=CARTESIAN_POINT ( 'NONE',  ( 4.458734124999999437, 28.18750000136559208, -5.460374474430324690E-16 ) ) ;
#35479=CARTESIAN_POINT ( 'NONE',  ( 4.458734124999999437, -52.81249999863440792, -5.460374474430324690E-16 ) ) ;
#35480=CARTESIAN_POINT ( 'NONE',  ( -4.458734124999999437, -34.56249999863440792, 0.000000000000000000 ) ) ;
#35483=CARTESIAN_POINT ( 'NONE',  ( -2.499999999999996447, 23.16666666666666430, 4.330127018922195425 ) ) ;
#35485=DIRECTION ( 'NONE',  ( -0.000000000000000000, -1.000000000000000000, -0.000000000000000000 ) ) ;
#35486=CARTESIAN_POINT ( 'NONE',  ( -2.229367062499996610, -44.14583333196774362, 3.861377020970582219 ) ) ;
#35487=CARTESIAN_POINT ( 'NONE',  ( -3.535250795749689387E-16, -71.12499999726880162, -5.773502691896257311 ) ) ;
#35489=DIRECTION ( 'NONE',  ( -0.000000000000000000, 1.000000000000000000, -0.000000000000000000 ) ) ;
#35491=CARTESIAN_POINT ( 'NONE',  ( -3.152548672688508926E-16, -79.81249999863440792, -5.148502694627439702 ) ) ;
#35493=CARTESIAN_POINT ( 'NONE',  ( 0.000000000000000000, -114.9999999999999858, 0.000000000000000000 ) ) ;
#35495=CARTESIAN_POINT ( 'NONE',  ( 5.000000000000000000, -29.50000000000000000, -6.123233995736766282E-16 ) ) ;
#35501=CARTESIAN_POINT ( 'NONE',  ( -3.535250795749689387E-16, 22.87500000273118772, -5.773502691896257311 ) ) ;
#35507=CARTESIAN_POINT ( 'NONE',  ( 1.339745962155612702, -99.16965819600733312, -5.000000000000000000 ) ) ;
#35511=CARTESIAN_POINT ( 'NONE',  ( 2.229367062500001939, -16.22916666530107577, 3.861377020970579999 ) ) ;
#35512=CARTESIAN_POINT ( 'NONE',  ( 1.339745962155627135, 17.83034180399266333, -4.999999999999991118 ) ) ;
#35518=CARTESIAN_POINT ( 'NONE',  ( -1.339745962155613812, 24.91965820146970501, -5.000000000000000000 ) ) ;
#35520=ORIENTED_EDGE ( 'NONE', *, *, #33419, .T. ) ;
#35522=LINE ( 'NONE', #1767, #8053 ) ;
#35524=ORIENTED_EDGE ( 'NONE', *, *, #57129, .T. ) ;
#35525=AXIS2_PLACEMENT_3D ( 'NONE', #8113, #22913, #27398 ) ;
#35531=CARTESIAN_POINT ( 'NONE',  ( 1.975475456537005874E-15, 11.24999999999999822, 5.000000000000000000 ) ) ;
#35532=CARTESIAN_POINT ( 'NONE',  ( 2.229367062500001939, 14.02083333469892779, 3.861377020970579999 ) ) ;
#35533=EDGE_CURVE ( 'NONE', #22435, #9796, #46685, .T. ) ;
#35536=CARTESIAN_POINT ( 'NONE',  ( 5.000000000000000000, -44.50000000000000000, -6.123233995736766282E-16 ) ) ;
#35538=( BOUNDED_CURVE ( )  B_SPLINE_CURVE ( 2, ( #20036, #19396, #24546, #63162, #121, #39641, #29675, #5246, #53187 ),
 .UNSPECIFIED., .F., .F. ) 
 B_SPLINE_CURVE_WITH_KNOTS ( ( 3, 2, 2, 2, 3 ),
 ( 0.6696428571428570953, 0.6702380952380951884, 0.6714285714285713746, 0.6726190476190476719, 0.6732142857142857650 ),
 .UNSPECIFIED. ) 
 CURVE ( )  GEOMETRIC_REPRESENTATION_ITEM ( )  RATIONAL_B_SPLINE_CURVE ( ( 0.9330127018922194093, 0.9330127018922194093, 1.000000000000000000, 0.8660254037844387076, 1.000000000000000000, 0.8660254037844387076, 1.000000000000000000, 0.9330127018922194093, 0.9330127018922194093 ) ) 
 REPRESENTATION_ITEM ( '' )  );
#35539=CARTESIAN_POINT ( 'NONE',  ( 4.458734125000000326, -62.89583333196774362, 2.574251347313718519 ) ) ;
#35540=CARTESIAN_POINT ( 'NONE',  ( 0.000000000000000000, -120.0000000000000000, 5.000000000000000000 ) ) ;
#35541=CARTESIAN_POINT ( 'NONE',  ( -4.458734124999998549, 10.77083333469892956, 2.574251347313722516 ) ) ;
#35546=CARTESIAN_POINT ( 'NONE',  ( -4.458734124999999437, -55.56249999863440081, 0.000000000000000000 ) ) ;
#35547=CARTESIAN_POINT ( 'NONE',  ( -2.500000000000000444, -9.041666663935483683, -4.330127018922193649 ) ) ;
#35548=CARTESIAN_POINT ( 'NONE',  ( -1.339745962155610925, -108.7946581987385315, 5.000000000000000000 ) ) ;
#35551=CARTESIAN_POINT ( 'NONE',  ( 5.000000000000000000, -104.3749999972688158, -6.123233995736766282E-16 ) ) ;
#35552=CARTESIAN_POINT ( 'NONE',  ( 2.229367062499998831, -18.89583333196774007, -3.861377020970580887 ) ) ;
#35555=CARTESIAN_POINT ( 'NONE',  ( -2.229367062500000163, -105.4791666653010651, -3.861377020970580443 ) ) ;
#35558=CARTESIAN_POINT ( 'NONE',  ( 2.229367062499998831, -98.89583333196773651, -3.861377020970580887 ) ) ;
#35559=CARTESIAN_POINT ( 'NONE',  ( 2.229367062500001939, -25.97916666530106866, 3.861377020970579999 ) ) ;
#35560=CARTESIAN_POINT ( 'NONE',  ( -3.535250795749689387E-16, -56.12499999726880162, -5.773502691896257311 ) ) ;
#35564=CARTESIAN_POINT ( 'NONE',  ( 4.458734124999999437, -21.81249999863440436, -5.460374474430324690E-16 ) ) ;
#35565=CARTESIAN_POINT ( 'NONE',  ( 4.458734124999998549, -63.97916666530106511, -2.574251347313721627 ) ) ;
#35566=CARTESIAN_POINT ( 'NONE',  ( 5.000000000000000888, -94.45833333060211601, 2.886751345948126879 ) ) ;
#35570=CARTESIAN_POINT ( 'NONE',  ( 2.499999999999998668, -9.333333333333332149, -4.330127018922193649 ) ) ;
#35572=ORIENTED_EDGE ( 'NONE', *, *, #16560, .F. ) ;
#35575=CARTESIAN_POINT ( 'NONE',  ( -4.999999999999998224, -37.91666666666667851, 2.886751345948131764 ) ) ;
#35576=CARTESIAN_POINT ( 'NONE',  ( 1.339745962155729053, -90.29465819873854571, -4.999999999999933387 ) ) ;
#35579=CARTESIAN_POINT ( 'NONE',  ( 5.000000000000000000, 1.708333336064519425, -2.886751345948130876 ) ) ;
#35583=CARTESIAN_POINT ( 'NONE',  ( -5.000000000000000000, -76.00000000000000000, 0.000000000000000000 ) ) ;
#35586=CARTESIAN_POINT ( 'NONE',  ( 2.499999999999998668, -80.20833333060213022, -4.330127018922193649 ) ) ;
#35588=AXIS2_PLACEMENT_3D ( 'NONE', #62574, #18494, #62877 ) ;
#35589=CARTESIAN_POINT ( 'NONE',  ( 1.339745962155615144, -85.70534180126146850, 4.999999999999999112 ) ) ;
#35597=VERTEX_POINT ( 'NONE', #38299 ) ;
#35601=CARTESIAN_POINT ( 'NONE',  ( 1.975475456537005874E-15, -0.7499999999999996669, 5.000000000000000000 ) ) ;
#35602=ORIENTED_EDGE ( 'NONE', *, *, #23969, .F. ) ;
#35605=DIRECTION ( 'NONE',  ( -0.000000000000000000, 1.000000000000000000, -0.000000000000000000 ) ) ;
#35606=VERTEX_POINT ( 'NONE', #43113 ) ;
#35607=CARTESIAN_POINT ( 'NONE',  ( 4.458734125000001214, -78.89583333196772230, 2.574251347313718519 ) ) ;
#35608=CARTESIAN_POINT ( 'NONE',  ( -4.458734124999999437, -108.5624999986343937, 0.000000000000000000 ) ) ;
#35609=CARTESIAN_POINT ( 'NONE',  ( 2.499999999999998668, 20.66666666666666785, -4.330127018922193649 ) ) ;
#35615=CARTESIAN_POINT ( 'NONE',  ( 4.458734125000000326, -43.89583333196773651, 2.574251347313718519 ) ) ;
#35617=DIRECTION ( 'NONE',  ( 0.000000000000000000, 0.000000000000000000, 1.000000000000000000 ) ) ;
#35618=CARTESIAN_POINT ( 'NONE',  ( 2.229367062500001939, -50.97916666530107221, 3.861377020970579999 ) ) ;
#35620=CARTESIAN_POINT ( 'NONE',  ( 5.000000000000000000, 29.58333333333332860, -2.886751345948130876 ) ) ;
#35621=CARTESIAN_POINT ( 'NONE',  ( -2.229367062500000163, -18.47916666530106866, -3.861377020970580443 ) ) ;
#35622=CARTESIAN_POINT ( 'NONE',  ( -3.535250795749689387E-16, -101.2500000000000000, -5.773502691896257311 ) ) ;
#35624=CARTESIAN_POINT ( 'NONE',  ( -2.229367062499996610, -35.39583333196772941, 3.861377020970582219 ) ) ;
#35625=CARTESIAN_POINT ( 'NONE',  ( 5.000000000000000000, 5.625000002731185056, -6.123233995736766282E-16 ) ) ;
#35626=CARTESIAN_POINT ( 'NONE',  ( 1.339745962155612702, -50.29465819873851729, -5.000000000000000000 ) ) ;
#35631=CARTESIAN_POINT ( 'NONE',  ( 4.458734125000000326, 0.8541666680322613781, 2.574251347313718519 ) ) ;
#35632=EDGE_LOOP ( 'NONE', ( #18301, #31895, #42154, #44291 ) ) ;
#35633=VECTOR ( 'NONE', #39625, 1000.000000000000000 ) ;
#35634=CARTESIAN_POINT ( 'NONE',  ( 3.044556291839386294E-14, 16.87500000273118417, -5.000000000000000000 ) ) ;
#35636=CARTESIAN_POINT ( 'NONE',  ( -2.229367062499996610, -89.14583333196773651, 3.861377020970582219 ) ) ;
#35637=CARTESIAN_POINT ( 'NONE',  ( 2.229367062500001939, -35.97916666530107221, 3.861377020970579999 ) ) ;
#35638=CARTESIAN_POINT ( 'NONE',  ( 0.000000000000000000, -120.0000000000000000, 0.000000000000000000 ) ) ;
#35639=CARTESIAN_POINT ( 'NONE',  ( 2.229367062500001939, -83.22916666530106511, 3.861377020970579999 ) ) ;
#35642=CARTESIAN_POINT ( 'NONE',  ( 0.000000000000000000, -120.0000000000000000, 0.000000000000000000 ) ) ;
#35645=CARTESIAN_POINT ( 'NONE',  ( -2.229367062500000163, -9.479166665301068662, -3.861377020970580443 ) ) ;
#35646=CARTESIAN_POINT ( 'NONE',  ( 9.457646018065525792E-16, 19.68750000136559208, 5.148502694627439702 ) ) ;
#35647=CARTESIAN_POINT ( 'NONE',  ( 4.458734124999999437, -48.06249999863440792, -5.460374474430324690E-16 ) ) ;
#35651=CARTESIAN_POINT ( 'NONE',  ( 0.000000000000000000, -120.0000000000000000, 0.000000000000000000 ) ) ;
#35652=ORIENTED_EDGE ( 'NONE', *, *, #61301, .F. ) ;
#35655=CARTESIAN_POINT ( 'NONE',  ( -3.152548672688508926E-16, -73.56249999863440792, -5.148502694627439702 ) ) ;
#35656=CARTESIAN_POINT ( 'NONE',  ( -2.229367062500000163, 29.27083333469892779, -3.861377020970580443 ) ) ;
#35658=( BOUNDED_CURVE ( )  B_SPLINE_CURVE ( 2, ( #51849, #42190, #52166, #7791, #21395, #22909, #52492, #42503, #12607 ),
 .UNSPECIFIED., .F., .F. ) 
 B_SPLINE_CURVE_WITH_KNOTS ( ( 3, 2, 2, 2, 3 ),
 ( 0.5589285714285714413, 0.5595238095238095344, 0.5607142857142857206, 0.5619047619047619069, 0.5625000000000000000 ),
 .UNSPECIFIED. ) 
 CURVE ( )  GEOMETRIC_REPRESENTATION_ITEM ( )  RATIONAL_B_SPLINE_CURVE ( ( 0.9330127018922194093, 0.9330127018922194093, 1.000000000000000000, 0.8660254037844387076, 1.000000000000000000, 0.8660254037844387076, 1.000000000000000000, 0.9330127018922194093, 0.9330127018922194093 ) ) 
 REPRESENTATION_ITEM ( '' )  );
#35660=CARTESIAN_POINT ( 'NONE',  ( -6.972266317189433020E-16, -65.24999999999998579, -5.000000000000000000 ) ) ;
#35663=CARTESIAN_POINT ( 'NONE',  ( 5.000000000000000000, -60.41666666666666430, -2.886751345948129988 ) ) ;
#35664=CARTESIAN_POINT ( 'NONE',  ( -2.500000000000000444, -75.16666666666665719, -4.330127018922193649 ) ) ;
#35668=CARTESIAN_POINT ( 'NONE',  ( 2.500000000000002220, -52.54166666393548013, 4.330127018922192761 ) ) ;
#35669=CARTESIAN_POINT ( 'NONE',  ( 1.975475456537005874E-15, -106.6249999972687874, 5.000000000000000000 ) ) ;
#35673=( BOUNDED_CURVE ( )  B_SPLINE_CURVE ( 2, ( #15377, #5407, #1555, #16010, #21157, #59447, #55263, #60410, #44634 ),
 .UNSPECIFIED., .F., .F. ) 
 B_SPLINE_CURVE_WITH_KNOTS ( ( 3, 2, 2, 2, 3 ),
 ( 0.6232142857142857206, 0.6238095238095238138, 0.6250000000000000000, 0.6261904761904761862, 0.6267857142857142794 ),
 .UNSPECIFIED. ) 
 CURVE ( )  GEOMETRIC_REPRESENTATION_ITEM ( )  RATIONAL_B_SPLINE_CURVE ( ( 0.9330127018922194093, 0.9330127018922194093, 1.000000000000000000, 0.8660254037844387076, 1.000000000000000000, 0.8660254037844387076, 1.000000000000000000, 0.9330127018922194093, 0.9330127018922194093 ) ) 
 REPRESENTATION_ITEM ( '' )  );
#35676=ORIENTED_EDGE ( 'NONE', *, *, #59400, .F. ) ;
#35677=LINE ( 'NONE', #1597, #15062 ) ;
#35679=ORIENTED_EDGE ( 'NONE', *, *, #3084, .F. ) ;
#35683=CARTESIAN_POINT ( 'NONE',  ( -2.229367062500000163, -45.72916666530106511, -3.861377020970580443 ) ) ;
#35685=AXIS2_PLACEMENT_3D ( 'NONE', #27941, #37596, #62059 ) ;
#35687=DIRECTION ( 'NONE',  ( 0.000000000000000000, 0.000000000000000000, 1.000000000000000000 ) ) ;
#35692=CARTESIAN_POINT ( 'NONE',  ( 1.339745962155619807, 22.70534180126147561, -4.999999999999996447 ) ) ;
#35694=CARTESIAN_POINT ( 'NONE',  ( 2.229367062499998831, -96.89583333196773651, -3.861377020970580887 ) ) ;
#35695=CYLINDRICAL_SURFACE ( 'NONE', #24556, 5.000000000000000000 ) ;
#35697=CARTESIAN_POINT ( 'NONE',  ( -1.339745962155610925, 14.33034180399266688, 5.000000000000000000 ) ) ;
#35700=ORIENTED_EDGE ( 'NONE', *, *, #17254, .F. ) ;
#35701=CARTESIAN_POINT ( 'NONE',  ( 4.458734124999998549, -2.729166665301069550, -2.574251347313721627 ) ) ;
#35703=CARTESIAN_POINT ( 'NONE',  ( 2.229367062499998831, -15.89583333196773651, -3.861377020970580887 ) ) ;
#35708=CARTESIAN_POINT ( 'NONE',  ( 2.229367062499998831, 17.10416666803225993, -3.861377020970580887 ) ) ;
#35709=ORIENTED_EDGE ( 'NONE', *, *, #50275, .F. ) ;
#35710=CARTESIAN_POINT ( 'NONE',  ( -2.500000000000000444, -14.04166666393548013, -4.330127018922193649 ) ) ;
#35711=CARTESIAN_POINT ( 'NONE',  ( -4.999999999999998224, -12.91666666666666607, 2.886751345948131764 ) ) ;
#35712=CARTESIAN_POINT ( 'NONE',  ( 4.458734124999999437, -21.81249999863440436, -5.460374474430324690E-16 ) ) ;
#35716=CARTESIAN_POINT ( 'NONE',  ( 2.499999999999998668, -49.20833333060213732, -4.330127018922193649 ) ) ;
#35718=CARTESIAN_POINT ( 'NONE',  ( -4.458734124999999437, 9.687500001365593860, 0.000000000000000000 ) ) ;
#35722=CARTESIAN_POINT ( 'NONE',  ( -2.229367062500000163, -66.47916666530106511, -3.861377020970580443 ) ) ;
#35725=CARTESIAN_POINT ( 'NONE',  ( 2.500000000000002220, 3.333333333333333925, 4.330127018922192761 ) ) ;
#35728=CARTESIAN_POINT ( 'NONE',  ( 4.458734124999999437, -60.81249999863440081, -5.460374474430324690E-16 ) ) ;
#35729=CARTESIAN_POINT ( 'NONE',  ( -5.000000000000000000, -94.87499999726881583, 0.000000000000000000 ) ) ;
#35732=CARTESIAN_POINT ( 'NONE',  ( -6.972266317189433020E-16, -42.12499999726880873, -5.000000000000000000 ) ) ;
#35734=CARTESIAN_POINT ( 'NONE',  ( 5.000000000000000888, 5.541666669397853795, 2.886751345948126879 ) ) ;
#35737=CARTESIAN_POINT ( 'NONE',  ( 1.060575238724906964E-15, -45.75000000000000000, 5.773502691896257311 ) ) ;
#35738=CARTESIAN_POINT ( 'NONE',  ( -6.972266317189433020E-16, -13.25000000000000000, -5.000000000000000000 ) ) ;
#35739=CARTESIAN_POINT ( 'NONE',  ( 2.499999999999998668, -86.20833333060214443, -4.330127018922193649 ) ) ;
#35740=VERTEX_POINT ( 'NONE', #47939 ) ;
#35741=CARTESIAN_POINT ( 'NONE',  ( -4.458734124999999437, -104.3958333319677365, -2.574251347313719407 ) ) ;
#35742=CARTESIAN_POINT ( 'NONE',  ( 4.458734124999999437, -2.062499998634406584, -5.460374474430324690E-16 ) ) ;
#35745=EDGE_CURVE ( 'NONE', #21770, #969, #58549, .T. ) ;
#35749=ORIENTED_EDGE ( 'NONE', *, *, #26466, .T. ) ;
#35750=CARTESIAN_POINT ( 'NONE',  ( 5.000000000000000888, -33.58333333333332860, 2.886751345948126879 ) ) ;
#35751=EDGE_CURVE ( 'NONE', #24823, #58440, #35471, .T. ) ;
#35754=CARTESIAN_POINT ( 'NONE',  ( -2.500000000000000444, -49.04166666393547303, -4.330127018922193649 ) ) ;
#35756=CARTESIAN_POINT ( 'NONE',  ( 4.458734125000001214, -33.14583333196774362, 2.574251347313718519 ) ) ;
#35767=CARTESIAN_POINT ( 'NONE',  ( 2.229367062500001939, -80.22916666530106511, 3.861377020970579999 ) ) ;
#35769=VERTEX_POINT ( 'NONE', #52471 ) ;
#35770=CARTESIAN_POINT ( 'NONE',  ( 0.000000000000000000, -120.0000000000000000, 0.000000000000000000 ) ) ;
#35771=VECTOR ( 'NONE', #35026, 1000.000000000000000 ) ;
#35772=( BOUNDED_CURVE ( )  B_SPLINE_CURVE ( 2, ( #53727, #9658, #19945, #14481, #48264, #49221, #29911, #58241, #24147 ),
 .UNSPECIFIED., .F., .F. ) 
 B_SPLINE_CURVE_WITH_KNOTS ( ( 3, 2, 2, 2, 3 ),
 ( 0.4482142857142857317, 0.4488095238095238249, 0.4500000000000000111, 0.4511904761904761973, 0.4517857142857142905 ),
 .UNSPECIFIED. ) 
 CURVE ( )  GEOMETRIC_REPRESENTATION_ITEM ( )  RATIONAL_B_SPLINE_CURVE ( ( 0.9330127018922194093, 0.9330127018922194093, 1.000000000000000000, 0.8660254037844387076, 1.000000000000000000, 0.8660254037844387076, 1.000000000000000000, 0.9330127018922194093, 0.9330127018922194093 ) ) 
 REPRESENTATION_ITEM ( '' )  );
#35775=CARTESIAN_POINT ( 'NONE',  ( -4.458734124999999437, -1.645833331967737401, -2.574251347313719407 ) ) ;
#35778=CARTESIAN_POINT ( 'NONE',  ( -6.972266317189433020E-16, 2.875000002731185500, -5.000000000000000000 ) ) ;
#35780=EDGE_CURVE ( 'NONE', #14985, #11315, #55204, .T. ) ;
#35781=FACE_OUTER_BOUND ( 'NONE', #31008, .T. ) ;
#35785=CARTESIAN_POINT ( 'NONE',  ( 2.500000000000002220, -75.54166666393547303, 4.330127018922192761 ) ) ;
#35787=CARTESIAN_POINT ( 'NONE',  ( 9.457646018065525792E-16, -79.06249999863440792, 5.148502694627439702 ) ) ;
#35789=CARTESIAN_POINT ( 'NONE',  ( -2.229367062500000163, -4.479166665301070438, -3.861377020970580443 ) ) ;
#35792=CARTESIAN_POINT ( 'NONE',  ( 2.229367062499998831, -72.89583333196773651, -3.861377020970580887 ) ) ;
#35793=CARTESIAN_POINT ( 'NONE',  ( 5.000000000000000000, -29.37499999726881228, -6.123233995736766282E-16 ) ) ;
#35794=CARTESIAN_POINT ( 'NONE',  ( 0.000000000000000000, -120.0000000000000000, 0.000000000000000000 ) ) ;
#35795=CARTESIAN_POINT ( 'NONE',  ( -2.500000000000000444, -1.041666663935479686, -4.330127018922193649 ) ) ;
#35796=CARTESIAN_POINT ( 'NONE',  ( 2.499999999999998668, -104.3333333333333286, -4.330127018922193649 ) ) ;
#35798=CARTESIAN_POINT ( 'NONE',  ( 2.229367062500001939, -49.97916666530107221, 3.861377020970579999 ) ) ;
#35799=CARTESIAN_POINT ( 'NONE',  ( 4.458734124999999437, -34.06249999863440792, -5.460374474430324690E-16 ) ) ;
#35801=CARTESIAN_POINT ( 'NONE',  ( -5.000000000000000000, -18.08333333333333215, -2.886751345948128211 ) ) ;
#35802=CARTESIAN_POINT ( 'NONE',  ( 2.500000000000002220, 20.33333333333333215, 4.330127018922192761 ) ) ;
#35804=CARTESIAN_POINT ( 'NONE',  ( 2.499999999999998668, -26.20833333060214798, -4.330127018922193649 ) ) ;
#35805=CARTESIAN_POINT ( 'NONE',  ( -2.229367062500000163, -43.47916666530106511, -3.861377020970580443 ) ) ;
#35806=CARTESIAN_POINT ( 'NONE',  ( -2.499999999999996447, -80.70833333060213022, 4.330127018922195425 ) ) ;
#35809=ADVANCED_FACE ( 'NONE', ( #33784 ), #47324, .T. ) ;
#35811=EDGE_CURVE ( 'NONE', #14927, #49915, #16121, .T. ) ;
#35812=CARTESIAN_POINT ( 'NONE',  ( -4.458734124999999437, -78.64583333196773651, -2.574251347313719407 ) ) ;
#35815=CARTESIAN_POINT ( 'NONE',  ( 5.000000000000000000, -27.41666666666666785, -2.886751345948129988 ) ) ;
#35821=CARTESIAN_POINT ( 'NONE',  ( 5.000000000000000888, 22.54166666939784847, 2.886751345948126879 ) ) ;
#35829=CARTESIAN_POINT ( 'NONE',  ( 1.975475456537005874E-15, -99.62499999726880162, 5.000000000000000000 ) ) ;
#35831=EDGE_CURVE ( 'NONE', #17008, #50534, #57651, .T. ) ;
#35832=CARTESIAN_POINT ( 'NONE',  ( -1.339745962155610925, -74.66965819600731891, 5.000000000000000000 ) ) ;
#35836=CARTESIAN_POINT ( 'NONE',  ( -3.152548672688508926E-16, -13.81249999863440436, -5.148502694627439702 ) ) ;
#35843=CARTESIAN_POINT ( 'NONE',  ( 5.000000000000000888, 13.41666666666666785, 2.886751345948126879 ) ) ;
#35845=CARTESIAN_POINT ( 'NONE',  ( 2.500000000000002220, -21.66666666666666785, 4.330127018922192761 ) ) ;
#35846=CARTESIAN_POINT ( 'NONE',  ( 5.000000000000000888, -103.5833333333333428, 2.886751345948126879 ) ) ;
#35848=ORIENTED_EDGE ( 'NONE', *, *, #11054, .F. ) ;
#35856=CARTESIAN_POINT ( 'NONE',  ( -3.152548672688508926E-16, 11.43750000136559386, -5.148502694627439702 ) ) ;
#35859=CARTESIAN_POINT ( 'NONE',  ( 5.000000000000000888, -44.58333333333333570, 2.886751345948126879 ) ) ;
#35860=CARTESIAN_POINT ( 'NONE',  ( 1.975475456537005874E-15, -100.7499999999999858, 5.000000000000000000 ) ) ;
#35862=EDGE_LOOP ( 'NONE', ( #37816, #42242, #9099, #32416 ) ) ;
#35863=CARTESIAN_POINT ( 'NONE',  ( -4.458734124999999437, -66.31249999863440792, 0.000000000000000000 ) ) ;
#35865=CARTESIAN_POINT ( 'NONE',  ( -4.458734124999999437, 13.68750000136559386, 0.000000000000000000 ) ) ;
#35866=CARTESIAN_POINT ( 'NONE',  ( -1.339745962155610925, -62.79465819873851729, 5.000000000000000000 ) ) ;
#35867=CARTESIAN_POINT ( 'NONE',  ( 0.000000000000000000, -120.0000000000000000, 0.000000000000000000 ) ) ;
#35868=CARTESIAN_POINT ( 'NONE',  ( -4.458734124999998549, -57.47916666530108643, 2.574251347313722516 ) ) ;
#35869=CARTESIAN_POINT ( 'NONE',  ( 5.000000000000000000, -12.37499999726881050, -6.123233995736766282E-16 ) ) ;
#35872=CARTESIAN_POINT ( 'NONE',  ( 2.499999999999998668, -104.2083333306021444, -4.330127018922193649 ) ) ;
#35873=CARTESIAN_POINT ( 'NONE',  ( 4.458734124999998549, -14.97916666530107399, -2.574251347313721627 ) ) ;
#35876=CARTESIAN_POINT ( 'NONE',  ( 4.458734124999998549, -105.7291666653010651, -2.574251347313721627 ) ) ;
#35879=CARTESIAN_POINT ( 'NONE',  ( -3.152548672688508926E-16, -102.8124999986344221, -5.148502694627439702 ) ) ;
#35880=CARTESIAN_POINT ( 'NONE',  ( -4.458734124999999437, -28.31249999863440081, 0.000000000000000000 ) ) ;
#35881=CARTESIAN_POINT ( 'NONE',  ( 5.000000000000000000, -62.37499999726880873, -6.123233995736766282E-16 ) ) ;
#35885=CARTESIAN_POINT ( 'NONE',  ( -3.152548672688508926E-16, -22.56249999863440436, -5.148502694627439702 ) ) ;
#35886=CARTESIAN_POINT ( 'NONE',  ( 2.229367062499998831, -61.89583333196774362, -3.861377020970580887 ) ) ;
#35887=CARTESIAN_POINT ( 'NONE',  ( -6.972266317189433020E-16, -40.12499999726880162, -5.000000000000000000 ) ) ;
#35891=CARTESIAN_POINT ( 'NONE',  ( 5.000000000000000888, -13.58333333333333570, 2.886751345948126879 ) ) ;
#35893=ORIENTED_EDGE ( 'NONE', *, *, #5153, .F. ) ;
#35895=CARTESIAN_POINT ( 'NONE',  ( 5.000000000000000000, -38.37499999726881583, -6.123233995736766282E-16 ) ) ;
#35902=CARTESIAN_POINT ( 'NONE',  ( 2.500000000000002220, -81.66666666666667140, 4.330127018922192761 ) ) ;
#35905=EDGE_CURVE ( 'NONE', #19582, #45000, #39544, .T. ) ;
#35908=ORIENTED_EDGE ( 'NONE', *, *, #42050, .F. ) ;
#35909=CARTESIAN_POINT ( 'NONE',  ( 5.000000000000000000, 26.50000000000000000, -6.123233995736766282E-16 ) ) ;
#35913=VECTOR ( 'NONE', #39190, 1000.000000000000000 ) ;
#35918=ORIENTED_EDGE ( 'NONE', *, *, #46347, .T. ) ;
#35929=CARTESIAN_POINT ( 'NONE',  ( 2.229367062499998831, -79.64583333196773651, -3.861377020970580887 ) ) ;
#35930=CARTESIAN_POINT ( 'NONE',  ( 4.458734125000001214, -109.1458333319677365, 2.574251347313718519 ) ) ;
#35937=CARTESIAN_POINT ( 'NONE',  ( 4.458734125000000326, -44.89583333196774362, 2.574251347313718519 ) ) ;
#35940=CARTESIAN_POINT ( 'NONE',  ( -2.229367062500000163, -48.47916666530106511, -3.861377020970580443 ) ) ;
#35942=CARTESIAN_POINT ( 'NONE',  ( -4.458734124999998549, 26.77083333469893134, 2.574251347313722516 ) ) ;
#35943=CARTESIAN_POINT ( 'NONE',  ( 4.458734124999998549, -16.72916666530107577, -2.574251347313721627 ) ) ;
#35944=CARTESIAN_POINT ( 'NONE',  ( -5.000000000000000000, -100.0000000000000000, 0.000000000000000000 ) ) ;
#35946=CARTESIAN_POINT ( 'NONE',  ( -2.229367062499996610, -39.39583333196773651, 3.861377020970582219 ) ) ;
#35947=CARTESIAN_POINT ( 'NONE',  ( 5.000000000000000000, 1.708333336064519425, -2.886751345948129988 ) ) ;
#35948=CARTESIAN_POINT ( 'NONE',  ( -6.972266317189433020E-16, -50.24999999999999289, -5.000000000000000000 ) ) ;
#35951=CARTESIAN_POINT ( 'NONE',  ( -5.000000000000000000, 5.999999999999998224, 0.000000000000000000 ) ) ;
#35954=( BOUNDED_CURVE ( )  B_SPLINE_CURVE ( 2, ( #13067, #21462, #22093, #32687, #60709, #36561, #2480, #36250, #27540 ),
 .UNSPECIFIED., .F., .F. ) 
 B_SPLINE_CURVE_WITH_KNOTS ( ( 3, 2, 2, 2, 3 ),
 ( 0.2017857142857142905, 0.2023809523809523836, 0.2035714285714285698, 0.2047619047619047561, 0.2053571428571428492 ),
 .UNSPECIFIED. ) 
 CURVE ( )  GEOMETRIC_REPRESENTATION_ITEM ( )  RATIONAL_B_SPLINE_CURVE ( ( 0.9330127018922194093, 0.9330127018922194093, 1.000000000000000000, 0.8660254037844387076, 1.000000000000000000, 0.8660254037844387076, 1.000000000000000000, 0.9330127018922194093, 0.9330127018922194093 ) ) 
 REPRESENTATION_ITEM ( '' )  );
#35955=CARTESIAN_POINT ( 'NONE',  ( 9.457646018065525792E-16, -0.3124999986344051961, 5.148502694627439702 ) ) ;
#35956=ORIENTED_EDGE ( 'NONE', *, *, #46042, .F. ) ;
#35957=CARTESIAN_POINT ( 'NONE',  ( -6.972266317189433020E-16, -89.12499999726880162, -5.000000000000000000 ) ) ;
#35959=CARTESIAN_POINT ( 'NONE',  ( 2.229367062499998831, -87.64583333196773651, -3.861377020970580887 ) ) ;
#35961=CARTESIAN_POINT ( 'NONE',  ( -4.458734124999999437, -84.56249999863439371, 0.000000000000000000 ) ) ;
#35963=DIRECTION ( 'NONE',  ( 0.000000000000000000, 0.000000000000000000, 1.000000000000000000 ) ) ;
#35965=CARTESIAN_POINT ( 'NONE',  ( -2.229367062500000163, -5.479166665301072214, -3.861377020970580443 ) ) ;
#35966=CARTESIAN_POINT ( 'NONE',  ( -2.229367062499996610, 23.60416666803225993, 3.861377020970582219 ) ) ;
#35967=CARTESIAN_POINT ( 'NONE',  ( -4.458734124999999437, -46.56249999863440792, 0.000000000000000000 ) ) ;
#35972=VERTEX_POINT ( 'NONE', #25082 ) ;
#35975=CARTESIAN_POINT ( 'NONE',  ( 9.457646018065525792E-16, -74.06249999863440792, 5.148502694627439702 ) ) ;
#35976=CARTESIAN_POINT ( 'NONE',  ( -4.458734124999999437, 28.43750000136559208, 0.000000000000000000 ) ) ;
#35981=CARTESIAN_POINT ( 'NONE',  ( -3.535250795749689387E-16, -62.25000000000000000, -5.773502691896257311 ) ) ;
#35982=CARTESIAN_POINT ( 'NONE',  ( -1.339745962155613812, -32.08034179853029855, -5.000000000000000000 ) ) ;
#35984=ORIENTED_EDGE ( 'NONE', *, *, #47152, .F. ) ;
#35985=CARTESIAN_POINT ( 'NONE',  ( -6.972266317189433020E-16, -83.24999999999998579, -5.000000000000000000 ) ) ;
#35992=VERTEX_POINT ( 'NONE', #16073 ) ;
#35994=CARTESIAN_POINT ( 'NONE',  ( 2.500000000000002220, 27.45833333606451632, 4.330127018922192761 ) ) ;
#35996=VERTEX_POINT ( 'NONE', #54995 ) ;
#35999=VECTOR ( 'NONE', #1632, 1000.000000000000000 ) ;
#36000=CARTESIAN_POINT ( 'NONE',  ( 4.458734124999999437, -47.06249999863440792, -5.460374474430324690E-16 ) ) ;
#36003=AXIS2_PLACEMENT_3D ( 'NONE', #20627, #25115, #15150 ) ;
#36007=CARTESIAN_POINT ( 'NONE',  ( 0.000000000000000000, -120.0000000000000000, 0.000000000000000000 ) ) ;
#36009=CARTESIAN_POINT ( 'NONE',  ( -3.152548672688508926E-16, -94.81249999863442213, -5.148502694627439702 ) ) ;
#36010=CARTESIAN_POINT ( 'NONE',  ( -5.000000000000000000, -106.9999999999999858, 0.000000000000000000 ) ) ;
#36016=VERTEX_POINT ( 'NONE', #10922 ) ;
#36017=CARTESIAN_POINT ( 'NONE',  ( 4.458734124999998549, 0.2708333346989263979, -2.574251347313721627 ) ) ;
#36018=CARTESIAN_POINT ( 'NONE',  ( 5.000000000000000000, -106.4166666666666572, -2.886751345948130876 ) ) ;
#36019=CARTESIAN_POINT ( 'NONE',  ( -4.458734124999999437, -23.64583333196773651, -2.574251347313719407 ) ) ;
#36020=CARTESIAN_POINT ( 'NONE',  ( 5.000000000000000000, -70.50000000000000000, -6.123233995736766282E-16 ) ) ;
#36024=CARTESIAN_POINT ( 'NONE',  ( -2.229367062500000163, 16.27083333469892779, -3.861377020970580443 ) ) ;
#36025=ORIENTED_EDGE ( 'NONE', *, *, #15318, .T. ) ;
#36026=CARTESIAN_POINT ( 'NONE',  ( -6.972266317189433020E-16, -14.12499999726881228, -5.000000000000000000 ) ) ;
#36028=CARTESIAN_POINT ( 'NONE',  ( 2.500000000000002220, -82.66666666666667140, 4.330127018922192761 ) ) ;
#36029=CARTESIAN_POINT ( 'NONE',  ( -4.458734124999999437, -20.39583333196774362, -2.574251347313719407 ) ) ;
#36032=( BOUNDED_CURVE ( )  B_SPLINE_CURVE ( 2, ( #30769, #17247, #45243, #20808, #40411, #55861, #60050, #11774, #26584 ),
 .UNSPECIFIED., .F., .F. ) 
 B_SPLINE_CURVE_WITH_KNOTS ( ( 3, 2, 2, 2, 3 ),
 ( 0.6089285714285714857, 0.6095238095238095788, 0.6107142857142857650, 0.6119047619047619513, 0.6125000000000000444 ),
 .UNSPECIFIED. ) 
 CURVE ( )  GEOMETRIC_REPRESENTATION_ITEM ( )  RATIONAL_B_SPLINE_CURVE ( ( 0.9330127018922194093, 0.9330127018922256266, 1.000000000000000000, 0.8660254037844387076, 1.000000000000000000, 0.8660254037844387076, 1.000000000000000000, 0.9330127018922194093, 0.9330127018922194093 ) ) 
 REPRESENTATION_ITEM ( '' )  );
#36034=CARTESIAN_POINT ( 'NONE',  ( -5.000000000000000000, -44.87499999726880873, 0.000000000000000000 ) ) ;
#36036=CARTESIAN_POINT ( 'NONE',  ( -2.229367062499996610, 10.85416666803225993, 3.861377020970582219 ) ) ;
#36037=DIRECTION ( 'NONE',  ( 0.000000000000000000, 0.000000000000000000, -1.000000000000000000 ) ) ;
#36040=CARTESIAN_POINT ( 'NONE',  ( -4.458734124999999437, -65.31249999863440792, 0.000000000000000000 ) ) ;
#36043=CARTESIAN_POINT ( 'NONE',  ( -2.499999999999996447, 1.166666666666666519, 4.330127018922195425 ) ) ;
#36047=CARTESIAN_POINT ( 'NONE',  ( 2.229367062500001939, -60.97916666530106511, 3.861377020970579999 ) ) ;
#36048=CARTESIAN_POINT ( 'NONE',  ( 2.499999999999998668, -95.20833333060213022, -4.330127018922193649 ) ) ;
#36049=( BOUNDED_CURVE ( )  B_SPLINE_CURVE ( 2, ( #27481, #12053, #7878, #2422, #32307, #22034, #41005, #21722, #57088 ),
 .UNSPECIFIED., .F., .F. ) 
 B_SPLINE_CURVE_WITH_KNOTS ( ( 3, 2, 2, 2, 3 ),
 ( 0.9410714285714285587, 0.9416666666666666519, 0.9428571428571428381, 0.9440476190476190244, 0.9446428571428571175 ),
 .UNSPECIFIED. ) 
 CURVE ( )  GEOMETRIC_REPRESENTATION_ITEM ( )  RATIONAL_B_SPLINE_CURVE ( ( 0.9330127018922194093, 0.9330127018922194093, 1.000000000000000000, 0.8660254037844387076, 1.000000000000000000, 0.8660254037844387076, 1.000000000000000000, 0.9330127018922194093, 0.9330127018922194093 ) ) 
 REPRESENTATION_ITEM ( '' )  );
#36050=CARTESIAN_POINT ( 'NONE',  ( -1.339745962155613812, -70.20534180126148271, -5.000000000000000000 ) ) ;
#36054=CARTESIAN_POINT ( 'NONE',  ( 1.060575238724906964E-15, -44.74999999999999289, 5.773502691896257311 ) ) ;
#36056=CARTESIAN_POINT ( 'NONE',  ( 5.000000000000000000, -17.29166666393548368, -2.886751345948130876 ) ) ;
#36057=ORIENTED_EDGE ( 'NONE', *, *, #26206, .T. ) ;
#36058=CARTESIAN_POINT ( 'NONE',  ( -4.458734124999998549, -105.2291666653010651, 2.574251347313722516 ) ) ;
#36059=CARTESIAN_POINT ( 'NONE',  ( -4.458734124999999437, -2.562499998634407028, 0.000000000000000000 ) ) ;
#36060=CARTESIAN_POINT ( 'NONE',  ( 2.499999999999998668, -73.20833333060214443, -4.330127018922193649 ) ) ;
#36070=CARTESIAN_POINT ( 'NONE',  ( 1.975475456537005874E-15, -101.6249999972688158, 5.000000000000000000 ) ) ;
#36072=CARTESIAN_POINT ( 'NONE',  ( 9.457646018065525792E-16, -29.31249999863440436, 5.148502694627439702 ) ) ;
#36079=CARTESIAN_POINT ( 'NONE',  ( -6.972266317189433020E-16, -94.12499999726880162, -5.000000000000000000 ) ) ;
#36081=CARTESIAN_POINT ( 'NONE',  ( -2.229367062499996610, -80.39583333196773651, 3.861377020970582219 ) ) ;
#36084=CARTESIAN_POINT ( 'NONE',  ( -6.972266317189433020E-16, -15.12499999726881050, -5.000000000000000000 ) ) ;
#36089=CARTESIAN_POINT ( 'NONE',  ( 9.457646018065525792E-16, -10.31249999863440614, 5.148502694627439702 ) ) ;
#36091=CYLINDRICAL_SURFACE ( 'NONE', #8143, 5.000000000000000000 ) ;
#36092=CARTESIAN_POINT ( 'NONE',  ( 1.975475456537005874E-15, -92.62499999726881583, 5.000000000000000000 ) ) ;
#36093=ORIENTED_EDGE ( 'NONE', *, *, #26359, .T. ) ;
#36094=CARTESIAN_POINT ( 'NONE',  ( 4.458734125000001214, -6.145833331967741842, 2.574251347313718519 ) ) ;
#36099=CYLINDRICAL_SURFACE ( 'NONE', #47109, 5.000000000000000000 ) ;
#36100=ORIENTED_EDGE ( 'NONE', *, *, #56294, .F. ) ;
#36101=CARTESIAN_POINT ( 'NONE',  ( -3.152548672688508926E-16, -87.56249999863440792, -5.148502694627439702 ) ) ;
#36102=CARTESIAN_POINT ( 'NONE',  ( 5.000000000000000888, -29.45833333060214443, 2.886751345948126879 ) ) ;
#36103=CARTESIAN_POINT ( 'NONE',  ( -4.458734124999998549, -4.229166665301070438, 2.574251347313722516 ) ) ;
#36106=CARTESIAN_POINT ( 'NONE',  ( 2.499999999999998668, -29.20833333060214798, -4.330127018922193649 ) ) ;
#36109=CARTESIAN_POINT ( 'NONE',  ( 2.229367062500001939, 22.02083333469892779, 3.861377020970579999 ) ) ;
#36112=CARTESIAN_POINT ( 'NONE',  ( -3.152548672688508926E-16, -50.56249999863440792, -5.148502694627439702 ) ) ;
#36113=CARTESIAN_POINT ( 'NONE',  ( -2.229367062499996610, -35.39583333196772941, 3.861377020970582219 ) ) ;
#36116=CARTESIAN_POINT ( 'NONE',  ( -5.000000000000000000, 13.91666666666666785, -2.886751345948128211 ) ) ;
#36119=CARTESIAN_POINT ( 'NONE',  ( -3.152548672688508926E-16, -44.56249999863440081, -5.148502694627439702 ) ) ;
#36120=CARTESIAN_POINT ( 'NONE',  ( 5.000000000000000000, -78.29166666393547303, -2.886751345948129988 ) ) ;
#36123=CARTESIAN_POINT ( 'NONE',  ( 1.339745962155612702, -24.16965819600733312, -5.000000000000000000 ) ) ;
#36125=CARTESIAN_POINT ( 'NONE',  ( 2.229367062499998831, -84.89583333196773651, -3.861377020970580887 ) ) ;
#36128=CARTESIAN_POINT ( 'NONE',  ( 5.000000000000000000, -29.41666666666666785, -2.886751345948129988 ) ) ;
#36130=VERTEX_POINT ( 'NONE', #6437 ) ;
#36133=CARTESIAN_POINT ( 'NONE',  ( -4.458734124999998549, -89.22916666530106511, 2.574251347313722516 ) ) ;
#36134=CARTESIAN_POINT ( 'NONE',  ( -3.152548672688508926E-16, 14.18750000136559386, -5.148502694627439702 ) ) ;
#36136=CARTESIAN_POINT ( 'NONE',  ( -2.499999999999996447, 17.29166666939785557, 4.330127018922195425 ) ) ;
#36141=CARTESIAN_POINT ( 'NONE',  ( 2.499999999999998668, -61.20833333060214443, -4.330127018922193649 ) ) ;
#36142=EDGE_CURVE ( 'NONE', #49141, #44569, #24375, .T. ) ;
#36145=CARTESIAN_POINT ( 'NONE',  ( 1.975475456537005874E-15, -1.749999999999999334, 5.000000000000000000 ) ) ;
#36148=CARTESIAN_POINT ( 'NONE',  ( 5.000000000000000000, -96.41666666666667140, -2.886751345948130876 ) ) ;
#36150=CARTESIAN_POINT ( 'NONE',  ( 2.229367062499998831, -12.89583333196774007, -3.861377020970580887 ) ) ;
#36151=CARTESIAN_POINT ( 'NONE',  ( 0.000000000000000000, -120.0000000000000000, 5.000000000000000000 ) ) ;
#36160=CARTESIAN_POINT ( 'NONE',  ( 1.975475456537005874E-15, -85.62499999726880162, 5.000000000000000000 ) ) ;
#36162=CARTESIAN_POINT ( 'NONE',  ( -2.500000000000000444, -28.16666666666666785, -4.330127018922193649 ) ) ;
#36163=DIRECTION ( 'NONE',  ( -0.000000000000000000, 1.000000000000000000, -0.000000000000000000 ) ) ;
#36168=DIRECTION ( 'NONE',  ( 0.000000000000000000, 0.000000000000000000, 1.000000000000000000 ) ) ;
#36173=CARTESIAN_POINT ( 'NONE',  ( 1.339745962155612702, 11.70534180126147916, -5.000000000000000000 ) ) ;
#36174=CARTESIAN_POINT ( 'NONE',  ( 4.458734125000001214, 14.10416666803225993, 2.574251347313718519 ) ) ;
#36177=CARTESIAN_POINT ( 'NONE',  ( 2.500000000000002220, -108.5416666639354730, 4.330127018922192761 ) ) ;
#36179=ORIENTED_EDGE ( 'NONE', *, *, #7957, .T. ) ;
#36180=CARTESIAN_POINT ( 'NONE',  ( 4.458734125000000326, -70.89583333196773651, 2.574251347313718519 ) ) ;
#36181=DIRECTION ( 'NONE',  ( -0.000000000000000000, 1.000000000000000000, -0.000000000000000000 ) ) ;
#36182=CARTESIAN_POINT ( 'NONE',  ( -2.229367062500000163, 10.52083333469892779, -3.861377020970580443 ) ) ;
#36183=CARTESIAN_POINT ( 'NONE',  ( 2.493747252781420335E-13, -78.12499999726881583, -5.000000000000000000 ) ) ;
#36185=CARTESIAN_POINT ( 'NONE',  ( -3.152548672688508926E-16, -56.81249999863439371, -5.148502694627439702 ) ) ;
#36186=CARTESIAN_POINT ( 'NONE',  ( -5.000000000000000000, -12.95833333060214976, -2.886751345948128211 ) ) ;
#36190=CARTESIAN_POINT ( 'NONE',  ( -4.458734124999997661, -20.47916666530107577, 2.574251347313722516 ) ) ;
#36192=CARTESIAN_POINT ( 'NONE',  ( -4.999999999999998224, -60.91666666666666430, 2.886751345948131764 ) ) ;
#36193=CARTESIAN_POINT ( 'NONE',  ( -2.229367062499996610, -105.1458333319677365, 3.861377020970582219 ) ) ;
#36196=CARTESIAN_POINT ( 'NONE',  ( 2.229367062499998831, -104.8958333319677365, -3.861377020970580887 ) ) ;
#36197=CARTESIAN_POINT ( 'NONE',  ( -2.229367062499996610, -26.14583333196773651, 3.861377020970582219 ) ) ;
#36198=CARTESIAN_POINT ( 'NONE',  ( -2.499999999999996447, -64.70833333060213022, 4.330127018922195425 ) ) ;
#36201=CARTESIAN_POINT ( 'NONE',  ( 2.229367062499998831, -22.64583333196773651, -3.861377020970580887 ) ) ;
#36202=CARTESIAN_POINT ( 'NONE',  ( -4.458734124999999437, -66.56249999863440792, 0.000000000000000000 ) ) ;
#36205=CARTESIAN_POINT ( 'NONE',  ( -6.972266317189433020E-16, -33.24999999999999289, -5.000000000000000000 ) ) ;
#36207=CARTESIAN_POINT ( 'NONE',  ( -4.999999999999999112, -11.91666666666666607, 2.886751345948131764 ) ) ;
#36209=ORIENTED_EDGE ( 'NONE', *, *, #11470, .T. ) ;
#36211=CARTESIAN_POINT ( 'NONE',  ( 5.000000000000000000, -92.41666666666665719, -2.886751345948130876 ) ) ;
#36213=CARTESIAN_POINT ( 'NONE',  ( 1.339745962155612702, -76.16965819600731891, -5.000000000000000000 ) ) ;
#36220=ORIENTED_EDGE ( 'NONE', *, *, #27521, .F. ) ;
#36221=CARTESIAN_POINT ( 'NONE',  ( 1.975475456537005874E-15, -80.62499999726881583, 5.000000000000000000 ) ) ;
#36223=CARTESIAN_POINT ( 'NONE',  ( -2.500000000000000444, -54.04166666393548013, -4.330127018922193649 ) ) ;
#36238=EDGE_LOOP ( 'NONE', ( #63268, #6448, #6412, #9603 ) ) ;
#36239=EDGE_CURVE ( 'NONE', #38937, #58224, #11561, .T. ) ;
#36240=ADVANCED_FACE ( 'NONE', ( #21544 ), #60788, .T. ) ;
#36241=CARTESIAN_POINT ( 'NONE',  ( -4.458734124999998549, -79.22916666530107932, 2.574251347313722516 ) ) ;
#36242=CARTESIAN_POINT ( 'NONE',  ( -2.229367062500000163, 28.52083333469892779, -3.861377020970580443 ) ) ;
#36250=CARTESIAN_POINT ( 'NONE',  ( 1.339745962155615144, 0.4196582014697064489, 4.999999999999999112 ) ) ;
#36253=CARTESIAN_POINT ( 'NONE',  ( -2.229367062500000163, -51.47916666530107221, -3.861377020970580443 ) ) ;
#36255=CARTESIAN_POINT ( 'NONE',  ( -4.458734124999999437, 29.60416666803225993, -2.574251347313719407 ) ) ;
#36256=EDGE_CURVE ( 'NONE', #4410, #60061, #159, .T. ) ;
#36258=CARTESIAN_POINT ( 'NONE',  ( 5.000000000000000888, -105.5833333333333428, 2.886751345948126879 ) ) ;
#36260=CARTESIAN_POINT ( 'NONE',  ( 9.457646018065525792E-16, -37.31249999863440792, 5.148502694627439702 ) ) ;
#36261=CARTESIAN_POINT ( 'NONE',  ( 5.000000000000000000, 0.6250000027311873874, -6.123233995736766282E-16 ) ) ;
#36265=EDGE_CURVE ( 'NONE', #8539, #19698, #27932, .T. ) ;
#36267=CARTESIAN_POINT ( 'NONE',  ( -3.152548672688508926E-16, -97.56249999863440792, -5.148502694627439702 ) ) ;
#36268=CARTESIAN_POINT ( 'NONE',  ( -3.152548672688508926E-16, -2.812499998634407472, -5.148502694627439702 ) ) ;
#36269=EDGE_LOOP ( 'NONE', ( #39984, #42527, #37908, #33205 ) ) ;
#36271=ADVANCED_FACE ( 'NONE', ( #62364 ), #23117, .T. ) ;
#36273=CARTESIAN_POINT ( 'NONE',  ( 4.458734124999999437, -87.81249999863439371, -5.460374474430324690E-16 ) ) ;
#36275=CARTESIAN_POINT ( 'NONE',  ( 2.499999999999998668, 27.66666666666666430, -4.330127018922193649 ) ) ;
#36276=CARTESIAN_POINT ( 'NONE',  ( -3.152548672688508926E-16, -87.81249999863439371, -5.148502694627439702 ) ) ;
#36280=CARTESIAN_POINT ( 'NONE',  ( -4.458734124999999437, -7.312499998634404363, 0.000000000000000000 ) ) ;
#36281=CARTESIAN_POINT ( 'NONE',  ( 4.458734124999999437, 14.93750000136559386, -5.460374474430324690E-16 ) ) ;
#36282=CARTESIAN_POINT ( 'NONE',  ( 9.457646018065525792E-16, -47.31249999863440792, 5.148502694627439702 ) ) ;
#36290=CARTESIAN_POINT ( 'NONE',  ( 4.458734124999998549, -75.72916666530106511, -2.574251347313721627 ) ) ;
#36291=CARTESIAN_POINT ( 'NONE',  ( 2.229367062500001939, 28.77083333469892779, 3.861377020970579999 ) ) ;
#36293=CARTESIAN_POINT ( 'NONE',  ( -6.972266317189433020E-16, -58.12499999726880162, -5.000000000000000000 ) ) ;
#36296=CARTESIAN_POINT ( 'NONE',  ( 5.000000000000000000, -66.50000000000000000, -6.123233995736766282E-16 ) ) ;
#36297=CARTESIAN_POINT ( 'NONE',  ( -5.000000000000000000, -31.87499999726880873, 0.000000000000000000 ) ) ;
#36300=CARTESIAN_POINT ( 'NONE',  ( -5.000000000000000000, -57.08333333333333570, -2.886751345948128211 ) ) ;
#36305=CARTESIAN_POINT ( 'NONE',  ( 2.499999999999998668, -62.33333333333333570, -4.330127018922193649 ) ) ;
#36308=ORIENTED_EDGE ( 'NONE', *, *, #9152, .F. ) ;
#36309=DIRECTION ( 'NONE',  ( -0.000000000000000000, 1.000000000000000000, -0.000000000000000000 ) ) ;
#36310=CARTESIAN_POINT ( 'NONE',  ( -4.999999999999998224, 11.20833333606451809, 2.886751345948131764 ) ) ;
#36315=CARTESIAN_POINT ( 'NONE',  ( 4.458734125000001214, -45.14583333196774362, 2.574251347313718519 ) ) ;
#36316=LINE ( 'NONE', #18195, #27590 ) ;
#36323=CARTESIAN_POINT ( 'NONE',  ( 4.458734124999999437, -94.06249999863440792, -5.460374474430324690E-16 ) ) ;
#36325=ORIENTED_EDGE ( 'NONE', *, *, #24754, .F. ) ;
#36331=CARTESIAN_POINT ( 'NONE',  ( 2.229367062500001939, -1.979166665301068662, 3.861377020970579999 ) ) ;
#36334=CARTESIAN_POINT ( 'NONE',  ( -4.458734124999998549, -23.47916666530107577, 2.574251347313722516 ) ) ;
#36339=CARTESIAN_POINT ( 'NONE',  ( 4.458734125000000326, 15.85416666803226171, 2.574251347313718519 ) ) ;
#36340=ORIENTED_EDGE ( 'NONE', *, *, #18522, .F. ) ;
#36341=CARTESIAN_POINT ( 'NONE',  ( -1.339745962155610925, -18.66965819600733312, 5.000000000000000000 ) ) ;
#36342=CARTESIAN_POINT ( 'NONE',  ( -1.339745962155613812, -21.20534180126147561, -5.000000000000000000 ) ) ;
#36343=CARTESIAN_POINT ( 'NONE',  ( 5.000000000000000888, -84.58333333333332860, 2.886751345948126879 ) ) ;
#36344=CARTESIAN_POINT ( 'NONE',  ( 4.458734124999999437, -18.81249999863440792, -5.460374474430324690E-16 ) ) ;
#36349=CARTESIAN_POINT ( 'NONE',  ( -2.499999999999996447, -47.70833333060215153, 4.330127018922195425 ) ) ;
#36350=CYLINDRICAL_SURFACE ( 'NONE', #21032, 5.000000000000000000 ) ;
#36351=CARTESIAN_POINT ( 'NONE',  ( -4.458734124999999437, 10.68750000136559386, 0.000000000000000000 ) ) ;
#36355=CARTESIAN_POINT ( 'NONE',  ( 9.457646018065525792E-16, -67.06249999863440792, 5.148502694627439702 ) ) ;
#36357=CARTESIAN_POINT ( 'NONE',  ( 2.499999999999998668, 0.6666666666666660745, -4.330127018922193649 ) ) ;
#36360=CARTESIAN_POINT ( 'NONE',  ( 4.458734124999999437, -59.81249999863440081, -5.460374474430324690E-16 ) ) ;
#36361=CARTESIAN_POINT ( 'NONE',  ( 2.500000000000002220, -92.54166666393547303, 4.330127018922192761 ) ) ;
#36362=CARTESIAN_POINT ( 'NONE',  ( -5.000000000000000000, -70.08333333333332860, -2.886751345948128211 ) ) ;
#36366=CARTESIAN_POINT ( 'NONE',  ( 5.000000000000000888, -50.58333333333332860, 2.886751345948126879 ) ) ;
#36367=LINE ( 'NONE', #51175, #52124 ) ;
#36368=CARTESIAN_POINT ( 'NONE',  ( 1.975475456537005874E-15, -17.62499999726881938, 5.000000000000000000 ) ) ;
#36369=ORIENTED_EDGE ( 'NONE', *, *, #24727, .F. ) ;
#36370=CARTESIAN_POINT ( 'NONE',  ( 2.229367062500001939, -107.9791666653010651, 3.861377020970579999 ) ) ;
#36371=CARTESIAN_POINT ( 'NONE',  ( 4.458734124999998549, 0.02083333469892617584, -2.574251347313721627 ) ) ;
#36380=CARTESIAN_POINT ( 'NONE',  ( -1.339745962155613812, -17.08034179853029144, -5.000000000000000000 ) ) ;
#36382=ORIENTED_EDGE ( 'NONE', *, *, #48011, .F. ) ;
#36383=CARTESIAN_POINT ( 'NONE',  ( 1.975475456537005874E-15, -108.7499999999999858, 5.000000000000000000 ) ) ;
#36386=CARTESIAN_POINT ( 'NONE',  ( -4.458734124999999437, -31.56249999863440436, 0.000000000000000000 ) ) ;
#36393=CARTESIAN_POINT ( 'NONE',  ( -6.972266317189433020E-16, -83.12499999726878741, -5.000000000000000000 ) ) ;
#36395=CARTESIAN_POINT ( 'NONE',  ( 4.458734125000001214, -80.14583333196773651, 2.574251347313718519 ) ) ;
#36397=ORIENTED_EDGE ( 'NONE', *, *, #30283, .T. ) ;
#36398=CARTESIAN_POINT ( 'NONE',  ( 5.000000000000000888, -16.58333333333333215, 2.886751345948126879 ) ) ;
#36402=CARTESIAN_POINT ( 'NONE',  ( -3.152548672688508926E-16, -7.812499998634405252, -5.148502694627439702 ) ) ;
#36405=CARTESIAN_POINT ( 'NONE',  ( -4.999999999999998224, -84.91666666666667140, 2.886751345948131764 ) ) ;
#36408=CARTESIAN_POINT ( 'NONE',  ( 4.458734124999998549, -4.979166665301072214, -2.574251347313721627 ) ) ;
#36409=FACE_OUTER_BOUND ( 'NONE', #29800, .T. ) ;
#36411=CARTESIAN_POINT ( 'NONE',  ( 2.499999999999998668, -64.33333333333332860, -4.330127018922193649 ) ) ;
#36415=CARTESIAN_POINT ( 'NONE',  ( -2.229367062500000163, -84.47916666530107932, -3.861377020970580443 ) ) ;
#36416=CARTESIAN_POINT ( 'NONE',  ( 0.000000000000000000, -120.0000000000000000, 0.000000000000000000 ) ) ;
#36417=CARTESIAN_POINT ( 'NONE',  ( -2.229367062499996610, -3.145833331967738733, 3.861377020970582219 ) ) ;
#36419=VECTOR ( 'NONE', #20317, 1000.000000000000000 ) ;
#36420=( BOUNDED_CURVE ( )  B_SPLINE_CURVE ( 2, ( #50130, #25697, #45307, #1275, #40477, #60118, #35668, #55615, #17314 ),
 .UNSPECIFIED., .F., .F. ) 
 B_SPLINE_CURVE_WITH_KNOTS ( ( 3, 2, 2, 2, 3 ),
 ( 0.5803571428571429047, 0.5809523809523809978, 0.5821428571428571841, 0.5833333333333333703, 0.5839285714285714635 ),
 .UNSPECIFIED. ) 
 CURVE ( )  GEOMETRIC_REPRESENTATION_ITEM ( )  RATIONAL_B_SPLINE_CURVE ( ( 0.9330127018922194093, 0.9330127018922194093, 1.000000000000000000, 0.8660254037844387076, 1.000000000000000000, 0.8660254037844387076, 1.000000000000000000, 0.9330127018922194093, 0.9330127018922194093 ) ) 
 REPRESENTATION_ITEM ( '' )  );
#36421=CARTESIAN_POINT ( 'NONE',  ( 5.000000000000000000, -28.29166666393548013, -2.886751345948129988 ) ) ;
#36423=CARTESIAN_POINT ( 'NONE',  ( -3.152548672688508926E-16, 22.43750000136559564, -5.148502694627439702 ) ) ;
#36424=CARTESIAN_POINT ( 'NONE',  ( 2.500000000000002220, -104.6666666666666572, 4.330127018922192761 ) ) ;
#36426=CARTESIAN_POINT ( 'NONE',  ( -3.152548672688508926E-16, -49.56249999863440792, -5.148502694627439702 ) ) ;
#36427=CARTESIAN_POINT ( 'NONE',  ( -4.458734124999997661, -38.47916666530107221, 2.574251347313722516 ) ) ;
#36429=CARTESIAN_POINT ( 'NONE',  ( -2.499999999999996447, 9.291666669397853795, 4.330127018922195425 ) ) ;
#36430=CARTESIAN_POINT ( 'NONE',  ( -5.000000000000000000, 16.91666666666666430, -2.886751345948128211 ) ) ;
#36432=CARTESIAN_POINT ( 'NONE',  ( 9.457646018065525792E-16, -45.06249999863440792, 5.148502694627439702 ) ) ;
#36433=CARTESIAN_POINT ( 'NONE',  ( 5.000000000000000000, -79.37499999726881583, -6.123233995736766282E-16 ) ) ;
#36437=CARTESIAN_POINT ( 'NONE',  ( -4.458734124999997661, -87.47916666530107932, 2.574251347313722516 ) ) ;
#36440=CARTESIAN_POINT ( 'NONE',  ( 1.060575238724906964E-15, -32.75000000000000711, 5.773502691896257311 ) ) ;
#36445=CARTESIAN_POINT ( 'NONE',  ( -4.458734124999999437, -93.31249999863440792, 0.000000000000000000 ) ) ;
#36446=CARTESIAN_POINT ( 'NONE',  ( -2.229367062499996610, 13.60416666803226171, 3.861377020970582219 ) ) ;
#36447=CARTESIAN_POINT ( 'NONE',  ( 5.000000000000000888, 14.54166666939785024, 2.886751345948126879 ) ) ;
#36457=CARTESIAN_POINT ( 'NONE',  ( -1.339745962155610925, 18.33034180399266333, 5.000000000000000000 ) ) ;
#36461=CARTESIAN_POINT ( 'NONE',  ( 2.229367062499998831, -15.89583333196773651, -3.861377020970580887 ) ) ;
#36462=CARTESIAN_POINT ( 'NONE',  ( -5.000000000000000000, -58.08333333333333570, -2.886751345948128211 ) ) ;
#36472=ORIENTED_EDGE ( 'NONE', *, *, #4501, .T. ) ;
#36473=CARTESIAN_POINT ( 'NONE',  ( 4.458734124999998549, -60.97916666530106511, -2.574251347313721627 ) ) ;
#36474=CARTESIAN_POINT ( 'NONE',  ( 1.339745962155612702, -21.29465819873852084, -5.000000000000000000 ) ) ;
#36475=CARTESIAN_POINT ( 'NONE',  ( -6.972266317189433020E-16, -103.2500000000000000, -5.000000000000000000 ) ) ;
#36477=ORIENTED_EDGE ( 'NONE', *, *, #24697, .T. ) ;
#36478=( BOUNDED_CURVE ( )  B_SPLINE_CURVE ( 2, ( #46709, #61521, #56052, #37375, #57008, #32544, #57640, #19640, #39250 ),
 .UNSPECIFIED., .F., .F. ) 
 B_SPLINE_CURVE_WITH_KNOTS ( ( 3, 2, 2, 2, 3 ),
 ( 0.8910714285714286254, 0.8916666666666667185, 0.8928571428571429047, 0.8940476190476190910, 0.8946428571428571841 ),
 .UNSPECIFIED. ) 
 CURVE ( )  GEOMETRIC_REPRESENTATION_ITEM ( )  RATIONAL_B_SPLINE_CURVE ( ( 0.9330127018922194093, 0.9330127018922256266, 1.000000000000000000, 0.8660254037844387076, 1.000000000000000000, 0.8660254037844387076, 1.000000000000000000, 0.9330127018922194093, 0.9330127018922194093 ) ) 
 REPRESENTATION_ITEM ( '' )  );
#36484=CARTESIAN_POINT ( 'NONE',  ( 4.458734124999999437, 7.187500001365594748, -5.460374474430324690E-16 ) ) ;
#36489=CARTESIAN_POINT ( 'NONE',  ( 9.457646018065525792E-16, -69.06249999863439371, 5.148502694627439702 ) ) ;
#36490=LINE ( 'NONE', #31024, #36645 ) ;
#36491=CARTESIAN_POINT ( 'NONE',  ( -2.229367062500000163, 13.52083333469892779, -3.861377020970580443 ) ) ;
#36492=CARTESIAN_POINT ( 'NONE',  ( 5.000000000000000000, 7.708333336064518093, -2.886751345948130876 ) ) ;
#36494=CARTESIAN_POINT ( 'NONE',  ( 4.458734124999999437, -57.06249999863440081, -5.460374474430324690E-16 ) ) ;
#36495=CARTESIAN_POINT ( 'NONE',  ( 2.500000000000002220, -14.54166666393548191, 4.330127018922192761 ) ) ;
#36496=CARTESIAN_POINT ( 'NONE',  ( -2.499999999999996447, -44.70833333060214443, 4.330127018922195425 ) ) ;
#36497=CARTESIAN_POINT ( 'NONE',  ( 1.339745962155615144, -65.70534180126148271, 4.999999999999999112 ) ) ;
#36499=CARTESIAN_POINT ( 'NONE',  ( 4.458734125000000326, -21.14583333196774362, 2.574251347313718519 ) ) ;
#36500=ORIENTED_EDGE ( 'NONE', *, *, #10187, .T. ) ;
#36501=CARTESIAN_POINT ( 'NONE',  ( 1.975475456537005874E-15, -60.75000000000000000, 5.000000000000000000 ) ) ;
#36502=CARTESIAN_POINT ( 'NONE',  ( 2.229367062500001939, -109.9791666653010651, 3.861377020970579999 ) ) ;
#36504=VERTEX_POINT ( 'NONE', #18289 ) ;
#36505=CARTESIAN_POINT ( 'NONE',  ( -4.458734124999998549, -102.4791666653010509, 2.574251347313722516 ) ) ;
#36506=CARTESIAN_POINT ( 'NONE',  ( -3.152548672688508926E-16, -25.56249999863440436, -5.148502694627439702 ) ) ;
#36507=CARTESIAN_POINT ( 'NONE',  ( 5.000000000000000000, -62.29166666393547303, -2.886751345948129988 ) ) ;
#36511=CARTESIAN_POINT ( 'NONE',  ( 9.457646018065525792E-16, -25.06249999863440792, 5.148502694627439702 ) ) ;
#36512=CARTESIAN_POINT ( 'NONE',  ( -2.229367062499996610, -70.39583333196773651, 3.861377020970582219 ) ) ;
#36513=CARTESIAN_POINT ( 'NONE',  ( 2.499999999999998668, 8.666666666666666075, -4.330127018922193649 ) ) ;
#36515=CARTESIAN_POINT ( 'NONE',  ( 2.500000000000002220, -32.54166666393547303, 4.330127018922192761 ) ) ;
#36517=CARTESIAN_POINT ( 'NONE',  ( 5.000000000000000000, -16.50000000000000000, -6.123233995736766282E-16 ) ) ;
#36522=LINE ( 'NONE', #56152, #49345 ) ;
#36524=EDGE_CURVE ( 'NONE', #25814, #22293, #534, .T. ) ;
#36527=CARTESIAN_POINT ( 'NONE',  ( 5.000000000000000888, 1.541666669397853795, 2.886751345948126879 ) ) ;
#36528=CARTESIAN_POINT ( 'NONE',  ( 2.500000000000002220, -95.54166666393547303, 4.330127018922192761 ) ) ;
#36533=LINE ( 'NONE', #52599, #5835 ) ;
#36535=CARTESIAN_POINT ( 'NONE',  ( -2.499999999999996447, -50.83333333333332860, 4.330127018922195425 ) ) ;
#36540=ORIENTED_EDGE ( 'NONE', *, *, #28841, .T. ) ;
#36542=EDGE_CURVE ( 'NONE', #3482, #32387, #18907, .T. ) ;
#36543=ORIENTED_EDGE ( 'NONE', *, *, #54997, .T. ) ;
#36546=DIRECTION ( 'NONE',  ( 0.000000000000000000, 0.000000000000000000, 1.000000000000000000 ) ) ;
#36550=CARTESIAN_POINT ( 'NONE',  ( -1.339745962155610925, 21.20534180126147561, 5.000000000000000000 ) ) ;
#36551=ORIENTED_EDGE ( 'NONE', *, *, #26360, .T. ) ;
#36552=VECTOR ( 'NONE', #7279, 1000.000000000000000 ) ;
#36553=CARTESIAN_POINT ( 'NONE',  ( -2.229367062499996610, -75.14583333196773651, 3.861377020970582219 ) ) ;
#36554=CARTESIAN_POINT ( 'NONE',  ( -3.152548672688508926E-16, 24.43750000136559564, -5.148502694627439702 ) ) ;
#36555=CARTESIAN_POINT ( 'NONE',  ( 1.339745962155615144, -18.70534180126147916, 4.999999999999999112 ) ) ;
#36561=CARTESIAN_POINT ( 'NONE',  ( 5.000000000000000888, 0.5416666693978527958, 2.886751345948126879 ) ) ;
#36564=CARTESIAN_POINT ( 'NONE',  ( -4.458734124999997661, -57.22916666530107932, 2.574251347313722516 ) ) ;
#36566=CARTESIAN_POINT ( 'NONE',  ( -2.229367062500000163, 26.52083333469892779, -3.861377020970580443 ) ) ;
#36567=CARTESIAN_POINT ( 'NONE',  ( 1.060575238724906964E-15, -108.7499999999999858, 5.773502691896257311 ) ) ;
#36569=CARTESIAN_POINT ( 'NONE',  ( 4.458734125000001214, -37.14583333196773651, 2.574251347313718519 ) ) ;
#36570=CARTESIAN_POINT ( 'NONE',  ( 2.500000000000002220, -0.5416666639354792423, 4.330127018922192761 ) ) ;
#36574=CARTESIAN_POINT ( 'NONE',  ( -1.339745962155610925, 6.205341801261478274, 5.000000000000000000 ) ) ;
#36575=CARTESIAN_POINT ( 'NONE',  ( 2.229367062499998831, -103.6458333319677365, -3.861377020970580887 ) ) ;
#36576=CARTESIAN_POINT ( 'NONE',  ( 2.229367062500001939, -4.229166665301070438, 3.861377020970579999 ) ) ;
#36577=ORIENTED_EDGE ( 'NONE', *, *, #46332, .F. ) ;
#36578=DIRECTION ( 'NONE',  ( 0.000000000000000000, 0.000000000000000000, 1.000000000000000000 ) ) ;
#36580=CARTESIAN_POINT ( 'NONE',  ( 2.229367062500001939, -93.97916666530106511, 3.861377020970579999 ) ) ;
#36582=CARTESIAN_POINT ( 'NONE',  ( 4.458734125000001214, -87.14583333196772230, 2.574251347313718519 ) ) ;
#36586=CARTESIAN_POINT ( 'NONE',  ( 4.458734124999998549, -6.729166665301073103, -2.574251347313721627 ) ) ;
#36587=CARTESIAN_POINT ( 'NONE',  ( 2.229367062500001939, 14.77083333469892779, 3.861377020970579999 ) ) ;
#36588=CARTESIAN_POINT ( 'NONE',  ( 2.229367062500001939, -51.22916666530107221, 3.861377020970579999 ) ) ;
#36589=CARTESIAN_POINT ( 'NONE',  ( -4.999999999999998224, 17.20833333606451987, 2.886751345948131764 ) ) ;
#36592=CARTESIAN_POINT ( 'NONE',  ( 5.000000000000000000, -106.3749999972688158, -6.123233995736766282E-16 ) ) ;
#36597=CARTESIAN_POINT ( 'NONE',  ( 4.458734125000001214, -80.89583333196773651, 2.574251347313718519 ) ) ;
#36598=CARTESIAN_POINT ( 'NONE',  ( 5.000000000000000000, -109.2916666639354872, -2.886751345948129988 ) ) ;
#36599=AXIS2_PLACEMENT_3D ( 'NONE', #25750, #61446, #55982 ) ;
#36600=AXIS2_PLACEMENT_3D ( 'NONE', #47027, #50657, #61516 ) ;
#36608=CARTESIAN_POINT ( 'NONE',  ( 2.499999999999998668, -63.33333333333332149, -4.330127018922193649 ) ) ;
#36610=FACE_OUTER_BOUND ( 'NONE', #23018, .T. ) ;
#36612=EDGE_LOOP ( 'NONE', ( #61312, #30514, #36551, #7848 ) ) ;
#36616=CARTESIAN_POINT ( 'NONE',  ( 1.975475456537005874E-15, -86.75000000000001421, 5.000000000000000000 ) ) ;
#36620=EDGE_LOOP ( 'NONE', ( #9991, #44658, #26257, #55196 ) ) ;
#36627=CARTESIAN_POINT ( 'NONE',  ( -4.458734124999999437, -50.56249999863440792, 0.000000000000000000 ) ) ;
#36628=CARTESIAN_POINT ( 'NONE',  ( -6.972266317189433020E-16, -65.12499999726880162, -5.000000000000000000 ) ) ;
#36638=CARTESIAN_POINT ( 'NONE',  ( -4.458734124999999437, -92.56249999863440792, 0.000000000000000000 ) ) ;
#36640=ORIENTED_EDGE ( 'NONE', *, *, #40533, .F. ) ;
#36643=AXIS2_PLACEMENT_3D ( 'NONE', #19470, #44548, #58714 ) ;
#36644=CARTESIAN_POINT ( 'NONE',  ( 4.458734124999999437, -0.8124999986344055847, -5.460374474430324690E-16 ) ) ;
#36645=VECTOR ( 'NONE', #61266, 1000.000000000000000 ) ;
#36646=CARTESIAN_POINT ( 'NONE',  ( 9.457646018065525792E-16, -96.31249999863439371, 5.148502694627439702 ) ) ;
#36648=CARTESIAN_POINT ( 'NONE',  ( 4.458734125000001214, -25.14583333196774007, 2.574251347313718519 ) ) ;
#36649=AXIS2_PLACEMENT_3D ( 'NONE', #38782, #53276, #13097 ) ;
#36650=CARTESIAN_POINT ( 'NONE',  ( -4.999999999999998224, -66.91666666666667140, 2.886751345948131764 ) ) ;
#36654=CARTESIAN_POINT ( 'NONE',  ( 5.000000000000000000, -72.50000000000000000, -6.123233995736766282E-16 ) ) ;
#36657=( BOUNDED_CURVE ( )  B_SPLINE_CURVE ( 2, ( #10745, #59315, #50301, #15250, #30354, #5604, #49978, #1121, #5930 ),
 .UNSPECIFIED., .F., .F. ) 
 B_SPLINE_CURVE_WITH_KNOTS ( ( 3, 2, 2, 2, 3 ),
 ( 0.7624999999999999556, 0.7630952380952380487, 0.7642857142857142350, 0.7654761904761904212, 0.7660714285714286254 ),
 .UNSPECIFIED. ) 
 CURVE ( )  GEOMETRIC_REPRESENTATION_ITEM ( )  RATIONAL_B_SPLINE_CURVE ( ( 0.9330127018922194093, 0.9330127018922194093, 1.000000000000000000, 0.8660254037844387076, 1.000000000000000000, 0.8660254037844387076, 1.000000000000000000, 0.9330127018922130810, 0.9330127018922194093 ) ) 
 REPRESENTATION_ITEM ( '' )  );
#36658=CARTESIAN_POINT ( 'NONE',  ( 4.458734124999999437, 10.93750000136559386, -5.460374474430324690E-16 ) ) ;
#36659=ORIENTED_EDGE ( 'NONE', *, *, #53167, .T. ) ;
#36661=CARTESIAN_POINT ( 'NONE',  ( 5.000000000000000000, -66.37499999726881583, -6.123233995736766282E-16 ) ) ;
#36662=CARTESIAN_POINT ( 'NONE',  ( -2.499999999999996447, -86.83333333333332860, 4.330127018922195425 ) ) ;
#36663=CARTESIAN_POINT ( 'NONE',  ( 2.229367062500001939, -26.97916666530106866, 3.861377020970579999 ) ) ;
#36665=DIRECTION ( 'NONE',  ( -0.000000000000000000, 1.000000000000000000, -0.000000000000000000 ) ) ;
#36667=CARTESIAN_POINT ( 'NONE',  ( -5.000000000000000000, -46.87499999726880873, 0.000000000000000000 ) ) ;
#36668=CARTESIAN_POINT ( 'NONE',  ( 1.975475456537005874E-15, -1.624999997268813834, 5.000000000000000000 ) ) ;
#36669=CARTESIAN_POINT ( 'NONE',  ( 4.458734124999998549, 9.270833334698927786, -2.574251347313721627 ) ) ;
#36673=CARTESIAN_POINT ( 'NONE',  ( -3.152548672688508926E-16, -66.56249999863440792, -5.148502694627439702 ) ) ;
#36675=CARTESIAN_POINT ( 'NONE',  ( 5.000000000000000000, -2.416666666666664298, -2.886751345948129988 ) ) ;
#36677=CARTESIAN_POINT ( 'NONE',  ( -5.000000000000000000, 22.00000000000000000, 0.000000000000000000 ) ) ;
#36678=CARTESIAN_POINT ( 'NONE',  ( -2.229367062499996610, -62.14583333196774362, 3.861377020970582219 ) ) ;
#36679=CARTESIAN_POINT ( 'NONE',  ( -5.000000000000000000, -92.87499999726881583, 0.000000000000000000 ) ) ;
#36680=CARTESIAN_POINT ( 'NONE',  ( -2.499999999999996447, -79.83333333333332860, 4.330127018922195425 ) ) ;
#36681=CARTESIAN_POINT ( 'NONE',  ( 5.000000000000000000, -56.49999999999999289, -6.123233995736766282E-16 ) ) ;
#36687=CARTESIAN_POINT ( 'NONE',  ( 2.500000000000002220, -46.66666666666666430, 4.330127018922192761 ) ) ;
#36690=VERTEX_POINT ( 'NONE', #38834 ) ;
#36691=CARTESIAN_POINT ( 'NONE',  ( -4.458734124999998549, -106.2291666653010793, 2.574251347313722516 ) ) ;
#36692=CARTESIAN_POINT ( 'NONE',  ( -4.458734124999998549, -3.479166665301069994, 2.574251347313722516 ) ) ;
#36693=CARTESIAN_POINT ( 'NONE',  ( 1.339745962155499015, -73.58034179853028434, 5.000000000000065725 ) ) ;
#36697=LINE ( 'NONE', #3251, #54452 ) ;
#36701=VECTOR ( 'NONE', #40351, 1000.000000000000000 ) ;
#36702=CARTESIAN_POINT ( 'NONE',  ( 5.000000000000000000, -100.2916666639354446, -2.886751345948130876 ) ) ;
#36709=CARTESIAN_POINT ( 'NONE',  ( -4.458734124999999437, -36.56249999863440792, 0.000000000000000000 ) ) ;
#36710=CARTESIAN_POINT ( 'NONE',  ( -5.000000000000000000, -87.08333333333331439, -2.886751345948128211 ) ) ;
#36712=( BOUNDED_CURVE ( )  B_SPLINE_CURVE ( 2, ( #43309, #58427, #62944, #35575, #30745, #11118, #21099, #20783, #39421 ),
 .UNSPECIFIED., .F., .F. ) 
 B_SPLINE_CURVE_WITH_KNOTS ( ( 3, 2, 2, 2, 3 ),
 ( 0.4839285714285714302, 0.4845238095238095233, 0.4857142857142857095, 0.4869047619047618958, 0.4874999999999999889 ),
 .UNSPECIFIED. ) 
 CURVE ( )  GEOMETRIC_REPRESENTATION_ITEM ( )  RATIONAL_B_SPLINE_CURVE ( ( 0.9330127018922194093, 0.9330127018922194093, 1.000000000000000000, 0.8660254037844387076, 1.000000000000000000, 0.8660254037844387076, 1.000000000000000000, 0.9330127018922194093, 0.9330127018922194093 ) ) 
 REPRESENTATION_ITEM ( '' )  );
#36714=EDGE_CURVE ( 'NONE', #3623, #50310, #9885, .T. ) ;
#36720=CARTESIAN_POINT ( 'NONE',  ( 0.000000000000000000, -120.0000000000000000, 0.000000000000000000 ) ) ;
#36721=CARTESIAN_POINT ( 'NONE',  ( 4.458734124999998549, -75.97916666530106511, -2.574251347313721627 ) ) ;
#36724=CARTESIAN_POINT ( 'NONE',  ( -1.339745962155610925, -14.66965819600733667, 5.000000000000000000 ) ) ;
#36727=CARTESIAN_POINT ( 'NONE',  ( -3.152548672688508926E-16, -10.81249999863440792, -5.148502694627439702 ) ) ;
#36730=CARTESIAN_POINT ( 'NONE',  ( -4.458734124999999437, -5.562499998634402587, 0.000000000000000000 ) ) ;
#36733=CARTESIAN_POINT ( 'NONE',  ( 5.000000000000000000, -64.41666666666665719, -2.886751345948130876 ) ) ;
#36736=CARTESIAN_POINT ( 'NONE',  ( -2.229367062500000163, 29.27083333469892779, -3.861377020970580443 ) ) ;
#36738=CARTESIAN_POINT ( 'NONE',  ( 4.458734125000000326, -85.89583333196775072, 2.574251347313718519 ) ) ;
#36740=CARTESIAN_POINT ( 'NONE',  ( -3.152548672688508926E-16, -4.562499998634401699, -5.148502694627439702 ) ) ;
#36741=VECTOR ( 'NONE', #56449, 1000.000000000000000 ) ;
#36743=STYLED_ITEM('',(#63705),#50626);
#36744=CARTESIAN_POINT ( 'NONE',  ( -2.500000000000000444, -32.04166666393548724, -4.330127018922193649 ) ) ;
#36745=CARTESIAN_POINT ( 'NONE',  ( -4.729367062499999719, -110.1562499993171969, 0.000000000000000000 ) ) ;
#36746=CARTESIAN_POINT ( 'NONE',  ( -4.458734124999999437, 25.60416666803225638, -2.574251347313719407 ) ) ;
#36749=CARTESIAN_POINT ( 'NONE',  ( -2.229367062500000163, -50.47916666530107221, -3.861377020970580443 ) ) ;
#36750=CARTESIAN_POINT ( 'NONE',  ( -4.458734124999999437, -39.56249999863440081, 0.000000000000000000 ) ) ;
#36753=CARTESIAN_POINT ( 'NONE',  ( -2.500000000000000444, 13.83333333333333215, -4.330127018922193649 ) ) ;
#36756=CARTESIAN_POINT ( 'NONE',  ( 4.458734124999999437, -40.81249999863440081, -5.460374474430324690E-16 ) ) ;
#36757=CARTESIAN_POINT ( 'NONE',  ( -4.999999999999999112, -80.79166666393547303, 2.886751345948131764 ) ) ;
#36763=CARTESIAN_POINT ( 'NONE',  ( 4.458734124999999437, -86.06249999863439371, -5.460374474430324690E-16 ) ) ;
#36765=CARTESIAN_POINT ( 'NONE',  ( -5.000000000000000000, -34.08333333333332860, -2.886751345948128211 ) ) ;
#36770=CARTESIAN_POINT ( 'NONE',  ( -2.229367062499996610, -89.14583333196773651, 3.861377020970582219 ) ) ;
#36771=CARTESIAN_POINT ( 'NONE',  ( 4.458734124999998549, 16.02083333469892423, -2.574251347313721627 ) ) ;
#36772=CARTESIAN_POINT ( 'NONE',  ( -3.535250795749689387E-16, 13.87500000273118417, -5.773502691896257311 ) ) ;
#36773=CARTESIAN_POINT ( 'NONE',  ( 1.975475456537005874E-15, -28.62499999726881583, 5.000000000000000000 ) ) ;
#36782=CARTESIAN_POINT ( 'NONE',  ( -4.458734124999999437, -15.56249999863440436, 0.000000000000000000 ) ) ;
#36790=( BOUNDED_CURVE ( )  B_SPLINE_CURVE ( 2, ( #38350, #57976, #33529, #13902, #23874, #54414, #48621, #34452, #19991 ),
 .UNSPECIFIED., .F., .F. ) 
 B_SPLINE_CURVE_WITH_KNOTS ( ( 3, 2, 2, 2, 3 ),
 ( 0.07321428571428571785, 0.07380952380952381098, 0.07499999999999999722, 0.07619047619047619735, 0.07678571428571429047 ),
 .UNSPECIFIED. ) 
 CURVE ( )  GEOMETRIC_REPRESENTATION_ITEM ( )  RATIONAL_B_SPLINE_CURVE ( ( 0.9330127018922194093, 0.9330127018922194093, 1.000000000000000000, 0.8660254037844387076, 1.000000000000000000, 0.8660254037844387076, 1.000000000000000000, 0.9330127018922194093, 0.9330127018922194093 ) ) 
 REPRESENTATION_ITEM ( '' )  );
#36796=CARTESIAN_POINT ( 'NONE',  ( 2.229367062499998831, -62.89583333196774362, -3.861377020970580887 ) ) ;
#36800=CARTESIAN_POINT ( 'NONE',  ( -5.000000000000000000, 27.12500000273118772, 0.000000000000000000 ) ) ;
#36802=CARTESIAN_POINT ( 'NONE',  ( 0.000000000000000000, -120.0000000000000000, 0.000000000000000000 ) ) ;
#36804=VERTEX_POINT ( 'NONE', #26602 ) ;
#36807=CARTESIAN_POINT ( 'NONE',  ( -5.000000000000000000, -109.9583333306021444, -2.886751345948128211 ) ) ;
#36808=CARTESIAN_POINT ( 'NONE',  ( -4.458734124999999437, 8.604166668032261711, -2.574251347313719407 ) ) ;
#36812=CARTESIAN_POINT ( 'NONE',  ( -6.972266317189433020E-16, -25.12499999726881228, -5.000000000000000000 ) ) ;
#36814=CARTESIAN_POINT ( 'NONE',  ( -4.458734124999997661, -73.22916666530106511, 2.574251347313722516 ) ) ;
#36815=DIRECTION ( 'NONE',  ( -0.000000000000000000, 1.000000000000000000, -0.000000000000000000 ) ) ;
#36816=CARTESIAN_POINT ( 'NONE',  ( -2.229367062500000163, 14.52083333469892779, -3.861377020970580443 ) ) ;
#36818=CARTESIAN_POINT ( 'NONE',  ( -2.500000000000000444, -89.16666666666665719, -4.330127018922193649 ) ) ;
#36819=CARTESIAN_POINT ( 'NONE',  ( -2.229367062499996610, -57.39583333196773651, 3.861377020970582219 ) ) ;
#36820=CARTESIAN_POINT ( 'NONE',  ( -4.999999999999999112, -15.79166666393548191, 2.886751345948131764 ) ) ;
#36824=CARTESIAN_POINT ( 'NONE',  ( 4.458734124999999437, -34.81249999863440792, -5.460374474430324690E-16 ) ) ;
#36825=CARTESIAN_POINT ( 'NONE',  ( -2.229367062499996610, -19.39583333196774007, 3.861377020970582219 ) ) ;
#36827=VECTOR ( 'NONE', #21622, 1000.000000000000000 ) ;
#36828=DIRECTION ( 'NONE',  ( 0.8660254037844347108, 0.000000000000000000, -0.5000000000000069944 ) ) ;
#36829=CARTESIAN_POINT ( 'NONE',  ( -5.000000000000000000, 30.00000000000000000, 0.000000000000000000 ) ) ;
#36831=ORIENTED_EDGE ( 'NONE', *, *, #24835, .T. ) ;
#36832=CARTESIAN_POINT ( 'NONE',  ( -4.458734124999999437, -102.6458333319677507, -2.574251347313719407 ) ) ;
#36833=CARTESIAN_POINT ( 'NONE',  ( -2.229367062499996610, -24.14583333196773651, 3.861377020970582219 ) ) ;
#36834=CARTESIAN_POINT ( 'NONE',  ( 2.499999999999998668, -60.20833333060214443, -4.330127018922193649 ) ) ;
#36837=CARTESIAN_POINT ( 'NONE',  ( 4.458734124999998549, -26.72916666530106866, -2.574251347313721627 ) ) ;
#36838=CARTESIAN_POINT ( 'NONE',  ( -4.458734124999997661, -68.47916666530107932, 2.574251347313722516 ) ) ;
#36839=DIRECTION ( 'NONE',  ( 1.000000000000000000, 0.000000000000000000, -3.305092117221761110E-15 ) ) ;
#36843=CARTESIAN_POINT ( 'NONE',  ( -5.000000000000000000, -15.08333333333333215, -2.886751345948128211 ) ) ;
#36846=CARTESIAN_POINT ( 'NONE',  ( -6.972266317189433020E-16, -66.12499999726881583, -5.000000000000000000 ) ) ;
#36848=CARTESIAN_POINT ( 'NONE',  ( 0.000000000000000000, -120.0000000000000000, 5.000000000000000000 ) ) ;
#36849=DIRECTION ( 'NONE',  ( 0.000000000000000000, 0.000000000000000000, 1.000000000000000000 ) ) ;
#36851=VECTOR ( 'NONE', #19147, 1000.000000000000000 ) ;
#36855=FACE_OUTER_BOUND ( 'NONE', #1181, .T. ) ;
#36859=VERTEX_POINT ( 'NONE', #40745 ) ;
#36860=CARTESIAN_POINT ( 'NONE',  ( 4.648177544792955347E-16, 29.75000000000000355, -5.000000000000000000 ) ) ;
#36871=CARTESIAN_POINT ( 'NONE',  ( 0.000000000000000000, -120.0000000000000000, 0.000000000000000000 ) ) ;
#36876=ORIENTED_EDGE ( 'NONE', *, *, #14223, .T. ) ;
#36877=CARTESIAN_POINT ( 'NONE',  ( 9.457646018065525792E-16, -76.06249999863440792, 5.148502694627439702 ) ) ;
#36878=CARTESIAN_POINT ( 'NONE',  ( -2.229367062500000163, 22.52083333469892423, -3.861377020970580443 ) ) ;
#36881=DIRECTION ( 'NONE',  ( 0.000000000000000000, 0.000000000000000000, 1.000000000000000000 ) ) ;
#36885=DIRECTION ( 'NONE',  ( 0.000000000000000000, 1.000000000000000000, 0.000000000000000000 ) ) ;
#36889=CARTESIAN_POINT ( 'NONE',  ( -4.458734124999997661, -54.22916666530107221, 2.574251347313722516 ) ) ;
#36893=CARTESIAN_POINT ( 'NONE',  ( 5.000000000000000000, -107.4999999999999858, -6.123233995736766282E-16 ) ) ;
#36894=CARTESIAN_POINT ( 'NONE',  ( -4.458734124999998549, -39.47916666530107932, 2.574251347313722516 ) ) ;
#36895=CARTESIAN_POINT ( 'NONE',  ( -3.535250795749689387E-16, 3.875000002731186832, -5.773502691896257311 ) ) ;
#36900=CARTESIAN_POINT ( 'NONE',  ( -4.458734124999999437, -105.3124999986344221, 0.000000000000000000 ) ) ;
#36901=CARTESIAN_POINT ( 'NONE',  ( -4.458734124999999437, -6.562499998634403475, 0.000000000000000000 ) ) ;
#36904=CARTESIAN_POINT ( 'NONE',  ( -3.152548672688508926E-16, -94.56249999863440792, -5.148502694627439702 ) ) ;
#36906=CARTESIAN_POINT ( 'NONE',  ( 2.229367062499998831, -85.89583333196773651, -3.861377020970580887 ) ) ;
#36911=CARTESIAN_POINT ( 'NONE',  ( 2.229367062500001939, -7.979166665301073991, 3.861377020970579999 ) ) ;
#36912=CARTESIAN_POINT ( 'NONE',  ( -2.229367062500000163, 17.27083333469892779, -3.861377020970580443 ) ) ;
#36913=ADVANCED_FACE ( 'NONE', ( #16631 ), #55567, .T. ) ;
#36914=CARTESIAN_POINT ( 'NONE',  ( 9.457646018065525792E-16, -55.31249999863439371, 5.148502694627439702 ) ) ;
#36923=CARTESIAN_POINT ( 'NONE',  ( 2.229367062499998831, -82.64583333196773651, -3.861377020970580887 ) ) ;
#36924=CARTESIAN_POINT ( 'NONE',  ( -2.229367062499996610, 25.60416666803225993, 3.861377020970582219 ) ) ;
#36925=VECTOR ( 'NONE', #51417, 1000.000000000000000 ) ;
#36932=CARTESIAN_POINT ( 'NONE',  ( -2.499999999999996447, -62.83333333333333570, 4.330127018922195425 ) ) ;
#36938=CARTESIAN_POINT ( 'NONE',  ( -4.999999999999998224, -71.91666666666667140, 2.886751345948131764 ) ) ;
#36950=CARTESIAN_POINT ( 'NONE',  ( 9.457646018065525792E-16, -50.31249999863440792, 5.148502694627439702 ) ) ;
#36953=ORIENTED_EDGE ( 'NONE', *, *, #34641, .F. ) ;
#36957=CARTESIAN_POINT ( 'NONE',  ( 2.499999999999998668, 22.66666666666666430, -4.330127018922193649 ) ) ;
#36959=CARTESIAN_POINT ( 'NONE',  ( 2.229367062499998831, -98.89583333196773651, -3.861377020970580887 ) ) ;
#36960=CARTESIAN_POINT ( 'NONE',  ( 0.000000000000000000, -120.0000000000000000, 0.000000000000000000 ) ) ;
#36961=ORIENTED_EDGE ( 'NONE', *, *, #21760, .F. ) ;
#36966=VECTOR ( 'NONE', #3945, 1000.000000000000000 ) ;
#36968=CARTESIAN_POINT ( 'NONE',  ( -4.458734124999999437, -6.312499998634403475, 0.000000000000000000 ) ) ;
#36969=CARTESIAN_POINT ( 'NONE',  ( -3.152548672688508926E-16, -94.81249999863439371, -5.148502694627439702 ) ) ;
#36973=CARTESIAN_POINT ( 'NONE',  ( 2.229367062499998831, -21.89583333196774007, -3.861377020970580887 ) ) ;
#36980=CARTESIAN_POINT ( 'NONE',  ( 2.229367062500001939, 12.77083333469892779, 3.861377020970579999 ) ) ;
#36982=CARTESIAN_POINT ( 'NONE',  ( -5.000000000000000000, -4.999999999999997335, 0.000000000000000000 ) ) ;
#36984=CARTESIAN_POINT ( 'NONE',  ( 5.000000000000000888, -92.58333333333332860, 2.886751345948126879 ) ) ;
#36985=CARTESIAN_POINT ( 'NONE',  ( 2.229367062500001939, -24.97916666530106866, 3.861377020970579999 ) ) ;
#36987=CARTESIAN_POINT ( 'NONE',  ( 9.457646018065525792E-16, -72.31249999863440792, 5.148502694627439702 ) ) ;
#36992=CARTESIAN_POINT ( 'NONE',  ( 2.500000000000002220, -52.54166666393548013, 4.330127018922192761 ) ) ;
#36994=CARTESIAN_POINT ( 'NONE',  ( 9.457646018065525792E-16, 8.937500001365595637, 5.148502694627439702 ) ) ;
#36996=EDGE_CURVE ( 'NONE', #34626, #29404, #7115, .T. ) ;
#36999=CARTESIAN_POINT ( 'NONE',  ( -4.458734124999998549, -73.22916666530106511, 2.574251347313722516 ) ) ;
#37001=CARTESIAN_POINT ( 'NONE',  ( -2.500000000000000444, 1.833333333333332593, -4.330127018922193649 ) ) ;
#37003=CARTESIAN_POINT ( 'NONE',  ( -6.972266317189433020E-16, -109.2499999999999858, -5.000000000000000000 ) ) ;
#37004=CARTESIAN_POINT ( 'NONE',  ( -4.458734124999999437, -65.39583333196773651, -2.574251347313719407 ) ) ;
#37005=CARTESIAN_POINT ( 'NONE',  ( 2.499999999999998668, -101.2083333306021444, -4.330127018922193649 ) ) ;
#37009=CARTESIAN_POINT ( 'NONE',  ( 2.499999999999998668, -50.33333333333332860, -4.330127018922193649 ) ) ;
#37012=EDGE_LOOP ( 'NONE', ( #21242, #52047, #8845, #13429 ) ) ;
#37019=CARTESIAN_POINT ( 'NONE',  ( -1.339745962155610925, -30.66965819600732956, 5.000000000000000000 ) ) ;
#37025=VERTEX_POINT ( 'NONE', #22419 ) ;
#37029=CARTESIAN_POINT ( 'NONE',  ( 2.229367062499998831, -34.89583333196772941, -3.861377020970580887 ) ) ;
#37037=DIRECTION ( 'NONE',  ( -0.000000000000000000, 1.000000000000000000, -0.000000000000000000 ) ) ;
#37038=CARTESIAN_POINT ( 'NONE',  ( -4.458734124999999437, -81.56249999863440792, 0.000000000000000000 ) ) ;
#37039=CARTESIAN_POINT ( 'NONE',  ( -6.031010364368858512E-14, 3.249999999999997335, 5.000000000000000000 ) ) ;
#37040=( BOUNDED_CURVE ( )  B_SPLINE_CURVE ( 2, ( #26419, #16769, #31877, #41837, #61482, #51817, #7759, #13208, #58532 ),
 .UNSPECIFIED., .F., .F. ) 
 B_SPLINE_CURVE_WITH_KNOTS ( ( 3, 2, 2, 2, 3 ),
 ( 0.2874999999999999778, 0.2880952380952380709, 0.2892857142857143127, 0.2904761904761904989, 0.2910714285714285920 ),
 .UNSPECIFIED. ) 
 CURVE ( )  GEOMETRIC_REPRESENTATION_ITEM ( )  RATIONAL_B_SPLINE_CURVE ( ( 0.9330127018922194093, 0.9330127018922194093, 1.000000000000000000, 0.8660254037844387076, 1.000000000000000000, 0.8660254037844387076, 1.000000000000000000, 0.9330127018922194093, 0.9330127018922194093 ) ) 
 REPRESENTATION_ITEM ( '' )  );
#37041=EDGE_LOOP ( 'NONE', ( #9722, #39689, #11942, #19273 ) ) ;
#37042=CARTESIAN_POINT ( 'NONE',  ( -5.000000000000000000, -94.95833333060213022, -2.886751345948128211 ) ) ;
#37045=CARTESIAN_POINT ( 'NONE',  ( 9.457646018065525792E-16, -8.312499998634406140, 5.148502694627439702 ) ) ;
#37048=EDGE_CURVE ( 'NONE', #62346, #36859, #19859, .T. ) ;
#37050=CARTESIAN_POINT ( 'NONE',  ( -4.458734124999999437, -4.562499998634401699, 0.000000000000000000 ) ) ;
#37053=AXIS2_PLACEMENT_3D ( 'NONE', #35651, #63410, #45614 ) ;
#37057=CARTESIAN_POINT ( 'NONE',  ( 4.458734125000000326, 28.85416666803226704, 2.574251347313718519 ) ) ;
#37058=EDGE_LOOP ( 'NONE', ( #40597, #10505, #2401, #29303 ) ) ;
#37059=CARTESIAN_POINT ( 'NONE',  ( -4.458734124999999437, -87.31249999863439371, 0.000000000000000000 ) ) ;
#37060=CARTESIAN_POINT ( 'NONE',  ( -1.339745962155613812, -78.20534180126146850, -5.000000000000000000 ) ) ;
#37061=CARTESIAN_POINT ( 'NONE',  ( -4.458734124999999437, -6.395833331967740953, -2.574251347313719407 ) ) ;
#37066=FACE_OUTER_BOUND ( 'NONE', #3580, .T. ) ;
#37067=DIRECTION ( 'NONE',  ( 0.000000000000000000, 0.000000000000000000, 1.000000000000000000 ) ) ;
#37068=CARTESIAN_POINT ( 'NONE',  ( -2.499999999999996447, -37.70833333060213732, 4.330127018922195425 ) ) ;
#37070=CARTESIAN_POINT ( 'NONE',  ( 2.229367062500001939, 27.02083333469892423, 3.861377020970579999 ) ) ;
#37072=( BOUNDED_CURVE ( )  B_SPLINE_CURVE ( 2, ( #49244, #44408, #21252, #20299, #368, #55030, #19971, #39581, #15792 ),
 .UNSPECIFIED., .F., .F. ) 
 B_SPLINE_CURVE_WITH_KNOTS ( ( 3, 2, 2, 2, 3 ),
 ( 0.06250000000000000000, 0.06309523809523809312, 0.06428571428571427937, 0.06547619047619047949, 0.06607142857142857262 ),
 .UNSPECIFIED. ) 
 CURVE ( )  GEOMETRIC_REPRESENTATION_ITEM ( )  RATIONAL_B_SPLINE_CURVE ( ( 0.9330127018922194093, 0.9330127018922194093, 1.000000000000000000, 0.8660254037844387076, 1.000000000000000000, 0.8660254037844387076, 1.000000000000000000, 0.9330127018922194093, 0.9330127018922194093 ) ) 
 REPRESENTATION_ITEM ( '' )  );
#37075=CARTESIAN_POINT ( 'NONE',  ( -3.152548672688508926E-16, -54.56249999863439371, -5.148502694627439702 ) ) ;
#37078=CARTESIAN_POINT ( 'NONE',  ( -2.500000000000000444, 16.83333333333333215, -4.330127018922193649 ) ) ;
#37082=CARTESIAN_POINT ( 'NONE',  ( 2.229367062499998831, -45.64583333196774362, -3.861377020970580887 ) ) ;
#37083=CARTESIAN_POINT ( 'NONE',  ( -3.535250795749689387E-16, -80.12499999726880162, -5.773502691896257311 ) ) ;
#37088=CARTESIAN_POINT ( 'NONE',  ( 4.458734124999998549, -87.97916666530107932, -2.574251347313721627 ) ) ;
#37090=CARTESIAN_POINT ( 'NONE',  ( 5.000000000000000000, -32.50000000000000000, -6.123233995736766282E-16 ) ) ;
#37094=CARTESIAN_POINT ( 'NONE',  ( -2.229367062500000163, -94.47916666530106511, -3.861377020970580443 ) ) ;
#37095=CARTESIAN_POINT ( 'NONE',  ( 9.457646018065525792E-16, 15.68750000136559386, 5.148502694627439702 ) ) ;
#37096=CARTESIAN_POINT ( 'NONE',  ( 2.500000000000002220, 15.45833333606451987, 4.330127018922192761 ) ) ;
#37102=CARTESIAN_POINT ( 'NONE',  ( 5.000000000000000000, -80.41666666666667140, -2.886751345948129988 ) ) ;
#37104=DIRECTION ( 'NONE',  ( 0.000000000000000000, 0.000000000000000000, 1.000000000000000000 ) ) ;
#37105=CARTESIAN_POINT ( 'NONE',  ( -5.000000000000000000, -25.87499999726881583, 0.000000000000000000 ) ) ;
#37108=CARTESIAN_POINT ( 'NONE',  ( 2.500000000000002220, -96.66666666666665719, 4.330127018922192761 ) ) ;
#37109=CARTESIAN_POINT ( 'NONE',  ( -5.000000000000000000, 13.99999999999999822, 0.000000000000000000 ) ) ;
#37110=CARTESIAN_POINT ( 'NONE',  ( -4.458734124999999437, -17.56249999863440792, 0.000000000000000000 ) ) ;
#37120=DIRECTION ( 'NONE',  ( -0.000000000000000000, 1.000000000000000000, -0.000000000000000000 ) ) ;
#37122=CARTESIAN_POINT ( 'NONE',  ( -3.152548672688508926E-16, -66.81249999863442213, -5.148502694627439702 ) ) ;
#37125=CARTESIAN_POINT ( 'NONE',  ( -2.500000000000000444, -47.16666666666666430, -4.330127018922193649 ) ) ;
#37132=CARTESIAN_POINT ( 'NONE',  ( 4.458734124999998549, 6.270833334698928674, -2.574251347313721627 ) ) ;
#37137=VERTEX_POINT ( 'NONE', #4988 ) ;
#37138=CARTESIAN_POINT ( 'NONE',  ( 9.457646018065525792E-16, -68.06249999863440792, 5.148502694627439702 ) ) ;
#37140=CARTESIAN_POINT ( 'NONE',  ( -2.229367062500000163, 5.520833334698927786, -3.861377020970580443 ) ) ;
#37141=CARTESIAN_POINT ( 'NONE',  ( -1.339745962155497683, -42.20534180126147561, -5.000000000000066613 ) ) ;
#37142=CARTESIAN_POINT ( 'NONE',  ( 4.458734124999999437, -61.06249999863440081, -5.460374474430324690E-16 ) ) ;
#37143=CARTESIAN_POINT ( 'NONE',  ( 5.000000000000000000, -17.37499999726881583, -6.123233995736766282E-16 ) ) ;
#37144=LINE ( 'NONE', #37767, #60461 ) ;
#37146=CARTESIAN_POINT ( 'NONE',  ( -2.499999999999996447, -83.70833333060214443, 4.330127018922195425 ) ) ;
#37147=CARTESIAN_POINT ( 'NONE',  ( -3.152548672688508926E-16, -35.56249999863440792, -5.148502694627439702 ) ) ;
#37148=CARTESIAN_POINT ( 'NONE',  ( -4.458734124999997661, -21.47916666530107221, 2.574251347313722516 ) ) ;
#37150=CARTESIAN_POINT ( 'NONE',  ( -6.972266317189433020E-16, -61.25000000000000000, -5.000000000000000000 ) ) ;
#37151=CARTESIAN_POINT ( 'NONE',  ( -2.499999999999996447, 29.16666666666666785, 4.330127018922195425 ) ) ;
#37153=ORIENTED_EDGE ( 'NONE', *, *, #12228, .T. ) ;
#37154=CARTESIAN_POINT ( 'NONE',  ( 4.458734124999998549, -104.9791666653010651, -2.574251347313721627 ) ) ;
#37156=CARTESIAN_POINT ( 'NONE',  ( -4.458734124999998549, -30.22916666530106866, 2.574251347313722516 ) ) ;
#37157=CARTESIAN_POINT ( 'NONE',  ( 5.000000000000000000, -63.37499999726880873, -6.123233995736766282E-16 ) ) ;
#37161=CARTESIAN_POINT ( 'NONE',  ( -4.458734124999999437, -27.39583333196774007, -2.574251347313719407 ) ) ;
#37162=CARTESIAN_POINT ( 'NONE',  ( 2.229367062500001939, -72.22916666530107932, 3.861377020970579999 ) ) ;
#37163=LINE ( 'NONE', #26550, #17181 ) ;
#37165=CARTESIAN_POINT ( 'NONE',  ( -4.999999999999998224, -32.91666666666666430, 2.886751345948131764 ) ) ;
#37167=CARTESIAN_POINT ( 'NONE',  ( 5.000000000000000000, -17.41666666666666430, -2.886751345948129988 ) ) ;
#37170=CARTESIAN_POINT ( 'NONE',  ( 6.123233995736766282E-16, -120.0000000000000000, -5.000000000000000000 ) ) ;
#37173=FACE_OUTER_BOUND ( 'NONE', #29785, .T. ) ;
#37177=CARTESIAN_POINT ( 'NONE',  ( 1.975475456537005874E-15, -92.74999999999998579, 5.000000000000000000 ) ) ;
#37178=CARTESIAN_POINT ( 'NONE',  ( 5.000000000000000000, -87.37499999726880162, -6.123233995736766282E-16 ) ) ;
#37180=ORIENTED_EDGE ( 'NONE', *, *, #14593, .F. ) ;
#37181=FACE_OUTER_BOUND ( 'NONE', #46755, .T. ) ;
#37186=( BOUNDED_CURVE ( )  B_SPLINE_CURVE ( 2, ( #42769, #48851, #4792, #23793, #62413, #53684, #53055, #19585, #58823 ),
 .UNSPECIFIED., .F., .F. ) 
 B_SPLINE_CURVE_WITH_KNOTS ( ( 3, 2, 2, 2, 3 ),
 ( 0.1196428571428571480, 0.1202380952380952411, 0.1214285714285714274, 0.1226190476190476136, 0.1232142857142857206 ),
 .UNSPECIFIED. ) 
 CURVE ( )  GEOMETRIC_REPRESENTATION_ITEM ( )  RATIONAL_B_SPLINE_CURVE ( ( 0.9330127018922192983, 0.9330127018922200755, 1.000000000000000000, 0.8660254037844387076, 1.000000000000000000, 0.8660254037844387076, 1.000000000000000000, 0.9330127018922185211, 0.9330127018922192983 ) ) 
 REPRESENTATION_ITEM ( '' )  );
#37188=VERTEX_POINT ( 'NONE', #54522 ) ;
#37190=ORIENTED_EDGE ( 'NONE', *, *, #28594, .T. ) ;
#37191=CARTESIAN_POINT ( 'NONE',  ( -6.972266317189433020E-16, -53.24999999999999289, -5.000000000000000000 ) ) ;
#37193=CARTESIAN_POINT ( 'NONE',  ( -2.500000000000000444, -51.04166666393547303, -4.330127018922193649 ) ) ;
#37198=CARTESIAN_POINT ( 'NONE',  ( 4.458734124999998549, -81.72916666530106511, -2.574251347313721627 ) ) ;
#37199=CARTESIAN_POINT ( 'NONE',  ( -4.458734124999998549, 24.77083333469893134, 2.574251347313722516 ) ) ;
#37202=CARTESIAN_POINT ( 'NONE',  ( 1.339745962155612702, -69.16965819600731891, -5.000000000000000000 ) ) ;
#37207=CARTESIAN_POINT ( 'NONE',  ( -6.972266317189433020E-16, -83.24999999999998579, -5.000000000000000000 ) ) ;
#37209=CARTESIAN_POINT ( 'NONE',  ( 9.457646018065525792E-16, -53.06249999863440792, 5.148502694627439702 ) ) ;
#37211=CARTESIAN_POINT ( 'NONE',  ( -2.229367062499996610, 26.85416666803225993, 3.861377020970582219 ) ) ;
#37212=CARTESIAN_POINT ( 'NONE',  ( 5.000000000000000000, -105.4166666666666572, -2.886751345948129988 ) ) ;
#37214=CARTESIAN_POINT ( 'NONE',  ( -2.229367062499996610, -43.39583333196773651, 3.861377020970582219 ) ) ;
#37215=CARTESIAN_POINT ( 'NONE',  ( -2.500000000000000444, -1.041666663935479686, -4.330127018922193649 ) ) ;
#37219=CARTESIAN_POINT ( 'NONE',  ( -4.458734124999999437, -102.3124999986344079, 0.000000000000000000 ) ) ;
#37220=CARTESIAN_POINT ( 'NONE',  ( 2.229367062499998831, -6.895833331967741842, -3.861377020970580887 ) ) ;
#37221=ORIENTED_EDGE ( 'NONE', *, *, #16123, .T. ) ;
#37222=CARTESIAN_POINT ( 'NONE',  ( -2.499999999999996447, -85.70833333060214443, 4.330127018922195425 ) ) ;
#37223=CARTESIAN_POINT ( 'NONE',  ( -2.229367062499996610, -95.14583333196773651, 3.861377020970582219 ) ) ;
#37225=CARTESIAN_POINT ( 'NONE',  ( 4.458734124999999437, -85.06249999863439371, -5.460374474430324690E-16 ) ) ;
#37229=CARTESIAN_POINT ( 'NONE',  ( -2.229367062500000163, -13.47916666530107221, -3.861377020970580443 ) ) ;
#37230=CARTESIAN_POINT ( 'NONE',  ( -4.458734124999999437, 17.35416666803225993, -2.574251347313719407 ) ) ;
#37231=CARTESIAN_POINT ( 'NONE',  ( 4.458734125000000326, -55.14583333196773651, 2.574251347313718519 ) ) ;
#37236=ORIENTED_EDGE ( 'NONE', *, *, #49609, .F. ) ;
#37238=( BOUNDED_CURVE ( )  B_SPLINE_CURVE ( 2, ( #21413, #25909, #36513, #12391, #51639, #22045, #45527, #21091, #7573 ),
 .UNSPECIFIED., .F., .F. ) 
 B_SPLINE_CURVE_WITH_KNOTS ( ( 3, 2, 2, 2, 3 ),
 ( 0.1517857142857143016, 0.1523809523809523947, 0.1535714285714285809, 0.1547619047619047672, 0.1553571428571428603 ),
 .UNSPECIFIED. ) 
 CURVE ( )  GEOMETRIC_REPRESENTATION_ITEM ( )  RATIONAL_B_SPLINE_CURVE ( ( 0.9330127018922194093, 0.9330127018922209636, 1.000000000000000000, 0.8660254037844387076, 1.000000000000000000, 0.8660254037844387076, 1.000000000000000000, 0.9330127018922194093, 0.9330127018922194093 ) ) 
 REPRESENTATION_ITEM ( '' )  );
#37240=CARTESIAN_POINT ( 'NONE',  ( 5.000000000000000888, 26.54166666939784847, 2.886751345948126879 ) ) ;
#37241=CARTESIAN_POINT ( 'NONE',  ( 2.229367062500001939, -77.97916666530106511, 3.861377020970579999 ) ) ;
#37242=CARTESIAN_POINT ( 'NONE',  ( -2.229367062500000163, 22.27083333469892423, -3.861377020970580443 ) ) ;
#37245=CARTESIAN_POINT ( 'NONE',  ( 0.000000000000000000, -120.0000000000000000, 5.000000000000000000 ) ) ;
#37247=CARTESIAN_POINT ( 'NONE',  ( -5.000000000000000000, -65.08333333333332860, -2.886751345948128211 ) ) ;
#37254=EDGE_CURVE ( 'NONE', #4410, #25201, #53563, .T. ) ;
#37255=CARTESIAN_POINT ( 'NONE',  ( -6.972266317189433020E-16, 4.749999999999999112, -5.000000000000000000 ) ) ;
#37264=CARTESIAN_POINT ( 'NONE',  ( -4.458734124999999437, -49.64583333196772941, -2.574251347313719407 ) ) ;
#37272=EDGE_CURVE ( 'NONE', #11599, #14930, #50684, .T. ) ;
#37275=CARTESIAN_POINT ( 'NONE',  ( 2.229367062500001939, -100.2291666653010651, 3.861377020970579999 ) ) ;
#37276=CARTESIAN_POINT ( 'NONE',  ( 1.975475456537005874E-15, -31.62499999726880873, 5.000000000000000000 ) ) ;
#37277=VERTEX_POINT ( 'NONE', #29737 ) ;
#37281=CARTESIAN_POINT ( 'NONE',  ( 9.457646018065525792E-16, -9.062499998634406140, 5.148502694627439702 ) ) ;
#37282=CARTESIAN_POINT ( 'NONE',  ( 4.458734125000000326, -96.14583333196773651, 2.574251347313718519 ) ) ;
#37284=CARTESIAN_POINT ( 'NONE',  ( -4.458734124999998549, -22.47916666530107577, 2.574251347313722516 ) ) ;
#37285=FACE_OUTER_BOUND ( 'NONE', #42699, .T. ) ;
#37289=CYLINDRICAL_SURFACE ( 'NONE', #63409, 5.000000000000000000 ) ;
#37291=CARTESIAN_POINT ( 'NONE',  ( 4.458734124999998549, 9.020833334698927786, -2.574251347313721627 ) ) ;
#37293=CARTESIAN_POINT ( 'NONE',  ( -5.000000000000000000, -5.083333333333334814, -2.886751345948128211 ) ) ;
#37294=CARTESIAN_POINT ( 'NONE',  ( 2.500000000000002220, -66.54166666393547303, 4.330127018922192761 ) ) ;
#37295=CARTESIAN_POINT ( 'NONE',  ( 5.000000000000000000, -89.41666666666667140, -2.886751345948129988 ) ) ;
#37296=CARTESIAN_POINT ( 'NONE',  ( -2.229367062499996610, -26.14583333196773651, 3.861377020970582219 ) ) ;
#37297=LINE ( 'NONE', #42424, #3820 ) ;
#37298=CARTESIAN_POINT ( 'NONE',  ( -2.229367062499996610, -73.39583333196773651, 3.861377020970582219 ) ) ;
#37300=CARTESIAN_POINT ( 'NONE',  ( 1.339745962155612702, -79.16965819600730470, -5.000000000000000000 ) ) ;
#37302=CARTESIAN_POINT ( 'NONE',  ( -4.458734124999997661, 1.770833334698928008, 2.574251347313722516 ) ) ;
#37306=CARTESIAN_POINT ( 'NONE',  ( 4.458734124999998549, -70.72916666530107932, -2.574251347313721627 ) ) ;
#37308=CARTESIAN_POINT ( 'NONE',  ( -2.500000000000000444, -1.166666666666666519, -4.330127018922193649 ) ) ;
#37311=CARTESIAN_POINT ( 'NONE',  ( -3.152548672688508926E-16, -63.56249999863440792, -5.148502694627439702 ) ) ;
#37312=CARTESIAN_POINT ( 'NONE',  ( 1.060575238724906964E-15, -102.6249999972688158, 5.773502691896257311 ) ) ;
#37313=CARTESIAN_POINT ( 'NONE',  ( -6.972266317189433020E-16, -51.25000000000000000, -5.000000000000000000 ) ) ;
#37315=CARTESIAN_POINT ( 'NONE',  ( 9.457646018065525792E-16, -108.3124999986343937, 5.148502694627439702 ) ) ;
#37317=CARTESIAN_POINT ( 'NONE',  ( 1.060575238724906964E-15, -49.75000000000000000, 5.773502691896257311 ) ) ;
#37321=CARTESIAN_POINT ( 'NONE',  ( -4.458734124999998549, -110.2291666653010651, 2.574251347313722516 ) ) ;
#37329=ORIENTED_EDGE ( 'NONE', *, *, #18947, .F. ) ;
#37335=CARTESIAN_POINT ( 'NONE',  ( -4.458734124999999437, -37.56249999863440792, 0.000000000000000000 ) ) ;
#37344=AXIS2_PLACEMENT_3D ( 'NONE', #46052, #11947, #22574 ) ;
#37347=CARTESIAN_POINT ( 'NONE',  ( 2.229367062499998831, -82.89583333196773651, -3.861377020970580887 ) ) ;
#37349=ORIENTED_EDGE ( 'NONE', *, *, #21984, .T. ) ;
#37350=EDGE_CURVE ( 'NONE', #29768, #33407, #59671, .T. ) ;
#37351=CARTESIAN_POINT ( 'NONE',  ( -6.972266317189433020E-16, -95.12499999726880162, -5.000000000000000000 ) ) ;
#37354=CARTESIAN_POINT ( 'NONE',  ( -4.458734124999999437, -38.39583333196773651, -2.574251347313719407 ) ) ;
#37355=CARTESIAN_POINT ( 'NONE',  ( 9.457646018065525792E-16, -11.31249999863440792, 5.148502694627439702 ) ) ;
#37356=ORIENTED_EDGE ( 'NONE', *, *, #34199, .F. ) ;
#37359=CARTESIAN_POINT ( 'NONE',  ( 5.000000000000000000, 2.708333336064520314, -2.886751345948130876 ) ) ;
#37360=CARTESIAN_POINT ( 'NONE',  ( -4.458734124999999437, -5.645833331967740953, -2.574251347313719407 ) ) ;
#37365=CARTESIAN_POINT ( 'NONE',  ( 2.229367062499998831, 27.10416666803225993, -3.861377020970580887 ) ) ;
#37367=CARTESIAN_POINT ( 'NONE',  ( 4.458734124999999437, -88.81249999863439371, -5.460374474430324690E-16 ) ) ;
#37368=CARTESIAN_POINT ( 'NONE',  ( -4.458734124999998549, -11.22916666530106866, 2.574251347313722516 ) ) ;
#37369=ADVANCED_FACE ( 'NONE', ( #26763 ), #25566, .T. ) ;
#37370=CYLINDRICAL_SURFACE ( 'NONE', #36600, 5.000000000000000000 ) ;
#37372=CARTESIAN_POINT ( 'NONE',  ( 2.499999999999998668, -37.20833333060213732, -4.330127018922193649 ) ) ;
#37374=CARTESIAN_POINT ( 'NONE',  ( 4.458734124999999437, 23.18750000136559564, -5.460374474430324690E-16 ) ) ;
#37375=CARTESIAN_POINT ( 'NONE',  ( -4.999999999999998224, -94.91666666666667140, 2.886751345948131764 ) ) ;
#37377=CARTESIAN_POINT ( 'NONE',  ( 4.458734124999998549, -57.72916666530107221, -2.574251347313721627 ) ) ;
#37380=CARTESIAN_POINT ( 'NONE',  ( 2.500000000000002220, 13.33333333333333215, 4.330127018922192761 ) ) ;
#37382=CARTESIAN_POINT ( 'NONE',  ( -1.339745962155610925, -45.79465819873851729, 5.000000000000000000 ) ) ;
#37383=CARTESIAN_POINT ( 'NONE',  ( 4.458734124999998549, -49.72916666530106511, -2.574251347313721627 ) ) ;
#37384=CARTESIAN_POINT ( 'NONE',  ( -3.535250795749689387E-16, -85.12499999726881583, -5.773502691896257311 ) ) ;
#37389=CARTESIAN_POINT ( 'NONE',  ( 9.457646018065525792E-16, -88.31249999863439371, 5.148502694627439702 ) ) ;
#37391=CARTESIAN_POINT ( 'NONE',  ( 5.000000000000000000, -34.50000000000000000, -6.123233995736766282E-16 ) ) ;
#37392=CARTESIAN_POINT ( 'NONE',  ( 5.000000000000000000, 8.625000002731184168, -6.123233995736766282E-16 ) ) ;
#37393=VERTEX_POINT ( 'NONE', #22259 ) ;
#37395=ORIENTED_EDGE ( 'NONE', *, *, #39355, .T. ) ;
#37396=CARTESIAN_POINT ( 'NONE',  ( -2.229367062499996610, -97.14583333196773651, 3.861377020970582219 ) ) ;
#37397=CARTESIAN_POINT ( 'NONE',  ( 4.458734125000001214, 8.854166668032261711, 2.574251347313718519 ) ) ;
#37398=CARTESIAN_POINT ( 'NONE',  ( -4.999999999999999112, 17.20833333606451987, 2.886751345948131764 ) ) ;
#37399=CARTESIAN_POINT ( 'NONE',  ( -5.000000000000000000, -28.87499999726881228, 0.000000000000000000 ) ) ;
#37403=CARTESIAN_POINT ( 'NONE',  ( 2.499999999999998668, -79.33333333333332860, -4.330127018922193649 ) ) ;
#37405=ADVANCED_FACE ( 'NONE', ( #51530 ), #41858, .T. ) ;
#37408=CARTESIAN_POINT ( 'NONE',  ( 1.975475456537005874E-15, -63.74999999999998579, 5.000000000000000000 ) ) ;
#37413=CARTESIAN_POINT ( 'NONE',  ( -6.972266317189433020E-16, 13.74999999999999822, -5.000000000000000000 ) ) ;
#37414=( BOUNDED_CURVE ( )  B_SPLINE_CURVE ( 2, ( #47976, #18707, #28981, #38332, #38630, #63106, #33510, #53127, #32560 ),
 .UNSPECIFIED., .F., .F. ) 
 B_SPLINE_CURVE_WITH_KNOTS ( ( 3, 2, 2, 2, 3 ),
 ( 0.8696428571428571619, 0.8702380952380952550, 0.8714285714285714413, 0.8726190476190476275, 0.8732142857142857206 ),
 .UNSPECIFIED. ) 
 CURVE ( )  GEOMETRIC_REPRESENTATION_ITEM ( )  RATIONAL_B_SPLINE_CURVE ( ( 0.9330127018922194093, 0.9330127018922194093, 1.000000000000000000, 0.8660254037844387076, 1.000000000000000000, 0.8660254037844387076, 1.000000000000000000, 0.9330127018922194093, 0.9330127018922194093 ) ) 
 REPRESENTATION_ITEM ( '' )  );
#37415=CARTESIAN_POINT ( 'NONE',  ( -2.229367062499996610, -17.39583333196773651, 3.861377020970582219 ) ) ;
#37416=CARTESIAN_POINT ( 'NONE',  ( 1.975475456537005874E-15, -107.6249999972687874, 5.000000000000000000 ) ) ;
#37425=CARTESIAN_POINT ( 'NONE',  ( 1.339745962155612702, -85.16965819600733312, -5.000000000000000000 ) ) ;
#37426=ADVANCED_FACE ( 'NONE', ( #7153 ), #7781, .T. ) ;
#37427=ORIENTED_EDGE ( 'NONE', *, *, #22815, .F. ) ;
#37428=CARTESIAN_POINT ( 'NONE',  ( 2.229367062500001939, -67.22916666530106511, 3.861377020970579999 ) ) ;
#37439=CARTESIAN_POINT ( 'NONE',  ( 9.457646018065525792E-16, 7.937500001365594748, 5.148502694627439702 ) ) ;
#37442=CARTESIAN_POINT ( 'NONE',  ( 2.499999999999998668, -108.2083333306021444, -4.330127018922193649 ) ) ;
#37443=CYLINDRICAL_SURFACE ( 'NONE', #38733, 5.000000000000000000 ) ;
#37444=ORIENTED_EDGE ( 'NONE', *, *, #5255, .F. ) ;
#37445=CARTESIAN_POINT ( 'NONE',  ( -2.229367062499996610, -72.14583333196773651, 3.861377020970582219 ) ) ;
#37447=CARTESIAN_POINT ( 'NONE',  ( -2.229367062499996610, 6.854166668032259935, 3.861377020970582219 ) ) ;
#37449=CARTESIAN_POINT ( 'NONE',  ( -2.229367062500000163, -60.72916666530106511, -3.861377020970580443 ) ) ;
#37450=CARTESIAN_POINT ( 'NONE',  ( 2.500000000000002220, -17.54166666393547658, 4.330127018922192761 ) ) ;
#37451=DIRECTION ( 'NONE',  ( -0.000000000000000000, 1.000000000000000000, -0.000000000000000000 ) ) ;
#37454=CARTESIAN_POINT ( 'NONE',  ( 4.458734124999998549, -40.72916666530107221, -2.574251347313721627 ) ) ;
#37455=CARTESIAN_POINT ( 'NONE',  ( -4.458734124999997661, -19.47916666530107221, 2.574251347313722516 ) ) ;
#37456=ORIENTED_EDGE ( 'NONE', *, *, #5153, .T. ) ;
#37458=FACE_OUTER_BOUND ( 'NONE', #3272, .T. ) ;
#37459=CARTESIAN_POINT ( 'NONE',  ( 2.229367062500001939, -108.9791666653010651, 3.861377020970579999 ) ) ;
#37461=VERTEX_POINT ( 'NONE', #16791 ) ;
#37462=CARTESIAN_POINT ( 'NONE',  ( 4.458734125000001214, -109.1458333319677365, 2.574251347313718519 ) ) ;
#37463=CARTESIAN_POINT ( 'NONE',  ( -4.458734124999999437, -34.31249999863440792, 0.000000000000000000 ) ) ;
#37464=CARTESIAN_POINT ( 'NONE',  ( 2.500000000000002220, -67.54166666393547303, 4.330127018922192761 ) ) ;
#37467=CARTESIAN_POINT ( 'NONE',  ( 4.458734125000000326, -26.89583333196774007, 2.574251347313718519 ) ) ;
#37468=CARTESIAN_POINT ( 'NONE',  ( -4.458734124999997661, -69.47916666530107932, 2.574251347313722516 ) ) ;
#37472=CARTESIAN_POINT ( 'NONE',  ( -4.999999999999999112, -15.91666666666666963, 2.886751345948131764 ) ) ;
#37474=ORIENTED_EDGE ( 'NONE', *, *, #53074, .F. ) ;
#37475=CARTESIAN_POINT ( 'NONE',  ( -1.339745962155613812, -82.20534180126146850, -5.000000000000000000 ) ) ;
#37479=LINE ( 'NONE', #41651, #12078 ) ;
#37480=VECTOR ( 'NONE', #50069, 1000.000000000000000 ) ;
#37483=CARTESIAN_POINT ( 'NONE',  ( 1.339745962155615144, -87.58034179853028434, 4.999999999999999112 ) ) ;
#37485=ORIENTED_EDGE ( 'NONE', *, *, #27238, .F. ) ;
#37487=VERTEX_POINT ( 'NONE', #17744 ) ;
#37495=CARTESIAN_POINT ( 'NONE',  ( -5.000000000000000000, -102.8749999972688158, 0.000000000000000000 ) ) ;
#37497=ADVANCED_FACE ( 'NONE', ( #36409 ), #56991, .T. ) ;
#37499=CARTESIAN_POINT ( 'NONE',  ( -1.339745962155613812, -51.08034179853027723, -5.000000000000000000 ) ) ;
#37504=ADVANCED_FACE ( 'NONE', ( #53096 ), #19305, .T. ) ;
#37505=CARTESIAN_POINT ( 'NONE',  ( -2.229367062500000163, -84.47916666530107932, -3.861377020970580443 ) ) ;
#37506=CARTESIAN_POINT ( 'NONE',  ( -2.229367062500000163, 25.52083333469892779, -3.861377020970580443 ) ) ;
#37512=CYLINDRICAL_SURFACE ( 'NONE', #2864, 5.000000000000000000 ) ;
#37514=CARTESIAN_POINT ( 'NONE',  ( 5.000000000000000000, 4.583333333333331261, -2.886751345948130876 ) ) ;
#37515=CARTESIAN_POINT ( 'NONE',  ( 2.229367062500001939, -53.97916666530107221, 3.861377020970579999 ) ) ;
#37517=CARTESIAN_POINT ( 'NONE',  ( 9.457646018065525792E-16, 24.93750000136559564, 5.148502694627439702 ) ) ;
#37518=CARTESIAN_POINT ( 'NONE',  ( 5.000000000000000888, -106.5833333333333286, 2.886751345948126879 ) ) ;
#37520=CARTESIAN_POINT ( 'NONE',  ( 9.457646018065525792E-16, -44.31249999863440081, 5.148502694627439702 ) ) ;
#37521=CARTESIAN_POINT ( 'NONE',  ( -4.999999999999999112, -4.791666663935479242, 2.886751345948131764 ) ) ;
#37525=CARTESIAN_POINT ( 'NONE',  ( -4.458734124999997661, -103.2291666653010509, 2.574251347313722516 ) ) ;
#37526=CARTESIAN_POINT ( 'NONE',  ( -4.458734124999999437, -5.562499998634402587, 0.000000000000000000 ) ) ;
#37528=DIRECTION ( 'NONE',  ( -0.000000000000000000, 1.000000000000000000, -0.000000000000000000 ) ) ;
#37529=CARTESIAN_POINT ( 'NONE',  ( 9.457646018065525792E-16, -93.06249999863440792, 5.148502694627439702 ) ) ;
#37531=CARTESIAN_POINT ( 'NONE',  ( 2.229367062499998831, -90.89583333196773651, -3.861377020970580887 ) ) ;
#37533=FACE_OUTER_BOUND ( 'NONE', #54707, .T. ) ;
#37536=CARTESIAN_POINT ( 'NONE',  ( 2.229367062500001939, -10.97916666530107044, 3.861377020970579999 ) ) ;
#37538=CARTESIAN_POINT ( 'NONE',  ( -3.152548672688508926E-16, 14.18750000136559386, -5.148502694627439702 ) ) ;
#37539=CARTESIAN_POINT ( 'NONE',  ( 4.458734124999998549, -55.97916666530107932, -2.574251347313721627 ) ) ;
#37542=CARTESIAN_POINT ( 'NONE',  ( 1.975475456537005874E-15, -109.6249999972688158, 5.000000000000000000 ) ) ;
#37546=CARTESIAN_POINT ( 'NONE',  ( 2.499999999999998668, -76.33333333333334281, -4.330127018922193649 ) ) ;
#37547=CARTESIAN_POINT ( 'NONE',  ( -4.458734124999999437, -80.39583333196772230, -2.574251347313719407 ) ) ;
#37548=CARTESIAN_POINT ( 'NONE',  ( 4.458734125000001214, 21.85416666803225993, 2.574251347313718519 ) ) ;
#37550=EDGE_CURVE ( 'NONE', #27142, #8539, #33396, .T. ) ;
#37551=CARTESIAN_POINT ( 'NONE',  ( -2.499999999999996447, -47.83333333333332149, 4.330127018922195425 ) ) ;
#37554=CARTESIAN_POINT ( 'NONE',  ( 1.060575238724906964E-15, -69.75000000000000000, 5.773502691896257311 ) ) ;
#37559=CARTESIAN_POINT ( 'NONE',  ( -1.339745962155497683, -90.20534180126148271, -5.000000000000066613 ) ) ;
#37560=CARTESIAN_POINT ( 'NONE',  ( -5.000000000000000000, -108.8749999972688016, 0.000000000000000000 ) ) ;
#37563=CARTESIAN_POINT ( 'NONE',  ( -4.999999999999998224, 5.083333333333332149, 2.886751345948131764 ) ) ;
#37573=CARTESIAN_POINT ( 'NONE',  ( -2.229367062499996610, -50.39583333196772941, 3.861377020970582219 ) ) ;
#37582=CARTESIAN_POINT ( 'NONE',  ( 2.229367062499998831, -101.8958333319677365, -3.861377020970580887 ) ) ;
#37583=CARTESIAN_POINT ( 'NONE',  ( 6.158835246850667461E-14, -2.250000000000001776, -4.999999999999999112 ) ) ;
#37584=ORIENTED_EDGE ( 'NONE', *, *, #7679, .F. ) ;
#37588=CARTESIAN_POINT ( 'NONE',  ( -2.229367062499996610, -6.145833331967740953, 3.861377020970582219 ) ) ;
#37589=CARTESIAN_POINT ( 'NONE',  ( -2.229367062500000163, -96.72916666530105090, -3.861377020970580443 ) ) ;
#37591=CARTESIAN_POINT ( 'NONE',  ( -4.458734124999999437, -26.64583333196773651, -2.574251347313719407 ) ) ;
#37592=DIRECTION ( 'NONE',  ( 0.000000000000000000, 0.000000000000000000, 1.000000000000000000 ) ) ;
#37595=CARTESIAN_POINT ( 'NONE',  ( -6.972266317189433020E-16, -21.12499999726881228, -5.000000000000000000 ) ) ;
#37596=DIRECTION ( 'NONE',  ( -0.000000000000000000, 1.000000000000000000, -0.000000000000000000 ) ) ;
#37598=CARTESIAN_POINT ( 'NONE',  ( 2.229367062499998831, 9.104166668032261711, -3.861377020970580887 ) ) ;
#37601=CARTESIAN_POINT ( 'NONE',  ( -6.972266317189433020E-16, -81.24999999999998579, -5.000000000000000000 ) ) ;
#37602=DIRECTION ( 'NONE',  ( 0.000000000000000000, 0.000000000000000000, 1.000000000000000000 ) ) ;
#37603=CARTESIAN_POINT ( 'NONE',  ( 1.060575238724906964E-15, -92.74999999999998579, 5.773502691896257311 ) ) ;
#37604=CARTESIAN_POINT ( 'NONE',  ( -2.229367062499996610, -25.14583333196773651, 3.861377020970582219 ) ) ;
#37606=CARTESIAN_POINT ( 'NONE',  ( 2.229367062499998831, -70.89583333196773651, -3.861377020970580887 ) ) ;
#37607=ADVANCED_FACE ( 'NONE', ( #43743 ), #38601, .T. ) ;
#37612=CARTESIAN_POINT ( 'NONE',  ( 4.458734124999998549, 5.270833334698926897, -2.574251347313721627 ) ) ;
#37613=CARTESIAN_POINT ( 'NONE',  ( -4.999999999999998224, -62.79166666393546592, 2.886751345948131764 ) ) ;
#37614=CYLINDRICAL_SURFACE ( 'NONE', #47977, 5.000000000000000000 ) ;
#37616=CARTESIAN_POINT ( 'NONE',  ( 2.229367062499998831, -71.64583333196773651, -3.861377020970580887 ) ) ;
#37618=CARTESIAN_POINT ( 'NONE',  ( -5.000000000000000000, -5.999999999999998224, 0.000000000000000000 ) ) ;
#37621=CARTESIAN_POINT ( 'NONE',  ( 4.458734124999999437, -61.81249999863440081, -5.460374474430324690E-16 ) ) ;
#37622=CARTESIAN_POINT ( 'NONE',  ( -2.500000000000000444, -101.0416666639354588, -4.330127018922193649 ) ) ;
#37626=CARTESIAN_POINT ( 'NONE',  ( -4.458734124999999437, -108.5624999986343937, 0.000000000000000000 ) ) ;
#37628=CARTESIAN_POINT ( 'NONE',  ( -5.000000000000000000, -53.99999999999999289, 0.000000000000000000 ) ) ;
#37630=DIRECTION ( 'NONE',  ( 0.8660254037844415942, -0.000000000000000000, 0.4999999999999948930 ) ) ;
#37633=( BOUNDED_CURVE ( )  B_SPLINE_CURVE ( 2, ( #50659, #6598, #26213, #5969, #60326, #41001, #45833, #5642, #505 ),
 .UNSPECIFIED., .F., .F. ) 
 B_SPLINE_CURVE_WITH_KNOTS ( ( 3, 2, 2, 2, 3 ),
 ( 0.6660714285714285365, 0.6666666666666666297, 0.6678571428571428159, 0.6690476190476190022, 0.6696428571428570953 ),
 .UNSPECIFIED. ) 
 CURVE ( )  GEOMETRIC_REPRESENTATION_ITEM ( )  RATIONAL_B_SPLINE_CURVE ( ( 0.9330127018922194093, 0.9330127018922194093, 1.000000000000000000, 0.8660254037844387076, 1.000000000000000000, 0.8660254037844387076, 1.000000000000000000, 0.9330127018922194093, 0.9330127018922194093 ) ) 
 REPRESENTATION_ITEM ( '' )  );
#37638=CARTESIAN_POINT ( 'NONE',  ( -6.972266317189433020E-16, -5.124999997268812280, -5.000000000000000000 ) ) ;
#37641=EDGE_LOOP ( 'NONE', ( #12971, #34314, #18856, #34073 ) ) ;
#37648=CARTESIAN_POINT ( 'NONE',  ( 4.458734125000001214, -38.14583333196773651, 2.574251347313718519 ) ) ;
#37649=CARTESIAN_POINT ( 'NONE',  ( -1.339745962155613812, -11.08034179853029322, -5.000000000000000000 ) ) ;
#37652=CARTESIAN_POINT ( 'NONE',  ( -5.000000000000000000, -30.08333333333332860, -2.886751345948128211 ) ) ;
#37654=VECTOR ( 'NONE', #29784, 1000.000000000000000 ) ;
#37656=VECTOR ( 'NONE', #183, 1000.000000000000000 ) ;
#37658=CARTESIAN_POINT ( 'NONE',  ( 5.000000000000000000, -26.41666666666666430, -2.886751345948130876 ) ) ;
#37659=CARTESIAN_POINT ( 'NONE',  ( 4.458734125000001214, -82.14583333196772230, 2.574251347313718519 ) ) ;
#37668=CARTESIAN_POINT ( 'NONE',  ( 4.458734124999998549, -12.97916666530107044, -2.574251347313721627 ) ) ;
#37671=DIRECTION ( 'NONE',  ( 0.000000000000000000, 0.000000000000000000, 1.000000000000000000 ) ) ;
#37673=CARTESIAN_POINT ( 'NONE',  ( 2.229367062500001939, 24.77083333469892779, 3.861377020970579999 ) ) ;
#37675=CARTESIAN_POINT ( 'NONE',  ( 2.229367062500001939, -92.97916666530106511, 3.861377020970579999 ) ) ;
#37676=CARTESIAN_POINT ( 'NONE',  ( -1.339745962155613812, -68.20534180126148271, -5.000000000000000000 ) ) ;
#37677=CARTESIAN_POINT ( 'NONE',  ( -2.480964764533239819E-13, -95.62499999726883004, 5.000000000000000000 ) ) ;
#37678=CARTESIAN_POINT ( 'NONE',  ( 4.458734125000001214, -6.895833331967734736, 2.574251347313718519 ) ) ;
#37680=CARTESIAN_POINT ( 'NONE',  ( 2.499999999999998668, -51.33333333333332860, -4.330127018922193649 ) ) ;
#37683=CARTESIAN_POINT ( 'NONE',  ( 2.499999999999998668, -36.20833333060213732, -4.330127018922193649 ) ) ;
#37684=CARTESIAN_POINT ( 'NONE',  ( 5.000000000000000000, -49.37499999726880873, -6.123233995736766282E-16 ) ) ;
#37685=CARTESIAN_POINT ( 'NONE',  ( -4.458734124999997661, 21.77083333469892779, 2.574251347313722516 ) ) ;
#37686=CARTESIAN_POINT ( 'NONE',  ( -6.972266317189433020E-16, -4.249999999999997335, -5.000000000000000000 ) ) ;
#37688=CARTESIAN_POINT ( 'NONE',  ( -4.458734124999999437, -57.39583333196773651, -2.574251347313719407 ) ) ;
#37691=CARTESIAN_POINT ( 'NONE',  ( -4.999999999999999112, 11.08333333333333393, 2.886751345948131764 ) ) ;
#37694=CARTESIAN_POINT ( 'NONE',  ( 4.458734124999999437, -45.81249999863440081, -5.460374474430324690E-16 ) ) ;
#37695=CARTESIAN_POINT ( 'NONE',  ( -5.000000000000000000, -85.87499999726880162, 0.000000000000000000 ) ) ;
#37702=EDGE_CURVE ( 'NONE', #6256, #28617, #33773, .T. ) ;
#37703=CARTESIAN_POINT ( 'NONE',  ( 2.229367062500001939, -91.22916666530106511, 3.861377020970579999 ) ) ;
#37705=CARTESIAN_POINT ( 'NONE',  ( 2.499999999999998668, -32.33333333333332860, -4.330127018922193649 ) ) ;
#37710=CARTESIAN_POINT ( 'NONE',  ( 4.458734124999998549, -98.72916666530105090, -2.574251347313721627 ) ) ;
#37711=CARTESIAN_POINT ( 'NONE',  ( 2.229367062499998831, 9.104166668032261711, -3.861377020970580887 ) ) ;
#37712=CARTESIAN_POINT ( 'NONE',  ( -2.500000000000000444, 9.958333336064519870, -4.330127018922193649 ) ) ;
#37713=CARTESIAN_POINT ( 'NONE',  ( -1.339745962155727277, -59.79465819873853150, 4.999999999999933387 ) ) ;
#37719=CARTESIAN_POINT ( 'NONE',  ( -3.535250795749689387E-16, -80.25000000000000000, -5.773502691896257311 ) ) ;
#37721=DIRECTION ( 'NONE',  ( -0.000000000000000000, 1.000000000000000000, -0.000000000000000000 ) ) ;
#37722=CARTESIAN_POINT ( 'NONE',  ( 2.500000000000002220, -63.66666666666666430, 4.330127018922192761 ) ) ;
#37725=CARTESIAN_POINT ( 'NONE',  ( 1.975475456537005874E-15, -75.62499999726880162, 5.000000000000000000 ) ) ;
#37727=CARTESIAN_POINT ( 'NONE',  ( -2.229367062500000163, -20.72916666530107221, -3.861377020970580443 ) ) ;
#37728=CARTESIAN_POINT ( 'NONE',  ( 5.000000000000000000, -107.2916666639354730, -2.886751345948130876 ) ) ;
#37736=ORIENTED_EDGE ( 'NONE', *, *, #14103, .T. ) ;
#37739=EDGE_LOOP ( 'NONE', ( #52394, #34060, #8072, #40005 ) ) ;
#37740=CARTESIAN_POINT ( 'NONE',  ( -4.458734124999999437, -66.64583333196773651, -2.574251347313719407 ) ) ;
#37741=CARTESIAN_POINT ( 'NONE',  ( 1.975475456537005874E-15, -7.624999997268812280, 5.000000000000000000 ) ) ;
#37743=ORIENTED_EDGE ( 'NONE', *, *, #34105, .F. ) ;
#37749=EDGE_LOOP ( 'NONE', ( #8901, #52056, #7472, #51939 ) ) ;
#37750=CARTESIAN_POINT ( 'NONE',  ( 1.975475456537005874E-15, -54.74999999999999289, 5.000000000000000000 ) ) ;
#37751=VECTOR ( 'NONE', #25243, 1000.000000000000000 ) ;
#37752=CARTESIAN_POINT ( 'NONE',  ( 2.229367062499998831, 10.35416666803225993, -3.861377020970580887 ) ) ;
#37757=ORIENTED_EDGE ( 'NONE', *, *, #42923, .T. ) ;
#37758=CARTESIAN_POINT ( 'NONE',  ( -4.458734124999999437, -77.31249999863440792, 0.000000000000000000 ) ) ;
#37760=CARTESIAN_POINT ( 'NONE',  ( 4.458734124999998549, 8.270833334698926009, -2.574251347313721627 ) ) ;
#37762=EDGE_CURVE ( 'NONE', #21496, #13829, #5029, .T. ) ;
#37765=CARTESIAN_POINT ( 'NONE',  ( -4.458734124999998549, -62.47916666530106511, 2.574251347313722516 ) ) ;
#37766=CARTESIAN_POINT ( 'NONE',  ( 2.500000000000002220, -22.54166666393548013, 4.330127018922192761 ) ) ;
#37767=CARTESIAN_POINT ( 'NONE',  ( 0.000000000000000000, -120.0000000000000000, 5.000000000000000000 ) ) ;
#37768=CARTESIAN_POINT ( 'NONE',  ( 5.000000000000000000, -28.29166666393548013, -2.886751345948130876 ) ) ;
#37770=CARTESIAN_POINT ( 'NONE',  ( -5.000000000000000000, -83.95833333060214443, -2.886751345948128211 ) ) ;
#37772=CARTESIAN_POINT ( 'NONE',  ( 9.457646018065525792E-16, -39.06249999863440081, 5.148502694627439702 ) ) ;
#37773=CARTESIAN_POINT ( 'NONE',  ( -2.229367062499996610, -27.39583333196774007, 3.861377020970582219 ) ) ;
#37775=CARTESIAN_POINT ( 'NONE',  ( 2.499999999999998668, 29.66666666666666430, -4.330127018922193649 ) ) ;
#37778=CARTESIAN_POINT ( 'NONE',  ( 2.229367062500001939, -110.2291666653010651, 3.861377020970579999 ) ) ;
#37779=CARTESIAN_POINT ( 'NONE',  ( -3.152548672688508926E-16, -29.56249999863440436, -5.148502694627439702 ) ) ;
#37780=CARTESIAN_POINT ( 'NONE',  ( -5.000000000000000000, -66.87499999726881583, 0.000000000000000000 ) ) ;
#37781=ADVANCED_FACE ( 'NONE', ( #29903 ), #25735, .T. ) ;
#37784=CARTESIAN_POINT ( 'NONE',  ( -2.229367062500000163, -31.47916666530107577, -3.861377020970580443 ) ) ;
#37785=EDGE_CURVE ( 'NONE', #36016, #6026, #42407, .T. ) ;
#37786=CARTESIAN_POINT ( 'NONE',  ( 2.229367062500001939, -71.22916666530107932, 3.861377020970579999 ) ) ;
#37790=CARTESIAN_POINT ( 'NONE',  ( 5.000000000000000000, -5.374999997268811391, -6.123233995736766282E-16 ) ) ;
#37791=CARTESIAN_POINT ( 'NONE',  ( 5.000000000000000000, -18.50000000000000355, -6.123233995736766282E-16 ) ) ;
#37794=CARTESIAN_POINT ( 'NONE',  ( -5.000000000000000000, -82.08333333333332860, -2.886751345948128211 ) ) ;
#37796=( BOUNDED_CURVE ( )  B_SPLINE_CURVE ( 2, ( #57657, #32565, #52187, #17773, #46725, #32244, #22292, #27735, #23554 ),
 .UNSPECIFIED., .F., .F. ) 
 B_SPLINE_CURVE_WITH_KNOTS ( ( 3, 2, 2, 2, 3 ),
 ( 0.04107142857142857123, 0.04166666666666666435, 0.04285714285714285754, 0.04404761904761905073, 0.04464285714285714385 ),
 .UNSPECIFIED. ) 
 CURVE ( )  GEOMETRIC_REPRESENTATION_ITEM ( )  RATIONAL_B_SPLINE_CURVE ( ( 0.9330127018922194093, 0.9330127018922194093, 1.000000000000000000, 0.8660254037844387076, 1.000000000000000000, 0.8660254037844387076, 1.000000000000000000, 0.9330127018922194093, 0.9330127018922194093 ) ) 
 REPRESENTATION_ITEM ( '' )  );
#37797=AXIS2_PLACEMENT_3D ( 'NONE', #23914, #38083, #62222 ) ;
#37798=CARTESIAN_POINT ( 'NONE',  ( 1.060575238724906964E-15, 25.37500000273118417, 5.773502691896257311 ) ) ;
#37799=LINE ( 'NONE', #27503, #52490 ) ;
#37804=CARTESIAN_POINT ( 'NONE',  ( -5.000000000000000000, -51.87499999726881583, 0.000000000000000000 ) ) ;
#37807=ORIENTED_EDGE ( 'NONE', *, *, #49164, .T. ) ;
#37808=CYLINDRICAL_SURFACE ( 'NONE', #28415, 5.000000000000000000 ) ;
#37810=DIRECTION ( 'NONE',  ( -0.000000000000000000, 1.000000000000000000, -0.000000000000000000 ) ) ;
#37816=ORIENTED_EDGE ( 'NONE', *, *, #50866, .F. ) ;
#37817=CARTESIAN_POINT ( 'NONE',  ( -5.000000000000000000, -96.08333333333331439, -2.886751345948128211 ) ) ;
#37823=CARTESIAN_POINT ( 'NONE',  ( 2.229367062499998831, -83.64583333196773651, -3.861377020970580887 ) ) ;
#37824=CARTESIAN_POINT ( 'NONE',  ( 4.458734125000001214, 23.10416666803225993, 2.574251347313718519 ) ) ;
#37825=DIRECTION ( 'NONE',  ( -0.000000000000000000, 1.000000000000000000, -0.000000000000000000 ) ) ;
#37832=CARTESIAN_POINT ( 'NONE',  ( -2.500000000000000444, -83.16666666666667140, -4.330127018922193649 ) ) ;
#37834=( BOUNDED_CURVE ( )  B_SPLINE_CURVE ( 2, ( #12339, #42544, #17790, #32263, #37109, #51892, #47067, #27434, #37413 ),
 .UNSPECIFIED., .F., .F. ) 
 B_SPLINE_CURVE_WITH_KNOTS ( ( 3, 2, 2, 2, 3 ),
 ( 0.1125000000000000028, 0.1130952380952380959, 0.1142857142857142821, 0.1154761904761904823, 0.1160714285714285754 ),
 .UNSPECIFIED. ) 
 CURVE ( )  GEOMETRIC_REPRESENTATION_ITEM ( )  RATIONAL_B_SPLINE_CURVE ( ( 0.9330127018922194093, 0.9330127018922194093, 1.000000000000000000, 0.8660254037844387076, 1.000000000000000000, 0.8660254037844387076, 1.000000000000000000, 0.9330127018922194093, 0.9330127018922194093 ) ) 
 REPRESENTATION_ITEM ( '' )  );
#37836=CARTESIAN_POINT ( 'NONE',  ( -4.458734124999999437, -56.31249999863440081, 0.000000000000000000 ) ) ;
#37837=CARTESIAN_POINT ( 'NONE',  ( 0.000000000000000000, -120.0000000000000000, 5.000000000000000000 ) ) ;
#37838=CARTESIAN_POINT ( 'NONE',  ( -4.458734124999998549, 21.77083333469892779, 2.574251347313722516 ) ) ;
#37839=VECTOR ( 'NONE', #19175, 1000.000000000000000 ) ;
#37840=CARTESIAN_POINT ( 'NONE',  ( 5.000000000000000888, -42.58333333333334281, 2.886751345948126879 ) ) ;
#37841=CARTESIAN_POINT ( 'NONE',  ( 1.975475456537005874E-15, 1.375000002731185500, 5.000000000000000000 ) ) ;
#37843=CARTESIAN_POINT ( 'NONE',  ( -2.229367062499996610, -42.39583333196773651, 3.861377020970582219 ) ) ;
#37844=CARTESIAN_POINT ( 'NONE',  ( -5.000000000000000000, -5.958333330602148870, -2.886751345948128211 ) ) ;
#37848=CARTESIAN_POINT ( 'NONE',  ( 2.229367062500001939, -103.9791666653010651, 3.861377020970579999 ) ) ;
#37849=CARTESIAN_POINT ( 'NONE',  ( 9.457646018065525792E-16, -3.312499998634407916, 5.148502694627439702 ) ) ;
#37853=CARTESIAN_POINT ( 'NONE',  ( 4.458734125000001214, -91.89583333196773651, 2.574251347313718519 ) ) ;
#37855=CARTESIAN_POINT ( 'NONE',  ( 9.457646018065525792E-16, -94.31249999863440792, 5.148502694627439702 ) ) ;
#37856=EDGE_CURVE ( 'NONE', #37137, #12070, #11605, .T. ) ;
#37858=CARTESIAN_POINT ( 'NONE',  ( 2.229367062499998831, -13.64583333196774184, -3.861377020970580887 ) ) ;
#37859=CARTESIAN_POINT ( 'NONE',  ( -4.458734124999998549, 10.52083333469892779, 2.574251347313722516 ) ) ;
#37860=CARTESIAN_POINT ( 'NONE',  ( -3.152548672688508926E-16, -53.81249999863439371, -5.148502694627439702 ) ) ;
#37864=CARTESIAN_POINT ( 'NONE',  ( -6.972266317189433020E-16, -39.25000000000000000, -5.000000000000000000 ) ) ;
#37866=VERTEX_POINT ( 'NONE', #42100 ) ;
#37868=CARTESIAN_POINT ( 'NONE',  ( 0.000000000000000000, -120.0000000000000000, 0.000000000000000000 ) ) ;
#37869=EDGE_CURVE ( 'NONE', #42628, #46066, #46937, .T. ) ;
#37871=DIRECTION ( 'NONE',  ( -0.000000000000000000, 1.000000000000000000, -0.000000000000000000 ) ) ;
#37872=CARTESIAN_POINT ( 'NONE',  ( 2.229367062500001939, -79.97916666530106511, 3.861377020970579999 ) ) ;
#37873=CARTESIAN_POINT ( 'NONE',  ( -2.229367062500000163, 24.27083333469892779, -3.861377020970580443 ) ) ;
#37875=EDGE_CURVE ( 'NONE', #63081, #41892, #50815, .T. ) ;
#37876=DIRECTION ( 'NONE',  ( 0.000000000000000000, 0.000000000000000000, 1.000000000000000000 ) ) ;
#37877=LINE ( 'NONE', #52356, #51207 ) ;
#37879=CARTESIAN_POINT ( 'NONE',  ( 5.000000000000000888, -67.58333333333332860, 2.886751345948126879 ) ) ;
#37881=EDGE_LOOP ( 'NONE', ( #31229, #61418, #3496, #16884 ) ) ;
#37884=CARTESIAN_POINT ( 'NONE',  ( -6.972266317189433020E-16, -40.24999999999999289, -5.000000000000000000 ) ) ;
#37888=DIRECTION ( 'NONE',  ( -0.000000000000000000, 1.000000000000000000, -0.000000000000000000 ) ) ;
#37896=FACE_OUTER_BOUND ( 'NONE', #29509, .T. ) ;
#37897=CARTESIAN_POINT ( 'NONE',  ( 4.458734124999999437, -50.06249999863440792, -5.460374474430324690E-16 ) ) ;
#37899=CARTESIAN_POINT ( 'NONE',  ( -6.972266317189433020E-16, 9.875000002731185944, -5.000000000000000000 ) ) ;
#37900=EDGE_LOOP ( 'NONE', ( #17145, #12796, #31145, #26760 ) ) ;
#37904=VERTEX_POINT ( 'NONE', #51769 ) ;
#37907=CARTESIAN_POINT ( 'NONE',  ( -3.152548672688508926E-16, -101.8124999986344079, -5.148502694627439702 ) ) ;
#37908=ORIENTED_EDGE ( 'NONE', *, *, #40980, .F. ) ;
#37911=CARTESIAN_POINT ( 'NONE',  ( -2.500000000000000444, 0.9583333360645186483, -4.330127018922193649 ) ) ;
#37912=CARTESIAN_POINT ( 'NONE',  ( -2.229367062499996610, -7.145833331967735624, 3.861377020970582219 ) ) ;
#37914=CARTESIAN_POINT ( 'NONE',  ( 2.229367062499998831, -102.8958333319677365, -3.861377020970580887 ) ) ;
#37916=CARTESIAN_POINT ( 'NONE',  ( -4.458734124999998549, -26.47916666530107221, 2.574251347313722516 ) ) ;
#37920=LINE ( 'NONE', #23448, #11710 ) ;
#37921=CARTESIAN_POINT ( 'NONE',  ( -4.999999999999998224, -33.91666666666666430, 2.886751345948131764 ) ) ;
#37923=CARTESIAN_POINT ( 'NONE',  ( 4.458734124999998549, 8.020833334698926009, -2.574251347313721627 ) ) ;
#37924=ORIENTED_EDGE ( 'NONE', *, *, #5458, .T. ) ;
#37925=CARTESIAN_POINT ( 'NONE',  ( -4.999999999999998224, -4.916666666666666075, 2.886751345948131764 ) ) ;
#37927=CARTESIAN_POINT ( 'NONE',  ( 5.000000000000000000, -88.41666666666665719, -2.886751345948129988 ) ) ;
#37928=CARTESIAN_POINT ( 'NONE',  ( -2.229367062499996610, -24.14583333196773651, 3.861377020970582219 ) ) ;
#37930=CARTESIAN_POINT ( 'NONE',  ( -3.152548672688508926E-16, -75.81249999863440792, -5.148502694627439702 ) ) ;
#37933=CARTESIAN_POINT ( 'NONE',  ( -6.972266317189433020E-16, -79.12499999726881583, -5.000000000000000000 ) ) ;
#37935=CARTESIAN_POINT ( 'NONE',  ( 9.457646018065525792E-16, 2.937500001365594304, 5.148502694627439702 ) ) ;
#37936=CARTESIAN_POINT ( 'NONE',  ( -4.458734124999998549, 28.52083333469892423, 2.574251347313722516 ) ) ;
#37937=CARTESIAN_POINT ( 'NONE',  ( 2.229367062499998831, -36.89583333196773651, -3.861377020970580887 ) ) ;
#37940=CARTESIAN_POINT ( 'NONE',  ( -2.229367062500000163, -71.47916666530107932, -3.861377020970580443 ) ) ;
#37942=CARTESIAN_POINT ( 'NONE',  ( 5.000000000000000000, -8.416666666666669627, -2.886751345948129988 ) ) ;
#37945=CARTESIAN_POINT ( 'NONE',  ( 4.458734124999998549, -65.72916666530106511, -2.574251347313721627 ) ) ;
#37946=CARTESIAN_POINT ( 'NONE',  ( -5.000000000000000000, -101.9583333306021444, -2.886751345948128211 ) ) ;
#37950=CARTESIAN_POINT ( 'NONE',  ( -4.458734124999999437, -104.5624999986344079, 0.000000000000000000 ) ) ;
#37952=CARTESIAN_POINT ( 'NONE',  ( -4.999999999999999112, -54.91666666666667140, 2.886751345948131764 ) ) ;
#37953=CARTESIAN_POINT ( 'NONE',  ( 5.000000000000000000, -72.37499999726880162, -6.123233995736766282E-16 ) ) ;
#37955=ORIENTED_EDGE ( 'NONE', *, *, #38200, .F. ) ;
#37956=CARTESIAN_POINT ( 'NONE',  ( -3.152548672688508926E-16, -109.5624999986344079, -5.148502694627439702 ) ) ;
#37966=ORIENTED_EDGE ( 'NONE', *, *, #20699, .T. ) ;
#37971=CARTESIAN_POINT ( 'NONE',  ( 4.458734124999999437, -36.06249999863440792, -5.460374474430324690E-16 ) ) ;
#37972=CARTESIAN_POINT ( 'NONE',  ( 1.339745962155612702, -45.16965819600733312, -5.000000000000000000 ) ) ;
#37982=CARTESIAN_POINT ( 'NONE',  ( 4.458734125000001214, -83.14583333196773651, 2.574251347313718519 ) ) ;
#37989=CARTESIAN_POINT ( 'NONE',  ( -1.339745962155613812, -71.08034179853027013, -5.000000000000000000 ) ) ;
#37990=CARTESIAN_POINT ( 'NONE',  ( 4.458734125000001214, -10.14583333196773829, 2.574251347313718519 ) ) ;
#37993=CARTESIAN_POINT ( 'NONE',  ( 5.000000000000000000, -77.29166666393547303, -2.886751345948130876 ) ) ;
#37995=CARTESIAN_POINT ( 'NONE',  ( 4.458734124999999437, 28.93750000136559208, -5.460374474430324690E-16 ) ) ;
#37996=ORIENTED_EDGE ( 'NONE', *, *, #50866, .T. ) ;
#37997=CARTESIAN_POINT ( 'NONE',  ( -2.229367062500000163, -90.47916666530106511, -3.861377020970580443 ) ) ;
#37999=CARTESIAN_POINT ( 'NONE',  ( -2.916731409357579869E-14, 17.37500000273118417, 5.000000000000000888 ) ) ;
#38000=CARTESIAN_POINT ( 'NONE',  ( -2.229367062499996610, -9.145833331967736513, 3.861377020970582219 ) ) ;
#38001=CARTESIAN_POINT ( 'NONE',  ( -5.000000000000000000, 19.91666666666666430, -2.886751345948128211 ) ) ;
#38004=CARTESIAN_POINT ( 'NONE',  ( -5.000000000000000000, -37.87499999726881583, 0.000000000000000000 ) ) ;
#38006=CARTESIAN_POINT ( 'NONE',  ( 9.457646018065525792E-16, 20.93750000136558853, 5.148502694627439702 ) ) ;
#38009=CARTESIAN_POINT ( 'NONE',  ( 2.229367062500001939, -55.97916666530107221, 3.861377020970579999 ) ) ;
#38011=( BOUNDED_CURVE ( )  B_SPLINE_CURVE ( 2, ( #3901, #13230, #23197, #37993, #23520, #43121, #62761, #25410, #30545 ),
 .UNSPECIFIED., .F., .F. ) 
 B_SPLINE_CURVE_WITH_KNOTS ( ( 3, 2, 2, 2, 3 ),
 ( 0.7589285714285713969, 0.7595238095238094900, 0.7607142857142856762, 0.7619047619047618625, 0.7624999999999999556 ),
 .UNSPECIFIED. ) 
 CURVE ( )  GEOMETRIC_REPRESENTATION_ITEM ( )  RATIONAL_B_SPLINE_CURVE ( ( 0.9330127018922194093, 0.9330127018922194093, 1.000000000000000000, 0.8660254037844387076, 1.000000000000000000, 0.8660254037844387076, 1.000000000000000000, 0.9330127018922194093, 0.9330127018922194093 ) ) 
 REPRESENTATION_ITEM ( '' )  );
#38012=DIRECTION ( 'NONE',  ( -0.000000000000000000, 1.000000000000000000, -0.000000000000000000 ) ) ;
#38013=CARTESIAN_POINT ( 'NONE',  ( 1.060575238724906964E-15, 12.25000000000000000, 5.773502691896257311 ) ) ;
#38017=CARTESIAN_POINT ( 'NONE',  ( 2.229367062499998831, -49.64583333196772941, -3.861377020970580887 ) ) ;
#38018=CARTESIAN_POINT ( 'NONE',  ( 5.000000000000000888, -86.45833333060213022, 2.886751345948126879 ) ) ;
#38021=CARTESIAN_POINT ( 'NONE',  ( 0.000000000000000000, -120.0000000000000000, 0.000000000000000000 ) ) ;
#38022=CARTESIAN_POINT ( 'NONE',  ( -4.458734124999999437, -91.64583333196773651, -2.574251347313719407 ) ) ;
#38024=CARTESIAN_POINT ( 'NONE',  ( -4.999999999999999112, -35.91666666666666430, 2.886751345948131764 ) ) ;
#38025=CARTESIAN_POINT ( 'NONE',  ( 6.158835246850667461E-14, 8.875000002731182391, -4.999999999999999112 ) ) ;
#38029=CARTESIAN_POINT ( 'NONE',  ( -4.458734124999999437, -95.39583333196772230, -2.574251347313719407 ) ) ;
#38030=CARTESIAN_POINT ( 'NONE',  ( 2.229367062500001939, 8.770833334698927786, 3.861377020970579999 ) ) ;
#38031=CARTESIAN_POINT ( 'NONE',  ( -5.000000000000000000, 11.04166666939785202, -2.886751345948128211 ) ) ;
#38038=DIRECTION ( 'NONE',  ( -0.000000000000000000, 1.000000000000000000, -0.000000000000000000 ) ) ;
#38039=LINE ( 'NONE', #57043, #47708 ) ;
#38043=CARTESIAN_POINT ( 'NONE',  ( -4.458734124999999437, -19.56249999863440081, 0.000000000000000000 ) ) ;
#38055=CARTESIAN_POINT ( 'NONE',  ( -4.458734124999999437, -67.64583333196773651, -2.574251347313719407 ) ) ;
#38056=CARTESIAN_POINT ( 'NONE',  ( 1.339745962155615144, -7.580341798530293218, 4.999999999999999112 ) ) ;
#38057=CARTESIAN_POINT ( 'NONE',  ( -4.729367062499999719, 29.28125000204839168, 0.000000000000000000 ) ) ;
#38060=CARTESIAN_POINT ( 'NONE',  ( 6.123233995736766282E-16, -120.0000000000000000, -5.000000000000000000 ) ) ;
#38061=VECTOR ( 'NONE', #59870, 1000.000000000000000 ) ;
#38063=CARTESIAN_POINT ( 'NONE',  ( 2.229367062499998831, 3.104166668032259935, -3.861377020970580887 ) ) ;
#38066=CARTESIAN_POINT ( 'NONE',  ( -5.000000000000000000, -55.08333333333332860, -2.886751345948128211 ) ) ;
#38068=CARTESIAN_POINT ( 'NONE',  ( -4.458734124999999437, 5.687500001365592972, 0.000000000000000000 ) ) ;
#38071=CARTESIAN_POINT ( 'NONE',  ( -6.972266317189433020E-16, -104.1249999972688016, -5.000000000000000000 ) ) ;
#38073=ORIENTED_EDGE ( 'NONE', *, *, #33470, .T. ) ;
#38074=CARTESIAN_POINT ( 'NONE',  ( 2.229367062500001939, -76.97916666530106511, 3.861377020970579999 ) ) ;
#38075=AXIS2_PLACEMENT_3D ( 'NONE', #36802, #6902, #2710 ) ;
#38077=CARTESIAN_POINT ( 'NONE',  ( -4.458734124999999437, 9.604166668032259935, -2.574251347313719407 ) ) ;
#38080=CARTESIAN_POINT ( 'NONE',  ( 4.458734125000001214, -59.14583333196773651, 2.574251347313718519 ) ) ;
#38081=CARTESIAN_POINT ( 'NONE',  ( 2.500000000000002220, -21.54166666393548013, 4.330127018922192761 ) ) ;
#38083=DIRECTION ( 'NONE',  ( -0.000000000000000000, 1.000000000000000000, -0.000000000000000000 ) ) ;
#38084=CARTESIAN_POINT ( 'NONE',  ( 5.000000000000000000, 19.62500000273118772, -6.123233995736766282E-16 ) ) ;
#38085=CARTESIAN_POINT ( 'NONE',  ( -5.000000000000000000, -105.9583333306021586, -2.886751345948128211 ) ) ;
#38087=CARTESIAN_POINT ( 'NONE',  ( 4.458734125000001214, -40.89583333196773651, 2.574251347313718519 ) ) ;
#38088=CARTESIAN_POINT ( 'NONE',  ( 2.229367062499998831, -28.89583333196774007, -3.861377020970580887 ) ) ;
#38090=CARTESIAN_POINT ( 'NONE',  ( 2.499999999999998668, 24.66666666666666785, -4.330127018922193649 ) ) ;
#38092=ORIENTED_EDGE ( 'NONE', *, *, #46814, .F. ) ;
#38093=CARTESIAN_POINT ( 'NONE',  ( 1.975475456537005874E-15, -49.74999999999999289, 5.000000000000000000 ) ) ;
#38094=CARTESIAN_POINT ( 'NONE',  ( -4.458734124999999437, -31.31249999863440436, 0.000000000000000000 ) ) ;
#38095=CARTESIAN_POINT ( 'NONE',  ( -4.999999999999999112, -67.79166666393547303, 2.886751345948131764 ) ) ;
#38100=CARTESIAN_POINT ( 'NONE',  ( 2.229367062500001939, -26.97916666530106866, 3.861377020970579999 ) ) ;
#38101=CARTESIAN_POINT ( 'NONE',  ( -2.229367062499996610, -74.39583333196773651, 3.861377020970582219 ) ) ;
#38106=CARTESIAN_POINT ( 'NONE',  ( -5.000000000000000000, -24.08333333333333215, -2.886751345948128211 ) ) ;
#38112=CARTESIAN_POINT ( 'NONE',  ( -2.500000000000000444, 24.95833333606451987, -4.330127018922193649 ) ) ;
#38113=CARTESIAN_POINT ( 'NONE',  ( 5.000000000000000000, -81.29166666393547303, -2.886751345948130876 ) ) ;
#38117=( BOUNDED_CURVE ( )  B_SPLINE_CURVE ( 2, ( #20919, #45674, #35074, #6759, #54693, #25416, #60166, #26372, #45034 ),
 .UNSPECIFIED., .F., .F. ) 
 B_SPLINE_CURVE_WITH_KNOTS ( ( 3, 2, 2, 2, 3 ),
 ( 0.7160714285714285809, 0.7166666666666666741, 0.7178571428571428603, 0.7190476190476190466, 0.7196428571428571397 ),
 .UNSPECIFIED. ) 
 CURVE ( )  GEOMETRIC_REPRESENTATION_ITEM ( )  RATIONAL_B_SPLINE_CURVE ( ( 0.9330127018922194093, 0.9330127018922194093, 1.000000000000000000, 0.8660254037844387076, 1.000000000000000000, 0.8660254037844387076, 1.000000000000000000, 0.9330127018922194093, 0.9330127018922194093 ) ) 
 REPRESENTATION_ITEM ( '' )  );
#38119=CARTESIAN_POINT ( 'NONE',  ( -1.339745962155613812, -81.08034179853028434, -5.000000000000000000 ) ) ;
#38121=LINE ( 'NONE', #24582, #58216 ) ;
#38122=VERTEX_POINT ( 'NONE', #43668 ) ;
#38126=EDGE_CURVE ( 'NONE', #4186, #800, #37920, .T. ) ;
#38130=ORIENTED_EDGE ( 'NONE', *, *, #22818, .F. ) ;
#38131=CARTESIAN_POINT ( 'NONE',  ( -1.339745962155610925, -95.79465819873851729, 5.000000000000000000 ) ) ;
#38139=CARTESIAN_POINT ( 'NONE',  ( -4.458734124999998549, -82.22916666530107932, 2.574251347313722516 ) ) ;
#38140=ADVANCED_FACE ( 'NONE', ( #27940 ), #13478, .T. ) ;
#38141=CARTESIAN_POINT ( 'NONE',  ( 4.458734125000001214, 19.10416666803225638, 2.574251347313718519 ) ) ;
#38143=ORIENTED_EDGE ( 'NONE', *, *, #39695, .F. ) ;
#38147=CARTESIAN_POINT ( 'NONE',  ( 2.500000000000002220, -4.541666663935479242, 4.330127018922192761 ) ) ;
#38150=CARTESIAN_POINT ( 'NONE',  ( 2.229367062500001939, -60.97916666530106511, 3.861377020970579999 ) ) ;
#38151=CARTESIAN_POINT ( 'NONE',  ( 2.499999999999998668, 10.66666666666666430, -4.330127018922193649 ) ) ;
#38153=CARTESIAN_POINT ( 'NONE',  ( 4.458734124999999437, 24.18750000136559564, -5.460374474430324690E-16 ) ) ;
#38154=CARTESIAN_POINT ( 'NONE',  ( 1.975475456537005874E-15, -102.6249999972688158, 5.000000000000000000 ) ) ;
#38156=CARTESIAN_POINT ( 'NONE',  ( -3.152548672688508926E-16, -44.81249999863440792, -5.148502694627439702 ) ) ;
#38157=CARTESIAN_POINT ( 'NONE',  ( 5.000000000000000888, -4.458333330602148870, 2.886751345948126879 ) ) ;
#38158=CARTESIAN_POINT ( 'NONE',  ( -6.972266317189433020E-16, 2.750000000000000000, -5.000000000000000000 ) ) ;
#38161=CARTESIAN_POINT ( 'NONE',  ( -2.229367062500000163, -106.4791666653010651, -3.861377020970580443 ) ) ;
#38163=CARTESIAN_POINT ( 'NONE',  ( -4.458734124999997661, -8.479166665301073991, 2.574251347313722516 ) ) ;
#38164=( BOUNDED_CURVE ( )  B_SPLINE_CURVE ( 2, ( #14099, #52096, #22834, #48514, #4453, #24082, #43677, #63319, #8035 ),
 .UNSPECIFIED., .F., .F. ) 
 B_SPLINE_CURVE_WITH_KNOTS ( ( 3, 2, 2, 2, 3 ),
 ( 0.7375000000000000444, 0.7380952380952381375, 0.7392857142857143238, 0.7404761904761905100, 0.7410714285714286031 ),
 .UNSPECIFIED. ) 
 CURVE ( )  GEOMETRIC_REPRESENTATION_ITEM ( )  RATIONAL_B_SPLINE_CURVE ( ( 0.9330127018922194093, 0.9330127018922194093, 1.000000000000000000, 0.8660254037844387076, 1.000000000000000000, 0.8660254037844387076, 1.000000000000000000, 0.9330127018922194093, 0.9330127018922194093 ) ) 
 REPRESENTATION_ITEM ( '' )  );
#38167=CARTESIAN_POINT ( 'NONE',  ( -2.229367062499996610, -99.14583333196773651, 3.861377020970582219 ) ) ;
#38169=CARTESIAN_POINT ( 'NONE',  ( -2.229367062499996610, -94.39583333196773651, 3.861377020970582219 ) ) ;
#38170=EDGE_CURVE ( 'NONE', #52469, #16995, #52709, .T. ) ;
#38171=CARTESIAN_POINT ( 'NONE',  ( -2.499999999999996447, -53.70833333060213732, 4.330127018922195425 ) ) ;
#38172=CARTESIAN_POINT ( 'NONE',  ( -6.972266317189433020E-16, -37.12499999726881583, -5.000000000000000000 ) ) ;
#38174=CARTESIAN_POINT ( 'NONE',  ( -4.458734124999997661, -15.22916666530107754, 2.574251347313722516 ) ) ;
#38175=CARTESIAN_POINT ( 'NONE',  ( 2.229367062499998831, 12.10416666803226171, -3.861377020970580887 ) ) ;
#38176=CARTESIAN_POINT ( 'NONE',  ( 4.458734125000000326, -61.14583333196773651, 2.574251347313718519 ) ) ;
#38177=FACE_OUTER_BOUND ( 'NONE', #9247, .T. ) ;
#38180=CARTESIAN_POINT ( 'NONE',  ( 1.975475456537005874E-15, -21.75000000000000000, 5.000000000000000000 ) ) ;
#38187=CARTESIAN_POINT ( 'NONE',  ( -2.229367062499996610, -87.14583333196773651, 3.861377020970582219 ) ) ;
#38188=CARTESIAN_POINT ( 'NONE',  ( -3.152548672688508926E-16, 26.18750000136559564, -5.148502694627439702 ) ) ;
#38192=CARTESIAN_POINT ( 'NONE',  ( -5.000000000000000000, -69.99999999999998579, 0.000000000000000000 ) ) ;
#38196=CARTESIAN_POINT ( 'NONE',  ( -4.999999999999998224, -89.91666666666667140, 2.886751345948131764 ) ) ;
#38197=CARTESIAN_POINT ( 'NONE',  ( -2.500000000000000444, -109.0416666639354730, -4.330127018922193649 ) ) ;
#38200=EDGE_CURVE ( 'NONE', #53062, #63665, #48971, .T. ) ;
#38202=EDGE_CURVE ( 'NONE', #15910, #60851, #53125, .T. ) ;
#38208=EDGE_CURVE ( 'NONE', #62028, #14857, #61783, .T. ) ;
#38211=CARTESIAN_POINT ( 'NONE',  ( -4.458734124999999437, -58.56249999863440081, 0.000000000000000000 ) ) ;
#38212=EDGE_CURVE ( 'NONE', #54588, #56025, #55589, .T. ) ;
#38213=( BOUNDED_CURVE ( )  B_SPLINE_CURVE ( 2, ( #25098, #28962, #59526, #43443, #63087, #28653, #34107, #18997, #24151 ),
 .UNSPECIFIED., .F., .F. ) 
 B_SPLINE_CURVE_WITH_KNOTS ( ( 3, 2, 2, 2, 3 ),
 ( 0.7339285714285714857, 0.7345238095238095788, 0.7357142857142857650, 0.7369047619047619513, 0.7375000000000000444 ),
 .UNSPECIFIED. ) 
 CURVE ( )  GEOMETRIC_REPRESENTATION_ITEM ( )  RATIONAL_B_SPLINE_CURVE ( ( 0.9330127018922194093, 0.9330127018922256266, 1.000000000000000000, 0.8660254037844387076, 1.000000000000000000, 0.8660254037844387076, 1.000000000000000000, 0.9330127018922194093, 0.9330127018922194093 ) ) 
 REPRESENTATION_ITEM ( '' )  );
#38216=ORIENTED_EDGE ( 'NONE', *, *, #54428, .T. ) ;
#38218=ADVANCED_FACE ( 'NONE', ( #59763 ), #39165, .T. ) ;
#38222=ORIENTED_EDGE ( 'NONE', *, *, #49885, .T. ) ;
#38225=CARTESIAN_POINT ( 'NONE',  ( -2.229367062499996610, -103.3958333319677365, 3.861377020970582219 ) ) ;
#38226=ORIENTED_EDGE ( 'NONE', *, *, #46381, .T. ) ;
#38232=DIRECTION ( 'NONE',  ( 0.000000000000000000, 0.000000000000000000, 1.000000000000000000 ) ) ;
#38233=CARTESIAN_POINT ( 'NONE',  ( -3.152548672688508926E-16, -7.562499998634404363, -5.148502694627439702 ) ) ;
#38234=CARTESIAN_POINT ( 'NONE',  ( -2.229367062499996610, -102.3958333319677365, 3.861377020970582219 ) ) ;
#38236=CARTESIAN_POINT ( 'NONE',  ( 2.229367062500001939, -28.22916666530107221, 3.861377020970579999 ) ) ;
#38241=CARTESIAN_POINT ( 'NONE',  ( -5.000000000000000000, -34.08333333333332860, -2.886751345948128211 ) ) ;
#38243=CARTESIAN_POINT ( 'NONE',  ( 4.458734125000000326, 6.854166668032259935, 2.574251347313718519 ) ) ;
#38245=CARTESIAN_POINT ( 'NONE',  ( -2.499999999999996447, -92.83333333333334281, 4.330127018922195425 ) ) ;
#38246=CARTESIAN_POINT ( 'NONE',  ( -2.229367062499996610, -28.14583333196774007, 3.861377020970582219 ) ) ;
#38247=CARTESIAN_POINT ( 'NONE',  ( -6.972266317189433020E-16, -77.12499999726881583, -5.000000000000000000 ) ) ;
#38248=CARTESIAN_POINT ( 'NONE',  ( 9.457646018065525792E-16, -75.31249999863440792, 5.148502694627439702 ) ) ;
#38250=CARTESIAN_POINT ( 'NONE',  ( -5.000000000000000000, -101.9583333306021444, -2.886751345948128211 ) ) ;
#38252=CARTESIAN_POINT ( 'NONE',  ( -2.229367062500000163, 0.5208333346989266754, -3.861377020970580443 ) ) ;
#38253=CARTESIAN_POINT ( 'NONE',  ( -4.458734124999999437, 26.43750000136559564, 0.000000000000000000 ) ) ;
#38254=CARTESIAN_POINT ( 'NONE',  ( -3.152548672688508926E-16, -36.81249999863440792, -5.148502694627439702 ) ) ;
#38259=CARTESIAN_POINT ( 'NONE',  ( 2.229367062499998831, -69.64583333196773651, -3.861377020970580887 ) ) ;
#38260=CARTESIAN_POINT ( 'NONE',  ( 5.000000000000000000, -99.37499999726881583, -6.123233995736766282E-16 ) ) ;
#38262=LINE ( 'NONE', #13809, #26682 ) ;
#38263=CARTESIAN_POINT ( 'NONE',  ( -3.152548672688508926E-16, -106.8124999986343937, -5.148502694627439702 ) ) ;
#38265=CARTESIAN_POINT ( 'NONE',  ( -2.499999999999996447, -52.83333333333332860, 4.330127018922195425 ) ) ;
#38266=CARTESIAN_POINT ( 'NONE',  ( -2.499999999999996447, -21.83333333333332860, 4.330127018922195425 ) ) ;
#38267=CYLINDRICAL_SURFACE ( 'NONE', #18130, 5.000000000000000000 ) ;
#38278=DIRECTION ( 'NONE',  ( -0.000000000000000000, 1.000000000000000000, -0.000000000000000000 ) ) ;
#38284=CARTESIAN_POINT ( 'NONE',  ( 4.458734125000001214, -39.14583333196773651, 2.574251347313718519 ) ) ;
#38292=CARTESIAN_POINT ( 'NONE',  ( 6.123233995736766282E-16, -120.0000000000000000, -5.000000000000000000 ) ) ;
#38294=CARTESIAN_POINT ( 'NONE',  ( 9.457646018065525792E-16, -82.31249999863440792, 5.148502694627439702 ) ) ;
#38295=CARTESIAN_POINT ( 'NONE',  ( 2.499999999999998668, -34.20833333060213732, -4.330127018922193649 ) ) ;
#38296=ORIENTED_EDGE ( 'NONE', *, *, #56183, .T. ) ;
#38299=CARTESIAN_POINT ( 'NONE',  ( -6.972266317189433020E-16, -96.25000000000000000, -5.000000000000000000 ) ) ;
#38302=ADVANCED_FACE ( 'NONE', ( #34666 ), #40441, .T. ) ;
#38304=CARTESIAN_POINT ( 'NONE',  ( -2.229367062499996610, -12.39583333196774007, 3.861377020970582219 ) ) ;
#38307=CARTESIAN_POINT ( 'NONE',  ( -5.000000000000000000, -95.87499999726881583, 0.000000000000000000 ) ) ;
#38309=CARTESIAN_POINT ( 'NONE',  ( -2.229367062500000163, 27.27083333469892779, -3.861377020970580443 ) ) ;
#38310=ORIENTED_EDGE ( 'NONE', *, *, #55804, .T. ) ;
#38311=CARTESIAN_POINT ( 'NONE',  ( -2.229367062499996610, -92.14583333196773651, 3.861377020970582219 ) ) ;
#38314=CARTESIAN_POINT ( 'NONE',  ( -4.458734124999999437, -9.312499998634406140, 0.000000000000000000 ) ) ;
#38318=CARTESIAN_POINT ( 'NONE',  ( 5.000000000000000000, -35.37499999726881583, -6.123233995736766282E-16 ) ) ;
#38320=CARTESIAN_POINT ( 'NONE',  ( -2.229367062500000163, 18.52083333469892779, -3.861377020970580443 ) ) ;
#38322=CARTESIAN_POINT ( 'NONE',  ( 9.457646018065525792E-16, -56.06249999863440792, 5.148502694627439702 ) ) ;
#38325=CARTESIAN_POINT ( 'NONE',  ( -2.500000000000000444, 11.83333333333333037, -4.330127018922193649 ) ) ;
#38328=CARTESIAN_POINT ( 'NONE',  ( -2.229367062500000163, -47.47916666530106511, -3.861377020970580443 ) ) ;
#38329=CARTESIAN_POINT ( 'NONE',  ( 2.499999999999998668, -83.20833333060214443, -4.330127018922193649 ) ) ;
#38332=CARTESIAN_POINT ( 'NONE',  ( -4.999999999999998224, -91.91666666666667140, 2.886751345948131764 ) ) ;
#38333=CARTESIAN_POINT ( 'NONE',  ( -4.458734124999999437, -91.56249999863440792, 0.000000000000000000 ) ) ;
#38336=CARTESIAN_POINT ( 'NONE',  ( -4.999999999999999112, -37.91666666666666430, 2.886751345948131764 ) ) ;
#38337=CARTESIAN_POINT ( 'NONE',  ( 5.000000000000000000, 8.708333336064518093, -2.886751345948130876 ) ) ;
#38339=ORIENTED_EDGE ( 'NONE', *, *, #36542, .F. ) ;
#38340=CARTESIAN_POINT ( 'NONE',  ( 9.457646018065525792E-16, -95.06249999863440792, 5.148502694627439702 ) ) ;
#38341=CARTESIAN_POINT ( 'NONE',  ( -4.458734124999999437, 8.354166668032261711, -2.574251347313719407 ) ) ;
#38342=CARTESIAN_POINT ( 'NONE',  ( 1.060575238724906964E-15, 9.375000002731184168, 5.773502691896257311 ) ) ;
#38343=CARTESIAN_POINT ( 'NONE',  ( 5.000000000000000000, -80.50000000000000000, -6.123233995736766282E-16 ) ) ;
#38346=CARTESIAN_POINT ( 'NONE',  ( -2.499999999999996447, -39.83333333333332860, 4.330127018922195425 ) ) ;
#38350=CARTESIAN_POINT ( 'NONE',  ( -6.972266317189433020E-16, 19.75000000000000000, -5.000000000000000000 ) ) ;
#38354=CARTESIAN_POINT ( 'NONE',  ( -3.152548672688508926E-16, -21.81249999863440436, -5.148502694627439702 ) ) ;
#38363=CARTESIAN_POINT ( 'NONE',  ( 2.499999999999998668, -93.20833333060214443, -4.330127018922193649 ) ) ;
#38365=CARTESIAN_POINT ( 'NONE',  ( 4.458734124999999437, -67.06249999863440792, -5.460374474430324690E-16 ) ) ;
#38367=DIRECTION ( 'NONE',  ( 0.000000000000000000, 0.000000000000000000, 1.000000000000000000 ) ) ;
#38368=ORIENTED_EDGE ( 'NONE', *, *, #35533, .F. ) ;
#38371=CARTESIAN_POINT ( 'NONE',  ( -4.458734124999999437, 0.3541666680322609340, -2.574251347313719407 ) ) ;
#38372=ORIENTED_EDGE ( 'NONE', *, *, #47180, .T. ) ;
#38373=CARTESIAN_POINT ( 'NONE',  ( 5.000000000000000000, -45.50000000000000000, -6.123233995736766282E-16 ) ) ;
#38380=CARTESIAN_POINT ( 'NONE',  ( -4.458734124999999437, -75.39583333196773651, -2.574251347313719407 ) ) ;
#38381=CARTESIAN_POINT ( 'NONE',  ( 5.000000000000000000, 14.62500000273118594, -6.123233995736766282E-16 ) ) ;
#38382=CARTESIAN_POINT ( 'NONE',  ( -4.458734124999998549, 7.770833334698925121, 2.574251347313722516 ) ) ;
#38384=CARTESIAN_POINT ( 'NONE',  ( -3.152548672688508926E-16, -59.81249999863440792, -5.148502694627439702 ) ) ;
#38385=CARTESIAN_POINT ( 'NONE',  ( 1.060575238724906964E-15, -21.62499999726881228, 5.773502691896257311 ) ) ;
#38389=CARTESIAN_POINT ( 'NONE',  ( 6.123233995736766282E-16, -120.0000000000000000, -5.000000000000000000 ) ) ;
#38390=FACE_OUTER_BOUND ( 'NONE', #20635, .T. ) ;
#38391=CARTESIAN_POINT ( 'NONE',  ( -4.458734124999999437, -41.31249999863440081, 0.000000000000000000 ) ) ;
#38393=CARTESIAN_POINT ( 'NONE',  ( 4.458734124999998549, -27.97916666530107221, -2.574251347313721627 ) ) ;
#38395=CARTESIAN_POINT ( 'NONE',  ( -3.535250795749689387E-16, 23.75000000000000000, -5.773502691896257311 ) ) ;
#38397=CARTESIAN_POINT ( 'NONE',  ( 4.458734124999998549, -105.9791666653010651, -2.574251347313721627 ) ) ;
#38398=EDGE_CURVE ( 'NONE', #19213, #53853, #59443, .T. ) ;
#38399=CARTESIAN_POINT ( 'NONE',  ( 4.458734125000001214, -32.89583333196774362, 2.574251347313718519 ) ) ;
#38400=CARTESIAN_POINT ( 'NONE',  ( 5.000000000000000000, -68.29166666393547303, -2.886751345948129988 ) ) ;
#38403=CARTESIAN_POINT ( 'NONE',  ( -3.152548672688508926E-16, -75.81249999863440792, -5.148502694627439702 ) ) ;
#38408=CARTESIAN_POINT ( 'NONE',  ( 5.000000000000000888, -24.58333333333333215, 2.886751345948126879 ) ) ;
#38410=ORIENTED_EDGE ( 'NONE', *, *, #11047, .F. ) ;
#38412=CARTESIAN_POINT ( 'NONE',  ( 1.060575238724906964E-15, 28.37500000273118417, 5.773502691896257311 ) ) ;
#38421=CARTESIAN_POINT ( 'NONE',  ( -6.972266317189433020E-16, -97.12499999726880162, -5.000000000000000000 ) ) ;
#38432=CARTESIAN_POINT ( 'NONE',  ( 1.975475456537005874E-15, -50.62499999726881583, 5.000000000000000000 ) ) ;
#38436=VERTEX_POINT ( 'NONE', #10223 ) ;
#38437=CARTESIAN_POINT ( 'NONE',  ( -3.152548672688508926E-16, -84.56249999863439371, -5.148502694627439702 ) ) ;
#38438=CARTESIAN_POINT ( 'NONE',  ( -3.152548672688508926E-16, 20.43750000136559208, -5.148502694627439702 ) ) ;
#38446=CARTESIAN_POINT ( 'NONE',  ( -2.229367062500000163, -62.47916666530106511, -3.861377020970580443 ) ) ;
#38448=CARTESIAN_POINT ( 'NONE',  ( 2.229367062500001939, 24.02083333469892779, 3.861377020970579999 ) ) ;
#38449=( BOUNDED_CURVE ( )  B_SPLINE_CURVE ( 2, ( #22063, #17560, #61625, #41655, #37178, #57121, #61943, #37483, #61306 ),
 .UNSPECIFIED., .F., .F. ) 
 B_SPLINE_CURVE_WITH_KNOTS ( ( 3, 2, 2, 2, 3 ),
 ( 0.8303571428571429047, 0.8309523809523809978, 0.8321428571428571841, 0.8333333333333333703, 0.8339285714285714635 ),
 .UNSPECIFIED. ) 
 CURVE ( )  GEOMETRIC_REPRESENTATION_ITEM ( )  RATIONAL_B_SPLINE_CURVE ( ( 0.9330127018922194093, 0.9330127018922194093, 1.000000000000000000, 0.8660254037844387076, 1.000000000000000000, 0.8660254037844387076, 1.000000000000000000, 0.9330127018922194093, 0.9330127018922194093 ) ) 
 REPRESENTATION_ITEM ( '' )  );
#38451=CARTESIAN_POINT ( 'NONE',  ( -4.458734124999999437, -45.64583333196774362, -2.574251347313719407 ) ) ;
#38452=CARTESIAN_POINT ( 'NONE',  ( 5.000000000000000000, -2.374999997268815388, -6.123233995736766282E-16 ) ) ;
#38454=DIRECTION ( 'NONE',  ( -0.000000000000000000, 1.000000000000000000, -0.000000000000000000 ) ) ;
#38456=CARTESIAN_POINT ( 'NONE',  ( -3.152548672688508926E-16, -109.5624999986344079, -5.148502694627439702 ) ) ;
#38457=CARTESIAN_POINT ( 'NONE',  ( -4.458734124999999437, -9.645833331967738289, -2.574251347313719407 ) ) ;
#38460=CARTESIAN_POINT ( 'NONE',  ( -4.458734124999999437, -97.39583333196773651, -2.574251347313719407 ) ) ;
#38462=CARTESIAN_POINT ( 'NONE',  ( -4.458734124999999437, -92.64583333196773651, -2.574251347313719407 ) ) ;
#38464=CARTESIAN_POINT ( 'NONE',  ( 2.500000000000002220, -54.54166666393548013, 4.330127018922192761 ) ) ;
#38465=CARTESIAN_POINT ( 'NONE',  ( 5.000000000000000000, -5.416666666666666963, -2.886751345948130876 ) ) ;
#38470=CARTESIAN_POINT ( 'NONE',  ( -4.458734124999999437, -14.31249999863440436, 0.000000000000000000 ) ) ;
#38471=CARTESIAN_POINT ( 'NONE',  ( 2.229367062500001939, 11.77083333469892601, 3.861377020970579999 ) ) ;
#38472=CARTESIAN_POINT ( 'NONE',  ( -2.229367062499996610, -60.39583333196774362, 3.861377020970582219 ) ) ;
#38476=ORIENTED_EDGE ( 'NONE', *, *, #7236, .F. ) ;
#38481=CARTESIAN_POINT ( 'NONE',  ( 2.229367062500001939, -87.97916666530107932, 3.861377020970579999 ) ) ;
#38482=CARTESIAN_POINT ( 'NONE',  ( -4.458734124999999437, 17.35416666803225993, -2.574251347313719407 ) ) ;
#38484=CARTESIAN_POINT ( 'NONE',  ( -2.500000000000000444, -48.16666666666666430, -4.330127018922193649 ) ) ;
#38485=EDGE_CURVE ( 'NONE', #2538, #58058, #2607, .T. ) ;
#38488=CARTESIAN_POINT ( 'NONE',  ( -3.535250795749689387E-16, -70.25000000000000000, -5.773502691896257311 ) ) ;
#38490=ORIENTED_EDGE ( 'NONE', *, *, #12576, .T. ) ;
#38491=CARTESIAN_POINT ( 'NONE',  ( 6.123233995736766282E-16, -120.0000000000000000, -5.000000000000000000 ) ) ;
#38492=ORIENTED_EDGE ( 'NONE', *, *, #6766, .T. ) ;
#38493=CARTESIAN_POINT ( 'NONE',  ( 1.975475456537005874E-15, -79.62499999726881583, 5.000000000000000000 ) ) ;
#38499=ORIENTED_EDGE ( 'NONE', *, *, #26451, .T. ) ;
#38505=CARTESIAN_POINT ( 'NONE',  ( 4.458734125000001214, -57.14583333196773651, 2.574251347313718519 ) ) ;
#38508=ORIENTED_EDGE ( 'NONE', *, *, #44508, .T. ) ;
#38512=ORIENTED_EDGE ( 'NONE', *, *, #56329, .F. ) ;
#38515=EDGE_CURVE ( 'NONE', #27636, #29896, #9159, .T. ) ;
#38516=CARTESIAN_POINT ( 'NONE',  ( -4.458734124999998549, -103.4791666653010509, 2.574251347313722516 ) ) ;
#38517=VERTEX_POINT ( 'NONE', #26612 ) ;
#38520=CARTESIAN_POINT ( 'NONE',  ( 2.229367062500001939, -39.97916666530107221, 3.861377020970579999 ) ) ;
#38521=( BOUNDED_CURVE ( )  B_SPLINE_CURVE ( 2, ( #50773, #6715, #60439, #1274, #30178, #25371, #30507, #16364, #26324 ),
 .UNSPECIFIED., .F., .F. ) 
 B_SPLINE_CURVE_WITH_KNOTS ( ( 3, 2, 2, 2, 3 ),
 ( 0.7267857142857142572, 0.7273809523809523503, 0.7285714285714285365, 0.7297619047619047228, 0.7303571428571428159 ),
 .UNSPECIFIED. ) 
 CURVE ( )  GEOMETRIC_REPRESENTATION_ITEM ( )  RATIONAL_B_SPLINE_CURVE ( ( 0.9330127018922194093, 0.9330127018922194093, 1.000000000000000000, 0.8660254037844387076, 1.000000000000000000, 0.8660254037844387076, 1.000000000000000000, 0.9330127018922194093, 0.9330127018922194093 ) ) 
 REPRESENTATION_ITEM ( '' )  );
#38522=CARTESIAN_POINT ( 'NONE',  ( 0.000000000000000000, -120.0000000000000000, 5.000000000000000000 ) ) ;
#38523=CARTESIAN_POINT ( 'NONE',  ( 2.229367062499998831, -10.64583333196773829, -3.861377020970580887 ) ) ;
#38524=CARTESIAN_POINT ( 'NONE',  ( 4.458734125000000326, -100.1458333319677365, 2.574251347313718519 ) ) ;
#38526=CARTESIAN_POINT ( 'NONE',  ( 4.458734124999998549, -26.97916666530107221, -2.574251347313721627 ) ) ;
#38530=DIRECTION ( 'NONE',  ( -0.000000000000000000, 1.000000000000000000, -0.000000000000000000 ) ) ;
#38531=CARTESIAN_POINT ( 'NONE',  ( -6.972266317189433020E-16, -88.12499999726880162, -5.000000000000000000 ) ) ;
#38533=CARTESIAN_POINT ( 'NONE',  ( -4.458734124999999437, 3.437500001365594748, 0.000000000000000000 ) ) ;
#38535=CARTESIAN_POINT ( 'NONE',  ( 1.975475456537005874E-15, 2.249999999999999556, 5.000000000000000000 ) ) ;
#38536=CARTESIAN_POINT ( 'NONE',  ( 0.000000000000000000, -120.0000000000000000, 5.000000000000000000 ) ) ;
#38537=CARTESIAN_POINT ( 'NONE',  ( 2.499999999999998668, -97.33333333333332860, -4.330127018922193649 ) ) ;
#38538=CARTESIAN_POINT ( 'NONE',  ( 4.458734124999998549, -27.72916666530107221, -2.574251347313721627 ) ) ;
#38539=CARTESIAN_POINT ( 'NONE',  ( 4.458734124999998549, -76.97916666530106511, -2.574251347313721627 ) ) ;
#38541=FACE_OUTER_BOUND ( 'NONE', #39434, .T. ) ;
#38543=EDGE_CURVE ( 'NONE', #7250, #17309, #48602, .T. ) ;
#38545=CARTESIAN_POINT ( 'NONE',  ( -4.458734124999999437, 2.604166668032263043, -2.574251347313719407 ) ) ;
#38546=CARTESIAN_POINT ( 'NONE',  ( 9.457646018065525792E-16, 25.68750000136559208, 5.148502694627439702 ) ) ;
#38547=CARTESIAN_POINT ( 'NONE',  ( -4.458734124999999437, -44.64583333196773651, -2.574251347313719407 ) ) ;
#38548=CARTESIAN_POINT ( 'NONE',  ( 1.975475456537005874E-15, -3.624999997268814056, 5.000000000000000000 ) ) ;
#38552=CARTESIAN_POINT ( 'NONE',  ( 2.229367062500001939, -69.97916666530107932, 3.861377020970579999 ) ) ;
#38553=CARTESIAN_POINT ( 'NONE',  ( -5.000000000000000000, -104.8749999972688158, 0.000000000000000000 ) ) ;
#38555=VECTOR ( 'NONE', #46392, 1000.000000000000000 ) ;
#38558=ADVANCED_FACE ( 'NONE', ( #7638 ), #6370, .T. ) ;
#38559=CARTESIAN_POINT ( 'NONE',  ( 2.229367062499998831, -106.8958333319677365, -3.861377020970580887 ) ) ;
#38561=CARTESIAN_POINT ( 'NONE',  ( 5.000000000000000000, -56.49999999999999289, -6.123233995736766282E-16 ) ) ;
#38562=CARTESIAN_POINT ( 'NONE',  ( -5.000000000000000000, -22.08333333333333215, -2.886751345948128211 ) ) ;
#38565=CARTESIAN_POINT ( 'NONE',  ( 1.975475456537005874E-15, -7.750000000000000000, 5.000000000000000000 ) ) ;
#38566=CARTESIAN_POINT ( 'NONE',  ( 5.000000000000000000, -27.29166666393548013, -2.886751345948130876 ) ) ;
#38573=ORIENTED_EDGE ( 'NONE', *, *, #46048, .T. ) ;
#38580=CARTESIAN_POINT ( 'NONE',  ( 4.458734124999999437, -39.06249999863440081, -5.460374474430324690E-16 ) ) ;
#38587=CARTESIAN_POINT ( 'NONE',  ( 1.339745962155612702, -26.29465819873852084, -5.000000000000000000 ) ) ;
#38589=CARTESIAN_POINT ( 'NONE',  ( 2.229367062500001939, -87.22916666530107932, 3.861377020970579999 ) ) ;
#38590=CARTESIAN_POINT ( 'NONE',  ( 2.499999999999998668, -108.3333333333333428, -4.330127018922193649 ) ) ;
#38592=CARTESIAN_POINT ( 'NONE',  ( -4.999999999999998224, -46.91666666666666430, 2.886751345948131764 ) ) ;
#38598=CARTESIAN_POINT ( 'NONE',  ( -1.339745962155610925, -13.79465819873852261, 5.000000000000000000 ) ) ;
#38599=CARTESIAN_POINT ( 'NONE',  ( -3.152548672688508926E-16, -13.81249999863440436, -5.148502694627439702 ) ) ;
#38600=PRODUCT_DEFINITION_CONTEXT ( 'detailed design', #51998, 'design' ) ;
#38601=CYLINDRICAL_SURFACE ( 'NONE', #55902, 5.000000000000000000 ) ;
#38605=CARTESIAN_POINT ( 'NONE',  ( 4.458734124999998549, 21.02083333469892779, -2.574251347313721627 ) ) ;
#38606=ORIENTED_EDGE ( 'NONE', *, *, #41769, .F. ) ;
#38607=CARTESIAN_POINT ( 'NONE',  ( -4.458734124999999437, -93.39583333196772230, -2.574251347313719407 ) ) ;
#38609=LINE ( 'NONE', #19947, #16475 ) ;
#38610=CARTESIAN_POINT ( 'NONE',  ( 4.458734124999999437, -12.81249999863440259, -5.460374474430324690E-16 ) ) ;
#38611=CYLINDRICAL_SURFACE ( 'NONE', #24280, 5.000000000000000000 ) ;
#38614=CARTESIAN_POINT ( 'NONE',  ( 5.000000000000000000, -39.29166666393548724, -2.886751345948129988 ) ) ;
#38616=CARTESIAN_POINT ( 'NONE',  ( 4.458734125000000326, 19.10416666803225638, 2.574251347313718519 ) ) ;
#38618=VERTEX_POINT ( 'NONE', #30691 ) ;
#38620=CARTESIAN_POINT ( 'NONE',  ( 2.229367062499998831, -63.64583333196772941, -3.861377020970580887 ) ) ;
#38623=CARTESIAN_POINT ( 'NONE',  ( 1.060575238724906964E-15, 9.250000000000001776, 5.773502691896257311 ) ) ;
#38625=CARTESIAN_POINT ( 'NONE',  ( -5.000000000000000000, -98.87499999726881583, 0.000000000000000000 ) ) ;
#38626=CARTESIAN_POINT ( 'NONE',  ( 2.229367062500001939, -55.97916666530107221, 3.861377020970579999 ) ) ;
#38627=CARTESIAN_POINT ( 'NONE',  ( 5.000000000000000000, -83.29166666393547303, -2.886751345948129988 ) ) ;
#38629=CARTESIAN_POINT ( 'NONE',  ( -5.000000000000000000, -17.00000000000000000, 0.000000000000000000 ) ) ;
#38630=CARTESIAN_POINT ( 'NONE',  ( -5.000000000000000000, -92.00000000000000000, 0.000000000000000000 ) ) ;
#38631=CARTESIAN_POINT ( 'NONE',  ( 4.458734124999998549, -88.97916666530106511, -2.574251347313721627 ) ) ;
#38633=CARTESIAN_POINT ( 'NONE',  ( -2.499999999999996447, -39.83333333333332860, 4.330127018922195425 ) ) ;
#38636=CARTESIAN_POINT ( 'NONE',  ( 5.000000000000000888, -22.58333333333332860, 2.886751345948126879 ) ) ;
#38638=CARTESIAN_POINT ( 'NONE',  ( -2.229367062500000163, -103.4791666653010651, -3.861377020970580443 ) ) ;
#38639=CARTESIAN_POINT ( 'NONE',  ( -2.229367062500000163, 6.270833334698928674, -3.861377020970580443 ) ) ;
#38640=CARTESIAN_POINT ( 'NONE',  ( -4.999999999999999112, 12.20833333606451632, 2.886751345948131764 ) ) ;
#38644=AXIS2_PLACEMENT_3D ( 'NONE', #59532, #16419, #36037 ) ;
#38647=CARTESIAN_POINT ( 'NONE',  ( -2.500000000000000444, 2.833333333333333481, -4.330127018922193649 ) ) ;
#38648=EDGE_CURVE ( 'NONE', #35135, #19195, #49916, .T. ) ;
#38656=CARTESIAN_POINT ( 'NONE',  ( -3.152548672688508926E-16, -27.81249999863440436, -5.148502694627439702 ) ) ;
#38664=ORIENTED_EDGE ( 'NONE', *, *, #7236, .T. ) ;
#38665=CARTESIAN_POINT ( 'NONE',  ( 5.000000000000000000, -93.37499999726881583, -6.123233995736766282E-16 ) ) ;
#38667=CARTESIAN_POINT ( 'NONE',  ( 9.457646018065525792E-16, -71.31249999863439371, 5.148502694627439702 ) ) ;
#38671=CARTESIAN_POINT ( 'NONE',  ( 5.000000000000000000, 12.50000000000000000, -6.123233995736766282E-16 ) ) ;
#38674=CARTESIAN_POINT ( 'NONE',  ( -2.229367062500000163, 2.270833334698928230, -3.861377020970580443 ) ) ;
#38676=CARTESIAN_POINT ( 'NONE',  ( 0.000000000000000000, -120.0000000000000000, 0.000000000000000000 ) ) ;
#38681=ORIENTED_EDGE ( 'NONE', *, *, #10688, .T. ) ;
#38682=CARTESIAN_POINT ( 'NONE',  ( 2.229367062499998831, -78.64583333196773651, -3.861377020970580887 ) ) ;
#38684=CARTESIAN_POINT ( 'NONE',  ( 9.457646018065525792E-16, -0.06249999863440491854, 5.148502694627439702 ) ) ;
#38687=CARTESIAN_POINT ( 'NONE',  ( -2.229367062499996610, -63.39583333196774362, 3.861377020970582219 ) ) ;
#38689=CARTESIAN_POINT ( 'NONE',  ( -3.535250795749689387E-16, -19.12499999726881228, -5.773502691896257311 ) ) ;
#38691=CYLINDRICAL_SURFACE ( 'NONE', #46005, 5.000000000000000000 ) ;
#38692=CARTESIAN_POINT ( 'NONE',  ( -4.999999999999998224, -58.91666666666665009, 2.886751345948131764 ) ) ;
#38694=LINE ( 'NONE', #38389, #16210 ) ;
#38695=CARTESIAN_POINT ( 'NONE',  ( 2.229367062499998831, -41.64583333196773651, -3.861377020970580887 ) ) ;
#38696=CARTESIAN_POINT ( 'NONE',  ( 4.458734124999998549, -25.97916666530107221, -2.574251347313721627 ) ) ;
#38699=CARTESIAN_POINT ( 'NONE',  ( 5.000000000000000888, 23.41666666666666785, 2.886751345948126879 ) ) ;
#38701=CARTESIAN_POINT ( 'NONE',  ( -4.458734124999999437, -107.6458333319677365, -2.574251347313719407 ) ) ;
#38702=CARTESIAN_POINT ( 'NONE',  ( 4.458734125000001214, -36.89583333196773651, 2.574251347313718519 ) ) ;
#38703=CARTESIAN_POINT ( 'NONE',  ( -4.999999999999999112, -65.79166666393547303, 2.886751345948131764 ) ) ;
#38706=CARTESIAN_POINT ( 'NONE',  ( 9.457646018065525792E-16, -75.31249999863440792, 5.148502694627439702 ) ) ;
#38710=CARTESIAN_POINT ( 'NONE',  ( -5.000000000000000000, -22.08333333333333215, -2.886751345948128211 ) ) ;
#38716=CARTESIAN_POINT ( 'NONE',  ( 2.499999999999998668, 26.79166666939785202, -4.330127018922193649 ) ) ;
#38717=CARTESIAN_POINT ( 'NONE',  ( 1.975475456537005874E-15, -48.62499999726880162, 5.000000000000000000 ) ) ;
#38719=CARTESIAN_POINT ( 'NONE',  ( 4.769696007084727185, -120.0000000000000000, 1.500000000000000000 ) ) ;
#38722=CARTESIAN_POINT ( 'NONE',  ( -5.000000000000000000, -77.00000000000000000, 0.000000000000000000 ) ) ;
#38724=( BOUNDED_CURVE ( )  B_SPLINE_CURVE ( 2, ( #23323, #18491, #7272, #46499, #4323 ),
 .UNSPECIFIED., .F., .F. ) 
 B_SPLINE_CURVE_WITH_KNOTS ( ( 3, 2, 3 ),
 ( 0.9982142857142857206, 0.9988095238095238138, 1.000000000000000000 ),
 .UNSPECIFIED. ) 
 CURVE ( )  GEOMETRIC_REPRESENTATION_ITEM ( )  RATIONAL_B_SPLINE_CURVE ( ( 0.9330127018922194093, 0.9330127018922194093, 1.000000000000000000, 0.8660254037844387076, 1.000000000000000000 ) ) 
 REPRESENTATION_ITEM ( '' )  );
#38725=CARTESIAN_POINT ( 'NONE',  ( 1.339745962155612702, -12.29465819873851906, -5.000000000000000000 ) ) ;
#38726=CARTESIAN_POINT ( 'NONE',  ( 2.229367062500001939, -19.97916666530107221, 3.861377020970579999 ) ) ;
#38728=CARTESIAN_POINT ( 'NONE',  ( 2.500000000000002220, -97.54166666393545881, 4.330127018922192761 ) ) ;
#38733=AXIS2_PLACEMENT_3D ( 'NONE', #47095, #22973, #42259 ) ;
#38736=CARTESIAN_POINT ( 'NONE',  ( 5.000000000000000888, -87.58333333333332860, 2.886751345948126879 ) ) ;
#38737=CARTESIAN_POINT ( 'NONE',  ( 1.975475456537005874E-15, -9.624999997268814056, 5.000000000000000000 ) ) ;
#38741=CARTESIAN_POINT ( 'NONE',  ( -6.972266317189433020E-16, -51.12499999726880873, -5.000000000000000000 ) ) ;
#38743=EDGE_CURVE ( 'NONE', #31992, #4978, #54170, .T. ) ;
#38747=DIRECTION ( 'NONE',  ( -0.000000000000000000, 1.000000000000000000, -0.000000000000000000 ) ) ;
#38748=CARTESIAN_POINT ( 'NONE',  ( -4.458734124999998549, 20.77083333469892779, 2.574251347313722516 ) ) ;
#38749=CYLINDRICAL_SURFACE ( 'NONE', #14267, 5.000000000000000000 ) ;
#38750=VERTEX_POINT ( 'NONE', #34881 ) ;
#38754=CARTESIAN_POINT ( 'NONE',  ( 2.500000000000002220, -39.66666666666667140, 4.330127018922192761 ) ) ;
#38756=CARTESIAN_POINT ( 'NONE',  ( -3.152548672688508926E-16, -60.56249999863440792, -5.148502694627439702 ) ) ;
#38758=CARTESIAN_POINT ( 'NONE',  ( -3.152548672688508926E-16, 21.43750000136559564, -5.148502694627439702 ) ) ;
#38759=CARTESIAN_POINT ( 'NONE',  ( 5.000000000000000000, -102.3749999972688158, -6.123233995736766282E-16 ) ) ;
#38760=CARTESIAN_POINT ( 'NONE',  ( -1.339745962155610925, -43.79465819873851729, 5.000000000000000000 ) ) ;
#38761=CARTESIAN_POINT ( 'NONE',  ( 2.229367062500001939, -48.22916666530106511, 3.861377020970579999 ) ) ;
#38762=CARTESIAN_POINT ( 'NONE',  ( 5.000000000000000888, -1.458333330602149092, 2.886751345948126879 ) ) ;
#38764=DIRECTION ( 'NONE',  ( 0.000000000000000000, 0.000000000000000000, 1.000000000000000000 ) ) ;
#38766=CARTESIAN_POINT ( 'NONE',  ( -3.152548672688508926E-16, -105.5624999986344221, -5.148502694627439702 ) ) ;
#38767=CARTESIAN_POINT ( 'NONE',  ( 2.229367062500001939, -13.22916666530107221, 3.861377020970579999 ) ) ;
#38768=VERTEX_POINT ( 'NONE', #45161 ) ;
#38771=CARTESIAN_POINT ( 'NONE',  ( -2.229367062500000163, -98.47916666530105090, -3.861377020970580443 ) ) ;
#38773=CARTESIAN_POINT ( 'NONE',  ( -4.458734124999999437, -92.56249999863440792, 0.000000000000000000 ) ) ;
#38774=VECTOR ( 'NONE', #10003, 1000.000000000000000 ) ;
#38775=CARTESIAN_POINT ( 'NONE',  ( -5.000000000000000000, -49.95833333060213022, -2.886751345948128211 ) ) ;
#38776=CARTESIAN_POINT ( 'NONE',  ( -2.499999999999996447, -36.70833333060213732, 4.330127018922195425 ) ) ;
#38779=CARTESIAN_POINT ( 'NONE',  ( -2.229367062499996610, -17.14583333196773651, 3.861377020970582219 ) ) ;
#38780=CARTESIAN_POINT ( 'NONE',  ( -2.229367062500000163, 12.27083333469892601, -3.861377020970580443 ) ) ;
#38781=CARTESIAN_POINT ( 'NONE',  ( 9.457646018065525792E-16, -57.31249999863440081, 5.148502694627439702 ) ) ;
#38782=CARTESIAN_POINT ( 'NONE',  ( 0.000000000000000000, -120.0000000000000000, 0.000000000000000000 ) ) ;
#38789=CYLINDRICAL_SURFACE ( 'NONE', #5183, 5.000000000000000000 ) ;
#38790=CARTESIAN_POINT ( 'NONE',  ( -1.339745962155610925, -66.66965819600733312, 5.000000000000000000 ) ) ;
#38791=CARTESIAN_POINT ( 'NONE',  ( -4.458734124999999437, -85.31249999863439371, 0.000000000000000000 ) ) ;
#38792=CARTESIAN_POINT ( 'NONE',  ( 4.458734124999999437, 18.93750000136559564, -5.460374474430324690E-16 ) ) ;
#38797=CARTESIAN_POINT ( 'NONE',  ( -3.535250795749689387E-16, -71.25000000000000000, -5.773502691896257311 ) ) ;
#38799=ORIENTED_EDGE ( 'NONE', *, *, #61301, .T. ) ;
#38801=ORIENTED_EDGE ( 'NONE', *, *, #19663, .T. ) ;
#38808=ORIENTED_EDGE ( 'NONE', *, *, #44705, .F. ) ;
#38812=EDGE_LOOP ( 'NONE', ( #34305, #62552, #20199, #56098 ) ) ;
#38814=DIRECTION ( 'NONE',  ( 0.000000000000000000, 0.000000000000000000, 1.000000000000000000 ) ) ;
#38815=CARTESIAN_POINT ( 'NONE',  ( -2.229367062499996610, -57.39583333196773651, 3.861377020970582219 ) ) ;
#38822=AXIS2_PLACEMENT_3D ( 'NONE', #49094, #54571, #34952 ) ;
#38828=CARTESIAN_POINT ( 'NONE',  ( -2.229367062499996610, -104.3958333319677365, 3.861377020970582219 ) ) ;
#38829=CARTESIAN_POINT ( 'NONE',  ( -2.500000000000000444, -69.04166666393547303, -4.330127018922193649 ) ) ;
#38833=CARTESIAN_POINT ( 'NONE',  ( 4.458734124999999437, -36.81249999863440792, -5.460374474430324690E-16 ) ) ;
#38834=CARTESIAN_POINT ( 'NONE',  ( 1.975475456537005874E-15, -56.75000000000000000, 5.000000000000000000 ) ) ;
#38835=DIRECTION ( 'NONE',  ( -0.000000000000000000, 1.000000000000000000, -0.000000000000000000 ) ) ;
#38836=CARTESIAN_POINT ( 'NONE',  ( -4.458734124999999437, -14.31249999863440436, 0.000000000000000000 ) ) ;
#38837=CARTESIAN_POINT ( 'NONE',  ( -2.229367062499996610, -98.39583333196773651, 3.861377020970582219 ) ) ;
#38840=EDGE_CURVE ( 'NONE', #1445, #14167, #50305, .T. ) ;
#38842=CARTESIAN_POINT ( 'NONE',  ( -4.458734124999999437, -28.64583333196774007, -2.574251347313719407 ) ) ;
#38844=CARTESIAN_POINT ( 'NONE',  ( -5.000000000000000000, 12.00000000000000000, 0.000000000000000000 ) ) ;
#38847=CARTESIAN_POINT ( 'NONE',  ( 1.339745962155612702, -17.29465819873852084, -5.000000000000000000 ) ) ;
#38850=CARTESIAN_POINT ( 'NONE',  ( 9.457646018065525792E-16, 2.687500001365593860, 5.148502694627439702 ) ) ;
#38852=CARTESIAN_POINT ( 'NONE',  ( 5.000000000000000888, 9.416666666666666075, 2.886751345948126879 ) ) ;
#38853=CARTESIAN_POINT ( 'NONE',  ( -5.000000000000000000, -94.08333333333332860, -2.886751345948128211 ) ) ;
#38854=CARTESIAN_POINT ( 'NONE',  ( -2.229367062499996610, -31.14583333196773651, 3.861377020970582219 ) ) ;
#38855=CARTESIAN_POINT ( 'NONE',  ( -1.339745962155610925, -22.66965819600732956, 5.000000000000000000 ) ) ;
#38856=CARTESIAN_POINT ( 'NONE',  ( -4.458734124999999437, -75.56249999863440792, 0.000000000000000000 ) ) ;
#38859=EDGE_CURVE ( 'NONE', #37487, #52254, #19482, .T. ) ;
#38861=CARTESIAN_POINT ( 'NONE',  ( -2.229367062500000163, -4.479166665301070438, -3.861377020970580443 ) ) ;
#38862=CARTESIAN_POINT ( 'NONE',  ( 2.229367062500001939, 27.77083333469892779, 3.861377020970579999 ) ) ;
#38863=CARTESIAN_POINT ( 'NONE',  ( -2.229367062500000163, -43.72916666530106511, -3.861377020970580443 ) ) ;
#38865=EDGE_LOOP ( 'NONE', ( #23724, #22967, #61716, #2026 ) ) ;
#38868=CARTESIAN_POINT ( 'NONE',  ( 2.229367062500001939, -71.97916666530107932, 3.861377020970579999 ) ) ;
#38869=CARTESIAN_POINT ( 'NONE',  ( 5.000000000000000000, -103.3749999972688158, -6.123233995736766282E-16 ) ) ;
#38876=CARTESIAN_POINT ( 'NONE',  ( 5.000000000000000000, -54.49999999999999289, -6.123233995736766282E-16 ) ) ;
#38877=LINE ( 'NONE', #4788, #6951 ) ;
#38880=CARTESIAN_POINT ( 'NONE',  ( -6.972266317189433020E-16, -56.25000000000000000, -5.000000000000000000 ) ) ;
#38896=CARTESIAN_POINT ( 'NONE',  ( -4.458734124999999437, -39.56249999863440081, 0.000000000000000000 ) ) ;
#38900=CARTESIAN_POINT ( 'NONE',  ( -5.000000000000000000, -30.00000000000000000, 0.000000000000000000 ) ) ;
#38902=EDGE_CURVE ( 'NONE', #14226, #33989, #40971, .T. ) ;
#38905=ADVANCED_FACE ( 'NONE', ( #1763 ), #12348, .T. ) ;
#38909=CARTESIAN_POINT ( 'NONE',  ( 9.457646018065525792E-16, -87.31249999863440792, 5.148502694627439702 ) ) ;
#38911=ORIENTED_EDGE ( 'NONE', *, *, #30374, .F. ) ;
#38915=DIRECTION ( 'NONE',  ( 0.000000000000000000, 0.000000000000000000, 1.000000000000000000 ) ) ;
#38917=CARTESIAN_POINT ( 'NONE',  ( -6.972266317189433020E-16, -78.24999999999998579, -5.000000000000000000 ) ) ;
#38918=CARTESIAN_POINT ( 'NONE',  ( -3.152548672688508926E-16, -12.81249999863440259, -5.148502694627439702 ) ) ;
#38921=CARTESIAN_POINT ( 'NONE',  ( -6.972266317189433020E-16, -74.12499999726878741, -5.000000000000000000 ) ) ;
#38923=( BOUNDED_CURVE ( )  B_SPLINE_CURVE ( 2, ( #9460, #23644, #10098, #151, #33600, #34215, #29706, #28764, #62880 ),
 .UNSPECIFIED., .F., .F. ) 
 B_SPLINE_CURVE_WITH_KNOTS ( ( 3, 2, 2, 2, 3 ),
 ( 0.4982142857142857206, 0.4988095238095238138, 0.5000000000000000000, 0.5011904761904761862, 0.5017857142857142794 ),
 .UNSPECIFIED. ) 
 CURVE ( )  GEOMETRIC_REPRESENTATION_ITEM ( )  RATIONAL_B_SPLINE_CURVE ( ( 0.9330127018922194093, 0.9330127018922194093, 1.000000000000000000, 0.8660254037844387076, 1.000000000000000000, 0.8660254037844387076, 1.000000000000000000, 0.9330127018922194093, 0.9330127018922194093 ) ) 
 REPRESENTATION_ITEM ( '' )  );
#38924=CARTESIAN_POINT ( 'NONE',  ( -2.229367062500000163, 21.27083333469892779, -3.861377020970580443 ) ) ;
#38925=ORIENTED_EDGE ( 'NONE', *, *, #26009, .F. ) ;
#38926=CARTESIAN_POINT ( 'NONE',  ( -2.229367062500000163, -93.47916666530106511, -3.861377020970580443 ) ) ;
#38927=CARTESIAN_POINT ( 'NONE',  ( 0.000000000000000000, -120.0000000000000000, 0.000000000000000000 ) ) ;
#38929=CARTESIAN_POINT ( 'NONE',  ( -3.152548672688508926E-16, -16.56249999863440792, -5.148502694627439702 ) ) ;
#38930=CARTESIAN_POINT ( 'NONE',  ( 5.000000000000000000, -39.29166666393548724, -2.886751345948130876 ) ) ;
#38933=CARTESIAN_POINT ( 'NONE',  ( -2.500000000000000444, -43.04166666393548013, -4.330127018922193649 ) ) ;
#38934=CARTESIAN_POINT ( 'NONE',  ( 1.975475456537005874E-15, -41.62499999726880162, 5.000000000000000000 ) ) ;
#38935=CARTESIAN_POINT ( 'NONE',  ( 4.458734124999999437, 18.18750000136559564, -5.460374474430324690E-16 ) ) ;
#38936=CARTESIAN_POINT ( 'NONE',  ( -2.500000000000000444, 11.95833333606451809, -4.330127018922193649 ) ) ;
#38937=VERTEX_POINT ( 'NONE', #56739 ) ;
#38939=CARTESIAN_POINT ( 'NONE',  ( -2.229367062499996610, -63.14583333196774362, 3.861377020970582219 ) ) ;
#38942=CARTESIAN_POINT ( 'NONE',  ( -2.500000000000000444, 10.83333333333333393, -4.330127018922193649 ) ) ;
#38944=CARTESIAN_POINT ( 'NONE',  ( -5.000000000000000000, -98.95833333060214443, -2.886751345948128211 ) ) ;
#38945=CARTESIAN_POINT ( 'NONE',  ( 4.458734125000001214, -50.89583333196772230, 2.574251347313718519 ) ) ;
#38946=CARTESIAN_POINT ( 'NONE',  ( -5.000000000000000000, -90.95833333060213022, -2.886751345948128211 ) ) ;
#38948=CARTESIAN_POINT ( 'NONE',  ( 5.000000000000000000, 25.70833333606452342, -2.886751345948130876 ) ) ;
#38951=CARTESIAN_POINT ( 'NONE',  ( -5.000000000000000000, -37.00000000000000711, 0.000000000000000000 ) ) ;
#38952=CARTESIAN_POINT ( 'NONE',  ( 5.000000000000000000, -98.29166666393545881, -2.886751345948130876 ) ) ;
#38955=CARTESIAN_POINT ( 'NONE',  ( -3.152548672688508926E-16, -100.5624999986344079, -5.148502694627439702 ) ) ;
#38956=CARTESIAN_POINT ( 'NONE',  ( 2.229367062500001939, 2.770833334698928674, 3.861377020970579999 ) ) ;
#38966=FACE_OUTER_BOUND ( 'NONE', #36620, .T. ) ;
#38968=CARTESIAN_POINT ( 'NONE',  ( -5.000000000000000000, 24.99999999999999645, 0.000000000000000000 ) ) ;
#38971=CARTESIAN_POINT ( 'NONE',  ( 4.458734124999999437, -27.06249999863440081, -5.460374474430324690E-16 ) ) ;
#38980=VERTEX_POINT ( 'NONE', #31647 ) ;
#38981=ADVANCED_FACE ( 'NONE', ( #16537 ), #17801, .T. ) ;
#38983=CARTESIAN_POINT ( 'NONE',  ( -3.152548672688508926E-16, -72.81249999863439371, -5.148502694627439702 ) ) ;
#38984=CARTESIAN_POINT ( 'NONE',  ( -1.339745962155612258, 28.79465819873852084, -5.000000000000000888 ) ) ;
#38986=SURFACE_STYLE_FILL_AREA ( #48327 ) ;
#38987=ORIENTED_EDGE ( 'NONE', *, *, #55706, .F. ) ;
#38988=CARTESIAN_POINT ( 'NONE',  ( 1.339745962155615144, 12.29465819873851906, 4.999999999999999112 ) ) ;
#38992=ADVANCED_FACE ( 'NONE', ( #22958 ), #42555, .T. ) ;
#38993=CARTESIAN_POINT ( 'NONE',  ( -2.229367062500000163, 1.270833334698927342, -3.861377020970580443 ) ) ;
#38995=EDGE_CURVE ( 'NONE', #57302, #25237, #28136, .T. ) ;
#38997=CARTESIAN_POINT ( 'NONE',  ( 1.339745962155615144, -69.58034179853028434, 4.999999999999999112 ) ) ;
#39004=ORIENTED_EDGE ( 'NONE', *, *, #51159, .F. ) ;
#39006=CARTESIAN_POINT ( 'NONE',  ( -3.152548672688508926E-16, -75.56249999863440792, -5.148502694627439702 ) ) ;
#39008=CARTESIAN_POINT ( 'NONE',  ( -3.152548672688508926E-16, 0.4375000013655955255, -5.148502694627439702 ) ) ;
#39012=CARTESIAN_POINT ( 'NONE',  ( 4.458734125000001214, -65.14583333196773651, 2.574251347313718519 ) ) ;
#39013=CARTESIAN_POINT ( 'NONE',  ( 2.499999999999998668, -24.20833333060214443, -4.330127018922193649 ) ) ;
#39017=CARTESIAN_POINT ( 'NONE',  ( 9.457646018065525792E-16, -47.06249999863440792, 5.148502694627439702 ) ) ;
#39018=CARTESIAN_POINT ( 'NONE',  ( 2.229367062499998831, -27.89583333196774007, -3.861377020970580887 ) ) ;
#39021=CARTESIAN_POINT ( 'NONE',  ( 1.060575238724906964E-15, 25.25000000000000355, 5.773502691896257311 ) ) ;
#39023=DIRECTION ( 'NONE',  ( -0.000000000000000000, 1.000000000000000000, -0.000000000000000000 ) ) ;
#39024=CARTESIAN_POINT ( 'NONE',  ( 2.229367062499998831, -39.64583333196773651, -3.861377020970580887 ) ) ;
#39025=CARTESIAN_POINT ( 'NONE',  ( -5.000000000000000000, -74.87499999726880162, 0.000000000000000000 ) ) ;
#39027=( BOUNDED_CURVE ( )  B_SPLINE_CURVE ( 2, ( #10436, #44526, #486, #20088, #49678, #21374, #50318, #5623, #39693 ),
 .UNSPECIFIED., .F., .F. ) 
 B_SPLINE_CURVE_WITH_KNOTS ( ( 3, 2, 2, 2, 3 ),
 ( 0.8303571428571429047, 0.8309523809523809978, 0.8321428571428571841, 0.8333333333333333703, 0.8339285714285714635 ),
 .UNSPECIFIED. ) 
 CURVE ( )  GEOMETRIC_REPRESENTATION_ITEM ( )  RATIONAL_B_SPLINE_CURVE ( ( 0.9330127018922194093, 0.9330127018922194093, 1.000000000000000000, 0.8660254037844387076, 1.000000000000000000, 0.8660254037844387076, 1.000000000000000000, 0.9330127018922194093, 0.9330127018922194093 ) ) 
 REPRESENTATION_ITEM ( '' )  );
#39029=CARTESIAN_POINT ( 'NONE',  ( 4.458734125000000326, -74.14583333196773651, 2.574251347313718519 ) ) ;
#39032=FACE_OUTER_BOUND ( 'NONE', #57409, .T. ) ;
#39033=CARTESIAN_POINT ( 'NONE',  ( 0.000000000000000000, -120.0000000000000000, 5.000000000000000000 ) ) ;
#39034=CARTESIAN_POINT ( 'NONE',  ( -4.999999999999999112, -23.91666666666667140, 2.886751345948131764 ) ) ;
#39036=ORIENTED_EDGE ( 'NONE', *, *, #58244, .T. ) ;
#39039=CARTESIAN_POINT ( 'NONE',  ( 0.000000000000000000, -120.0000000000000000, 5.000000000000000000 ) ) ;
#39047=CARTESIAN_POINT ( 'NONE',  ( 2.499999999999998668, 18.66666666666666430, -4.330127018922193649 ) ) ;
#39048=CARTESIAN_POINT ( 'NONE',  ( -4.458734124999998549, -22.22916666530107221, 2.574251347313722516 ) ) ;
#39049=CARTESIAN_POINT ( 'NONE',  ( 2.500000000000002220, 10.45833333606451987, 4.330127018922192761 ) ) ;
#39052=AXIS2_PLACEMENT_3D ( 'NONE', #58271, #19335, #8441 ) ;
#39054=ORIENTED_EDGE ( 'NONE', *, *, #1931, .T. ) ;
#39057=CARTESIAN_POINT ( 'NONE',  ( 2.499999999999998668, -4.333333333333334814, -4.330127018922193649 ) ) ;
#39058=CARTESIAN_POINT ( 'NONE',  ( -1.339745962155613812, -3.205341801261480938, -5.000000000000000000 ) ) ;
#39060=ORIENTED_EDGE ( 'NONE', *, *, #18161, .T. ) ;
#39062=FACE_OUTER_BOUND ( 'NONE', #4047, .T. ) ;
#39064=CARTESIAN_POINT ( 'NONE',  ( 2.500000000000002220, -53.54166666393548013, 4.330127018922192761 ) ) ;
#39067=CARTESIAN_POINT ( 'NONE',  ( -4.330127018922205195, 45.00000000000000000, -7.499999999999943157 ) ) ;
#39068=CARTESIAN_POINT ( 'NONE',  ( 4.458734124999998549, 19.27083333469893134, -2.574251347313721627 ) ) ;
#39069=DIRECTION ( 'NONE',  ( -0.000000000000000000, 1.000000000000000000, -0.000000000000000000 ) ) ;
#39070=( BOUNDED_CURVE ( )  B_SPLINE_CURVE ( 2, ( #15428, #40494, #11227, #1294, #637, #39849, #6101, #60135, #34717 ),
 .UNSPECIFIED., .F., .F. ) 
 B_SPLINE_CURVE_WITH_KNOTS ( ( 3, 2, 2, 2, 3 ),
 ( 0.3803571428571428381, 0.3809523809523809312, 0.3821428571428571175, 0.3833333333333333592, 0.3839285714285714524 ),
 .UNSPECIFIED. ) 
 CURVE ( )  GEOMETRIC_REPRESENTATION_ITEM ( )  RATIONAL_B_SPLINE_CURVE ( ( 0.9330127018922194093, 0.9330127018922194093, 1.000000000000000000, 0.8660254037844387076, 1.000000000000000000, 0.8660254037844387076, 1.000000000000000000, 0.9330127018922194093, 0.9330127018922194093 ) ) 
 REPRESENTATION_ITEM ( '' )  );
#39071=ORIENTED_EDGE ( 'NONE', *, *, #56737, .F. ) ;
#39075=CARTESIAN_POINT ( 'NONE',  ( 2.499999999999998668, -100.3333333333333286, -4.330127018922193649 ) ) ;
#39076=( BOUNDED_CURVE ( )  B_SPLINE_CURVE ( 2, ( #30365, #33922, #49027, #25547, #40011, #29081, #15589, #48708, #38737 ),
 .UNSPECIFIED., .F., .F. ) 
 B_SPLINE_CURVE_WITH_KNOTS ( ( 3, 2, 2, 2, 3 ),
 ( 0.2732142857142857428, 0.2738095238095238360, 0.2750000000000000222, 0.2761904761904762085, 0.2767857142857143016 ),
 .UNSPECIFIED. ) 
 CURVE ( )  GEOMETRIC_REPRESENTATION_ITEM ( )  RATIONAL_B_SPLINE_CURVE ( ( 0.9330127018922194093, 0.9330127018922225179, 1.000000000000000000, 0.8660254037844387076, 1.000000000000000000, 0.8660254037844387076, 1.000000000000000000, 0.9330127018922194093, 0.9330127018922194093 ) ) 
 REPRESENTATION_ITEM ( '' )  );
#39077=CARTESIAN_POINT ( 'NONE',  ( 2.229367062499998831, -58.64583333196773651, -3.861377020970580887 ) ) ;
#39079=CARTESIAN_POINT ( 'NONE',  ( -4.458734124999999437, 18.68750000136559564, 0.000000000000000000 ) ) ;
#39081=CARTESIAN_POINT ( 'NONE',  ( -4.458734124999998549, -49.47916666530106511, 2.574251347313722516 ) ) ;
#39082=CARTESIAN_POINT ( 'NONE',  ( -2.499999999999996447, -8.708333330602144429, 4.330127018922195425 ) ) ;
#39085=CARTESIAN_POINT ( 'NONE',  ( -3.152548672688508926E-16, -108.5624999986343937, -5.148502694627439702 ) ) ;
#39086=CARTESIAN_POINT ( 'NONE',  ( 4.458734125000000326, -10.14583333196773829, 2.574251347313718519 ) ) ;
#39087=ORIENTED_EDGE ( 'NONE', *, *, #4010, .T. ) ;
#39089=CARTESIAN_POINT ( 'NONE',  ( -3.152548672688508926E-16, -98.56249999863442213, -5.148502694627439702 ) ) ;
#39091=CARTESIAN_POINT ( 'NONE',  ( -4.458734124999999437, -98.56249999863440792, 0.000000000000000000 ) ) ;
#39094=CARTESIAN_POINT ( 'NONE',  ( -2.499999999999996447, -49.70833333060213732, 4.330127018922195425 ) ) ;
#39095=CARTESIAN_POINT ( 'NONE',  ( 1.975475456537005874E-15, -84.62499999726880162, 5.000000000000000000 ) ) ;
#39098=CARTESIAN_POINT ( 'NONE',  ( 4.458734124999998549, -20.72916666530107221, -2.574251347313721627 ) ) ;
#39099=CARTESIAN_POINT ( 'NONE',  ( 4.458734124999998549, 5.020833334698926897, -2.574251347313721627 ) ) ;
#39100=( BOUNDED_CURVE ( )  B_SPLINE_CURVE ( 2, ( #27818, #3395, #52278, #38113, #27195, #28134, #32648, #62571, #56479 ),
 .UNSPECIFIED., .F., .F. ) 
 B_SPLINE_CURVE_WITH_KNOTS ( ( 3, 2, 2, 2, 3 ),
 ( 0.7874999999999999778, 0.7880952380952380709, 0.7892857142857142572, 0.7904761904761904434, 0.7910714285714285365 ),
 .UNSPECIFIED. ) 
 CURVE ( )  GEOMETRIC_REPRESENTATION_ITEM ( )  RATIONAL_B_SPLINE_CURVE ( ( 0.9330127018922194093, 0.9330127018922194093, 1.000000000000000000, 0.8660254037844387076, 1.000000000000000000, 0.8660254037844387076, 1.000000000000000000, 0.9330127018922194093, 0.9330127018922194093 ) ) 
 REPRESENTATION_ITEM ( '' )  );
#39101=CARTESIAN_POINT ( 'NONE',  ( -3.152548672688508926E-16, -57.81249999863440081, -5.148502694627439702 ) ) ;
#39106=CARTESIAN_POINT ( 'NONE',  ( 2.500000000000002220, -8.666666666666669627, 4.330127018922192761 ) ) ;
#39107=VERTEX_POINT ( 'NONE', #14538 ) ;
#39111=CARTESIAN_POINT ( 'NONE',  ( -5.000000000000000000, -66.87499999726881583, 0.000000000000000000 ) ) ;
#39112=CARTESIAN_POINT ( 'NONE',  ( 4.458734124999999437, -87.81249999863439371, -5.460374474430324690E-16 ) ) ;
#39113=CARTESIAN_POINT ( 'NONE',  ( 2.229367062500001939, 18.77083333469892779, 3.861377020970579999 ) ) ;
#39115=CARTESIAN_POINT ( 'NONE',  ( -6.972266317189433020E-16, -82.24999999999998579, -5.000000000000000000 ) ) ;
#39116=LINE ( 'NONE', #19182, #19402 ) ;
#39119=CARTESIAN_POINT ( 'NONE',  ( 1.060575238724906964E-15, -77.75000000000000000, 5.773502691896257311 ) ) ;
#39124=( BOUNDED_CURVE ( )  B_SPLINE_CURVE ( 2, ( #61527, #57956, #18702, #17765, #47039, #48281, #62475, #52808, #13877 ),
 .UNSPECIFIED., .F., .F. ) 
 B_SPLINE_CURVE_WITH_KNOTS ( ( 3, 2, 2, 2, 3 ),
 ( 0.7089285714285714635, 0.7095238095238095566, 0.7107142857142857428, 0.7119047619047619291, 0.7125000000000000222 ),
 .UNSPECIFIED. ) 
 CURVE ( )  GEOMETRIC_REPRESENTATION_ITEM ( )  RATIONAL_B_SPLINE_CURVE ( ( 0.9330127018922194093, 0.9330127018922194093, 1.000000000000000000, 0.8660254037844387076, 1.000000000000000000, 0.8660254037844387076, 1.000000000000000000, 0.9330127018922194093, 0.9330127018922194093 ) ) 
 REPRESENTATION_ITEM ( '' )  );
#39137=CARTESIAN_POINT ( 'NONE',  ( -2.229367062499996610, -58.39583333196773651, 3.861377020970582219 ) ) ;
#39146=CARTESIAN_POINT ( 'NONE',  ( 2.229367062500001939, -106.2291666653010651, 3.861377020970579999 ) ) ;
#39147=CARTESIAN_POINT ( 'NONE',  ( -1.339745962155613812, -69.08034179853028434, -5.000000000000000000 ) ) ;
#39150=AXIS2_PLACEMENT_3D ( 'NONE', #1215, #35605, #49437 ) ;
#39152=CARTESIAN_POINT ( 'NONE',  ( 2.229367062499998831, -39.64583333196773651, -3.861377020970580887 ) ) ;
#39155=CARTESIAN_POINT ( 'NONE',  ( 5.000000000000000000, 29.50000000000000000, -6.123233995736766282E-16 ) ) ;
#39156=CARTESIAN_POINT ( 'NONE',  ( -4.458734124999998549, -15.22916666530107754, 2.574251347313722516 ) ) ;
#39157=CARTESIAN_POINT ( 'NONE',  ( 4.458734125000000326, -101.1458333319677365, 2.574251347313718519 ) ) ;
#39158=ORIENTED_EDGE ( 'NONE', *, *, #57204, .T. ) ;
#39160=CARTESIAN_POINT ( 'NONE',  ( -4.458734124999998549, -35.47916666530107221, 2.574251347313722516 ) ) ;
#39161=CARTESIAN_POINT ( 'NONE',  ( 1.060575238724906964E-15, 5.375000002731184168, 5.773502691896257311 ) ) ;
#39165=CYLINDRICAL_SURFACE ( 'NONE', #18864, 5.000000000000000000 ) ;
#39168=CARTESIAN_POINT ( 'NONE',  ( -4.458734124999999437, 6.354166668032259047, -2.574251347313719407 ) ) ;
#39169=ORIENTED_EDGE ( 'NONE', *, *, #18881, .T. ) ;
#39170=CARTESIAN_POINT ( 'NONE',  ( -5.000000000000000000, 16.04166666939785202, -2.886751345948128211 ) ) ;
#39171=CARTESIAN_POINT ( 'NONE',  ( 5.000000000000000888, -93.58333333333332860, 2.886751345948126879 ) ) ;
#39172=CARTESIAN_POINT ( 'NONE',  ( 9.457646018065525792E-16, -28.06249999863440081, 5.148502694627439702 ) ) ;
#39173=CARTESIAN_POINT ( 'NONE',  ( 1.339745962155612702, -95.29465819873851729, -5.000000000000000000 ) ) ;
#39174=CARTESIAN_POINT ( 'NONE',  ( 4.458734125000001214, -82.14583333196772230, 2.574251347313718519 ) ) ;
#39178=CARTESIAN_POINT ( 'NONE',  ( -2.229367062499996610, -1.145833331967736957, 3.861377020970582219 ) ) ;
#39179=CARTESIAN_POINT ( 'NONE',  ( -2.229367062500000163, 27.27083333469892779, -3.861377020970580443 ) ) ;
#39180=CARTESIAN_POINT ( 'NONE',  ( 2.229367062499998831, -41.89583333196773651, -3.861377020970580887 ) ) ;
#39183=ORIENTED_EDGE ( 'NONE', *, *, #29558, .F. ) ;
#39186=CARTESIAN_POINT ( 'NONE',  ( 2.229367062500001939, -66.97916666530106511, 3.861377020970579999 ) ) ;
#39187=CARTESIAN_POINT ( 'NONE',  ( -3.535250795749689387E-16, -106.1249999972688300, -5.773502691896257311 ) ) ;
#39188=EDGE_CURVE ( 'NONE', #13925, #60011, #13915, .T. ) ;
#39190=DIRECTION ( 'NONE',  ( -0.000000000000000000, 1.000000000000000000, -0.000000000000000000 ) ) ;
#39193=CARTESIAN_POINT ( 'NONE',  ( -2.499999999999996447, -60.83333333333333570, 4.330127018922195425 ) ) ;
#39194=CARTESIAN_POINT ( 'NONE',  ( -1.339745962155613812, -22.20534180126147561, -5.000000000000000000 ) ) ;
#39196=EDGE_LOOP ( 'NONE', ( #8850, #40386, #6486, #62621 ) ) ;
#39201=( BOUNDED_CURVE ( )  B_SPLINE_CURVE ( 2, ( #27430, #12643, #8149, #47063, #32580, #41905, #27125, #62178, #47377 ),
 .UNSPECIFIED., .F., .F. ) 
 B_SPLINE_CURVE_WITH_KNOTS ( ( 3, 2, 2, 2, 3 ),
 ( 0.2982142857142857095, 0.2988095238095238027, 0.2999999999999999889, 0.3011904761904761751, 0.3017857142857142683 ),
 .UNSPECIFIED. ) 
 CURVE ( )  GEOMETRIC_REPRESENTATION_ITEM ( )  RATIONAL_B_SPLINE_CURVE ( ( 0.9330127018922194093, 0.9330127018922194093, 1.000000000000000000, 0.8660254037844387076, 1.000000000000000000, 0.8660254037844387076, 1.000000000000000000, 0.9330127018922194093, 0.9330127018922194093 ) ) 
 REPRESENTATION_ITEM ( '' )  );
#39203=EDGE_CURVE ( 'NONE', #19510, #57924, #61413, .T. ) ;
#39207=CARTESIAN_POINT ( 'NONE',  ( -6.972266317189433020E-16, -24.24999999999999645, -5.000000000000000000 ) ) ;
#39214=CARTESIAN_POINT ( 'NONE',  ( -4.458734124999999437, -41.64583333196773651, -2.574251347313719407 ) ) ;
#39221=( BOUNDED_CURVE ( )  B_SPLINE_CURVE ( 2, ( #59642, #35832, #41267, #25534, #16837, #50297, #46109, #21677, #45151 ),
 .UNSPECIFIED., .F., .F. ) 
 B_SPLINE_CURVE_WITH_KNOTS ( ( 3, 2, 2, 2, 3 ),
 ( 0.7410714285714286031, 0.7416666666666666963, 0.7428571428571428825, 0.7440476190476190688, 0.7446428571428571619 ),
 .UNSPECIFIED. ) 
 CURVE ( )  GEOMETRIC_REPRESENTATION_ITEM ( )  RATIONAL_B_SPLINE_CURVE ( ( 0.9330127018922194093, 0.9330127018922194093, 1.000000000000000000, 0.8660254037844387076, 1.000000000000000000, 0.8660254037844387076, 1.000000000000000000, 0.9330127018922194093, 0.9330127018922194093 ) ) 
 REPRESENTATION_ITEM ( '' )  );
#39224=CARTESIAN_POINT ( 'NONE',  ( -4.458734124999999437, -87.64583333196773651, -2.574251347313719407 ) ) ;
#39226=ORIENTED_EDGE ( 'NONE', *, *, #42264, .T. ) ;
#39227=CARTESIAN_POINT ( 'NONE',  ( 1.339745962155615144, -19.58034179853029499, 4.999999999999999112 ) ) ;
#39232=CARTESIAN_POINT ( 'NONE',  ( -4.458734124999999437, 0.6875000013655957476, 0.000000000000000000 ) ) ;
#39233=CARTESIAN_POINT ( 'NONE',  ( 1.339745962155615144, -78.70534180126148271, 4.999999999999999112 ) ) ;
#39234=CARTESIAN_POINT ( 'NONE',  ( 4.458734124999998549, -14.97916666530107221, -2.574251347313721627 ) ) ;
#39238=CARTESIAN_POINT ( 'NONE',  ( -4.458734124999999437, 21.43750000136559208, 0.000000000000000000 ) ) ;
#39240=CARTESIAN_POINT ( 'NONE',  ( -4.458734124999999437, -99.39583333196772230, -2.574251347313719407 ) ) ;
#39241=DIRECTION ( 'NONE',  ( -0.000000000000000000, 1.000000000000000000, -0.000000000000000000 ) ) ;
#39243=CARTESIAN_POINT ( 'NONE',  ( -3.152548672688508926E-16, -13.56249999863440259, -5.148502694627439702 ) ) ;
#39244=CARTESIAN_POINT ( 'NONE',  ( 1.975475456537005874E-15, -39.62499999726880162, 5.000000000000000000 ) ) ;
#39247=CARTESIAN_POINT ( 'NONE',  ( -5.000000000000000000, -39.87499999726880162, 0.000000000000000000 ) ) ;
#39248=CARTESIAN_POINT ( 'NONE',  ( 2.499999999999998668, -67.20833333060214443, -4.330127018922193649 ) ) ;
#39249=CARTESIAN_POINT ( 'NONE',  ( -2.229367062500000163, 12.52083333469892601, -3.861377020970580443 ) ) ;
#39250=CARTESIAN_POINT ( 'NONE',  ( -6.972266317189433020E-16, -95.25000000000000000, -5.000000000000000000 ) ) ;
#39251=VERTEX_POINT ( 'NONE', #20396 ) ;
#39253=CARTESIAN_POINT ( 'NONE',  ( -2.229367062500000163, -59.47916666530106511, -3.861377020970580443 ) ) ;
#39257=CARTESIAN_POINT ( 'NONE',  ( 5.000000000000000888, 6.416666666666666963, 2.886751345948126879 ) ) ;
#39260=CARTESIAN_POINT ( 'NONE',  ( 4.458734124999999437, -51.81249999863440792, -5.460374474430324690E-16 ) ) ;
#39261=CARTESIAN_POINT ( 'NONE',  ( 5.000000000000000000, -87.37499999726880162, -6.123233995736766282E-16 ) ) ;
#39263=CARTESIAN_POINT ( 'NONE',  ( -2.229367062499996610, -32.14583333196773651, 3.861377020970582219 ) ) ;
#39264=FACE_OUTER_BOUND ( 'NONE', #58942, .T. ) ;
#39267=CARTESIAN_POINT ( 'NONE',  ( -3.535250795749689387E-16, -40.24999999999998579, -5.773502691896257311 ) ) ;
#39269=CARTESIAN_POINT ( 'NONE',  ( 6.123233995736766282E-16, -120.0000000000000000, -5.000000000000000000 ) ) ;
#39271=CARTESIAN_POINT ( 'NONE',  ( -4.458734124999998549, -99.22916666530105090, 2.574251347313722516 ) ) ;
#39272=CARTESIAN_POINT ( 'NONE',  ( -4.458734124999998549, 0.5208333346989265644, 2.574251347313722516 ) ) ;
#39281=ORIENTED_EDGE ( 'NONE', *, *, #10240, .T. ) ;
#39282=CARTESIAN_POINT ( 'NONE',  ( 1.975475456537005874E-15, -10.75000000000000000, 5.000000000000000000 ) ) ;
#39284=EDGE_CURVE ( 'NONE', #19571, #6165, #25702, .T. ) ;
#39288=CARTESIAN_POINT ( 'NONE',  ( -4.458734124999998549, -24.47916666530107577, 2.574251347313722516 ) ) ;
#39289=CARTESIAN_POINT ( 'NONE',  ( -1.336351044127974539E-14, 22.37500000273118417, 5.000000000000000000 ) ) ;
#39298=ORIENTED_EDGE ( 'NONE', *, *, #767, .F. ) ;
#39299=CARTESIAN_POINT ( 'NONE',  ( 4.458734124999998549, -73.97916666530106511, -2.574251347313721627 ) ) ;
#39301=ORIENTED_EDGE ( 'NONE', *, *, #57129, .F. ) ;
#39302=CARTESIAN_POINT ( 'NONE',  ( -6.000000000000000000, -114.9999999999999858, -1.500000000000000000 ) ) ;
#39303=( BOUNDED_CURVE ( )  B_SPLINE_CURVE ( 2, ( #41314, #47417, #7873, #46472, #52250, #21719, #32942, #36497, #51623 ),
 .UNSPECIFIED., .F., .F. ) 
 B_SPLINE_CURVE_WITH_KNOTS ( ( 3, 2, 2, 2, 3 ),
 ( 0.6803571428571428825, 0.6809523809523809756, 0.6821428571428571619, 0.6833333333333333481, 0.6839285714285714413 ),
 .UNSPECIFIED. ) 
 CURVE ( )  GEOMETRIC_REPRESENTATION_ITEM ( )  RATIONAL_B_SPLINE_CURVE ( ( 0.9330127018922194093, 0.9330127018922194093, 1.000000000000000000, 0.8660254037844387076, 1.000000000000000000, 0.8660254037844387076, 1.000000000000000000, 0.9330127018922194093, 0.9330127018922194093 ) ) 
 REPRESENTATION_ITEM ( '' )  );
#39305=EDGE_CURVE ( 'NONE', #27512, #42376, #4959, .T. ) ;
#39307=CARTESIAN_POINT ( 'NONE',  ( -4.458734124999999437, 2.437500001365593860, 0.000000000000000000 ) ) ;
#39308=ORIENTED_EDGE ( 'NONE', *, *, #11795, .F. ) ;
#39310=CARTESIAN_POINT ( 'NONE',  ( -6.972266317189433020E-16, -108.2499999999999858, -5.000000000000000000 ) ) ;
#39315=CARTESIAN_POINT ( 'NONE',  ( -4.458734124999999437, -81.31249999863440792, 0.000000000000000000 ) ) ;
#39317=CARTESIAN_POINT ( 'NONE',  ( -4.458734124999999437, 0.6875000013655957476, 0.000000000000000000 ) ) ;
#39318=CARTESIAN_POINT ( 'NONE',  ( -5.000000000000000000, -86.08333333333334281, -2.886751345948128211 ) ) ;
#39320=CARTESIAN_POINT ( 'NONE',  ( -3.152548672688508926E-16, -65.81249999863440792, -5.148502694627439702 ) ) ;
#39321=CARTESIAN_POINT ( 'NONE',  ( -2.499999999999996447, -23.70833333060214443, 4.330127018922195425 ) ) ;
#39323=CARTESIAN_POINT ( 'NONE',  ( -1.339745962155610925, -40.79465819873852439, 5.000000000000000000 ) ) ;
#39326=CARTESIAN_POINT ( 'NONE',  ( -4.458734124999999437, -48.31249999863440792, 0.000000000000000000 ) ) ;
#39327=CARTESIAN_POINT ( 'NONE',  ( -4.458734124999997661, -33.47916666530107221, 2.574251347313722516 ) ) ;
#39330=CARTESIAN_POINT ( 'NONE',  ( -4.999999999999999112, 25.08333333333333215, 2.886751345948131764 ) ) ;
#39333=CARTESIAN_POINT ( 'NONE',  ( -4.458734124999999437, -36.39583333196772941, -2.574251347313719407 ) ) ;
#39334=CARTESIAN_POINT ( 'NONE',  ( 1.060575238724906964E-15, -74.62499999726880162, 5.773502691896257311 ) ) ;
#39339=CARTESIAN_POINT ( 'NONE',  ( 5.000000000000000000, -37.50000000000000711, -6.123233995736766282E-16 ) ) ;
#39341=CARTESIAN_POINT ( 'NONE',  ( -2.229367062499996610, -75.39583333196773651, 3.861377020970582219 ) ) ;
#39347=CARTESIAN_POINT ( 'NONE',  ( 2.500000000000002220, -21.66666666666666785, 4.330127018922192761 ) ) ;
#39351=ORIENTED_EDGE ( 'NONE', *, *, #58568, .F. ) ;
#39353=CARTESIAN_POINT ( 'NONE',  ( -2.499999999999996447, 24.29166666939785202, 4.330127018922195425 ) ) ;
#39355=EDGE_CURVE ( 'NONE', #50310, #9796, #56899, .T. ) ;
#39358=CARTESIAN_POINT ( 'NONE',  ( -2.499999999999996447, 4.166666666666666075, 4.330127018922195425 ) ) ;
#39360=CARTESIAN_POINT ( 'NONE',  ( 2.493747252781420335E-13, -56.12499999726880873, -5.000000000000000000 ) ) ;
#39362=CARTESIAN_POINT ( 'NONE',  ( 9.457646018065525792E-16, -20.06249999863440081, 5.148502694627439702 ) ) ;
#39366=EDGE_CURVE ( 'NONE', #40791, #7933, #12918, .T. ) ;
#39368=ORIENTED_EDGE ( 'NONE', *, *, #53512, .F. ) ;
#39371=EDGE_LOOP ( 'NONE', ( #18770, #57863, #53797, #47167 ) ) ;
#39373=CARTESIAN_POINT ( 'NONE',  ( -5.000000000000000000, -67.95833333060214443, -2.886751345948128211 ) ) ;
#39376=CARTESIAN_POINT ( 'NONE',  ( -6.972266317189433020E-16, 10.75000000000000000, -5.000000000000000000 ) ) ;
#39382=CARTESIAN_POINT ( 'NONE',  ( -4.458734124999999437, 17.60416666803225993, -2.574251347313719407 ) ) ;
#39383=CARTESIAN_POINT ( 'NONE',  ( -5.000000000000000000, -85.08333333333332860, -2.886751345948128211 ) ) ;
#39390=CARTESIAN_POINT ( 'NONE',  ( 2.229367062500001939, -59.97916666530106511, 3.861377020970579999 ) ) ;
#39391=CARTESIAN_POINT ( 'NONE',  ( 4.458734124999998549, 20.27083333469892779, -2.574251347313721627 ) ) ;
#39394=CARTESIAN_POINT ( 'NONE',  ( -2.229367062499996610, -48.39583333196772941, 3.861377020970582219 ) ) ;
#39395=CARTESIAN_POINT ( 'NONE',  ( -4.999999999999999112, -7.791666663935482795, 2.886751345948131764 ) ) ;
#39397=FACE_OUTER_BOUND ( 'NONE', #57530, .T. ) ;
#39398=CARTESIAN_POINT ( 'NONE',  ( 4.458734124999998549, -106.7291666653010509, -2.574251347313721627 ) ) ;
#39399=CARTESIAN_POINT ( 'NONE',  ( 9.457646018065525792E-16, -9.312499998634406140, 5.148502694627439702 ) ) ;
#39400=VERTEX_POINT ( 'NONE', #11683 ) ;
#39401=CARTESIAN_POINT ( 'NONE',  ( 1.975475456537005874E-15, -46.62499999726880873, 5.000000000000000000 ) ) ;
#39402=CARTESIAN_POINT ( 'NONE',  ( 4.458734124999998549, -96.72916666530105090, -2.574251347313721627 ) ) ;
#39404=CARTESIAN_POINT ( 'NONE',  ( 4.458734124999998549, -99.97916666530106511, -2.574251347313721627 ) ) ;
#39405=CARTESIAN_POINT ( 'NONE',  ( -5.000000000000000000, -8.083333333333332149, -2.886751345948128211 ) ) ;
#39406=CARTESIAN_POINT ( 'NONE',  ( -3.535250795749689387E-16, -59.12499999726880873, -5.773502691896257311 ) ) ;
#39407=CYLINDRICAL_SURFACE ( 'NONE', #20209, 5.000000000000000000 ) ;
#39410=ADVANCED_FACE ( 'NONE', ( #41266 ), #6556, .T. ) ;
#39411=CARTESIAN_POINT ( 'NONE',  ( 4.458734124999998549, -15.72916666530107399, -2.574251347313721627 ) ) ;
#39412=CARTESIAN_POINT ( 'NONE',  ( -3.152548672688508926E-16, 8.187500001365595637, -5.148502694627439702 ) ) ;
#39413=CARTESIAN_POINT ( 'NONE',  ( 9.457646018065525792E-16, -58.31249999863440792, 5.148502694627439702 ) ) ;
#39414=CARTESIAN_POINT ( 'NONE',  ( 2.493747252781420335E-13, -56.12499999726880873, -5.000000000000000000 ) ) ;
#39416=CARTESIAN_POINT ( 'NONE',  ( 2.499999999999998668, -8.208333330602144429, -4.330127018922193649 ) ) ;
#39418=CARTESIAN_POINT ( 'NONE',  ( 5.000000000000000000, -6.499999999999999112, -6.123233995736766282E-16 ) ) ;
#39421=CARTESIAN_POINT ( 'NONE',  ( -6.972266317189433020E-16, -38.25000000000000000, -5.000000000000000000 ) ) ;
#39422=DIRECTION ( 'NONE',  ( 0.000000000000000000, 0.000000000000000000, 1.000000000000000000 ) ) ;
#39423=CARTESIAN_POINT ( 'NONE',  ( 4.458734125000001214, -84.89583333196773651, 2.574251347313718519 ) ) ;
#39424=CARTESIAN_POINT ( 'NONE',  ( 2.229367062499998831, 21.10416666803226349, -3.861377020970580887 ) ) ;
#39425=AXIS2_PLACEMENT_3D ( 'NONE', #13228, #43119, #18679 ) ;
#39427=CARTESIAN_POINT ( 'NONE',  ( -5.000000000000000000, -88.95833333060214443, -2.886751345948128211 ) ) ;
#39431=CARTESIAN_POINT ( 'NONE',  ( 5.000000000000000000, -73.41666666666665719, -2.886751345948129988 ) ) ;
#39433=EDGE_CURVE ( 'NONE', #42937, #21194, #41650, .T. ) ;
#39434=EDGE_LOOP ( 'NONE', ( #3485, #29968, #47128, #54652 ) ) ;
#39435=CARTESIAN_POINT ( 'NONE',  ( 1.975475456537005874E-15, -96.62499999726880162, 5.000000000000000000 ) ) ;
#39436=ADVANCED_FACE ( 'NONE', ( #50296 ), #50938, .T. ) ;
#39438=CARTESIAN_POINT ( 'NONE',  ( 1.975475456537005874E-15, -103.7500000000000000, 5.000000000000000000 ) ) ;
#39453=CARTESIAN_POINT ( 'NONE',  ( -4.458734124999998549, -56.47916666530107221, 2.574251347313722516 ) ) ;
#39454=( BOUNDED_CURVE ( )  B_SPLINE_CURVE ( 2, ( #40546, #41489, #16107, #11274, #61141, #36362, #23076, #36050, #31213 ),
 .UNSPECIFIED., .F., .F. ) 
 B_SPLINE_CURVE_WITH_KNOTS ( ( 3, 2, 2, 2, 3 ),
 ( 0.7125000000000000222, 0.7130952380952381153, 0.7142857142857143016, 0.7154761904761904878, 0.7160714285714285809 ),
 .UNSPECIFIED. ) 
 CURVE ( )  GEOMETRIC_REPRESENTATION_ITEM ( )  RATIONAL_B_SPLINE_CURVE ( ( 0.9330127018922194093, 0.9330127018922194093, 1.000000000000000000, 0.8660254037844387076, 1.000000000000000000, 0.8660254037844387076, 1.000000000000000000, 0.9330127018922194093, 0.9330127018922194093 ) ) 
 REPRESENTATION_ITEM ( '' )  );
#39457=ORIENTED_EDGE ( 'NONE', *, *, #59143, .F. ) ;
#39463=CARTESIAN_POINT ( 'NONE',  ( -2.229367062500000163, -105.7291666653010651, -3.861377020970580443 ) ) ;
#39465=ORIENTED_EDGE ( 'NONE', *, *, #51869, .F. ) ;
#39468=CARTESIAN_POINT ( 'NONE',  ( -3.152548672688508926E-16, -43.56249999863439371, -5.148502694627439702 ) ) ;
#39471=CARTESIAN_POINT ( 'NONE',  ( -2.500000000000000444, -71.16666666666667140, -4.330127018922193649 ) ) ;
#39472=CARTESIAN_POINT ( 'NONE',  ( -4.458734124999999437, -12.39583333196774184, -2.574251347313719407 ) ) ;
#39473=CARTESIAN_POINT ( 'NONE',  ( 5.000000000000000000, -101.5000000000000000, -6.123233995736766282E-16 ) ) ;
#39477=CARTESIAN_POINT ( 'NONE',  ( -4.458734124999999437, -34.56249999863440792, 0.000000000000000000 ) ) ;
#39478=CARTESIAN_POINT ( 'NONE',  ( 2.500000000000002220, 8.458333336064518093, 4.330127018922192761 ) ) ;
#39484=DIRECTION ( 'NONE',  ( 1.000000000000000000, 0.000000000000000000, -3.614007241618347908E-17 ) ) ;
#39485=CARTESIAN_POINT ( 'NONE',  ( 4.458734124999998549, 5.020833334698926897, -2.574251347313721627 ) ) ;
#39486=ORIENTED_EDGE ( 'NONE', *, *, #20596, .T. ) ;
#39488=CARTESIAN_POINT ( 'NONE',  ( -5.000000000000000000, -76.08333333333334281, -2.886751345948128211 ) ) ;
#39489=CARTESIAN_POINT ( 'NONE',  ( -3.535250795749689387E-16, -96.25000000000000000, -5.773502691896257311 ) ) ;
#39490=CARTESIAN_POINT ( 'NONE',  ( -4.458734124999999437, -29.39583333196773296, -2.574251347313719407 ) ) ;
#39491=CARTESIAN_POINT ( 'NONE',  ( 0.000000000000000000, -120.0000000000000000, 0.000000000000000000 ) ) ;
#39492=CARTESIAN_POINT ( 'NONE',  ( -3.152548672688508926E-16, -81.81249999863440792, -5.148502694627439702 ) ) ;
#39496=CARTESIAN_POINT ( 'NONE',  ( 2.229367062500001939, -1.979166665301068662, 3.861377020970579999 ) ) ;
#39497=CARTESIAN_POINT ( 'NONE',  ( -2.229367062500000163, 23.27083333469892779, -3.861377020970580443 ) ) ;
#39498=CARTESIAN_POINT ( 'NONE',  ( -2.229367062499996610, -43.39583333196773651, 3.861377020970582219 ) ) ;
#39503=( BOUNDED_CURVE ( )  B_SPLINE_CURVE ( 2, ( #26695, #3210, #47265, #56610, #46628, #17678, #21873, #12527, #22830 ),
 .UNSPECIFIED., .F., .F. ) 
 B_SPLINE_CURVE_WITH_KNOTS ( ( 3, 2, 2, 2, 3 ),
 ( 0.5839285714285714635, 0.5845238095238095566, 0.5857142857142857428, 0.5869047619047619291, 0.5875000000000000222 ),
 .UNSPECIFIED. ) 
 CURVE ( )  GEOMETRIC_REPRESENTATION_ITEM ( )  RATIONAL_B_SPLINE_CURVE ( ( 0.9330127018922194093, 0.9330127018922194093, 1.000000000000000000, 0.8660254037844387076, 1.000000000000000000, 0.8660254037844387076, 1.000000000000000000, 0.9330127018922194093, 0.9330127018922194093 ) ) 
 REPRESENTATION_ITEM ( '' )  );
#39504=CARTESIAN_POINT ( 'NONE',  ( -4.458734124999999437, -67.39583333196773651, -2.574251347313719407 ) ) ;
#39505=CARTESIAN_POINT ( 'NONE',  ( 2.499999999999998668, -106.2083333306021444, -4.330127018922193649 ) ) ;
#39507=CARTESIAN_POINT ( 'NONE',  ( 5.000000000000000000, -58.37499999726880873, -6.123233995736766282E-16 ) ) ;
#39510=CARTESIAN_POINT ( 'NONE',  ( 5.000000000000000000, -58.50000000000000000, -6.123233995736766282E-16 ) ) ;
#39523=CARTESIAN_POINT ( 'NONE',  ( 1.339745962155615144, -45.58034179853028434, 4.999999999999999112 ) ) ;
#39529=CARTESIAN_POINT ( 'NONE',  ( -3.152548672688508926E-16, -43.81249999863440081, -5.148502694627439702 ) ) ;
#39530=CARTESIAN_POINT ( 'NONE',  ( 5.000000000000000000, -68.29166666393547303, -2.886751345948130876 ) ) ;
#39536=CARTESIAN_POINT ( 'NONE',  ( 5.000000000000000000, -89.50000000000000000, -6.123233995736766282E-16 ) ) ;
#39538=CARTESIAN_POINT ( 'NONE',  ( -3.152548672688508926E-16, -90.81249999863440792, -5.148502694627439702 ) ) ;
#39539=CARTESIAN_POINT ( 'NONE',  ( 1.975475456537005874E-15, -17.62499999726881583, 5.000000000000000000 ) ) ;
#39540=ORIENTED_EDGE ( 'NONE', *, *, #52384, .F. ) ;
#39541=CARTESIAN_POINT ( 'NONE',  ( -6.972266317189433020E-16, -32.24999999999999289, -5.000000000000000000 ) ) ;
#39544=LINE ( 'NONE', #60152, #10602 ) ;
#39547=CARTESIAN_POINT ( 'NONE',  ( 2.229367062500001939, 1.020833334698927120, 3.861377020970579999 ) ) ;
#39549=CARTESIAN_POINT ( 'NONE',  ( -4.458734124999999437, -18.64583333196774007, -2.574251347313719407 ) ) ;
#39554=CARTESIAN_POINT ( 'NONE',  ( 9.457646018065525792E-16, 20.68750000136559208, 5.148502694627439702 ) ) ;
#39555=ORIENTED_EDGE ( 'NONE', *, *, #19324, .T. ) ;
#39556=CARTESIAN_POINT ( 'NONE',  ( 4.458734124999998549, -99.72916666530106511, -2.574251347313721627 ) ) ;
#39559=CARTESIAN_POINT ( 'NONE',  ( 4.458734124999998549, -13.72916666530107399, -2.574251347313721627 ) ) ;
#39561=LINE ( 'NONE', #54379, #34503 ) ;
#39564=CARTESIAN_POINT ( 'NONE',  ( -2.500000000000000444, -40.04166666393548013, -4.330127018922193649 ) ) ;
#39566=CARTESIAN_POINT ( 'NONE',  ( 2.229367062499998831, 11.35416666803225993, -3.861377020970580887 ) ) ;
#39567=CARTESIAN_POINT ( 'NONE',  ( -6.972266317189433020E-16, -35.25000000000000000, -5.000000000000000000 ) ) ;
#39568=LINE ( 'NONE', #11264, #55159 ) ;
#39570=CARTESIAN_POINT ( 'NONE',  ( -4.458734124999999437, -62.39583333196774362, -2.574251347313719407 ) ) ;
#39571=VERTEX_POINT ( 'NONE', #13597 ) ;
#39574=CARTESIAN_POINT ( 'NONE',  ( 5.000000000000000000, 3.583333333333333925, -2.886751345948129988 ) ) ;
#39577=CARTESIAN_POINT ( 'NONE',  ( 4.458734124999998549, -53.72916666530106511, -2.574251347313721627 ) ) ;
#39578=CARTESIAN_POINT ( 'NONE',  ( -4.999999999999999112, -89.79166666393547303, 2.886751345948131764 ) ) ;
#39579=CARTESIAN_POINT ( 'NONE',  ( 4.458734124999999437, -34.81249999863440792, -5.460374474430324690E-16 ) ) ;
#39580=( BOUNDED_CURVE ( )  B_SPLINE_CURVE ( 2, ( #4496, #8083, #43725, #63369, #38900, #37652, #32509, #52141, #62112 ),
 .UNSPECIFIED., .F., .F. ) 
 B_SPLINE_CURVE_WITH_KNOTS ( ( 3, 2, 2, 2, 3 ),
 ( 0.4267857142857142683, 0.4273809523809523614, 0.4285714285714285476, 0.4297619047619047894, 0.4303571428571428825 ),
 .UNSPECIFIED. ) 
 CURVE ( )  GEOMETRIC_REPRESENTATION_ITEM ( )  RATIONAL_B_SPLINE_CURVE ( ( 0.9330127018922194093, 0.9330127018922194093, 1.000000000000000000, 0.8660254037844387076, 1.000000000000000000, 0.8660254037844387076, 1.000000000000000000, 0.9330127018922194093, 0.9330127018922194093 ) ) 
 REPRESENTATION_ITEM ( '' )  );
#39581=CARTESIAN_POINT ( 'NONE',  ( -1.339745962155613812, 19.91965820146970501, -5.000000000000000000 ) ) ;
#39583=CARTESIAN_POINT ( 'NONE',  ( -1.339745962155613812, -108.0803417985302985, -5.000000000000000000 ) ) ;
#39585=CARTESIAN_POINT ( 'NONE',  ( -5.000000000000000000, -45.00000000000000000, 0.000000000000000000 ) ) ;
#39589=CARTESIAN_POINT ( 'NONE',  ( 4.458734124999999437, -99.81249999863440792, -5.460374474430324690E-16 ) ) ;
#39590=CARTESIAN_POINT ( 'NONE',  ( -2.229367062499996610, 2.604166668032259491, 3.861377020970582219 ) ) ;
#39594=CARTESIAN_POINT ( 'NONE',  ( -8.660254037844341113, 45.00000000000000000, 6.047423072554883697E-14 ) ) ;
#39598=CARTESIAN_POINT ( 'NONE',  ( -2.500000000000000444, -11.16666666666666430, -4.330127018922193649 ) ) ;
#39604=CARTESIAN_POINT ( 'NONE',  ( 4.458734124999998549, -23.97916666530107221, -2.574251347313721627 ) ) ;
#39616=CARTESIAN_POINT ( 'NONE',  ( -2.229367062500000163, -71.72916666530107932, -3.861377020970580443 ) ) ;
#39622=CARTESIAN_POINT ( 'NONE',  ( -4.458734124999999437, -5.645833331967740953, -2.574251347313719407 ) ) ;
#39623=ORIENTED_EDGE ( 'NONE', *, *, #57558, .F. ) ;
#39625=DIRECTION ( 'NONE',  ( -0.000000000000000000, 1.000000000000000000, -0.000000000000000000 ) ) ;
#39630=ORIENTED_EDGE ( 'NONE', *, *, #21654, .F. ) ;
#39631=CARTESIAN_POINT ( 'NONE',  ( 2.229367062499998831, -81.64583333196773651, -3.861377020970580887 ) ) ;
#39632=CARTESIAN_POINT ( 'NONE',  ( 2.229367062499998831, 3.354166668032259935, -3.861377020970580887 ) ) ;
#39633=CARTESIAN_POINT ( 'NONE',  ( 5.000000000000000888, -86.58333333333334281, 2.886751345948126879 ) ) ;
#39634=EDGE_CURVE ( 'NONE', #59356, #41437, #43341, .T. ) ;
#39636=CARTESIAN_POINT ( 'NONE',  ( 2.229367062500001939, -64.22916666530106511, 3.861377020970579999 ) ) ;
#39637=CARTESIAN_POINT ( 'NONE',  ( -2.499999999999996447, -27.70833333060214798, 4.330127018922195425 ) ) ;
#39639=CARTESIAN_POINT ( 'NONE',  ( -4.999999999999998224, -14.91666666666666785, 2.886751345948131764 ) ) ;
#39640=CARTESIAN_POINT ( 'NONE',  ( -6.972266317189433020E-16, -1.124999997268814278, -5.000000000000000000 ) ) ;
#39641=CARTESIAN_POINT ( 'NONE',  ( -5.000000000000000000, -64.95833333060213022, -2.886751345948128211 ) ) ;
#39642=CARTESIAN_POINT ( 'NONE',  ( -2.229367062500000163, -46.47916666530106511, -3.861377020970580443 ) ) ;
#39643=CARTESIAN_POINT ( 'NONE',  ( -4.458734124999997661, -34.47916666530107221, 2.574251347313722516 ) ) ;
#39645=( BOUNDED_CURVE ( )  B_SPLINE_CURVE ( 2, ( #11499, #42270, #61910, #61593, #38084, #32622, #18141, #17527, #52565 ),
 .UNSPECIFIED., .F., .F. ) 
 B_SPLINE_CURVE_WITH_KNOTS ( ( 3, 2, 2, 2, 3 ),
 ( 0.06607142857142857262, 0.06666666666666666574, 0.06785714285714285199, 0.06904761904761905211, 0.06964285714285714524 ),
 .UNSPECIFIED. ) 
 CURVE ( )  GEOMETRIC_REPRESENTATION_ITEM ( )  RATIONAL_B_SPLINE_CURVE ( ( 0.9330127018922194093, 0.9330127018922194093, 1.000000000000000000, 0.8660254037844387076, 1.000000000000000000, 0.8660254037844387076, 1.000000000000000000, 0.9330127018922194093, 0.9330127018922194093 ) ) 
 REPRESENTATION_ITEM ( '' )  );
#39647=CARTESIAN_POINT ( 'NONE',  ( -4.999999999999999112, 22.08333333333333215, 2.886751345948131764 ) ) ;
#39650=CARTESIAN_POINT ( 'NONE',  ( 2.229367062499998831, -35.64583333196772941, -3.861377020970580887 ) ) ;
#39651=CARTESIAN_POINT ( 'NONE',  ( -2.500000000000000444, -76.04166666393547303, -4.330127018922193649 ) ) ;
#39652=EDGE_CURVE ( 'NONE', #53365, #62346, #39201, .T. ) ;
#39656=CARTESIAN_POINT ( 'NONE',  ( -2.229367062500000163, -77.72916666530106511, -3.861377020970580443 ) ) ;
#39658=CARTESIAN_POINT ( 'NONE',  ( 5.000000000000000888, 18.54166666939785202, 2.886751345948126879 ) ) ;
#39659=DIRECTION ( 'NONE',  ( -0.000000000000000000, 1.000000000000000000, -0.000000000000000000 ) ) ;
#39660=CARTESIAN_POINT ( 'NONE',  ( -3.535250795749689387E-16, -26.25000000000000355, -5.773502691896257311 ) ) ;
#39664=ORIENTED_EDGE ( 'NONE', *, *, #58125, .T. ) ;
#39666=CARTESIAN_POINT ( 'NONE',  ( 2.500000000000002220, 22.45833333606451987, 4.330127018922192761 ) ) ;
#39672=EDGE_CURVE ( 'NONE', #36130, #29318, #26077, .T. ) ;
#39674=CARTESIAN_POINT ( 'NONE',  ( -1.339745962155613812, -0.2053418012614791066, -5.000000000000000000 ) ) ;
#39675=FACE_OUTER_BOUND ( 'NONE', #22411, .T. ) ;
#39676=( BOUNDED_CURVE ( )  B_SPLINE_CURVE ( 2, ( #31972, #51608, #17812, #52231, #13303, #22656, #57694, #13621, #52859 ),
 .UNSPECIFIED., .F., .F. ) 
 B_SPLINE_CURVE_WITH_KNOTS ( ( 3, 2, 2, 2, 3 ),
 ( 0.1910714285714285865, 0.1916666666666666796, 0.1928571428571428659, 0.1940476190476190521, 0.1946428571428571452 ),
 .UNSPECIFIED. ) 
 CURVE ( )  GEOMETRIC_REPRESENTATION_ITEM ( )  RATIONAL_B_SPLINE_CURVE ( ( 0.9330127018922194093, 0.9330127018922209636, 1.000000000000000000, 0.8660254037844387076, 1.000000000000000000, 0.8660254037844387076, 1.000000000000000000, 0.9330127018922194093, 0.9330127018922194093 ) ) 
 REPRESENTATION_ITEM ( '' )  );
#39678=CARTESIAN_POINT ( 'NONE',  ( -3.152548672688508926E-16, -21.56249999863440081, -5.148502694627439702 ) ) ;
#39687=CARTESIAN_POINT ( 'NONE',  ( 1.975475456537005874E-15, -28.74999999999999645, 5.000000000000000000 ) ) ;
#39689=ORIENTED_EDGE ( 'NONE', *, *, #42145, .T. ) ;
#39691=CARTESIAN_POINT ( 'NONE',  ( 1.975475456537005874E-15, -23.62499999726880873, 5.000000000000000000 ) ) ;
#39693=CARTESIAN_POINT ( 'NONE',  ( 1.975475456537005874E-15, -86.75000000000001421, 5.000000000000000000 ) ) ;
#39695=EDGE_CURVE ( 'NONE', #27676, #51084, #38039, .T. ) ;
#39696=ORIENTED_EDGE ( 'NONE', *, *, #53011, .F. ) ;
#39698=EDGE_CURVE ( 'NONE', #6727, #52469, #36790, .T. ) ;
#39699=CARTESIAN_POINT ( 'NONE',  ( 2.229367062499998831, 14.35416666803226171, -3.861377020970580887 ) ) ;
#39704=CARTESIAN_POINT ( 'NONE',  ( 5.000000000000000000, -39.49999999999999289, -6.123233995736766282E-16 ) ) ;
#39705=CARTESIAN_POINT ( 'NONE',  ( 6.123233995736766282E-16, -120.0000000000000000, -5.000000000000000000 ) ) ;
#39706=CARTESIAN_POINT ( 'NONE',  ( -4.458734124999999437, -64.31249999863440792, 0.000000000000000000 ) ) ;
#39708=CARTESIAN_POINT ( 'NONE',  ( 2.229367062499998831, 20.35416666803225993, -3.861377020970580887 ) ) ;
#39710=CARTESIAN_POINT ( 'NONE',  ( 1.975475456537005874E-15, -83.62499999726878741, 5.000000000000000000 ) ) ;
#39711=CARTESIAN_POINT ( 'NONE',  ( -3.152548672688508926E-16, -48.81249999863440792, -5.148502694627439702 ) ) ;
#39712=CARTESIAN_POINT ( 'NONE',  ( 5.000000000000000888, -7.458333330602143540, 2.886751345948126879 ) ) ;
#39713=CARTESIAN_POINT ( 'NONE',  ( -6.972266317189433020E-16, -109.2499999999999716, -5.000000000000000000 ) ) ;
#39716=CARTESIAN_POINT ( 'NONE',  ( 1.975475456537005874E-15, -73.75000000000000000, 5.000000000000000000 ) ) ;
#39718=CARTESIAN_POINT ( 'NONE',  ( -2.229367062499996610, -16.39583333196773651, 3.861377020970582219 ) ) ;
#39719=ORIENTED_EDGE ( 'NONE', *, *, #40185, .F. ) ;
#39721=CARTESIAN_POINT ( 'NONE',  ( -4.458734124999999437, -101.3124999986344079, 0.000000000000000000 ) ) ;
#39723=CARTESIAN_POINT ( 'NONE',  ( -4.458734124999998549, -96.47916666530105090, 2.574251347313722516 ) ) ;
#39724=CARTESIAN_POINT ( 'NONE',  ( -1.339745962155555858, -8.205341801261482715, -5.000000000000032863 ) ) ;
#39725=CARTESIAN_POINT ( 'NONE',  ( 2.499999999999998668, -58.20833333060214443, -4.330127018922193649 ) ) ;
#39726=CYLINDRICAL_SURFACE ( 'NONE', #9908, 5.000000000000000000 ) ;
#39729=CARTESIAN_POINT ( 'NONE',  ( 4.458734125000000326, -17.89583333196773651, 2.574251347313718519 ) ) ;
#39730=CARTESIAN_POINT ( 'NONE',  ( -4.458734124999998549, 4.520833334698926009, 2.574251347313722516 ) ) ;
#39731=CARTESIAN_POINT ( 'NONE',  ( -4.458734124999999437, -64.56249999863440792, 0.000000000000000000 ) ) ;
#39735=CARTESIAN_POINT ( 'NONE',  ( -5.000000000000000000, -7.083333333333330373, -2.886751345948128211 ) ) ;
#39741=CARTESIAN_POINT ( 'NONE',  ( 2.229367062500001939, -90.97916666530106511, 3.861377020970579999 ) ) ;
#39742=CARTESIAN_POINT ( 'NONE',  ( 9.457646018065525792E-16, 17.68750000136559564, 5.148502694627439702 ) ) ;
#39744=CARTESIAN_POINT ( 'NONE',  ( 2.500000000000002220, -82.66666666666667140, 4.330127018922192761 ) ) ;
#39746=CARTESIAN_POINT ( 'NONE',  ( 1.975475456537005874E-15, -67.62499999726881583, 5.000000000000000000 ) ) ;
#39748=CARTESIAN_POINT ( 'NONE',  ( -2.500000000000000444, -75.16666666666665719, -4.330127018922193649 ) ) ;
#39750=VERTEX_POINT ( 'NONE', #44746 ) ;
#39754=( BOUNDED_CURVE ( )  B_SPLINE_CURVE ( 2, ( #42984, #62628, #18550, #15624, #44885, #44558, #34582, #50026, #35241 ),
 .UNSPECIFIED., .F., .F. ) 
 B_SPLINE_CURVE_WITH_KNOTS ( ( 3, 2, 2, 2, 3 ),
 ( 0.06964285714285714524, 0.07023809523809523836, 0.07142857142857142461, 0.07261904761904762473, 0.07321428571428571785 ),
 .UNSPECIFIED. ) 
 CURVE ( )  GEOMETRIC_REPRESENTATION_ITEM ( )  RATIONAL_B_SPLINE_CURVE ( ( 0.9330127018922194093, 0.9330127018922194093, 1.000000000000000000, 0.8660254037844387076, 1.000000000000000000, 0.8660254037844387076, 1.000000000000000000, 0.9330127018922194093, 0.9330127018922194093 ) ) 
 REPRESENTATION_ITEM ( '' )  );
#39756=ORIENTED_EDGE ( 'NONE', *, *, #29529, .F. ) ;
#39763=CARTESIAN_POINT ( 'NONE',  ( -3.152548672688508926E-16, -64.81249999863440792, -5.148502694627439702 ) ) ;
#39771=( BOUNDED_CURVE ( )  B_SPLINE_CURVE ( 2, ( #8281, #7021, #7656, #62315, #22448, #27569, #7342, #18240, #26629 ),
 .UNSPECIFIED., .F., .F. ) 
 B_SPLINE_CURVE_WITH_KNOTS ( ( 3, 2, 2, 2, 3 ),
 ( 0.8160714285714285587, 0.8166666666666666519, 0.8178571428571428381, 0.8190476190476190244, 0.8196428571428571175 ),
 .UNSPECIFIED. ) 
 CURVE ( )  GEOMETRIC_REPRESENTATION_ITEM ( )  RATIONAL_B_SPLINE_CURVE ( ( 0.9330127018922194093, 0.9330127018922194093, 1.000000000000000000, 0.8660254037844387076, 1.000000000000000000, 0.8660254037844387076, 1.000000000000000000, 0.9330127018922194093, 0.9330127018922194093 ) ) 
 REPRESENTATION_ITEM ( '' )  );
#39772=ADVANCED_FACE ( 'NONE', ( #49578 ), #71, .T. ) ;
#39775=CARTESIAN_POINT ( 'NONE',  ( 4.458734125000001214, -110.1458333319677507, 2.574251347313718519 ) ) ;
#39777=ORIENTED_EDGE ( 'NONE', *, *, #47515, .T. ) ;
#39781=CARTESIAN_POINT ( 'NONE',  ( -3.152548672688508926E-16, -46.56249999863440792, -5.148502694627439702 ) ) ;
#39783=EDGE_CURVE ( 'NONE', #11315, #28751, #63438, .T. ) ;
#39785=CARTESIAN_POINT ( 'NONE',  ( -4.458734124999999437, -47.31249999863440792, 0.000000000000000000 ) ) ;
#39789=CARTESIAN_POINT ( 'NONE',  ( 4.458734124999999437, -12.81249999863440259, -5.460374474430324690E-16 ) ) ;
#39790=CARTESIAN_POINT ( 'NONE',  ( -5.000000000000000000, -100.0833333333333286, -2.886751345948128211 ) ) ;
#39792=CARTESIAN_POINT ( 'NONE',  ( 9.457646018065525792E-16, -31.31249999863440436, 5.148502694627439702 ) ) ;
#39793=CARTESIAN_POINT ( 'NONE',  ( -5.000000000000000000, 7.041666669397851130, -2.886751345948128211 ) ) ;
#39794=FACE_OUTER_BOUND ( 'NONE', #53692, .T. ) ;
#39799=DIRECTION ( 'NONE',  ( 0.000000000000000000, 0.000000000000000000, 1.000000000000000000 ) ) ;
#39801=CARTESIAN_POINT ( 'NONE',  ( 4.458734124999999437, -0.06249999863440491854, -5.460374474430324690E-16 ) ) ;
#39803=CARTESIAN_POINT ( 'NONE',  ( 2.500000000000002220, 16.45833333606451987, 4.330127018922192761 ) ) ;
#39806=CARTESIAN_POINT ( 'NONE',  ( -5.000000000000000000, -96.08333333333331439, -2.886751345948128211 ) ) ;
#39807=CARTESIAN_POINT ( 'NONE',  ( 4.458734125000001214, -34.89583333196772941, 2.574251347313718519 ) ) ;
#39808=CARTESIAN_POINT ( 'NONE',  ( 1.975475456537005874E-15, 9.250000000000000000, 5.000000000000000000 ) ) ;
#39809=CARTESIAN_POINT ( 'NONE',  ( 4.458734125000001214, -80.14583333196773651, 2.574251347313718519 ) ) ;
#39811=CARTESIAN_POINT ( 'NONE',  ( -6.972266317189433020E-16, -53.24999999999999289, -5.000000000000000000 ) ) ;
#39813=ADVANCED_FACE ( 'NONE', ( #15498 ), #53144, .T. ) ;
#39814=CARTESIAN_POINT ( 'NONE',  ( -4.458734124999997661, -4.229166665301070438, 2.574251347313722516 ) ) ;
#39815=CARTESIAN_POINT ( 'NONE',  ( -3.152548672688508926E-16, 23.18750000136559208, -5.148502694627439702 ) ) ;
#39816=CARTESIAN_POINT ( 'NONE',  ( 2.229367062499998831, -42.89583333196773651, -3.861377020970580887 ) ) ;
#39817=DIRECTION ( 'NONE',  ( -0.000000000000000000, 1.000000000000000000, -0.000000000000000000 ) ) ;
#39821=CARTESIAN_POINT ( 'NONE',  ( 9.457646018065525792E-16, -75.06249999863439371, 5.148502694627439702 ) ) ;
#39822=CARTESIAN_POINT ( 'NONE',  ( 1.060575238724906964E-15, -107.6249999972687874, 5.773502691896257311 ) ) ;
#39827=CARTESIAN_POINT ( 'NONE',  ( -3.535250795749689387E-16, -61.25000000000000000, -5.773502691896257311 ) ) ;
#39828=CARTESIAN_POINT ( 'NONE',  ( 0.000000000000000000, -120.0000000000000000, 0.000000000000000000 ) ) ;
#39840=ORIENTED_EDGE ( 'NONE', *, *, #62274, .T. ) ;
#39841=CARTESIAN_POINT ( 'NONE',  ( -5.000000000000000000, -24.00000000000000000, 0.000000000000000000 ) ) ;
#39842=CARTESIAN_POINT ( 'NONE',  ( -5.000000000000000000, 11.04166666939785202, -2.886751345948128211 ) ) ;
#39848=CARTESIAN_POINT ( 'NONE',  ( -4.458734124999998549, -48.47916666530106511, 2.574251347313722516 ) ) ;
#39849=CARTESIAN_POINT ( 'NONE',  ( 5.000000000000000888, -23.58333333333333215, 2.886751345948126879 ) ) ;
#39857=CARTESIAN_POINT ( 'NONE',  ( -4.458734124999999437, -86.56249999863439371, 0.000000000000000000 ) ) ;
#39860=CARTESIAN_POINT ( 'NONE',  ( -6.972266317189433020E-16, 13.87500000273118594, -5.000000000000000000 ) ) ;
#39861=DIRECTION ( 'NONE',  ( 0.000000000000000000, 0.000000000000000000, 1.000000000000000000 ) ) ;
#39865=CARTESIAN_POINT ( 'NONE',  ( 2.229367062499998831, 5.354166668032261711, -3.861377020970580887 ) ) ;
#39866=CARTESIAN_POINT ( 'NONE',  ( 1.339745962155612702, -50.16965819600732601, -5.000000000000000000 ) ) ;
#39867=CARTESIAN_POINT ( 'NONE',  ( 4.458734125000001214, -16.14583333196773651, 2.574251347313718519 ) ) ;
#39868=CARTESIAN_POINT ( 'NONE',  ( -5.000000000000000000, -100.8749999972688158, 0.000000000000000000 ) ) ;
#39870=CARTESIAN_POINT ( 'NONE',  ( 6.123233995736766282E-16, -120.0000000000000000, -5.000000000000000000 ) ) ;
#39873=( BOUNDED_CURVE ( )  B_SPLINE_CURVE ( 2, ( #42615, #29065, #48690, #13350, #9765, #24255, #43858, #53837, #63505 ),
 .UNSPECIFIED., .F., .F. ) 
 B_SPLINE_CURVE_WITH_KNOTS ( ( 3, 2, 2, 2, 3 ),
 ( 0.1482142857142857151, 0.1488095238095238082, 0.1499999999999999944, 0.1511904761904761807, 0.1517857142857143016 ),
 .UNSPECIFIED. ) 
 CURVE ( )  GEOMETRIC_REPRESENTATION_ITEM ( )  RATIONAL_B_SPLINE_CURVE ( ( 0.9330127018922194093, 0.9330127018922194093, 1.000000000000000000, 0.8660254037844387076, 1.000000000000000000, 0.8660254037844387076, 1.000000000000000000, 0.9330127018922178550, 0.9330127018922194093 ) ) 
 REPRESENTATION_ITEM ( '' )  );
#39874=CARTESIAN_POINT ( 'NONE',  ( 2.229367062499998831, 13.10416666803226171, -3.861377020970580887 ) ) ;
#39876=CARTESIAN_POINT ( 'NONE',  ( -4.458734124999999437, -96.31249999863440792, 0.000000000000000000 ) ) ;
#39877=CARTESIAN_POINT ( 'NONE',  ( -5.000000000000000000, -18.87499999726881583, 0.000000000000000000 ) ) ;
#39879=CARTESIAN_POINT ( 'NONE',  ( 9.457646018065525792E-16, -16.06249999863440436, 5.148502694627439702 ) ) ;
#39880=AXIS2_PLACEMENT_3D ( 'NONE', #28145, #37810, #17565 ) ;
#39882=DIRECTION ( 'NONE',  ( 0.000000000000000000, 0.000000000000000000, 1.000000000000000000 ) ) ;
#39884=CARTESIAN_POINT ( 'NONE',  ( 5.000000000000000000, -43.37499999726880873, -6.123233995736766282E-16 ) ) ;
#39886=CARTESIAN_POINT ( 'NONE',  ( -2.229367062499996610, 15.85416666803226171, 3.861377020970582219 ) ) ;
#39889=CARTESIAN_POINT ( 'NONE',  ( -4.458734124999998549, -61.22916666530106511, 2.574251347313722516 ) ) ;
#39892=CARTESIAN_POINT ( 'NONE',  ( -5.000000000000000000, 2.999999999999999112, 0.000000000000000000 ) ) ;
#39895=CARTESIAN_POINT ( 'NONE',  ( -4.458734124999998549, -51.22916666530107221, 2.574251347313722516 ) ) ;
#39896=CARTESIAN_POINT ( 'NONE',  ( -2.499999999999996447, -88.70833333060214443, 4.330127018922195425 ) ) ;
#39897=CARTESIAN_POINT ( 'NONE',  ( -3.152548672688508926E-16, -31.56249999863440436, -5.148502694627439702 ) ) ;
#39899=FACE_OUTER_BOUND ( 'NONE', #30722, .T. ) ;
#39904=CARTESIAN_POINT ( 'NONE',  ( -4.999999999999999112, -43.91666666666665719, 2.886751345948131764 ) ) ;
#39906=CARTESIAN_POINT ( 'NONE',  ( 5.000000000000000888, -6.458333330602150646, 2.886751345948126879 ) ) ;
#39908=CARTESIAN_POINT ( 'NONE',  ( -3.152548672688508926E-16, -101.5624999986344221, -5.148502694627439702 ) ) ;
#39909=CARTESIAN_POINT ( 'NONE',  ( -2.229367062499996610, 3.604166668032260379, 3.861377020970582219 ) ) ;
#39916=VERTEX_POINT ( 'NONE', #48308 ) ;
#39917=CARTESIAN_POINT ( 'NONE',  ( -1.339745962155610925, -81.79465819873850307, 5.000000000000000000 ) ) ;
#39919=ORIENTED_EDGE ( 'NONE', *, *, #39366, .T. ) ;
#39920=CARTESIAN_POINT ( 'NONE',  ( 1.339745962155612702, -101.2946581987385031, -5.000000000000000000 ) ) ;
#39923=CARTESIAN_POINT ( 'NONE',  ( -4.458734124999999437, -23.64583333196773651, -2.574251347313719407 ) ) ;
#39924=VECTOR ( 'NONE', #13036, 1000.000000000000000 ) ;
#39933=ORIENTED_EDGE ( 'NONE', *, *, #4706, .T. ) ;
#39934=CARTESIAN_POINT ( 'NONE',  ( -6.972266317189433020E-16, -83.12499999726878741, -5.000000000000000000 ) ) ;
#39935=ORIENTED_EDGE ( 'NONE', *, *, #21651, .F. ) ;
#39936=CARTESIAN_POINT ( 'NONE',  ( -2.229367062500000163, -70.72916666530107932, -3.861377020970580443 ) ) ;
#39938=ORIENTED_EDGE ( 'NONE', *, *, #18881, .F. ) ;
#39940=CARTESIAN_POINT ( 'NONE',  ( 1.975475456537005874E-15, -65.62499999726881583, 5.000000000000000000 ) ) ;
#39942=CARTESIAN_POINT ( 'NONE',  ( 2.229367062500001939, -5.229166665301071326, 3.861377020970579999 ) ) ;
#39943=ORIENTED_EDGE ( 'NONE', *, *, #51470, .T. ) ;
#39944=CARTESIAN_POINT ( 'NONE',  ( -1.339745962155610925, -44.79465819873851018, 5.000000000000000000 ) ) ;
#39951=CARTESIAN_POINT ( 'NONE',  ( -4.458734124999999437, -79.31249999863440792, 0.000000000000000000 ) ) ;
#39953=CARTESIAN_POINT ( 'NONE',  ( 4.458734125000001214, 1.104166668032261711, 2.574251347313718519 ) ) ;
#39956=CARTESIAN_POINT ( 'NONE',  ( 1.060575238724906964E-15, -87.75000000000000000, 5.773502691896257311 ) ) ;
#39958=CARTESIAN_POINT ( 'NONE',  ( -4.458734124999999437, -67.56249999863440792, 0.000000000000000000 ) ) ;
#39959=CARTESIAN_POINT ( 'NONE',  ( -5.000000000000000000, -23.95833333060214443, -2.886751345948128211 ) ) ;
#39960=CARTESIAN_POINT ( 'NONE',  ( -5.000000000000000000, -15.08333333333333215, -2.886751345948128211 ) ) ;
#39961=CARTESIAN_POINT ( 'NONE',  ( -3.152548672688508926E-16, 28.43750000136559564, -5.148502694627439702 ) ) ;
#39962=CARTESIAN_POINT ( 'NONE',  ( 2.499999999999998668, -110.2083333306021444, -4.330127018922193649 ) ) ;
#39963=CARTESIAN_POINT ( 'NONE',  ( 1.339745962155641346, -3.169658196007335782, -4.999999999999983125 ) ) ;
#39964=CARTESIAN_POINT ( 'NONE',  ( 4.458734125000001214, -45.89583333196774362, 2.574251347313718519 ) ) ;
#39966=CARTESIAN_POINT ( 'NONE',  ( -4.458734124999999437, -31.64583333196773651, -2.574251347313719407 ) ) ;
#39968=VECTOR ( 'NONE', #42559, 1000.000000000000114 ) ;
#39970=CARTESIAN_POINT ( 'NONE',  ( -3.535250795749689387E-16, 19.74999999999999645, -5.773502691896257311 ) ) ;
#39972=CARTESIAN_POINT ( 'NONE',  ( 5.000000000000000888, -54.45833333060214443, 2.886751345948126879 ) ) ;
#39973=VECTOR ( 'NONE', #39659, 1000.000000000000000 ) ;
#39974=CARTESIAN_POINT ( 'NONE',  ( -2.229367062500000163, -38.47916666530107221, -3.861377020970580443 ) ) ;
#39975=CARTESIAN_POINT ( 'NONE',  ( -5.000000000000000000, -73.87499999726880162, 0.000000000000000000 ) ) ;
#39978=CARTESIAN_POINT ( 'NONE',  ( -2.229367062499996610, -78.39583333196773651, 3.861377020970582219 ) ) ;
#39980=CARTESIAN_POINT ( 'NONE',  ( 5.000000000000000000, 18.70833333606451632, -2.886751345948130876 ) ) ;
#39982=CARTESIAN_POINT ( 'NONE',  ( -3.535250795749689387E-16, -29.25000000000000000, -5.773502691896257311 ) ) ;
#39984=ORIENTED_EDGE ( 'NONE', *, *, #56157, .T. ) ;
#39986=VERTEX_POINT ( 'NONE', #53764 ) ;
#39988=CARTESIAN_POINT ( 'NONE',  ( 1.060575238724906964E-15, 22.37500000273118772, 5.773502691896257311 ) ) ;
#39996=CARTESIAN_POINT ( 'NONE',  ( -1.339745962155610925, -61.79465819873851729, 5.000000000000000000 ) ) ;
#39999=CARTESIAN_POINT ( 'NONE',  ( 4.458734125000001214, -23.89583333196774007, 2.574251347313718519 ) ) ;
#40000=CARTESIAN_POINT ( 'NONE',  ( 1.975475456537005874E-15, -32.74999999999999289, 5.000000000000000000 ) ) ;
#40003=ADVANCED_FACE ( 'NONE', ( #4883 ), #24505, .T. ) ;
#40005=ORIENTED_EDGE ( 'NONE', *, *, #16664, .T. ) ;
#40006=CARTESIAN_POINT ( 'NONE',  ( 2.500000000000002220, 13.33333333333333215, 4.330127018922192761 ) ) ;
#40009=ORIENTED_EDGE ( 'NONE', *, *, #39634, .F. ) ;
#40010=CARTESIAN_POINT ( 'NONE',  ( -5.000000000000000000, -28.08333333333333925, -2.886751345948128211 ) ) ;
#40011=CARTESIAN_POINT ( 'NONE',  ( 5.000000000000000000, -9.374999997268814056, -6.123233995736766282E-16 ) ) ;
#40022=CARTESIAN_POINT ( 'NONE',  ( -3.152548672688508926E-16, 15.43750000136559564, -5.148502694627439702 ) ) ;
#40025=CARTESIAN_POINT ( 'NONE',  ( 1.339745962155612702, 12.83034180399266511, -5.000000000000000000 ) ) ;
#40027=( BOUNDED_CURVE ( )  B_SPLINE_CURVE ( 2, ( #29848, #16021, #49480, #25992, #40139, #54946, #25681, #6387, #11193 ),
 .UNSPECIFIED., .F., .F. ) 
 B_SPLINE_CURVE_WITH_KNOTS ( ( 3, 2, 2, 2, 3 ),
 ( 0.9660714285714285809, 0.9666666666666666741, 0.9678571428571428603, 0.9690476190476190466, 0.9696428571428571397 ),
 .UNSPECIFIED. ) 
 CURVE ( )  GEOMETRIC_REPRESENTATION_ITEM ( )  RATIONAL_B_SPLINE_CURVE ( ( 0.9330127018922194093, 0.9330127018922194093, 1.000000000000000000, 0.8660254037844387076, 1.000000000000000000, 0.8660254037844387076, 1.000000000000000000, 0.9330127018922194093, 0.9330127018922194093 ) ) 
 REPRESENTATION_ITEM ( '' )  );
#40028=DIRECTION ( 'NONE',  ( -0.000000000000000000, 1.000000000000000000, -0.000000000000000000 ) ) ;
#40029=CARTESIAN_POINT ( 'NONE',  ( 4.458734124999999437, -67.81249999863440792, -5.460374474430324690E-16 ) ) ;
#40031=CARTESIAN_POINT ( 'NONE',  ( -3.152548672688508926E-16, 17.43750000136559564, -5.148502694627439702 ) ) ;
#40033=CARTESIAN_POINT ( 'NONE',  ( 2.229367062499998831, -46.89583333196774362, -3.861377020970580887 ) ) ;
#40035=CARTESIAN_POINT ( 'NONE',  ( -4.999999999999999112, -10.79166666393547658, 2.886751345948131764 ) ) ;
#40040=CARTESIAN_POINT ( 'NONE',  ( -4.458734124999999437, -16.56249999863440436, 0.000000000000000000 ) ) ;
#40042=DIRECTION ( 'NONE',  ( -0.000000000000000000, 1.000000000000000000, -0.000000000000000000 ) ) ;
#40043=CARTESIAN_POINT ( 'NONE',  ( 2.229367062500001939, -101.9791666653010651, 3.861377020970579999 ) ) ;
#40045=ORIENTED_EDGE ( 'NONE', *, *, #18522, .T. ) ;
#40046=CARTESIAN_POINT ( 'NONE',  ( -2.229367062500000163, -96.72916666530105090, -3.861377020970580443 ) ) ;
#40048=CARTESIAN_POINT ( 'NONE',  ( 5.000000000000000000, -59.37499999726880873, -6.123233995736766282E-16 ) ) ;
#40049=CARTESIAN_POINT ( 'NONE',  ( 1.339745962155615144, -62.58034179853028434, 4.999999999999999112 ) ) ;
#40052=CARTESIAN_POINT ( 'NONE',  ( 4.458734125000000326, -16.89583333196773651, 2.574251347313718519 ) ) ;
#40053=CARTESIAN_POINT ( 'NONE',  ( -2.229367062500000163, 6.270833334698928674, -3.861377020970580443 ) ) ;
#40054=CARTESIAN_POINT ( 'NONE',  ( 4.458734124999998549, -65.97916666530106511, -2.574251347313721627 ) ) ;
#40057=CARTESIAN_POINT ( 'NONE',  ( 6.123233995736766282E-16, -120.0000000000000000, -5.000000000000000000 ) ) ;
#40059=CARTESIAN_POINT ( 'NONE',  ( -3.535250795749689387E-16, -13.24999999999999822, -5.773502691896257311 ) ) ;
#40061=ORIENTED_EDGE ( 'NONE', *, *, #41769, .T. ) ;
#40065=CARTESIAN_POINT ( 'NONE',  ( 1.975475456537005874E-15, -38.62499999726880873, 5.000000000000000000 ) ) ;
#40068=EDGE_CURVE ( 'NONE', #25319, #40086, #17446, .T. ) ;
#40070=FACE_OUTER_BOUND ( 'NONE', #62823, .T. ) ;
#40074=CARTESIAN_POINT ( 'NONE',  ( 1.060575238724906964E-15, -75.75000000000000000, 5.773502691896257311 ) ) ;
#40076=ORIENTED_EDGE ( 'NONE', *, *, #20596, .F. ) ;
#40079=CARTESIAN_POINT ( 'NONE',  ( -2.499999999999996447, -53.70833333060213732, 4.330127018922195425 ) ) ;
#40082=ORIENTED_EDGE ( 'NONE', *, *, #91, .F. ) ;
#40084=EDGE_CURVE ( 'NONE', #10009, #22588, #41278, .T. ) ;
#40086=VERTEX_POINT ( 'NONE', #1670 ) ;
#40089=EDGE_CURVE ( 'NONE', #57423, #62194, #8054, .T. ) ;
#40090=CARTESIAN_POINT ( 'NONE',  ( -4.458734124999999437, -61.64583333196773651, -2.574251347313719407 ) ) ;
#40092=CYLINDRICAL_SURFACE ( 'NONE', #2594, 5.000000000000000000 ) ;
#40096=FACE_OUTER_BOUND ( 'NONE', #27420, .T. ) ;
#40100=CARTESIAN_POINT ( 'NONE',  ( 4.458734125000001214, 29.10416666803225993, 2.574251347313718519 ) ) ;
#40102=ORIENTED_EDGE ( 'NONE', *, *, #12586, .F. ) ;
#40107=CARTESIAN_POINT ( 'NONE',  ( -2.229367062500000163, -44.47916666530106511, -3.861377020970580443 ) ) ;
#40110=CARTESIAN_POINT ( 'NONE',  ( -4.458734124999999437, -50.39583333196772941, -2.574251347313719407 ) ) ;
#40111=VECTOR ( 'NONE', #47817, 1000.000000000000000 ) ;
#40113=EDGE_CURVE ( 'NONE', #1919, #19582, #63462, .T. ) ;
#40114=CARTESIAN_POINT ( 'NONE',  ( 4.458734124999998549, -15.72916666530107399, -2.574251347313721627 ) ) ;
#40115=CARTESIAN_POINT ( 'NONE',  ( -4.999999999999999112, -102.9166666666666714, 2.886751345948131764 ) ) ;
#40117=CARTESIAN_POINT ( 'NONE',  ( 4.458734124999998549, -32.97916666530106511, -2.574251347313721627 ) ) ;
#40118=CARTESIAN_POINT ( 'NONE',  ( 2.500000000000002220, 4.458333336064518093, 4.330127018922192761 ) ) ;
#40124=DIRECTION ( 'NONE',  ( 0.000000000000000000, 0.000000000000000000, 1.000000000000000000 ) ) ;
#40125=CARTESIAN_POINT ( 'NONE',  ( 4.458734124999999437, -1.062499998634405696, -5.460374474430324690E-16 ) ) ;
#40126=ORIENTED_EDGE ( 'NONE', *, *, #56171, .F. ) ;
#40129=CARTESIAN_POINT ( 'NONE',  ( -4.458734124999999437, -85.39583333196773651, -2.574251347313719407 ) ) ;
#40130=CARTESIAN_POINT ( 'NONE',  ( 4.458734124999999437, -35.81249999863440792, -5.460374474430324690E-16 ) ) ;
#40131=CARTESIAN_POINT ( 'NONE',  ( 1.339745962155612702, -9.294658198738520838, -5.000000000000000000 ) ) ;
#40132=CARTESIAN_POINT ( 'NONE',  ( -3.152548672688508926E-16, -83.81249999863439371, -5.148502694627439702 ) ) ;
#40136=CARTESIAN_POINT ( 'NONE',  ( -3.152548672688508926E-16, -0.5624999986344053626, -5.148502694627439702 ) ) ;
#40137=CARTESIAN_POINT ( 'NONE',  ( 4.458734125000001214, 22.85416666803225993, 2.574251347313718519 ) ) ;
#40138=CARTESIAN_POINT ( 'NONE',  ( 2.229367062500001939, -46.22916666530106511, 3.861377020970579999 ) ) ;
#40139=CARTESIAN_POINT ( 'NONE',  ( 5.000000000000000000, -105.5000000000000142, -6.123233995736766282E-16 ) ) ;
#40145=CARTESIAN_POINT ( 'NONE',  ( 4.458734124999998549, -73.72916666530106511, -2.574251347313721627 ) ) ;
#40146=CARTESIAN_POINT ( 'NONE',  ( 5.000000000000000000, -108.3749999972688016, -6.123233995736766282E-16 ) ) ;
#40147=( BOUNDED_CURVE ( )  B_SPLINE_CURVE ( 2, ( #59179, #14781, #59504, #5463, #10918, #15113, #10596, #10287, #39541 ),
 .UNSPECIFIED., .F., .F. ) 
 B_SPLINE_CURVE_WITH_KNOTS ( ( 3, 2, 2, 2, 3 ),
 ( 0.4410714285714285587, 0.4416666666666666519, 0.4428571428571428381, 0.4440476190476190244, 0.4446428571428571175 ),
 .UNSPECIFIED. ) 
 CURVE ( )  GEOMETRIC_REPRESENTATION_ITEM ( )  RATIONAL_B_SPLINE_CURVE ( ( 0.9330127018922194093, 0.9330127018922194093, 1.000000000000000000, 0.8660254037844387076, 1.000000000000000000, 0.8660254037844387076, 1.000000000000000000, 0.9330127018922194093, 0.9330127018922194093 ) ) 
 REPRESENTATION_ITEM ( '' )  );
#40149=EDGE_CURVE ( 'NONE', #14229, #30563, #46030, .T. ) ;
#40151=FACE_OUTER_BOUND ( 'NONE', #52258, .T. ) ;
#40154=CARTESIAN_POINT ( 'NONE',  ( 5.000000000000000888, -58.58333333333333570, 2.886751345948126879 ) ) ;
#40155=EDGE_CURVE ( 'NONE', #13355, #11557, #4282, .T. ) ;
#40160=EDGE_CURVE ( 'NONE', #2538, #14167, #31870, .T. ) ;
#40161=CARTESIAN_POINT ( 'NONE',  ( -2.500000000000000444, -99.16666666666665719, -4.330127018922193649 ) ) ;
#40170=VECTOR ( 'NONE', #44073, 1000.000000000000000 ) ;
#40174=CARTESIAN_POINT ( 'NONE',  ( -2.499999999999996447, 11.29166666939785202, 4.330127018922195425 ) ) ;
#40182=CARTESIAN_POINT ( 'NONE',  ( 2.229367062499998831, -46.89583333196774362, -3.861377020970580887 ) ) ;
#40185=EDGE_CURVE ( 'NONE', #24668, #36016, #45801, .T. ) ;
#40186=ADVANCED_FACE ( 'NONE', ( #43093 ), #41831, .T. ) ;
#40190=CARTESIAN_POINT ( 'NONE',  ( 5.000000000000000888, -89.58333333333332860, 2.886751345948126879 ) ) ;
#40192=CARTESIAN_POINT ( 'NONE',  ( -2.229367062500000163, -92.72916666530106511, -3.861377020970580443 ) ) ;
#40199=ORIENTED_EDGE ( 'NONE', *, *, #59045, .F. ) ;
#40200=CARTESIAN_POINT ( 'NONE',  ( 2.229367062499998831, -0.6458333319677399542, -3.861377020970580887 ) ) ;
#40201=CARTESIAN_POINT ( 'NONE',  ( 1.339745962155612702, 6.705341801261480050, -5.000000000000000000 ) ) ;
#40202=CARTESIAN_POINT ( 'NONE',  ( 4.458734124999998549, -17.97916666530106866, -2.574251347313721627 ) ) ;
#40203=CARTESIAN_POINT ( 'NONE',  ( -1.339745962155613812, -101.2053418012614827, -5.000000000000000000 ) ) ;
#40205=LINE ( 'NONE', #39870, #5929 ) ;
#40207=CARTESIAN_POINT ( 'NONE',  ( -2.229367062499996610, 17.60416666803225993, 3.861377020970582219 ) ) ;
#40210=CARTESIAN_POINT ( 'NONE',  ( 6.123233995736766282E-16, -120.0000000000000000, -5.000000000000000000 ) ) ;
#40211=CARTESIAN_POINT ( 'NONE',  ( 9.457646018065525792E-16, -20.06249999863440081, 5.148502694627439702 ) ) ;
#40216=CARTESIAN_POINT ( 'NONE',  ( 1.060575238724906964E-15, -48.62499999726881583, 5.773502691896257311 ) ) ;
#40218=CARTESIAN_POINT ( 'NONE',  ( -2.229367062499996610, 14.85416666803226171, 3.861377020970582219 ) ) ;
#40221=DIRECTION ( 'NONE',  ( -0.000000000000000000, 1.000000000000000000, -0.000000000000000000 ) ) ;
#40223=CARTESIAN_POINT ( 'NONE',  ( 4.458734124999999437, -64.81249999863440792, -5.460374474430324690E-16 ) ) ;
#40227=CARTESIAN_POINT ( 'NONE',  ( -4.999999999999999112, 6.083333333333333037, 2.886751345948131764 ) ) ;
#40230=CARTESIAN_POINT ( 'NONE',  ( -4.458734124999998549, -56.22916666530107221, 2.574251347313722516 ) ) ;
#40231=CARTESIAN_POINT ( 'NONE',  ( 2.499999999999998668, -91.20833333060214443, -4.330127018922193649 ) ) ;
#40232=CARTESIAN_POINT ( 'NONE',  ( 4.458734124999998549, -34.72916666530107221, -2.574251347313721627 ) ) ;
#40233=FACE_OUTER_BOUND ( 'NONE', #172, .T. ) ;
#40234=CARTESIAN_POINT ( 'NONE',  ( 0.000000000000000000, -120.0000000000000000, 0.000000000000000000 ) ) ;
#40238=CARTESIAN_POINT ( 'NONE',  ( 5.000000000000000000, -42.41666666666667140, -2.886751345948129988 ) ) ;
#40241=EDGE_LOOP ( 'NONE', ( #22295, #1377, #56431, #24589 ) ) ;
#40242=CARTESIAN_POINT ( 'NONE',  ( -4.458734124999999437, -107.3124999986343937, 0.000000000000000000 ) ) ;
#40243=CARTESIAN_POINT ( 'NONE',  ( -2.229367062499996610, 4.604166668032261711, 3.861377020970582219 ) ) ;
#40244=CARTESIAN_POINT ( 'NONE',  ( -1.339745962155610925, -96.66965819600731891, 5.000000000000000000 ) ) ;
#40250=VERTEX_POINT ( 'NONE', #12881 ) ;
#40252=CARTESIAN_POINT ( 'NONE',  ( 1.339745962155615144, -6.705341801261480050, 4.999999999999999112 ) ) ;
#40254=CARTESIAN_POINT ( 'NONE',  ( -6.972266317189433020E-16, -101.2499999999999858, -5.000000000000000000 ) ) ;
#40257=CARTESIAN_POINT ( 'NONE',  ( -3.152548672688508926E-16, -31.81249999863440792, -5.148502694627439702 ) ) ;
#40266=LINE ( 'NONE', #6183, #23830 ) ;
#40268=CARTESIAN_POINT ( 'NONE',  ( 2.229367062500001939, -79.22916666530106511, 3.861377020970579999 ) ) ;
#40271=VECTOR ( 'NONE', #35134, 1000.000000000000000 ) ;
#40273=( BOUNDED_CURVE ( )  B_SPLINE_CURVE ( 2, ( #24218, #43825, #14557, #5556, #29029, #53489, #24862, #48653, #113 ),
 .UNSPECIFIED., .F., .F. ) 
 B_SPLINE_CURVE_WITH_KNOTS ( ( 3, 2, 2, 2, 3 ),
 ( 0.2089285714285714357, 0.2095238095238095288, 0.2107142857142857151, 0.2119047619047619013, 0.2124999999999999944 ),
 .UNSPECIFIED. ) 
 CURVE ( )  GEOMETRIC_REPRESENTATION_ITEM ( )  RATIONAL_B_SPLINE_CURVE ( ( 0.9330127018922194093, 0.9330127018922194093, 1.000000000000000000, 0.8660254037844387076, 1.000000000000000000, 0.8660254037844387076, 1.000000000000000000, 0.9330127018922194093, 0.9330127018922194093 ) ) 
 REPRESENTATION_ITEM ( '' )  );
#40274=LINE ( 'NONE', #19695, #56869 ) ;
#40276=CARTESIAN_POINT ( 'NONE',  ( 9.457646018065525792E-16, -1.312499998634405918, 5.148502694627439702 ) ) ;
#40282=CYLINDRICAL_SURFACE ( 'NONE', #41862, 5.000000000000000000 ) ;
#40284=CARTESIAN_POINT ( 'NONE',  ( 1.975475456537005874E-15, -21.62499999726880873, 5.000000000000000000 ) ) ;
#40286=CARTESIAN_POINT ( 'NONE',  ( 4.458734124999999437, -80.81249999863440792, -5.460374474430324690E-16 ) ) ;
#40287=CARTESIAN_POINT ( 'NONE',  ( -6.972266317189433020E-16, -60.24999999999999289, -5.000000000000000000 ) ) ;
#40288=CARTESIAN_POINT ( 'NONE',  ( 9.457646018065525792E-16, -5.062499998634401699, 5.148502694627439702 ) ) ;
#40291=CARTESIAN_POINT ( 'NONE',  ( 2.229367062500001939, -72.22916666530107932, 3.861377020970579999 ) ) ;
#40292=CARTESIAN_POINT ( 'NONE',  ( 2.499999999999998668, -31.20833333060214443, -4.330127018922193649 ) ) ;
#40295=CARTESIAN_POINT ( 'NONE',  ( -6.972266317189433020E-16, -45.24999999999999289, -5.000000000000000000 ) ) ;
#40297=CARTESIAN_POINT ( 'NONE',  ( -4.458734124999998549, -44.22916666530106511, 2.574251347313722516 ) ) ;
#40298=CARTESIAN_POINT ( 'NONE',  ( -4.458734124999999437, -33.56249999863440792, 0.000000000000000000 ) ) ;
#40301=CARTESIAN_POINT ( 'NONE',  ( 1.060575238724906964E-15, 20.24999999999999645, 5.773502691896257311 ) ) ;
#40304=CARTESIAN_POINT ( 'NONE',  ( -4.458734124999999437, -43.31249999863440081, 0.000000000000000000 ) ) ;
#40305=CARTESIAN_POINT ( 'NONE',  ( 5.000000000000000000, -72.29166666393547303, -2.886751345948129988 ) ) ;
#40309=DIRECTION ( 'NONE',  ( -0.000000000000000000, 1.000000000000000000, -0.000000000000000000 ) ) ;
#40310=CARTESIAN_POINT ( 'NONE',  ( -2.229367062499996610, -81.39583333196773651, 3.861377020970582219 ) ) ;
#40314=CARTESIAN_POINT ( 'NONE',  ( -5.000000000000000000, -25.08333333333333215, -2.886751345948128211 ) ) ;
#40316=ORIENTED_EDGE ( 'NONE', *, *, #2776, .F. ) ;
#40320=CARTESIAN_POINT ( 'NONE',  ( 2.500000000000002220, 21.45833333606451987, 4.330127018922192761 ) ) ;
#40321=CARTESIAN_POINT ( 'NONE',  ( -1.339745962155727277, -60.66965819600734022, 4.999999999999933387 ) ) ;
#40326=CARTESIAN_POINT ( 'NONE',  ( 1.975475456537005874E-15, -66.74999999999998579, 5.000000000000000000 ) ) ;
#40327=DIRECTION ( 'NONE',  ( 0.000000000000000000, 0.000000000000000000, 1.000000000000000000 ) ) ;
#40328=CARTESIAN_POINT ( 'NONE',  ( -2.229367062499996610, -13.39583333196774007, 3.861377020970582219 ) ) ;
#40337=CARTESIAN_POINT ( 'NONE',  ( -6.972266317189433020E-16, -4.124999997268814056, -5.000000000000000000 ) ) ;
#40339=ORIENTED_EDGE ( 'NONE', *, *, #53535, .F. ) ;
#40347=CARTESIAN_POINT ( 'NONE',  ( 9.457646018065525792E-16, 14.93750000136559564, 5.148502694627439702 ) ) ;
#40351=DIRECTION ( 'NONE',  ( -0.000000000000000000, 1.000000000000000000, -0.000000000000000000 ) ) ;
#40352=DIRECTION ( 'NONE',  ( 0.000000000000000000, 0.000000000000000000, 1.000000000000000000 ) ) ;
#40353=CARTESIAN_POINT ( 'NONE',  ( 9.457646018065525792E-16, -65.06249999863440792, 5.148502694627439702 ) ) ;
#40355=CARTESIAN_POINT ( 'NONE',  ( -2.229367062500000163, 20.52083333469892779, -3.861377020970580443 ) ) ;
#40357=CARTESIAN_POINT ( 'NONE',  ( -2.500000000000000444, 17.83333333333333215, -4.330127018922193649 ) ) ;
#40358=DIRECTION ( 'NONE',  ( -0.000000000000000000, 1.000000000000000000, -0.000000000000000000 ) ) ;
#40359=CARTESIAN_POINT ( 'NONE',  ( -4.458734124999999437, -54.64583333196774362, -2.574251347313719407 ) ) ;
#40360=CARTESIAN_POINT ( 'NONE',  ( -5.000000000000000000, -6.958333330602150646, -2.886751345948128211 ) ) ;
#40362=CARTESIAN_POINT ( 'NONE',  ( -6.000000000000000000, -114.9999999999999858, 1.499999999999999556 ) ) ;
#40365=CARTESIAN_POINT ( 'NONE',  ( -4.458734124999999437, -18.64583333196774362, -2.574251347313719407 ) ) ;
#40368=CARTESIAN_POINT ( 'NONE',  ( 9.457646018065525792E-16, -106.0624999986343795, 5.148502694627439702 ) ) ;
#40371=CARTESIAN_POINT ( 'NONE',  ( -4.458734124999998549, -98.47916666530105090, 2.574251347313722516 ) ) ;
#40372=CARTESIAN_POINT ( 'NONE',  ( 2.229367062499998831, -28.64583333196774007, -3.861377020970580887 ) ) ;
#40373=CARTESIAN_POINT ( 'NONE',  ( -5.000000000000000000, -58.87499999726880873, 0.000000000000000000 ) ) ;
#40374=CARTESIAN_POINT ( 'NONE',  ( 5.000000000000000888, -62.45833333060213732, 2.886751345948126879 ) ) ;
#40377=CARTESIAN_POINT ( 'NONE',  ( -2.229367062500000163, -24.47916666530106866, -3.861377020970580443 ) ) ;
#40378=CARTESIAN_POINT ( 'NONE',  ( -4.458734124999999437, 6.354166668032259047, -2.574251347313719407 ) ) ;
#40379=CARTESIAN_POINT ( 'NONE',  ( 4.458734125000000326, -63.14583333196774362, 2.574251347313718519 ) ) ;
#40380=CARTESIAN_POINT ( 'NONE',  ( 0.000000000000000000, -120.0000000000000000, 0.000000000000000000 ) ) ;
#40382=FACE_OUTER_BOUND ( 'NONE', #37012, .T. ) ;
#40384=CARTESIAN_POINT ( 'NONE',  ( -4.999999999999999112, -13.91666666666666785, 2.886751345948131764 ) ) ;
#40386=ORIENTED_EDGE ( 'NONE', *, *, #49918, .F. ) ;
#40388=CARTESIAN_POINT ( 'NONE',  ( 5.000000000000000000, -38.29166666393548013, -2.886751345948130876 ) ) ;
#40391=CARTESIAN_POINT ( 'NONE',  ( 1.975475456537005874E-15, 1.375000002731185500, 5.000000000000000000 ) ) ;
#40392=CARTESIAN_POINT ( 'NONE',  ( -2.480964764533239819E-13, -95.62499999726883004, 5.000000000000000000 ) ) ;
#40393=CARTESIAN_POINT ( 'NONE',  ( -5.926426369611017623E-15, 26.25000000000000000, 5.000000000000000000 ) ) ;
#40395=CARTESIAN_POINT ( 'NONE',  ( 5.000000000000000000, -75.41666666666667140, -2.886751345948129988 ) ) ;
#40396=( BOUNDED_CURVE ( )  B_SPLINE_CURVE ( 2, ( #24650, #58432, #44256, #220, #19818, #39427, #44909, #59386, #865 ),
 .UNSPECIFIED., .F., .F. ) 
 B_SPLINE_CURVE_WITH_KNOTS ( ( 3, 2, 2, 2, 3 ),
 ( 0.8410714285714285809, 0.8416666666666666741, 0.8428571428571428603, 0.8440476190476190466, 0.8446428571428571397 ),
 .UNSPECIFIED. ) 
 CURVE ( )  GEOMETRIC_REPRESENTATION_ITEM ( )  RATIONAL_B_SPLINE_CURVE ( ( 0.9330127018922194093, 0.9330127018922194093, 1.000000000000000000, 0.8660254037844387076, 1.000000000000000000, 0.8660254037844387076, 1.000000000000000000, 0.9330127018922194093, 0.9330127018922194093 ) ) 
 REPRESENTATION_ITEM ( '' )  );
#40399=CARTESIAN_POINT ( 'NONE',  ( -2.499999999999996447, -97.83333333333332860, 4.330127018922195425 ) ) ;
#40400=ORIENTED_EDGE ( 'NONE', *, *, #30369, .T. ) ;
#40401=CARTESIAN_POINT ( 'NONE',  ( -1.339745962155613812, -51.20534180126148271, -5.000000000000000000 ) ) ;
#40405=EDGE_LOOP ( 'NONE', ( #62679, #7579, #45458, #5869 ) ) ;
#40411=CARTESIAN_POINT ( 'NONE',  ( 5.000000000000000000, -55.49999999999999289, -6.123233995736766282E-16 ) ) ;
#40412=ORIENTED_EDGE ( 'NONE', *, *, #63257, .T. ) ;
#40418=CARTESIAN_POINT ( 'NONE',  ( -3.152548672688508926E-16, -74.56249999863440792, -5.148502694627439702 ) ) ;
#40419=CARTESIAN_POINT ( 'NONE',  ( 4.458734124999998549, 27.27083333469892423, -2.574251347313721627 ) ) ;
#40422=CARTESIAN_POINT ( 'NONE',  ( -2.500000000000000444, 4.958333336064518981, -4.330127018922193649 ) ) ;
#40426=CARTESIAN_POINT ( 'NONE',  ( 2.229367062499998831, -43.64583333196773651, -3.861377020970580887 ) ) ;
#40429=CARTESIAN_POINT ( 'NONE',  ( -4.458734124999997661, -50.22916666530107221, 2.574251347313722516 ) ) ;
#40433=CARTESIAN_POINT ( 'NONE',  ( 4.458734125000001214, -17.89583333196774007, 2.574251347313718519 ) ) ;
#40434=CARTESIAN_POINT ( 'NONE',  ( -2.500000000000000444, -100.1666666666666572, -4.330127018922193649 ) ) ;
#40436=CARTESIAN_POINT ( 'NONE',  ( 2.229367062499998831, -35.89583333196773651, -3.861377020970580887 ) ) ;
#40437=CARTESIAN_POINT ( 'NONE',  ( -2.500000000000000444, 3.958333336064518093, -4.330127018922193649 ) ) ;
#40438=CARTESIAN_POINT ( 'NONE',  ( -1.339745962155613812, -7.080341798530293218, -5.000000000000000000 ) ) ;
#40441=CYLINDRICAL_SURFACE ( 'NONE', #4500, 5.000000000000000000 ) ;
#40442=DIRECTION ( 'NONE',  ( -0.000000000000000000, 1.000000000000000000, -0.000000000000000000 ) ) ;
#40443=( BOUNDED_CURVE ( )  B_SPLINE_CURVE ( 2, ( #13940, #53807, #34185, #53496, #9119, #48353, #19071, #58644, #33877 ),
 .UNSPECIFIED., .F., .F. ) 
 B_SPLINE_CURVE_WITH_KNOTS ( ( 3, 2, 2, 2, 3 ),
 ( 0.5232142857142857428, 0.5238095238095238360, 0.5250000000000000222, 0.5261904761904762085, 0.5267857142857143016 ),
 .UNSPECIFIED. ) 
 CURVE ( )  GEOMETRIC_REPRESENTATION_ITEM ( )  RATIONAL_B_SPLINE_CURVE ( ( 0.9330127018922194093, 0.9330127018922194093, 1.000000000000000000, 0.8660254037844387076, 1.000000000000000000, 0.8660254037844387076, 1.000000000000000000, 0.9330127018922194093, 0.9330127018922194093 ) ) 
 REPRESENTATION_ITEM ( '' )  );
#40444=CARTESIAN_POINT ( 'NONE',  ( -2.229367062499996610, 1.604166668032262155, 3.861377020970582219 ) ) ;
#40446=CARTESIAN_POINT ( 'NONE',  ( 1.975475456537005874E-15, -30.74999999999999645, 5.000000000000000000 ) ) ;
#40448=CARTESIAN_POINT ( 'NONE',  ( -3.152548672688508926E-16, -86.56249999863440792, -5.148502694627439702 ) ) ;
#40449=CARTESIAN_POINT ( 'NONE',  ( 2.229367062500001939, -36.97916666530107221, 3.861377020970579999 ) ) ;
#40450=EDGE_CURVE ( 'NONE', #19298, #43561, #56521, .T. ) ;
#40451=CARTESIAN_POINT ( 'NONE',  ( 1.339745962155616255, 27.70534180126147916, -4.999999999999997335 ) ) ;
#40452=CARTESIAN_POINT ( 'NONE',  ( 4.458734125000001214, -84.14583333196772230, 2.574251347313718519 ) ) ;
#40454=CARTESIAN_POINT ( 'NONE',  ( 0.000000000000000000, -120.0000000000000000, 5.000000000000000000 ) ) ;
#40457=CARTESIAN_POINT ( 'NONE',  ( -4.458734124999999437, -8.312499998634406140, 0.000000000000000000 ) ) ;
#40458=CARTESIAN_POINT ( 'NONE',  ( 4.458734124999999437, 19.93750000136559208, -5.460374474430324690E-16 ) ) ;
#40459=EDGE_CURVE ( 'NONE', #23800, #27082, #4187, .T. ) ;
#40460=CARTESIAN_POINT ( 'NONE',  ( 4.458734124999998549, -47.97916666530106511, -2.574251347313721627 ) ) ;
#40461=CARTESIAN_POINT ( 'NONE',  ( 5.000000000000000000, -11.49999999999999645, -6.123233995736766282E-16 ) ) ;
#40467=CARTESIAN_POINT ( 'NONE',  ( -4.458734124999999437, -77.39583333196772230, -2.574251347313719407 ) ) ;
#40468=CARTESIAN_POINT ( 'NONE',  ( -4.458734124999999437, 29.35416666803225993, -2.574251347313719407 ) ) ;
#40473=CARTESIAN_POINT ( 'NONE',  ( -5.000000000000000000, -56.99999999999999289, 0.000000000000000000 ) ) ;
#40477=CARTESIAN_POINT ( 'NONE',  ( 5.000000000000000000, -52.37499999726881583, -6.123233995736766282E-16 ) ) ;
#40487=CARTESIAN_POINT ( 'NONE',  ( 1.975475456537005874E-15, 11.37500000273118239, 5.000000000000000000 ) ) ;
#40493=CARTESIAN_POINT ( 'NONE',  ( -4.458734124999999437, -45.56249999863440081, 0.000000000000000000 ) ) ;
#40494=CARTESIAN_POINT ( 'NONE',  ( 1.339745962155612702, -23.29465819873851729, -5.000000000000000000 ) ) ;
#40501=CARTESIAN_POINT ( 'NONE',  ( 0.000000000000000000, -120.0000000000000000, 0.000000000000000000 ) ) ;
#40503=CARTESIAN_POINT ( 'NONE',  ( -4.458734124999998549, -96.47916666530105090, 2.574251347313722516 ) ) ;
#40504=FACE_OUTER_BOUND ( 'NONE', #63461, .T. ) ;
#40505=VERTEX_POINT ( 'NONE', #34380 ) ;
#40509=CARTESIAN_POINT ( 'NONE',  ( 5.000000000000000000, -38.41666666666667140, -2.886751345948130876 ) ) ;
#40511=CARTESIAN_POINT ( 'NONE',  ( -3.152548672688508926E-16, -4.562499998634401699, -5.148502694627439702 ) ) ;
#40512=EDGE_CURVE ( 'NONE', #38980, #8862, #9311, .T. ) ;
#40514=CARTESIAN_POINT ( 'NONE',  ( 5.000000000000000000, 6.499999999999999112, -6.123233995736766282E-16 ) ) ;
#40515=CARTESIAN_POINT ( 'NONE',  ( -4.458734124999999437, -17.64583333196773651, -2.574251347313719407 ) ) ;
#40516=CARTESIAN_POINT ( 'NONE',  ( -5.000000000000000000, -100.9583333306021444, -2.886751345948128211 ) ) ;
#40519=CARTESIAN_POINT ( 'NONE',  ( -4.458734124999999437, 15.43750000136559386, 0.000000000000000000 ) ) ;
#40521=CARTESIAN_POINT ( 'NONE',  ( -2.499999999999996447, -13.70833333060214976, 4.330127018922195425 ) ) ;
#40522=CARTESIAN_POINT ( 'NONE',  ( -4.999999999999998224, -20.91666666666666785, 2.886751345948131764 ) ) ;
#40523=CARTESIAN_POINT ( 'NONE',  ( -2.229367062500000163, -19.47916666530106866, -3.861377020970580443 ) ) ;
#40529=CARTESIAN_POINT ( 'NONE',  ( -3.535250795749689387E-16, -49.12499999726881583, -5.773502691896257311 ) ) ;
#40531=CARTESIAN_POINT ( 'NONE',  ( -4.458734124999997661, 13.77083333469892779, 2.574251347313722516 ) ) ;
#40532=CARTESIAN_POINT ( 'NONE',  ( 1.339745962155615144, -35.70534180126148271, 4.999999999999999112 ) ) ;
#40533=EDGE_CURVE ( 'NONE', #57369, #26645, #19101, .T. ) ;
#40534=FACE_OUTER_BOUND ( 'NONE', #14542, .T. ) ;
#40536=CARTESIAN_POINT ( 'NONE',  ( 4.458734124999998549, -66.72916666530106511, -2.574251347313721627 ) ) ;
#40538=CARTESIAN_POINT ( 'NONE',  ( 1.060575238724906964E-15, 2.249999999999998668, 5.773502691896257311 ) ) ;
#40541=CARTESIAN_POINT ( 'NONE',  ( 9.457646018065525792E-16, -57.06249999863440081, 5.148502694627439702 ) ) ;
#40542=CARTESIAN_POINT ( 'NONE',  ( -2.500000000000000444, -96.04166666393548724, -4.330127018922193649 ) ) ;
#40544=CARTESIAN_POINT ( 'NONE',  ( 0.000000000000000000, -120.0000000000000000, 5.000000000000000000 ) ) ;
#40546=CARTESIAN_POINT ( 'NONE',  ( 1.975475456537005874E-15, -69.74999999999998579, 5.000000000000000000 ) ) ;
#40550=CARTESIAN_POINT ( 'NONE',  ( -3.535250795749689387E-16, -42.24999999999999289, -5.773502691896257311 ) ) ;
#40552=CARTESIAN_POINT ( 'NONE',  ( -2.500000000000000444, -108.1666666666666572, -4.330127018922193649 ) ) ;
#40554=CARTESIAN_POINT ( 'NONE',  ( -2.229367062499996610, -109.1458333319677365, 3.861377020970582219 ) ) ;
#40555=CARTESIAN_POINT ( 'NONE',  ( 2.229367062499998831, -1.895833331967737623, -3.861377020970580887 ) ) ;
#40562=EDGE_LOOP ( 'NONE', ( #6477, #49807, #15591, #20992 ) ) ;
#40564=CARTESIAN_POINT ( 'NONE',  ( -2.499999999999996447, 28.29166666939785202, 4.330127018922195425 ) ) ;
#40567=CARTESIAN_POINT ( 'NONE',  ( 5.000000000000000000, -101.4166666666666572, -2.886751345948130876 ) ) ;
#40569=CARTESIAN_POINT ( 'NONE',  ( -2.229367062499996610, -31.39583333196773651, 3.861377020970582219 ) ) ;
#40577=CARTESIAN_POINT ( 'NONE',  ( -2.499999999999996447, -82.70833333060214443, 4.330127018922195425 ) ) ;
#40579=CARTESIAN_POINT ( 'NONE',  ( 4.458734124999998549, -78.97916666530106511, -2.574251347313721627 ) ) ;
#40582=LINE ( 'NONE', #11946, #16234 ) ;
#40583=CARTESIAN_POINT ( 'NONE',  ( -6.972266317189433020E-16, -31.12499999726880873, -5.000000000000000000 ) ) ;
#40585=CARTESIAN_POINT ( 'NONE',  ( -4.458734124999999437, -4.645833331967739177, -2.574251347313719407 ) ) ;
#40586=ORIENTED_EDGE ( 'NONE', *, *, #27521, .T. ) ;
#40590=CARTESIAN_POINT ( 'NONE',  ( 1.339745962155612702, -27.29465819873852084, -5.000000000000000000 ) ) ;
#40597=ORIENTED_EDGE ( 'NONE', *, *, #48531, .F. ) ;
#40598=CARTESIAN_POINT ( 'NONE',  ( -3.152548672688508926E-16, -82.56249999863440792, -5.148502694627439702 ) ) ;
#40600=CARTESIAN_POINT ( 'NONE',  ( -2.229367062500000163, -5.479166665301072214, -3.861377020970580443 ) ) ;
#40603=CARTESIAN_POINT ( 'NONE',  ( -4.458734124999998549, -69.47916666530107932, 2.574251347313722516 ) ) ;
#40604=CARTESIAN_POINT ( 'NONE',  ( -2.499999999999996447, -28.70833333060214798, 4.330127018922195425 ) ) ;
#40606=CARTESIAN_POINT ( 'NONE',  ( -2.499999999999996447, -0.7083333306021483144, 4.330127018922195425 ) ) ;
#40607=CARTESIAN_POINT ( 'NONE',  ( -2.500000000000000444, 22.83333333333333215, -4.330127018922193649 ) ) ;
#40610=CARTESIAN_POINT ( 'NONE',  ( 4.458734124999999437, -53.81249999863439371, -5.460374474430324690E-16 ) ) ;
#40611=CARTESIAN_POINT ( 'NONE',  ( -2.229367062500000163, -32.72916666530106511, -3.861377020970580443 ) ) ;
#40614=CARTESIAN_POINT ( 'NONE',  ( 5.000000000000000000, 21.58333333333333215, -2.886751345948129988 ) ) ;
#40615=EDGE_CURVE ( 'NONE', #9483, #39986, #8425, .T. ) ;
#40617=CARTESIAN_POINT ( 'NONE',  ( -6.972266317189433020E-16, -26.12499999726881583, -5.000000000000000000 ) ) ;
#40618=CARTESIAN_POINT ( 'NONE',  ( -2.229367062500000163, -40.47916666530107221, -3.861377020970580443 ) ) ;
#40619=CARTESIAN_POINT ( 'NONE',  ( -2.500000000000000444, -80.04166666393547303, -4.330127018922193649 ) ) ;
#40622=EDGE_CURVE ( 'NONE', #40086, #16789, #14974, .T. ) ;
#40623=CARTESIAN_POINT ( 'NONE',  ( 1.339745962155612702, -15.16965819600733134, -5.000000000000000000 ) ) ;
#40624=CARTESIAN_POINT ( 'NONE',  ( -2.229367062499996610, -80.39583333196773651, 3.861377020970582219 ) ) ;
#40626=CARTESIAN_POINT ( 'NONE',  ( 5.000000000000000000, 13.62500000273118417, -6.123233995736766282E-16 ) ) ;
#40627=CARTESIAN_POINT ( 'NONE',  ( -5.000000000000000000, -28.08333333333333925, -2.886751345948128211 ) ) ;
#40629=ORIENTED_EDGE ( 'NONE', *, *, #11470, .F. ) ;
#40631=ORIENTED_EDGE ( 'NONE', *, *, #7231, .F. ) ;
#40634=CARTESIAN_POINT ( 'NONE',  ( -2.499999999999996447, 23.29166666939785202, 4.330127018922195425 ) ) ;
#40641=CARTESIAN_POINT ( 'NONE',  ( -6.972266317189433020E-16, -99.12499999726880162, -5.000000000000000000 ) ) ;
#40645=CARTESIAN_POINT ( 'NONE',  ( 5.000000000000000000, -74.41666666666665719, -2.886751345948130876 ) ) ;
#40647=CARTESIAN_POINT ( 'NONE',  ( 9.457646018065525792E-16, -15.31249999863440436, 5.148502694627439702 ) ) ;
#40648=DIRECTION ( 'NONE',  ( -0.000000000000000000, 1.000000000000000000, -0.000000000000000000 ) ) ;
#40657=DIRECTION ( 'NONE',  ( -0.000000000000000000, 1.000000000000000000, -0.000000000000000000 ) ) ;
#40659=ORIENTED_EDGE ( 'NONE', *, *, #11829, .F. ) ;
#40660=CARTESIAN_POINT ( 'NONE',  ( -1.339745962155613812, -10.20534180126147739, -5.000000000000000000 ) ) ;
#40662=CARTESIAN_POINT ( 'NONE',  ( -6.972266317189433020E-16, 4.749999999999999112, -5.000000000000000000 ) ) ;
#40665=CARTESIAN_POINT ( 'NONE',  ( 4.458734124999999437, 14.18750000136559386, -5.460374474430324690E-16 ) ) ;
#40671=CARTESIAN_POINT ( 'NONE',  ( 9.457646018065525792E-16, -64.06249999863440792, 5.148502694627439702 ) ) ;
#40673=CARTESIAN_POINT ( 'NONE',  ( -3.152548672688508926E-16, 14.43750000136559386, -5.148502694627439702 ) ) ;
#40674=CARTESIAN_POINT ( 'NONE',  ( -2.499999999999996447, -69.70833333060214443, 4.330127018922195425 ) ) ;
#40676=CARTESIAN_POINT ( 'NONE',  ( 2.229367062499998831, -56.89583333196773651, -3.861377020970580887 ) ) ;
#40677=CARTESIAN_POINT ( 'NONE',  ( -2.500000000000000444, -17.04166666393548368, -4.330127018922193649 ) ) ;
#40678=CARTESIAN_POINT ( 'NONE',  ( -1.975475456537005874E-15, 29.25000000000000000, 5.000000000000000000 ) ) ;
#40680=CARTESIAN_POINT ( 'NONE',  ( -8.660254037844341113, 45.00000000000000000, 6.047423072554883697E-14 ) ) ;
#40682=CARTESIAN_POINT ( 'NONE',  ( 4.458734124999998549, -18.97916666530106511, -2.574251347313721627 ) ) ;
#40684=CARTESIAN_POINT ( 'NONE',  ( 2.500000000000002220, 23.33333333333333215, 4.330127018922192761 ) ) ;
#40685=CARTESIAN_POINT ( 'NONE',  ( 2.229367062499998831, -102.6458333319677365, -3.861377020970580887 ) ) ;
#40687=ORIENTED_EDGE ( 'NONE', *, *, #16123, .F. ) ;
#40688=CARTESIAN_POINT ( 'NONE',  ( -2.229367062500000163, -101.7291666653010651, -3.861377020970580443 ) ) ;
#40689=CARTESIAN_POINT ( 'NONE',  ( 4.458734124999998549, -26.72916666530106866, -2.574251347313721627 ) ) ;
#40690=CARTESIAN_POINT ( 'NONE',  ( 5.000000000000000000, -56.29166666393548013, -2.886751345948129988 ) ) ;
#40693=CARTESIAN_POINT ( 'NONE',  ( -2.229367062499996610, -26.14583333196773651, 3.861377020970582219 ) ) ;
#40694=CARTESIAN_POINT ( 'NONE',  ( -2.229367062499996610, -64.39583333196773651, 3.861377020970582219 ) ) ;
#40695=CARTESIAN_POINT ( 'NONE',  ( -1.339745962155610925, -39.66965819600733312, 5.000000000000000000 ) ) ;
#40699=CARTESIAN_POINT ( 'NONE',  ( 2.499999999999998668, -13.33333333333333570, -4.330127018922193649 ) ) ;
#40701=ORIENTED_EDGE ( 'NONE', *, *, #1374, .T. ) ;
#40703=FACE_OUTER_BOUND ( 'NONE', #37900, .T. ) ;
#40704=CARTESIAN_POINT ( 'NONE',  ( 1.975475456537005874E-15, -90.74999999999998579, 5.000000000000000000 ) ) ;
#40707=DIRECTION ( 'NONE',  ( 0.000000000000000000, 0.000000000000000000, 1.000000000000000000 ) ) ;
#40709=FACE_OUTER_BOUND ( 'NONE', #41120, .T. ) ;
#40711=CARTESIAN_POINT ( 'NONE',  ( -5.000000000000000000, -80.08333333333332860, -2.886751345948128211 ) ) ;
#40717=LINE ( 'NONE', #59722, #59415 ) ;
#40721=( BOUNDED_CURVE ( )  B_SPLINE_CURVE ( 2, ( #26113, #50876, #45732, #1685, #11622, #22569, #21286, #60538, #36079 ),
 .UNSPECIFIED., .F., .F. ) 
 B_SPLINE_CURVE_WITH_KNOTS ( ( 3, 2, 2, 2, 3 ),
 ( 0.8767857142857142794, 0.8773809523809523725, 0.8785714285714285587, 0.8797619047619047450, 0.8803571428571428381 ),
 .UNSPECIFIED. ) 
 CURVE ( )  GEOMETRIC_REPRESENTATION_ITEM ( )  RATIONAL_B_SPLINE_CURVE ( ( 0.9330127018922194093, 0.9330127018922194093, 1.000000000000000000, 0.8660254037844387076, 1.000000000000000000, 0.8660254037844387076, 1.000000000000000000, 0.9330127018922194093, 0.9330127018922194093 ) ) 
 REPRESENTATION_ITEM ( '' )  );
#40733=CARTESIAN_POINT ( 'NONE',  ( 2.500000000000002220, -41.54166666393548013, 4.330127018922192761 ) ) ;
#40734=ORIENTED_EDGE ( 'NONE', *, *, #55138, .F. ) ;
#40735=CARTESIAN_POINT ( 'NONE',  ( -2.229367062500000163, -79.47916666530106511, -3.861377020970580443 ) ) ;
#40736=CARTESIAN_POINT ( 'NONE',  ( 2.229367062500001939, -108.2291666653010651, 3.861377020970579999 ) ) ;
#40739=CARTESIAN_POINT ( 'NONE',  ( 0.000000000000000000, -120.0000000000000000, 5.000000000000000000 ) ) ;
#40743=CARTESIAN_POINT ( 'NONE',  ( -2.229367062499996610, -45.14583333196774362, 3.861377020970582219 ) ) ;
#40745=CARTESIAN_POINT ( 'NONE',  ( 1.975475456537005874E-15, -13.62499999726881228, 5.000000000000000000 ) ) ;
#40746=CARTESIAN_POINT ( 'NONE',  ( -2.229367062499996610, -50.14583333196772941, 3.861377020970582219 ) ) ;
#40748=CARTESIAN_POINT ( 'NONE',  ( -3.152548672688508926E-16, 29.43750000136559564, -5.148502694627439702 ) ) ;
#40749=CARTESIAN_POINT ( 'NONE',  ( -4.458734124999999437, -16.31249999863440436, 0.000000000000000000 ) ) ;
#40750=CARTESIAN_POINT ( 'NONE',  ( -3.535250795749689387E-16, -102.2500000000000000, -5.773502691896257311 ) ) ;
#40752=CARTESIAN_POINT ( 'NONE',  ( -2.229367062500000163, -37.72916666530107221, -3.861377020970580443 ) ) ;
#40753=CARTESIAN_POINT ( 'NONE',  ( 1.060575238724906964E-15, 3.375000002731186388, 5.773502691896257311 ) ) ;
#40757=CARTESIAN_POINT ( 'NONE',  ( 2.499999999999998668, -71.33333333333332860, -4.330127018922193649 ) ) ;
#40759=CARTESIAN_POINT ( 'NONE',  ( -4.458734124999997661, 1.520833334698927564, 2.574251347313722516 ) ) ;
#40760=ORIENTED_EDGE ( 'NONE', *, *, #57812, .T. ) ;
#40764=CARTESIAN_POINT ( 'NONE',  ( -2.229367062500000163, -90.47916666530106511, -3.861377020970580443 ) ) ;
#40765=CARTESIAN_POINT ( 'NONE',  ( -4.458734124999998549, -37.22916666530107221, 2.574251347313722516 ) ) ;
#40767=CARTESIAN_POINT ( 'NONE',  ( -2.229367062499996610, -86.39583333196773651, 3.861377020970582219 ) ) ;
#40768=VECTOR ( 'NONE', #5124, 1000.000000000000000 ) ;
#40770=DIRECTION ( 'NONE',  ( -0.000000000000000000, 1.000000000000000000, -0.000000000000000000 ) ) ;
#40772=CARTESIAN_POINT ( 'NONE',  ( -2.229367062499996610, -8.145833331967736513, 3.861377020970582219 ) ) ;
#40773=CARTESIAN_POINT ( 'NONE',  ( 4.458734124999999437, 23.93750000136559564, -5.460374474430324690E-16 ) ) ;
#40774=CARTESIAN_POINT ( 'NONE',  ( 4.458734125000000326, -50.14583333196772230, 2.574251347313718519 ) ) ;
#40779=ORIENTED_EDGE ( 'NONE', *, *, #57123, .T. ) ;
#40782=CARTESIAN_POINT ( 'NONE',  ( 4.458734124999999437, -72.81249999863439371, -5.460374474430324690E-16 ) ) ;
#40783=CARTESIAN_POINT ( 'NONE',  ( -4.458734124999999437, 27.35416666803225993, -2.574251347313719407 ) ) ;
#40788=CARTESIAN_POINT ( 'NONE',  ( -4.999999999999999112, -62.91666666666667140, 2.886751345948131764 ) ) ;
#40789=FACE_OUTER_BOUND ( 'NONE', #47532, .T. ) ;
#40791=VERTEX_POINT ( 'NONE', #10901 ) ;
#40792=CYLINDRICAL_SURFACE ( 'NONE', #9851, 5.000000000000000000 ) ;
#40793=CARTESIAN_POINT ( 'NONE',  ( -6.972266317189433020E-16, -67.25000000000000000, -5.000000000000000000 ) ) ;
#40797=EDGE_CURVE ( 'NONE', #55752, #14724, #54441, .T. ) ;
#40807=CARTESIAN_POINT ( 'NONE',  ( 4.458734125000001214, -46.14583333196773651, 2.574251347313718519 ) ) ;
#40810=CARTESIAN_POINT ( 'NONE',  ( 1.975475456537005874E-15, -21.62499999726880873, 5.000000000000000000 ) ) ;
#40816=CARTESIAN_POINT ( 'NONE',  ( -5.000000000000000000, -58.87499999726880873, 0.000000000000000000 ) ) ;
#40819=CARTESIAN_POINT ( 'NONE',  ( 2.229367062499998831, -94.89583333196773651, -3.861377020970580887 ) ) ;
#40827=ORIENTED_EDGE ( 'NONE', *, *, #3219, .T. ) ;
#40829=CARTESIAN_POINT ( 'NONE',  ( 2.229367062499998831, -4.645833331967740065, -3.861377020970580887 ) ) ;
#40830=CARTESIAN_POINT ( 'NONE',  ( 2.499999999999998668, -1.208333330602148870, -4.330127018922193649 ) ) ;
#40831=CARTESIAN_POINT ( 'NONE',  ( 2.229367062500001939, -23.22916666530107221, 3.861377020970579999 ) ) ;
#40832=CARTESIAN_POINT ( 'NONE',  ( 1.339745962155615144, -70.70534180126148271, 4.999999999999999112 ) ) ;
#40836=CARTESIAN_POINT ( 'NONE',  ( -4.458734124999999437, 16.35416666803225993, -2.574251347313719407 ) ) ;
#40839=CARTESIAN_POINT ( 'NONE',  ( 1.975475456537005874E-15, -98.74999999999998579, 5.000000000000000000 ) ) ;
#40840=CARTESIAN_POINT ( 'NONE',  ( 4.458734124999999437, -17.81249999863440792, -5.460374474430324690E-16 ) ) ;
#40845=CARTESIAN_POINT ( 'NONE',  ( 5.000000000000000888, -44.45833333060214443, 2.886751345948126879 ) ) ;
#40846=CARTESIAN_POINT ( 'NONE',  ( 0.000000000000000000, -120.0000000000000000, 0.000000000000000000 ) ) ;
#40847=CARTESIAN_POINT ( 'NONE',  ( -4.458734124999999437, 6.687500001365593860, 0.000000000000000000 ) ) ;
#40851=CARTESIAN_POINT ( 'NONE',  ( 4.458734124999999437, -67.81249999863440792, -5.460374474430324690E-16 ) ) ;
#40853=CARTESIAN_POINT ( 'NONE',  ( -3.535250795749689387E-16, -3.250000000000003109, -5.773502691896257311 ) ) ;
#40856=CARTESIAN_POINT ( 'NONE',  ( -4.458734124999999437, -61.31249999863440081, 0.000000000000000000 ) ) ;
#40857=CARTESIAN_POINT ( 'NONE',  ( 1.060575238724906964E-15, -96.62499999726880162, 5.773502691896257311 ) ) ;
#40858=AXIS2_PLACEMENT_3D ( 'NONE', #38021, #57653, #13579 ) ;
#40859=CARTESIAN_POINT ( 'NONE',  ( -1.339745962155613812, -80.20534180126148271, -5.000000000000000000 ) ) ;
#40860=DIRECTION ( 'NONE',  ( -0.000000000000000000, 1.000000000000000000, -0.000000000000000000 ) ) ;
#40863=CARTESIAN_POINT ( 'NONE',  ( -2.499999999999996447, -45.83333333333333570, 4.330127018922195425 ) ) ;
#40866=EDGE_LOOP ( 'NONE', ( #37743, #11991, #37395, #38368 ) ) ;
#40867=CARTESIAN_POINT ( 'NONE',  ( 4.458734124999999437, -108.8124999986343937, -5.460374474430324690E-16 ) ) ;
#40868=CARTESIAN_POINT ( 'NONE',  ( 2.229367062499998831, -3.895833331967739177, -3.861377020970580887 ) ) ;
#40869=CARTESIAN_POINT ( 'NONE',  ( 2.500000000000002220, -59.66666666666665719, 4.330127018922192761 ) ) ;
#40874=EDGE_CURVE ( 'NONE', #62900, #45629, #10465, .T. ) ;
#40879=CARTESIAN_POINT ( 'NONE',  ( 1.975475456537005874E-15, -22.62499999726880873, 5.000000000000000000 ) ) ;
#40884=CARTESIAN_POINT ( 'NONE',  ( 4.458734124999998549, -29.97916666530107577, -2.574251347313721627 ) ) ;
#40891=CARTESIAN_POINT ( 'NONE',  ( -6.972266317189433020E-16, -70.12499999726880162, -5.000000000000000000 ) ) ;
#40892=ORIENTED_EDGE ( 'NONE', *, *, #13548, .F. ) ;
#40894=CARTESIAN_POINT ( 'NONE',  ( 2.229367062499998831, -80.89583333196773651, -3.861377020970580887 ) ) ;
#40899=CYLINDRICAL_SURFACE ( 'NONE', #37344, 5.000000000000000000 ) ;
#40902=CARTESIAN_POINT ( 'NONE',  ( -2.229367062499996610, -2.395833331967737845, 3.861377020970582219 ) ) ;
#40904=( BOUNDED_CURVE ( )  B_SPLINE_CURVE ( 2, ( #50615, #41264, #11681, #60914, #2375, #12001, #41578, #17153, #56409 ),
 .UNSPECIFIED., .F., .F. ) 
 B_SPLINE_CURVE_WITH_KNOTS ( ( 3, 2, 2, 2, 3 ),
 ( 0.5839285714285714635, 0.5845238095238095566, 0.5857142857142857428, 0.5869047619047619291, 0.5875000000000000222 ),
 .UNSPECIFIED. ) 
 CURVE ( )  GEOMETRIC_REPRESENTATION_ITEM ( )  RATIONAL_B_SPLINE_CURVE ( ( 0.9330127018922194093, 0.9330127018922194093, 1.000000000000000000, 0.8660254037844387076, 1.000000000000000000, 0.8660254037844387076, 1.000000000000000000, 0.9330127018922194093, 0.9330127018922194093 ) ) 
 REPRESENTATION_ITEM ( '' )  );
#40905=CARTESIAN_POINT ( 'NONE',  ( 1.975475456537005874E-15, -9.624999997268814056, 5.000000000000000000 ) ) ;
#40906=EDGE_LOOP ( 'NONE', ( #2149, #33228, #4338, #59629 ) ) ;
#40907=CARTESIAN_POINT ( 'NONE',  ( 1.975475456537005874E-15, -91.74999999999998579, 5.000000000000000000 ) ) ;
#40913=CARTESIAN_POINT ( 'NONE',  ( -4.458734124999999437, -86.39583333196772230, -2.574251347313719407 ) ) ;
#40914=CARTESIAN_POINT ( 'NONE',  ( 1.339745962155615144, -75.70534180126148271, 4.999999999999999112 ) ) ;
#40915=CARTESIAN_POINT ( 'NONE',  ( -2.229367062499996610, -2.145833331967737845, 3.861377020970582219 ) ) ;
#40917=( BOUNDED_CURVE ( )  B_SPLINE_CURVE ( 2, ( #48309, #43792, #63439, #19355, #38968, #58606, #50863, #11613, #49580 ),
 .UNSPECIFIED., .F., .F. ) 
 B_SPLINE_CURVE_WITH_KNOTS ( ( 3, 2, 2, 2, 3 ),
 ( 0.03392857142857143293, 0.03452380952380952606, 0.03571428571428571230, 0.03690476190476190549, 0.03750000000000000555 ),
 .UNSPECIFIED. ) 
 CURVE ( )  GEOMETRIC_REPRESENTATION_ITEM ( )  RATIONAL_B_SPLINE_CURVE ( ( 0.9330127018922194093, 0.9330127018922197424, 1.000000000000000000, 0.8660254037844387076, 1.000000000000000000, 0.8660254037844387076, 1.000000000000000000, 0.9330127018922189652, 0.9330127018922194093 ) ) 
 REPRESENTATION_ITEM ( '' )  );
#40918=CARTESIAN_POINT ( 'NONE',  ( 2.499999999999998668, -30.20833333060214443, -4.330127018922193649 ) ) ;
#40919=CYLINDRICAL_SURFACE ( 'NONE', #7057, 5.000000000000000000 ) ;
#40920=CARTESIAN_POINT ( 'NONE',  ( -4.458734124999997661, 23.77083333469892423, 2.574251347313722516 ) ) ;
#40923=CARTESIAN_POINT ( 'NONE',  ( 4.458734124999998549, -48.72916666530107221, -2.574251347313721627 ) ) ;
#40924=CARTESIAN_POINT ( 'NONE',  ( -2.229367062499996610, -38.39583333196773651, 3.861377020970582219 ) ) ;
#40926=CARTESIAN_POINT ( 'NONE',  ( -5.000000000000000000, 19.91666666666666785, -2.886751345948128211 ) ) ;
#40928=CARTESIAN_POINT ( 'NONE',  ( 0.000000000000000000, -120.0000000000000000, 0.000000000000000000 ) ) ;
#40929=CARTESIAN_POINT ( 'NONE',  ( -4.458734124999999437, -40.39583333196773651, -2.574251347313719407 ) ) ;
#40930=CARTESIAN_POINT ( 'NONE',  ( -2.499999999999996447, -78.70833333060214443, 4.330127018922195425 ) ) ;
#40934=CARTESIAN_POINT ( 'NONE',  ( -4.458734124999999437, -82.64583333196773651, -2.574251347313719407 ) ) ;
#40937=CARTESIAN_POINT ( 'NONE',  ( -4.999999999999999112, -28.91666666666666430, 2.886751345948131764 ) ) ;
#40942=CARTESIAN_POINT ( 'NONE',  ( -3.152548672688508926E-16, -89.56249999863439371, -5.148502694627439702 ) ) ;
#40943=CARTESIAN_POINT ( 'NONE',  ( -4.458734124999998549, 12.52083333469892779, 2.574251347313722516 ) ) ;
#40944=CARTESIAN_POINT ( 'NONE',  ( -2.500000000000000444, 15.95833333606451809, -4.330127018922193649 ) ) ;
#40947=AXIS2_PLACEMENT_3D ( 'NONE', #53547, #58685, #30043 ) ;
#40950=CARTESIAN_POINT ( 'NONE',  ( -6.972266317189433020E-16, -61.12499999726880162, -5.000000000000000000 ) ) ;
#40957=CARTESIAN_POINT ( 'NONE',  ( -5.000000000000000000, -62.08333333333332860, -2.886751345948128211 ) ) ;
#40959=CARTESIAN_POINT ( 'NONE',  ( 5.000000000000000888, -74.58333333333332860, 2.886751345948126879 ) ) ;
#40961=CARTESIAN_POINT ( 'NONE',  ( 2.229367062499998831, -13.89583333196774184, -3.861377020970580887 ) ) ;
#40962=LINE ( 'NONE', #59647, #54310 ) ;
#40967=ADVANCED_FACE ( 'NONE', ( #27148 ), #27770, .T. ) ;
#40971=LINE ( 'NONE', #2701, #53801 ) ;
#40974=CARTESIAN_POINT ( 'NONE',  ( 1.339745962155615144, -58.70534180126147561, 4.999999999999999112 ) ) ;
#40978=( BOUNDED_CURVE ( )  B_SPLINE_CURVE ( 2, ( #47346, #42823, #8115, #47031, #22598, #42508, #27400, #18388, #12611 ),
 .UNSPECIFIED., .F., .F. ) 
 B_SPLINE_CURVE_WITH_KNOTS ( ( 3, 2, 2, 2, 3 ),
 ( 0.9053571428571428603, 0.9059523809523809534, 0.9071428571428571397, 0.9083333333333333259, 0.9089285714285714191 ),
 .UNSPECIFIED. ) 
 CURVE ( )  GEOMETRIC_REPRESENTATION_ITEM ( )  RATIONAL_B_SPLINE_CURVE ( ( 0.9330127018922194093, 0.9330127018922194093, 1.000000000000000000, 0.8660254037844387076, 1.000000000000000000, 0.8660254037844387076, 1.000000000000000000, 0.9330127018922194093, 0.9330127018922194093 ) ) 
 REPRESENTATION_ITEM ( '' )  );
#40980=EDGE_CURVE ( 'NONE', #63269, #17397, #15442, .T. ) ;
#40984=VERTEX_POINT ( 'NONE', #48879 ) ;
#40986=CARTESIAN_POINT ( 'NONE',  ( -3.152548672688508926E-16, 12.43750000136559564, -5.148502694627439702 ) ) ;
#40989=CARTESIAN_POINT ( 'NONE',  ( 2.499999999999998668, -78.20833333060214443, -4.330127018922193649 ) ) ;
#40992=CARTESIAN_POINT ( 'NONE',  ( -3.152548672688508926E-16, -65.56249999863440792, -5.148502694627439702 ) ) ;
#40993=CARTESIAN_POINT ( 'NONE',  ( 6.123233995736766282E-16, -120.0000000000000000, -5.000000000000000000 ) ) ;
#40994=CARTESIAN_POINT ( 'NONE',  ( -2.229367062500000163, 12.52083333469892601, -3.861377020970580443 ) ) ;
#40997=CARTESIAN_POINT ( 'NONE',  ( -2.229367062500000163, -55.72916666530107221, -3.861377020970580443 ) ) ;
#40998=CARTESIAN_POINT ( 'NONE',  ( 1.060575238724906964E-15, -12.62499999726881050, 5.773502691896257311 ) ) ;
#40999=CARTESIAN_POINT ( 'NONE',  ( 0.000000000000000000, -120.0000000000000000, 0.000000000000000000 ) ) ;
#41001=CARTESIAN_POINT ( 'NONE',  ( 5.000000000000000888, -64.45833333060213022, 2.886751345948126879 ) ) ;
#41002=( BOUNDED_CURVE ( )  B_SPLINE_CURVE ( 2, ( #55996, #7106, #26720, #16433, #27343, #11595, #31216, #50846, #26396 ),
 .UNSPECIFIED., .F., .F. ) 
 B_SPLINE_CURVE_WITH_KNOTS ( ( 3, 2, 2, 2, 3 ),
 ( 0.8553571428571428159, 0.8559523809523809090, 0.8571428571428570953, 0.8583333333333332815, 0.8589285714285714857 ),
 .UNSPECIFIED. ) 
 CURVE ( )  GEOMETRIC_REPRESENTATION_ITEM ( )  RATIONAL_B_SPLINE_CURVE ( ( 0.9330127018922194093, 0.9330127018922194093, 1.000000000000000000, 0.8660254037844387076, 1.000000000000000000, 0.8660254037844387076, 1.000000000000000000, 0.9330127018922130810, 0.9330127018922194093 ) ) 
 REPRESENTATION_ITEM ( '' )  );
#41003=CARTESIAN_POINT ( 'NONE',  ( -3.152548672688508926E-16, -22.81249999863440436, -5.148502694627439702 ) ) ;
#41005=CARTESIAN_POINT ( 'NONE',  ( -2.500000000000000444, -102.1666666666666572, -4.330127018922193649 ) ) ;
#41006=CARTESIAN_POINT ( 'NONE',  ( 4.458734124999998549, -103.7291666653010651, -2.574251347313721627 ) ) ;
#41009=CARTESIAN_POINT ( 'NONE',  ( 9.457646018065525792E-16, -100.3124999986344079, 5.148502694627439702 ) ) ;
#41010=CARTESIAN_POINT ( 'NONE',  ( -4.458734124999999437, -29.31249999863440436, 0.000000000000000000 ) ) ;
#41011=CARTESIAN_POINT ( 'NONE',  ( 5.000000000000000000, -64.37499999726881583, -6.123233995736766282E-16 ) ) ;
#41014=CARTESIAN_POINT ( 'NONE',  ( -4.458734124999999437, -23.39583333196773651, -2.574251347313719407 ) ) ;
#41015=CARTESIAN_POINT ( 'NONE',  ( -3.152548672688508926E-16, -63.81249999863440792, -5.148502694627439702 ) ) ;
#41020=CARTESIAN_POINT ( 'NONE',  ( 1.060575238724906964E-15, -11.74999999999999467, 5.773502691896257311 ) ) ;
#41025=CARTESIAN_POINT ( 'NONE',  ( 5.000000000000000000, -90.41666666666667140, -2.886751345948130876 ) ) ;
#41030=CARTESIAN_POINT ( 'NONE',  ( -2.500000000000000444, 25.83333333333333215, -4.330127018922193649 ) ) ;
#41037=CARTESIAN_POINT ( 'NONE',  ( 5.000000000000000000, -85.49999999999998579, -6.123233995736766282E-16 ) ) ;
#41042=ORIENTED_EDGE ( 'NONE', *, *, #11047, .T. ) ;
#41044=ORIENTED_EDGE ( 'NONE', *, *, #44341, .F. ) ;
#41045=CARTESIAN_POINT ( 'NONE',  ( 0.000000000000000000, -120.0000000000000000, 0.000000000000000000 ) ) ;
#41051=CARTESIAN_POINT ( 'NONE',  ( -1.339745962155613812, 22.91965820146970501, -5.000000000000000000 ) ) ;
#41054=CARTESIAN_POINT ( 'NONE',  ( -4.458734124999999437, -77.39583333196772230, -2.574251347313719407 ) ) ;
#41055=CARTESIAN_POINT ( 'NONE',  ( -4.458734124999999437, -109.5624999986343937, 0.000000000000000000 ) ) ;
#41058=CARTESIAN_POINT ( 'NONE',  ( 1.975475456537005874E-15, 5.375000002731185944, 5.000000000000000000 ) ) ;
#41062=DIRECTION ( 'NONE',  ( -0.000000000000000000, 1.000000000000000000, -0.000000000000000000 ) ) ;
#41064=CARTESIAN_POINT ( 'NONE',  ( 4.458734125000000326, -50.89583333196772230, 2.574251347313718519 ) ) ;
#41066=CARTESIAN_POINT ( 'NONE',  ( -2.229367062500000163, 29.52083333469892779, -3.861377020970580443 ) ) ;
#41067=CARTESIAN_POINT ( 'NONE',  ( 5.000000000000000000, -108.4999999999999858, -6.123233995736766282E-16 ) ) ;
#41068=CARTESIAN_POINT ( 'NONE',  ( 6.158835246850666199E-14, 9.749999999999996447, -4.999999999999999112 ) ) ;
#41069=CARTESIAN_POINT ( 'NONE',  ( 2.229367062500001939, -40.22916666530107221, 3.861377020970579999 ) ) ;
#41070=CARTESIAN_POINT ( 'NONE',  ( 1.060575238724906964E-15, -0.6249999972688138339, 5.773502691896257311 ) ) ;
#41074=CARTESIAN_POINT ( 'NONE',  ( 1.975475456537005874E-15, 6.249999999999998224, 5.000000000000000000 ) ) ;
#41075=CARTESIAN_POINT ( 'NONE',  ( -4.458734124999999437, -95.31249999863440792, 0.000000000000000000 ) ) ;
#41076=CARTESIAN_POINT ( 'NONE',  ( 1.975475456537005874E-15, -30.62499999726881583, 5.000000000000000000 ) ) ;
#41077=CARTESIAN_POINT ( 'NONE',  ( 4.458734125000000326, -1.145833331967740287, 2.574251347313718519 ) ) ;
#41080=CARTESIAN_POINT ( 'NONE',  ( 0.000000000000000000, -120.0000000000000000, 5.000000000000000000 ) ) ;
#41081=CARTESIAN_POINT ( 'NONE',  ( -4.458734124999998549, -85.22916666530107932, 2.574251347313722516 ) ) ;
#41082=CARTESIAN_POINT ( 'NONE',  ( 1.339745962155611592, 27.29465819873851729, 5.000000000000000888 ) ) ;
#41083=CARTESIAN_POINT ( 'NONE',  ( -2.229367062500000163, -84.72916666530107932, -3.861377020970580443 ) ) ;
#41085=CARTESIAN_POINT ( 'NONE',  ( -2.500000000000000444, -53.16666666666666430, -4.330127018922193649 ) ) ;
#41087=CARTESIAN_POINT ( 'NONE',  ( -4.458734124999997661, -8.229166665301073991, 2.574251347313722516 ) ) ;
#41088=CARTESIAN_POINT ( 'NONE',  ( -3.152548672688508926E-16, 17.18750000136559919, -5.148502694627439702 ) ) ;
#41089=CARTESIAN_POINT ( 'NONE',  ( 4.458734125000000326, -46.14583333196773651, 2.574251347313718519 ) ) ;
#41090=CARTESIAN_POINT ( 'NONE',  ( 5.000000000000000888, -11.58333333333333393, 2.886751345948126879 ) ) ;
#41097=CARTESIAN_POINT ( 'NONE',  ( 2.229367062500001939, -76.97916666530106511, 3.861377020970579999 ) ) ;
#41098=CARTESIAN_POINT ( 'NONE',  ( -2.499999999999996447, -109.7083333306021444, 4.330127018922195425 ) ) ;
#41105=CARTESIAN_POINT ( 'NONE',  ( -5.000000000000000000, -66.00000000000000000, 0.000000000000000000 ) ) ;
#41110=DIRECTION ( 'NONE',  ( -0.000000000000000000, 1.000000000000000000, -0.000000000000000000 ) ) ;
#41116=ORIENTED_EDGE ( 'NONE', *, *, #44419, .F. ) ;
#41118=CARTESIAN_POINT ( 'NONE',  ( -6.972266317189433020E-16, 10.87500000273118417, -5.000000000000000000 ) ) ;
#41120=EDGE_LOOP ( 'NONE', ( #46162, #30916, #39486, #63523 ) ) ;
#41123=CARTESIAN_POINT ( 'NONE',  ( 2.229367062499998831, -43.89583333196774362, -3.861377020970580887 ) ) ;
#41124=CARTESIAN_POINT ( 'NONE',  ( 5.000000000000000000, -34.50000000000000000, -6.123233995736766282E-16 ) ) ;
#41127=CARTESIAN_POINT ( 'NONE',  ( -5.000000000000000000, -81.87499999726881583, 0.000000000000000000 ) ) ;
#41128=AXIS2_PLACEMENT_3D ( 'NONE', #34771, #10636, #30249 ) ;
#41132=CARTESIAN_POINT ( 'NONE',  ( -5.000000000000000000, 0.9166666666666664076, -2.886751345948128211 ) ) ;
#41134=CARTESIAN_POINT ( 'NONE',  ( -2.229367062500000163, -93.72916666530106511, -3.861377020970580443 ) ) ;
#41136=ORIENTED_EDGE ( 'NONE', *, *, #11033, .T. ) ;
#41140=CARTESIAN_POINT ( 'NONE',  ( 5.000000000000000000, -60.50000000000000000, -6.123233995736766282E-16 ) ) ;
#41141=CARTESIAN_POINT ( 'NONE',  ( 4.458734124999999437, -3.812499998634408360, -5.460374474430324690E-16 ) ) ;
#41143=CARTESIAN_POINT ( 'NONE',  ( 4.458734125000001214, -24.14583333196773651, 2.574251347313718519 ) ) ;
#41150=( BOUNDED_CURVE ( )  B_SPLINE_CURVE ( 2, ( #42522, #24168, #47666, #9060, #52508, #3618, #27731, #3931, #58272 ),
 .UNSPECIFIED., .F., .F. ) 
 B_SPLINE_CURVE_WITH_KNOTS ( ( 3, 2, 2, 2, 3 ),
 ( 0.9553571428571429047, 0.9559523809523809978, 0.9571428571428571841, 0.9583333333333333703, 0.9589285714285714635 ),
 .UNSPECIFIED. ) 
 CURVE ( )  GEOMETRIC_REPRESENTATION_ITEM ( )  RATIONAL_B_SPLINE_CURVE ( ( 0.9330127018922194093, 0.9330127018922194093, 1.000000000000000000, 0.8660254037844387076, 1.000000000000000000, 0.8660254037844387076, 1.000000000000000000, 0.9330127018922194093, 0.9330127018922194093 ) ) 
 REPRESENTATION_ITEM ( '' )  );
#41151=CARTESIAN_POINT ( 'NONE',  ( 2.229367062499998831, 15.10416666803225993, -3.861377020970580887 ) ) ;
#41152=EDGE_LOOP ( 'NONE', ( #12944, #26121, #59236, #16825 ) ) ;
#41154=CARTESIAN_POINT ( 'NONE',  ( 5.000000000000000000, -87.41666666666667140, -2.886751345948129988 ) ) ;
#41155=CARTESIAN_POINT ( 'NONE',  ( 9.457646018065525792E-16, -18.06249999863440436, 5.148502694627439702 ) ) ;
#41157=DIRECTION ( 'NONE',  ( 0.000000000000000000, 0.000000000000000000, 1.000000000000000000 ) ) ;
#41160=CARTESIAN_POINT ( 'NONE',  ( -2.499999999999996447, -44.70833333060214443, 4.330127018922195425 ) ) ;
#41161=CARTESIAN_POINT ( 'NONE',  ( -6.972266317189433020E-16, -41.12499999726880162, -5.000000000000000000 ) ) ;
#41162=CARTESIAN_POINT ( 'NONE',  ( 4.458734125000000326, 9.104166668032261711, 2.574251347313718519 ) ) ;
#41163=CARTESIAN_POINT ( 'NONE',  ( 1.975475456537005874E-15, -62.62499999726880873, 5.000000000000000000 ) ) ;
#41165=CARTESIAN_POINT ( 'NONE',  ( 4.458734124999998549, -64.72916666530106511, -2.574251347313721627 ) ) ;
#41166=VECTOR ( 'NONE', #19720, 1000.000000000000000 ) ;
#41168=CARTESIAN_POINT ( 'NONE',  ( -4.999999999999999112, -2.916666666666664742, 2.886751345948131764 ) ) ;
#41172=CARTESIAN_POINT ( 'NONE',  ( -4.458734124999999437, -58.31249999863440081, 0.000000000000000000 ) ) ;
#41173=CARTESIAN_POINT ( 'NONE',  ( 5.000000000000000000, -97.29166666393547303, -2.886751345948129988 ) ) ;
#41175=CARTESIAN_POINT ( 'NONE',  ( -6.972266317189433020E-16, -56.25000000000000000, -5.000000000000000000 ) ) ;
#41177=LINE ( 'NONE', #60189, #59507 ) ;
#41178=( BOUNDED_CURVE ( )  B_SPLINE_CURVE ( 2, ( #2933, #8383, #62419, #2608, #47603, #22546, #32495, #12252, #42148 ),
 .UNSPECIFIED., .F., .F. ) 
 B_SPLINE_CURVE_WITH_KNOTS ( ( 3, 2, 2, 2, 3 ),
 ( 0.2553571428571428381, 0.2559523809523809312, 0.2571428571428571175, 0.2583333333333333592, 0.2589285714285714524 ),
 .UNSPECIFIED. ) 
 CURVE ( )  GEOMETRIC_REPRESENTATION_ITEM ( )  RATIONAL_B_SPLINE_CURVE ( ( 0.9330127018922194093, 0.9330127018922194093, 1.000000000000000000, 0.8660254037844387076, 1.000000000000000000, 0.8660254037844387076, 1.000000000000000000, 0.9330127018922194093, 0.9330127018922194093 ) ) 
 REPRESENTATION_ITEM ( '' )  );
#41179=CARTESIAN_POINT ( 'NONE',  ( 5.000000000000000888, -47.58333333333333570, 2.886751345948126879 ) ) ;
#41182=ORIENTED_EDGE ( 'NONE', *, *, #60184, .F. ) ;
#41183=CARTESIAN_POINT ( 'NONE',  ( 2.229367062500001939, -104.9791666653010651, 3.861377020970579999 ) ) ;
#41184=CARTESIAN_POINT ( 'NONE',  ( -4.458734124999998549, -1.479166665301071770, 2.574251347313722516 ) ) ;
#41191=ORIENTED_EDGE ( 'NONE', *, *, #36524, .F. ) ;
#41192=DIRECTION ( 'NONE',  ( 0.000000000000000000, 0.000000000000000000, 1.000000000000000000 ) ) ;
#41197=CARTESIAN_POINT ( 'NONE',  ( 4.458734124999998549, -30.97916666530107577, -2.574251347313721627 ) ) ;
#41206=CARTESIAN_POINT ( 'NONE',  ( 4.458734124999999437, -80.06249999863440792, -5.460374474430324690E-16 ) ) ;
#41208=ORIENTED_EDGE ( 'NONE', *, *, #1962, .T. ) ;
#41213=CARTESIAN_POINT ( 'NONE',  ( -4.458734124999999437, -11.64583333196773829, -2.574251347313719407 ) ) ;
#41216=CARTESIAN_POINT ( 'NONE',  ( -6.972266317189433020E-16, -93.12499999726881583, -5.000000000000000000 ) ) ;
#41217=ORIENTED_EDGE ( 'NONE', *, *, #32650, .T. ) ;
#41218=CARTESIAN_POINT ( 'NONE',  ( 4.458734124999998549, -7.979166665301073991, -2.574251347313721627 ) ) ;
#41223=ORIENTED_EDGE ( 'NONE', *, *, #33470, .F. ) ;
#41224=CARTESIAN_POINT ( 'NONE',  ( 2.229367062500001939, -84.97916666530107932, 3.861377020970579999 ) ) ;
#41226=CARTESIAN_POINT ( 'NONE',  ( 4.458734124999999437, -0.8124999986344055847, -5.460374474430324690E-16 ) ) ;
#41227=ADVANCED_FACE ( 'NONE', ( #330 ), #19616, .T. ) ;
#41229=CARTESIAN_POINT ( 'NONE',  ( 2.499999999999998668, -32.20833333060215153, -4.330127018922193649 ) ) ;
#41230=LINE ( 'NONE', #27090, #7806 ) ;
#41231=CARTESIAN_POINT ( 'NONE',  ( 2.229367062499998831, 23.35416666803225993, -3.861377020970580887 ) ) ;
#41232=CARTESIAN_POINT ( 'NONE',  ( -2.499999999999996447, 23.16666666666666430, 4.330127018922195425 ) ) ;
#41234=CARTESIAN_POINT ( 'NONE',  ( 9.457646018065525792E-16, -49.06249999863440792, 5.148502694627439702 ) ) ;
#41235=CARTESIAN_POINT ( 'NONE',  ( 2.229367062500001939, -35.22916666530107221, 3.861377020970579999 ) ) ;
#41237=CARTESIAN_POINT ( 'NONE',  ( 1.975475456537005874E-15, -17.75000000000000355, 5.000000000000000000 ) ) ;
#41238=CARTESIAN_POINT ( 'NONE',  ( -2.499999999999996447, 17.16666666666666430, 4.330127018922195425 ) ) ;
#41240=CARTESIAN_POINT ( 'NONE',  ( 1.339745962155557191, -26.58034179853029499, 5.000000000000032863 ) ) ;
#41242=CARTESIAN_POINT ( 'NONE',  ( -4.458734124999998549, -41.22916666530107221, 2.574251347313722516 ) ) ;
#41243=CARTESIAN_POINT ( 'NONE',  ( -5.000000000000000000, -78.87499999726881583, 0.000000000000000000 ) ) ;
#41245=CARTESIAN_POINT ( 'NONE',  ( -6.972266317189433020E-16, -93.24999999999998579, -5.000000000000000000 ) ) ;
#41246=DIRECTION ( 'NONE',  ( -0.000000000000000000, 1.000000000000000000, -0.000000000000000000 ) ) ;
#41248=CARTESIAN_POINT ( 'NONE',  ( 2.229367062500001939, -87.22916666530107932, 3.861377020970579999 ) ) ;
#41251=CARTESIAN_POINT ( 'NONE',  ( -4.999999999999999112, -30.91666666666666785, 2.886751345948131764 ) ) ;
#41255=VERTEX_POINT ( 'NONE', #25401 ) ;
#41256=CARTESIAN_POINT ( 'NONE',  ( -2.229367062500000163, -92.47916666530106511, -3.861377020970580443 ) ) ;
#41257=CARTESIAN_POINT ( 'NONE',  ( 2.229367062499998831, 14.10416666803226171, -3.861377020970580887 ) ) ;
#41258=CARTESIAN_POINT ( 'NONE',  ( 5.000000000000000000, 14.70833333606451987, -2.886751345948129988 ) ) ;
#41264=CARTESIAN_POINT ( 'NONE',  ( -1.339745962155610925, -51.79465819873851729, 5.000000000000000000 ) ) ;
#41265=CARTESIAN_POINT ( 'NONE',  ( 2.499999999999998668, -99.20833333060214443, -4.330127018922193649 ) ) ;
#41266=FACE_OUTER_BOUND ( 'NONE', #61062, .T. ) ;
#41267=CARTESIAN_POINT ( 'NONE',  ( -2.499999999999996447, -74.70833333060214443, 4.330127018922195425 ) ) ;
#41269=CARTESIAN_POINT ( 'NONE',  ( 2.499999999999998668, -107.3333333333333428, -4.330127018922193649 ) ) ;
#41270=LINE ( 'NONE', #61874, #3865 ) ;
#41271=CARTESIAN_POINT ( 'NONE',  ( -4.458734124999998549, -12.47916666530107221, 2.574251347313722516 ) ) ;
#41278=( BOUNDED_CURVE ( )  B_SPLINE_CURVE ( 2, ( #45075, #10656, #31230, #60837, #45718, #6804, #54735, #36380, #56010 ),
 .UNSPECIFIED., .F., .F. ) 
 B_SPLINE_CURVE_WITH_KNOTS ( ( 3, 2, 2, 2, 3 ),
 ( 0.3267857142857142905, 0.3273809523809523836, 0.3285714285714285698, 0.3297619047619047561, 0.3303571428571428492 ),
 .UNSPECIFIED. ) 
 CURVE ( )  GEOMETRIC_REPRESENTATION_ITEM ( )  RATIONAL_B_SPLINE_CURVE ( ( 0.9330127018922194093, 0.9330127018922194093, 1.000000000000000000, 0.8660254037844387076, 1.000000000000000000, 0.8660254037844387076, 1.000000000000000000, 0.9330127018922194093, 0.9330127018922194093 ) ) 
 REPRESENTATION_ITEM ( '' )  );
#41282=ORIENTED_EDGE ( 'NONE', *, *, #60517, .T. ) ;
#41283=CARTESIAN_POINT ( 'NONE',  ( -2.229367062499996610, -61.39583333196774362, 3.861377020970582219 ) ) ;
#41285=CARTESIAN_POINT ( 'NONE',  ( 5.000000000000000000, -8.416666666666669627, -2.886751345948130876 ) ) ;
#41294=( BOUNDED_CURVE ( )  B_SPLINE_CURVE ( 2, ( #40793, #30836, #302, #26014, #30179, #5433, #49495, #59475, #9928 ),
 .UNSPECIFIED., .F., .F. ) 
 B_SPLINE_CURVE_WITH_KNOTS ( ( 3, 2, 2, 2, 3 ),
 ( 0.6946428571428571175, 0.6952380952380952106, 0.6964285714285713969, 0.6976190476190475831, 0.6982142857142856762 ),
 .UNSPECIFIED. ) 
 CURVE ( )  GEOMETRIC_REPRESENTATION_ITEM ( )  RATIONAL_B_SPLINE_CURVE ( ( 0.9330127018922194093, 0.9330127018922194093, 1.000000000000000000, 0.8660254037844387076, 1.000000000000000000, 0.8660254037844387076, 1.000000000000000000, 0.9330127018922194093, 0.9330127018922194093 ) ) 
 REPRESENTATION_ITEM ( '' )  );
#41296=CARTESIAN_POINT ( 'NONE',  ( 4.458734124999999437, 10.18750000136559386, -5.460374474430324690E-16 ) ) ;
#41299=CARTESIAN_POINT ( 'NONE',  ( -5.000000000000000000, -23.87499999726881228, 0.000000000000000000 ) ) ;
#41302=CARTESIAN_POINT ( 'NONE',  ( -2.229367062499996610, -73.14583333196773651, 3.861377020970582219 ) ) ;
#41304=CARTESIAN_POINT ( 'NONE',  ( 4.458734125000001214, 10.10416666803226171, 2.574251347313718519 ) ) ;
#41307=CYLINDRICAL_SURFACE ( 'NONE', #51118, 5.000000000000000000 ) ;
#41309=CARTESIAN_POINT ( 'NONE',  ( -2.229367062500000163, -54.72916666530107221, -3.861377020970580443 ) ) ;
#41310=CARTESIAN_POINT ( 'NONE',  ( 5.000000000000000000, -13.29166666393548191, -2.886751345948129988 ) ) ;
#41311=CARTESIAN_POINT ( 'NONE',  ( 1.975475456537005874E-15, -99.74999999999998579, 5.000000000000000000 ) ) ;
#41312=DIRECTION ( 'NONE',  ( -0.000000000000000000, 1.000000000000000000, -0.000000000000000000 ) ) ;
#41314=CARTESIAN_POINT ( 'NONE',  ( -6.972266317189433020E-16, -65.24999999999998579, -5.000000000000000000 ) ) ;
#41315=CARTESIAN_POINT ( 'NONE',  ( 9.457646018065525792E-16, -19.31249999863440792, 5.148502694627439702 ) ) ;
#41317=DIRECTION ( 'NONE',  ( -0.5000000000000068834, 0.000000000000000000, -0.8660254037844345998 ) ) ;
#41318=CARTESIAN_POINT ( 'NONE',  ( 4.458734124999999437, -107.8124999986343937, -5.460374474430324690E-16 ) ) ;
#41321=CARTESIAN_POINT ( 'NONE',  ( 4.458734125000001214, -104.1458333319677365, 2.574251347313718519 ) ) ;
#41322=CARTESIAN_POINT ( 'NONE',  ( -3.152548672688508926E-16, -24.56249999863440792, -5.148502694627439702 ) ) ;
#41323=CARTESIAN_POINT ( 'NONE',  ( 2.499999999999998668, -61.20833333060214443, -4.330127018922193649 ) ) ;
#41324=EDGE_CURVE ( 'NONE', #942, #43496, #9013, .T. ) ;
#41327=CARTESIAN_POINT ( 'NONE',  ( -4.458734124999999437, -24.39583333196773651, -2.574251347313719407 ) ) ;
#41329=CARTESIAN_POINT ( 'NONE',  ( -2.229367062500000163, -68.72916666530107932, -3.861377020970580443 ) ) ;
#41330=DIRECTION ( 'NONE',  ( -0.000000000000000000, 1.000000000000000000, -0.000000000000000000 ) ) ;
#41333=CARTESIAN_POINT ( 'NONE',  ( -3.535250795749689387E-16, -10.25000000000000355, -5.773502691896257311 ) ) ;
#41342=LINE ( 'NONE', #56154, #13988 ) ;
#41346=LINE ( 'NONE', #51340, #36552 ) ;
#41352=( BOUNDED_CURVE ( )  B_SPLINE_CURVE ( 2, ( #62182, #8152, #41269, #51891, #57047, #60919, #17158, #7203, #27752 ),
 .UNSPECIFIED., .F., .F. ) 
 B_SPLINE_CURVE_WITH_KNOTS ( ( 3, 2, 2, 2, 3 ),
 ( 0.9803571428571428159, 0.9809523809523809090, 0.9821428571428570953, 0.9833333333333332815, 0.9839285714285714857 ),
 .UNSPECIFIED. ) 
 CURVE ( )  GEOMETRIC_REPRESENTATION_ITEM ( )  RATIONAL_B_SPLINE_CURVE ( ( 0.9330127018922194093, 0.9330127018922194093, 1.000000000000000000, 0.8660254037844387076, 1.000000000000000000, 0.8660254037844387076, 1.000000000000000000, 0.9330127018922130810, 0.9330127018922194093 ) ) 
 REPRESENTATION_ITEM ( '' )  );
#41353=CARTESIAN_POINT ( 'NONE',  ( 1.975475456537005874E-15, -50.75000000000000000, 5.000000000000000000 ) ) ;
#41357=ORIENTED_EDGE ( 'NONE', *, *, #5458, .F. ) ;
#41363=ORIENTED_EDGE ( 'NONE', *, *, #13304, .T. ) ;
#41368=CARTESIAN_POINT ( 'NONE',  ( -3.152548672688508926E-16, -78.56249999863440792, -5.148502694627439702 ) ) ;
#41369=CARTESIAN_POINT ( 'NONE',  ( -2.229367062499996610, 26.85416666803225993, 3.861377020970582219 ) ) ;
#41370=CARTESIAN_POINT ( 'NONE',  ( -1.339745962155610925, -53.79465819873851018, 5.000000000000000000 ) ) ;
#41371=EDGE_LOOP ( 'NONE', ( #54115, #32841, #30443, #45555 ) ) ;
#41378=( BOUNDED_CURVE ( )  B_SPLINE_CURVE ( 2, ( #21377, #36173, #55793, #1458, #21058, #46457, #26196, #21703, #35531 ),
 .UNSPECIFIED., .F., .F. ) 
 B_SPLINE_CURVE_WITH_KNOTS ( ( 3, 2, 2, 2, 3 ),
 ( 0.1303571428571428659, 0.1309523809523809590, 0.1321428571428571452, 0.1333333333333333315, 0.1339285714285714246 ),
 .UNSPECIFIED. ) 
 CURVE ( )  GEOMETRIC_REPRESENTATION_ITEM ( )  RATIONAL_B_SPLINE_CURVE ( ( 0.9330127018922194093, 0.9330127018922194093, 1.000000000000000000, 0.8660254037844387076, 1.000000000000000000, 0.8660254037844387076, 1.000000000000000000, 0.9330127018922194093, 0.9330127018922194093 ) ) 
 REPRESENTATION_ITEM ( '' )  );
#41380=CARTESIAN_POINT ( 'NONE',  ( -4.458734124999997661, -55.22916666530107932, 2.574251347313722516 ) ) ;
#41383=CARTESIAN_POINT ( 'NONE',  ( 1.060575238724906964E-15, -104.7500000000000142, 5.773502691896257311 ) ) ;
#41385=EDGE_CURVE ( 'NONE', #22249, #11403, #39580, .T. ) ;
#41386=CARTESIAN_POINT ( 'NONE',  ( -3.152548672688508926E-16, -36.81249999863440792, -5.148502694627439702 ) ) ;
#41387=CARTESIAN_POINT ( 'NONE',  ( -3.535250795749689387E-16, 0.8750000027311874984, -5.773502691896257311 ) ) ;
#41392=CARTESIAN_POINT ( 'NONE',  ( 4.458734124999999437, -95.81249999863440792, -5.460374474430324690E-16 ) ) ;
#41393=CARTESIAN_POINT ( 'NONE',  ( -2.229367062500000163, -6.729166665301073103, -3.861377020970580443 ) ) ;
#41394=ORIENTED_EDGE ( 'NONE', *, *, #60217, .F. ) ;
#41395=DIRECTION ( 'NONE',  ( -0.000000000000000000, 1.000000000000000000, -0.000000000000000000 ) ) ;
#41397=CARTESIAN_POINT ( 'NONE',  ( 9.457646018065525792E-16, -90.06249999863440792, 5.148502694627439702 ) ) ;
#41399=CARTESIAN_POINT ( 'NONE',  ( -2.229367062499996610, -84.39583333196773651, 3.861377020970582219 ) ) ;
#41403=CARTESIAN_POINT ( 'NONE',  ( 2.229367062500001939, -4.979166665301071326, 3.861377020970579999 ) ) ;
#41404=CARTESIAN_POINT ( 'NONE',  ( 4.458734125000001214, 15.85416666803226171, 2.574251347313718519 ) ) ;
#41405=CARTESIAN_POINT ( 'NONE',  ( -3.152548672688508926E-16, -47.81249999863440792, -5.148502694627439702 ) ) ;
#41409=CARTESIAN_POINT ( 'NONE',  ( -5.000000000000000000, -38.99999999999999289, 0.000000000000000000 ) ) ;
#41410=ADVANCED_FACE ( 'NONE', ( #27686 ), #47313, .T. ) ;
#41415=CARTESIAN_POINT ( 'NONE',  ( 4.458734125000001214, -77.89583333196773651, 2.574251347313718519 ) ) ;
#41416=CARTESIAN_POINT ( 'NONE',  ( -5.000000000000000000, -108.8749999972688016, 0.000000000000000000 ) ) ;
#41418=ADVANCED_FACE ( 'NONE', ( #30525 ), #29243, .T. ) ;
#41422=CARTESIAN_POINT ( 'NONE',  ( -3.535250795749689387E-16, -63.25000000000000000, -5.773502691896257311 ) ) ;
#41423=DIRECTION ( 'NONE',  ( -0.000000000000000000, 1.000000000000000000, -0.000000000000000000 ) ) ;
#41426=FACE_OUTER_BOUND ( 'NONE', #35213, .T. ) ;
#41437=VERTEX_POINT ( 'NONE', #29565 ) ;
#41440=CARTESIAN_POINT ( 'NONE',  ( -4.458734124999999437, -51.56249999863440792, 0.000000000000000000 ) ) ;
#41441=CARTESIAN_POINT ( 'NONE',  ( 1.975475456537005874E-15, -34.75000000000000000, 5.000000000000000000 ) ) ;
#41443=CARTESIAN_POINT ( 'NONE',  ( -2.500000000000000444, -82.04166666393547303, -4.330127018922193649 ) ) ;
#41447=CARTESIAN_POINT ( 'NONE',  ( -6.972266317189433020E-16, -50.12499999726881583, -5.000000000000000000 ) ) ;
#41449=CARTESIAN_POINT ( 'NONE',  ( -4.458734124999999437, -96.64583333196773651, -2.574251347313719407 ) ) ;
#41451=ORIENTED_EDGE ( 'NONE', *, *, #22380, .F. ) ;
#41452=LINE ( 'NONE', #46612, #56034 ) ;
#41456=CARTESIAN_POINT ( 'NONE',  ( -2.229367062499996610, -3.145833331967738733, 3.861377020970582219 ) ) ;
#41457=CARTESIAN_POINT ( 'NONE',  ( 4.458734124999998549, -92.97916666530106511, -2.574251347313721627 ) ) ;
#41458=EDGE_CURVE ( 'NONE', #27288, #49758, #44679, .T. ) ;
#41460=CARTESIAN_POINT ( 'NONE',  ( 2.229367062499998831, -24.89583333196773651, -3.861377020970580887 ) ) ;
#41461=CARTESIAN_POINT ( 'NONE',  ( 5.000000000000000000, -46.41666666666666430, -2.886751345948130876 ) ) ;
#41464=CARTESIAN_POINT ( 'NONE',  ( 6.123233995736766282E-16, -120.0000000000000000, -5.000000000000000000 ) ) ;
#41466=CARTESIAN_POINT ( 'NONE',  ( -3.152548672688508926E-16, 9.187500001365592084, -5.148502694627439702 ) ) ;
#41468=FACE_OUTER_BOUND ( 'NONE', #44120, .T. ) ;
#41470=CARTESIAN_POINT ( 'NONE',  ( 5.000000000000000888, -85.58333333333332860, 2.886751345948126879 ) ) ;
#41471=CARTESIAN_POINT ( 'NONE',  ( 2.229367062499998831, -20.64583333196774007, -3.861377020970580887 ) ) ;
#41476=CARTESIAN_POINT ( 'NONE',  ( 5.000000000000000888, -46.45833333060214443, 2.886751345948126879 ) ) ;
#41478=CARTESIAN_POINT ( 'NONE',  ( -4.458734124999999437, 8.687500001365595637, 0.000000000000000000 ) ) ;
#41482=CARTESIAN_POINT ( 'NONE',  ( 9.457646018065525792E-16, -66.06249999863440792, 5.148502694627439702 ) ) ;
#41484=CARTESIAN_POINT ( 'NONE',  ( 5.000000000000000000, -2.500000000000002220, -6.123233995736766282E-16 ) ) ;
#41487=CARTESIAN_POINT ( 'NONE',  ( -4.458734124999998549, -63.22916666530106511, 2.574251347313722516 ) ) ;
#41488=CARTESIAN_POINT ( 'NONE',  ( 2.499999999999998668, -94.20833333060213022, -4.330127018922193649 ) ) ;
#41489=CARTESIAN_POINT ( 'NONE',  ( -1.339745962155610925, -69.79465819873850307, 5.000000000000000000 ) ) ;
#41492=DIRECTION ( 'NONE',  ( -0.000000000000000000, 1.000000000000000000, -0.000000000000000000 ) ) ;
#41493=CARTESIAN_POINT ( 'NONE',  ( -3.535250795749689387E-16, -51.25000000000000000, -5.773502691896257311 ) ) ;
#41494=CARTESIAN_POINT ( 'NONE',  ( -1.339745962155614700, 27.20534180126147916, 4.999999999999999112 ) ) ;
#41496=EDGE_LOOP ( 'NONE', ( #2164, #42879, #29079, #58794 ) ) ;
#41497=CARTESIAN_POINT ( 'NONE',  ( -4.458734124999999437, -105.3958333319677365, -2.574251347313719407 ) ) ;
#41498=CARTESIAN_POINT ( 'NONE',  ( -4.458734124999999437, -2.645833331967737845, -2.574251347313719407 ) ) ;
#41499=CYLINDRICAL_SURFACE ( 'NONE', #3183, 5.000000000000000000 ) ;
#41502=CARTESIAN_POINT ( 'NONE',  ( -5.000000000000000000, -30.95833333060214443, -2.886751345948128211 ) ) ;
#41506=CARTESIAN_POINT ( 'NONE',  ( 1.339745962155612702, -81.29465819873850307, -5.000000000000000000 ) ) ;
#41508=ORIENTED_EDGE ( 'NONE', *, *, #56265, .T. ) ;
#41512=CARTESIAN_POINT ( 'NONE',  ( 2.229367062499998831, -30.89583333196773651, -3.861377020970580887 ) ) ;
#41521=CARTESIAN_POINT ( 'NONE',  ( 1.975475456537005874E-15, -24.74999999999999645, 5.000000000000000000 ) ) ;
#41522=CARTESIAN_POINT ( 'NONE',  ( 9.457646018065525792E-16, -79.31249999863439371, 5.148502694627439702 ) ) ;
#41524=( BOUNDED_CURVE ( )  B_SPLINE_CURVE ( 2, ( #13368, #45958, #42631, #21528, #41124, #52608, #21845, #23345, #41441 ),
 .UNSPECIFIED., .F., .F. ) 
 B_SPLINE_CURVE_WITH_KNOTS ( ( 3, 2, 2, 2, 3 ),
 ( 0.4589285714285714080, 0.4595238095238095011, 0.4607142857142856873, 0.4619047619047619291, 0.4625000000000000222 ),
 .UNSPECIFIED. ) 
 CURVE ( )  GEOMETRIC_REPRESENTATION_ITEM ( )  RATIONAL_B_SPLINE_CURVE ( ( 0.9330127018922194093, 0.9330127018922194093, 1.000000000000000000, 0.8660254037844387076, 1.000000000000000000, 0.8660254037844387076, 1.000000000000000000, 0.9330127018922194093, 0.9330127018922194093 ) ) 
 REPRESENTATION_ITEM ( '' )  );
#41527=( BOUNDED_CURVE ( )  B_SPLINE_CURVE ( 2, ( #41353, #25294, #36535, #10493, #30107, #45550, #49737, #40401, #11763 ),
 .UNSPECIFIED., .F., .F. ) 
 B_SPLINE_CURVE_WITH_KNOTS ( ( 3, 2, 2, 2, 3 ),
 ( 0.5767857142857142350, 0.5773809523809523281, 0.5785714285714286254, 0.5797619047619048116, 0.5803571428571429047 ),
 .UNSPECIFIED. ) 
 CURVE ( )  GEOMETRIC_REPRESENTATION_ITEM ( )  RATIONAL_B_SPLINE_CURVE ( ( 0.9330127018922194093, 0.9330127018922194093, 1.000000000000000000, 0.8660254037844387076, 1.000000000000000000, 0.8660254037844387076, 1.000000000000000000, 0.9330127018922194093, 0.9330127018922194093 ) ) 
 REPRESENTATION_ITEM ( '' )  );
#41530=CARTESIAN_POINT ( 'NONE',  ( 2.229367062499998831, -8.895833331967736513, -3.861377020970580887 ) ) ;
#41532=CARTESIAN_POINT ( 'NONE',  ( 1.975475456537005874E-15, 17.25000000000000000, 5.000000000000000000 ) ) ;
#41533=CARTESIAN_POINT ( 'NONE',  ( 4.458734124999999437, -5.062499998634402587, -5.460374474430324690E-16 ) ) ;
#41540=CARTESIAN_POINT ( 'NONE',  ( 9.457646018065525792E-16, -85.06249999863440792, 5.148502694627439702 ) ) ;
#41541=CARTESIAN_POINT ( 'NONE',  ( -1.339745962155610925, -77.79465819873853150, 5.000000000000000000 ) ) ;
#41542=CARTESIAN_POINT ( 'NONE',  ( 2.229367062500001939, -0.9791666653010712151, 3.861377020970579999 ) ) ;
#41543=CARTESIAN_POINT ( 'NONE',  ( 0.000000000000000000, -120.0000000000000000, 0.000000000000000000 ) ) ;
#41545=CARTESIAN_POINT ( 'NONE',  ( 2.500000000000002220, -28.54166666393548013, 4.330127018922192761 ) ) ;
#41546=PLANE ( 'NONE',  #910 ) ;
#41547=CARTESIAN_POINT ( 'NONE',  ( 4.458734125000000326, 25.10416666803225993, 2.574251347313718519 ) ) ;
#41548=CARTESIAN_POINT ( 'NONE',  ( 0.000000000000000000, -120.0000000000000000, 0.000000000000000000 ) ) ;
#41550=CARTESIAN_POINT ( 'NONE',  ( -4.458734124999998549, -49.22916666530106511, 2.574251347313722516 ) ) ;
#41551=CARTESIAN_POINT ( 'NONE',  ( 4.458734125000000326, -36.14583333196773651, 2.574251347313718519 ) ) ;
#41553=CARTESIAN_POINT ( 'NONE',  ( -5.000000000000000000, 9.041666669397853795, -2.886751345948128211 ) ) ;
#41554=CARTESIAN_POINT ( 'NONE',  ( -3.535250795749689387E-16, 17.75000000000000355, -5.773502691896257311 ) ) ;
#41557=CARTESIAN_POINT ( 'NONE',  ( 4.458734124999998549, -41.72916666530107932, -2.574251347313721627 ) ) ;
#41558=CARTESIAN_POINT ( 'NONE',  ( 2.500000000000002220, -76.54166666393547303, 4.330127018922192761 ) ) ;
#41560=CARTESIAN_POINT ( 'NONE',  ( 2.500000000000002220, -65.54166666393547303, 4.330127018922192761 ) ) ;
#41562=CARTESIAN_POINT ( 'NONE',  ( -3.152548672688508926E-16, -83.81249999863437949, -5.148502694627439702 ) ) ;
#41564=CARTESIAN_POINT ( 'NONE',  ( 1.339745962155612702, 9.830341803992665106, -5.000000000000000000 ) ) ;
#41565=CARTESIAN_POINT ( 'NONE',  ( 2.500000000000002220, -34.66666666666666430, 4.330127018922192761 ) ) ;
#41570=CARTESIAN_POINT ( 'NONE',  ( -4.458734124999999437, -91.31249999863440792, 0.000000000000000000 ) ) ;
#41571=CARTESIAN_POINT ( 'NONE',  ( 2.229367062499998831, 11.10416666803225993, -3.861377020970580887 ) ) ;
#41572=CARTESIAN_POINT ( 'NONE',  ( 2.499999999999998668, 17.79166666939785557, -4.330127018922193649 ) ) ;
#41574=CARTESIAN_POINT ( 'NONE',  ( -6.972266317189433020E-16, -17.12499999726881583, -5.000000000000000000 ) ) ;
#41578=CARTESIAN_POINT ( 'NONE',  ( -2.500000000000000444, -52.16666666666666430, -4.330127018922193649 ) ) ;
#41580=CARTESIAN_POINT ( 'NONE',  ( 6.158835246850667461E-14, -1.250000000000002442, -4.999999999999999112 ) ) ;
#41585=CARTESIAN_POINT ( 'NONE',  ( -3.152548672688508926E-16, -16.81249999863440436, -5.148502694627439702 ) ) ;
#41590=EDGE_CURVE ( 'NONE', #31117, #19049, #54817, .T. ) ;
#41597=CARTESIAN_POINT ( 'NONE',  ( 4.458734124999998549, -62.97916666530107221, -2.574251347313721627 ) ) ;
#41600=ORIENTED_EDGE ( 'NONE', *, *, #41762, .F. ) ;
#41608=CARTESIAN_POINT ( 'NONE',  ( 4.458734124999998549, 9.270833334698927786, -2.574251347313721627 ) ) ;
#41611=CARTESIAN_POINT ( 'NONE',  ( -4.999999999999998224, -23.79166666393548368, 2.886751345948131764 ) ) ;
#41614=CARTESIAN_POINT ( 'NONE',  ( 9.457646018065525792E-16, -71.06249999863439371, 5.148502694627439702 ) ) ;
#41616=CARTESIAN_POINT ( 'NONE',  ( -4.458734124999998549, 11.77083333469892601, 2.574251347313722516 ) ) ;
#41617=ADVANCED_FACE ( 'NONE', ( #20578 ), #24752, .T. ) ;
#41619=CARTESIAN_POINT ( 'NONE',  ( -2.229367062500000163, -53.72916666530107221, -3.861377020970580443 ) ) ;
#41620=CARTESIAN_POINT ( 'NONE',  ( 1.060575238724906964E-15, -14.62499999726881228, 5.773502691896257311 ) ) ;
#41621=DIRECTION ( 'NONE',  ( -0.000000000000000000, 1.000000000000000000, -0.000000000000000000 ) ) ;
#41623=CARTESIAN_POINT ( 'NONE',  ( 9.457646018065525792E-16, -21.31249999863440081, 5.148502694627439702 ) ) ;
#41624=ORIENTED_EDGE ( 'NONE', *, *, #61814, .F. ) ;
#41626=CARTESIAN_POINT ( 'NONE',  ( -2.500000000000000444, 28.83333333333333215, -4.330127018922193649 ) ) ;
#41629=CARTESIAN_POINT ( 'NONE',  ( -4.458734124999998549, -100.4791666653010509, 2.574251347313722516 ) ) ;
#41630=CARTESIAN_POINT ( 'NONE',  ( 4.458734124999999437, -26.81249999863440081, -5.460374474430324690E-16 ) ) ;
#41631=CARTESIAN_POINT ( 'NONE',  ( 5.000000000000000000, -65.37499999726881583, -6.123233995736766282E-16 ) ) ;
#41632=CIRCLE ( 'NONE', #63228, 5.000000000000000000 ) ;
#41636=CARTESIAN_POINT ( 'NONE',  ( 4.458734124999999437, -25.81249999863440792, -5.460374474430324690E-16 ) ) ;
#41637=CARTESIAN_POINT ( 'NONE',  ( 9.457646018065525792E-16, -70.31249999863439371, 5.148502694627439702 ) ) ;
#41638=FACE_OUTER_BOUND ( 'NONE', #628, .T. ) ;
#41642=CARTESIAN_POINT ( 'NONE',  ( -3.535250795749689387E-16, -19.24999999999999645, -5.773502691896257311 ) ) ;
#41645=DIRECTION ( 'NONE',  ( -0.000000000000000000, 1.000000000000000000, -0.000000000000000000 ) ) ;
#41647=CARTESIAN_POINT ( 'NONE',  ( -5.000000000000000000, -86.95833333060214443, -2.886751345948128211 ) ) ;
#41650=( BOUNDED_CURVE ( )  B_SPLINE_CURVE ( 2, ( #60916, #31631, #31301, #16836, #1115, #26809, #46429, #31946, #51576 ),
 .UNSPECIFIED., .F., .F. ) 
 B_SPLINE_CURVE_WITH_KNOTS ( ( 3, 2, 2, 2, 3 ),
 ( 0.4446428571428571175, 0.4452380952380952106, 0.4464285714285714524, 0.4476190476190476386, 0.4482142857142857317 ),
 .UNSPECIFIED. ) 
 CURVE ( )  GEOMETRIC_REPRESENTATION_ITEM ( )  RATIONAL_B_SPLINE_CURVE ( ( 0.9330127018922194093, 0.9330127018922194093, 1.000000000000000000, 0.8660254037844387076, 1.000000000000000000, 0.8660254037844387076, 1.000000000000000000, 0.9330127018922194093, 0.9330127018922194093 ) ) 
 REPRESENTATION_ITEM ( '' )  );
#41651=CARTESIAN_POINT ( 'NONE',  ( 0.000000000000000000, -120.0000000000000000, 5.000000000000000000 ) ) ;
#41654=DIRECTION ( 'NONE',  ( -0.000000000000000000, 1.000000000000000000, -0.000000000000000000 ) ) ;
#41655=CARTESIAN_POINT ( 'NONE',  ( 5.000000000000000000, -87.29166666393547303, -2.886751345948130876 ) ) ;
#41658=ORIENTED_EDGE ( 'NONE', *, *, #55511, .T. ) ;
#41659=CARTESIAN_POINT ( 'NONE',  ( -5.000000000000000000, -29.95833333060214443, -2.886751345948128211 ) ) ;
#41660=ORIENTED_EDGE ( 'NONE', *, *, #42264, .F. ) ;
#41664=EDGE_CURVE ( 'NONE', #3938, #14927, #2247, .T. ) ;
#41665=( BOUNDED_CURVE ( )  B_SPLINE_CURVE ( 2, ( #32082, #23398, #13728, #47511, #47207, #57806, #51719, #17924, #62320 ),
 .UNSPECIFIED., .F., .F. ) 
 B_SPLINE_CURVE_WITH_KNOTS ( ( 3, 2, 2, 2, 3 ),
 ( 0.7017857142857142350, 0.7023809523809523281, 0.7035714285714286254, 0.7047619047619048116, 0.7053571428571429047 ),
 .UNSPECIFIED. ) 
 CURVE ( )  GEOMETRIC_REPRESENTATION_ITEM ( )  RATIONAL_B_SPLINE_CURVE ( ( 0.9330127018922194093, 0.9330127018922194093, 1.000000000000000000, 0.8660254037844387076, 1.000000000000000000, 0.8660254037844387076, 1.000000000000000000, 0.9330127018922194093, 0.9330127018922194093 ) ) 
 REPRESENTATION_ITEM ( '' )  );
#41668=EDGE_CURVE ( 'NONE', #60851, #57423, #8791, .T. ) ;
#41671=VERTEX_POINT ( 'NONE', #30853 ) ;
#41675=ORIENTED_EDGE ( 'NONE', *, *, #33067, .T. ) ;
#41679=ADVANCED_FACE ( 'NONE', ( #11549 ), #21847, .T. ) ;
#41681=VECTOR ( 'NONE', #60486, 1000.000000000000000 ) ;
#41683=CARTESIAN_POINT ( 'NONE',  ( 9.457646018065525792E-16, -79.06249999863440792, 5.148502694627439702 ) ) ;
#41685=CARTESIAN_POINT ( 'NONE',  ( 2.229367062499998831, 23.35416666803225993, -3.861377020970580887 ) ) ;
#41687=VERTEX_POINT ( 'NONE', #46285 ) ;
#41693=CARTESIAN_POINT ( 'NONE',  ( -1.339745962155613812, -83.20534180126146850, -5.000000000000000000 ) ) ;
#41694=CARTESIAN_POINT ( 'NONE',  ( -3.152548672688508926E-16, -54.56249999863439371, -5.148502694627439702 ) ) ;
#41697=CARTESIAN_POINT ( 'NONE',  ( -2.499999999999996447, -108.8333333333333428, 4.330127018922195425 ) ) ;
#41699=CARTESIAN_POINT ( 'NONE',  ( -2.229367062499996610, -40.39583333196773651, 3.861377020970582219 ) ) ;
#41700=CARTESIAN_POINT ( 'NONE',  ( -2.500000000000000444, 1.958333336064519647, -4.330127018922193649 ) ) ;
#41705=CARTESIAN_POINT ( 'NONE',  ( -4.458734124999997661, -102.2291666653010793, 2.574251347313722516 ) ) ;
#41706=CARTESIAN_POINT ( 'NONE',  ( 4.458734124999999437, -8.062499998634404363, -5.460374474430324690E-16 ) ) ;
#41708=CARTESIAN_POINT ( 'NONE',  ( -2.500000000000000444, -36.04166666393547303, -4.330127018922193649 ) ) ;
#41709=CARTESIAN_POINT ( 'NONE',  ( 4.458734125000001214, -92.89583333196775072, 2.574251347313718519 ) ) ;
#41710=CARTESIAN_POINT ( 'NONE',  ( -1.336351044127974539E-14, 23.24999999999999645, 5.000000000000000000 ) ) ;
#41711=CARTESIAN_POINT ( 'NONE',  ( -3.152548672688508926E-16, -84.81249999863439371, -5.148502694627439702 ) ) ;
#41713=DIRECTION ( 'NONE',  ( -0.000000000000000000, 1.000000000000000000, -0.000000000000000000 ) ) ;
#41715=CARTESIAN_POINT ( 'NONE',  ( 2.229367062500001939, -6.979166665301073103, 3.861377020970579999 ) ) ;
#41716=CARTESIAN_POINT ( 'NONE',  ( -2.229367062499996610, 18.60416666803225993, 3.861377020970582219 ) ) ;
#41717=CARTESIAN_POINT ( 'NONE',  ( 4.458734124999998549, -51.97916666530107221, -2.574251347313721627 ) ) ;
#41719=CARTESIAN_POINT ( 'NONE',  ( -5.000000000000000000, -37.08333333333332860, -2.886751345948128211 ) ) ;
#41727=CARTESIAN_POINT ( 'NONE',  ( -3.152548672688508926E-16, -82.56249999863442213, -5.148502694627439702 ) ) ;
#41728=CARTESIAN_POINT ( 'NONE',  ( -2.229367062500000163, 26.27083333469892779, -3.861377020970580443 ) ) ;
#41735=CARTESIAN_POINT ( 'NONE',  ( 5.000000000000000000, -66.41666666666667140, -2.886751345948129988 ) ) ;
#41739=DIRECTION ( 'NONE',  ( 0.000000000000000000, 0.000000000000000000, 1.000000000000000000 ) ) ;
#41740=CARTESIAN_POINT ( 'NONE',  ( -1.339745962155585168, 8.794658198738517285, -5.000000000000015987 ) ) ;
#41748=ORIENTED_EDGE ( 'NONE', *, *, #12644, .F. ) ;
#41754=CARTESIAN_POINT ( 'NONE',  ( 2.229367062500001939, -50.22916666530107221, 3.861377020970579999 ) ) ;
#41762=EDGE_CURVE ( 'NONE', #11950, #62422, #5214, .T. ) ;
#41764=CARTESIAN_POINT ( 'NONE',  ( -1.339745962155613812, 0.7946581987385198387, -5.000000000000000000 ) ) ;
#41766=CARTESIAN_POINT ( 'NONE',  ( 9.457646018065525792E-16, -102.3124999986344221, 5.148502694627439702 ) ) ;
#41767=CYLINDRICAL_SURFACE ( 'NONE', #25570, 5.000000000000000000 ) ;
#41768=ORIENTED_EDGE ( 'NONE', *, *, #22758, .F. ) ;
#41769=EDGE_CURVE ( 'NONE', #47799, #55067, #53674, .T. ) ;
#41775=VECTOR ( 'NONE', #60363, 1000.000000000000000 ) ;
#41776=CARTESIAN_POINT ( 'NONE',  ( -2.229367062499996610, -5.145833331967740065, 3.861377020970582219 ) ) ;
#41777=CARTESIAN_POINT ( 'NONE',  ( 4.458734124999999437, -98.06249999863440792, -5.460374474430324690E-16 ) ) ;
#41780=CARTESIAN_POINT ( 'NONE',  ( -4.458734124999999437, -20.56249999863440081, 0.000000000000000000 ) ) ;
#41781=AXIS2_PLACEMENT_3D ( 'NONE', #55350, #40221, #16097 ) ;
#41782=CARTESIAN_POINT ( 'NONE',  ( -6.972266317189433020E-16, -67.25000000000000000, -5.000000000000000000 ) ) ;
#41788=CARTESIAN_POINT ( 'NONE',  ( -4.458734124999997661, 11.52083333469892423, 2.574251347313722516 ) ) ;
#41792=CARTESIAN_POINT ( 'NONE',  ( 2.499999999999998668, -91.33333333333334281, -4.330127018922193649 ) ) ;
#41793=CARTESIAN_POINT ( 'NONE',  ( -4.458734124999998549, -24.22916666530107577, 2.574251347313722516 ) ) ;
#41795=CARTESIAN_POINT ( 'NONE',  ( 2.229367062499998831, -68.89583333196773651, -3.861377020970580887 ) ) ;
#41799=CARTESIAN_POINT ( 'NONE',  ( 2.499999999999998668, -52.20833333060213732, -4.330127018922193649 ) ) ;
#41801=CARTESIAN_POINT ( 'NONE',  ( -4.458734124999997661, 10.77083333469892956, 2.574251347313722516 ) ) ;
#41805=CARTESIAN_POINT ( 'NONE',  ( -4.458734124999999437, -71.39583333196773651, -2.574251347313719407 ) ) ;
#41807=CARTESIAN_POINT ( 'NONE',  ( 2.500000000000002220, 1.333333333333332149, 4.330127018922192761 ) ) ;
#41809=CARTESIAN_POINT ( 'NONE',  ( 9.457646018065525792E-16, -66.06249999863440792, 5.148502694627439702 ) ) ;
#41810=CARTESIAN_POINT ( 'NONE',  ( 5.000000000000000000, -93.29166666393547303, -2.886751345948129988 ) ) ;
#41811=CARTESIAN_POINT ( 'NONE',  ( 2.499999999999998668, 5.791666669397853795, -4.330127018922193649 ) ) ;
#41815=CARTESIAN_POINT ( 'NONE',  ( -2.500000000000000444, -50.16666666666666430, -4.330127018922193649 ) ) ;
#41816=CARTESIAN_POINT ( 'NONE',  ( 5.000000000000000888, -72.45833333060213022, 2.886751345948126879 ) ) ;
#41818=EDGE_LOOP ( 'NONE', ( #1197, #39935, #42920, #9555 ) ) ;
#41821=CARTESIAN_POINT ( 'NONE',  ( 0.000000000000000000, -120.0000000000000000, 0.000000000000000000 ) ) ;
#41823=VECTOR ( 'NONE', #4922, 1000.000000000000000 ) ;
#41826=CARTESIAN_POINT ( 'NONE',  ( -1.339745962155613812, -5.080341798530291442, -5.000000000000000000 ) ) ;
#41831=CYLINDRICAL_SURFACE ( 'NONE', #45652, 5.000000000000000000 ) ;
#41836=CARTESIAN_POINT ( 'NONE',  ( 4.458734125000001214, -34.14583333196772941, 2.574251347313718519 ) ) ;
#41837=CARTESIAN_POINT ( 'NONE',  ( 5.000000000000000000, -10.41666666666666607, -2.886751345948130876 ) ) ;
#41845=CARTESIAN_POINT ( 'NONE',  ( -4.458734124999998549, -85.47916666530106511, 2.574251347313722516 ) ) ;
#41847=ORIENTED_EDGE ( 'NONE', *, *, #37762, .T. ) ;
#41851=CARTESIAN_POINT ( 'NONE',  ( -2.229367062500000163, -7.729166665301073991, -3.861377020970580443 ) ) ;
#41854=( BOUNDED_CURVE ( )  B_SPLINE_CURVE ( 2, ( #49213, #38598, #47943, #29258, #13549, #4213, #24771, #14158, #57621 ),
 .UNSPECIFIED., .F., .F. ) 
 B_SPLINE_CURVE_WITH_KNOTS ( ( 3, 2, 2, 2, 3 ),
 ( 0.3125000000000000000, 0.3130952380952380931, 0.3142857142857142794, 0.3154761904761904656, 0.3160714285714285587 ),
 .UNSPECIFIED. ) 
 CURVE ( )  GEOMETRIC_REPRESENTATION_ITEM ( )  RATIONAL_B_SPLINE_CURVE ( ( 0.9330127018922194093, 0.9330127018922194093, 1.000000000000000000, 0.8660254037844387076, 1.000000000000000000, 0.8660254037844387076, 1.000000000000000000, 0.9330127018922194093, 0.9330127018922194093 ) ) 
 REPRESENTATION_ITEM ( '' )  );
#41856=FACE_OUTER_BOUND ( 'NONE', #16823, .T. ) ;
#41857=CARTESIAN_POINT ( 'NONE',  ( 9.457646018065525792E-16, -9.312499998634406140, 5.148502694627439702 ) ) ;
#41858=CYLINDRICAL_SURFACE ( 'NONE', #19922, 5.000000000000000000 ) ;
#41860=CARTESIAN_POINT ( 'NONE',  ( 1.975475456537005874E-15, -64.74999999999998579, 5.000000000000000000 ) ) ;
#41862=AXIS2_PLACEMENT_3D ( 'NONE', #53795, #24855, #45424 ) ;
#41863=CARTESIAN_POINT ( 'NONE',  ( 9.457646018065525792E-16, 25.68750000136559208, 5.148502694627439702 ) ) ;
#41864=VERTEX_POINT ( 'NONE', #62669 ) ;
#41865=CARTESIAN_POINT ( 'NONE',  ( 2.229367062499998831, -85.64583333196773651, -3.861377020970580887 ) ) ;
#41866=CARTESIAN_POINT ( 'NONE',  ( -4.999999999999998224, -77.91666666666665719, 2.886751345948131764 ) ) ;
#41867=CARTESIAN_POINT ( 'NONE',  ( -4.458734124999999437, -10.39583333196773829, -2.574251347313719407 ) ) ;
#41869=DIRECTION ( 'NONE',  ( -0.000000000000000000, 1.000000000000000000, -0.000000000000000000 ) ) ;
#41870=CARTESIAN_POINT ( 'NONE',  ( 0.000000000000000000, -120.0000000000000000, 0.000000000000000000 ) ) ;
#41871=CARTESIAN_POINT ( 'NONE',  ( -2.500000000000000444, -34.04166666393547303, -4.330127018922193649 ) ) ;
#41873=CARTESIAN_POINT ( 'NONE',  ( -4.458734124999997661, 22.77083333469892068, 2.574251347313722516 ) ) ;
#41874=FACE_OUTER_BOUND ( 'NONE', #37749, .T. ) ;
#41876=CARTESIAN_POINT ( 'NONE',  ( -4.458734124999999437, -50.39583333196773651, -2.574251347313719407 ) ) ;
#41878=CARTESIAN_POINT ( 'NONE',  ( -2.500000000000000444, 8.958333336064518093, -4.330127018922193649 ) ) ;
#41879=CARTESIAN_POINT ( 'NONE',  ( -3.535250795749689387E-16, 12.75000000000000000, -5.773502691896257311 ) ) ;
#41882=CARTESIAN_POINT ( 'NONE',  ( 4.458734124999999437, -47.81249999863440792, -5.460374474430324690E-16 ) ) ;
#41883=CARTESIAN_POINT ( 'NONE',  ( 5.000000000000000000, -81.29166666393547303, -2.886751345948129988 ) ) ;
#41886=CARTESIAN_POINT ( 'NONE',  ( 1.975475456537005874E-15, -27.74999999999999645, 5.000000000000000000 ) ) ;
#41887=VECTOR ( 'NONE', #2322, 1000.000000000000000 ) ;
#41888=CARTESIAN_POINT ( 'NONE',  ( 4.458734125000000326, -84.14583333196773651, 2.574251347313718519 ) ) ;
#41890=CARTESIAN_POINT ( 'NONE',  ( 5.000000000000000000, -31.50000000000000000, -6.123233995736766282E-16 ) ) ;
#41892=VERTEX_POINT ( 'NONE', #18589 ) ;
#41895=CARTESIAN_POINT ( 'NONE',  ( -4.458734124999999437, -92.31249999863440792, 0.000000000000000000 ) ) ;
#41896=CARTESIAN_POINT ( 'NONE',  ( -4.458734124999998549, 14.52083333469892779, 2.574251347313722516 ) ) ;
#41897=CARTESIAN_POINT ( 'NONE',  ( 5.000000000000000000, 15.70833333606451809, -2.886751345948129988 ) ) ;
#41901=CARTESIAN_POINT ( 'NONE',  ( -5.000000000000000000, -39.99999999999999289, 0.000000000000000000 ) ) ;
#41902=CARTESIAN_POINT ( 'NONE',  ( -3.535250795749689387E-16, -82.25000000000000000, -5.773502691896257311 ) ) ;
#41905=CARTESIAN_POINT ( 'NONE',  ( -5.000000000000000000, -12.95833333060214798, -2.886751345948128211 ) ) ;
#41906=CARTESIAN_POINT ( 'NONE',  ( 5.000000000000000888, -109.5833333333333428, 2.886751345948126879 ) ) ;
#41910=( BOUNDED_CURVE ( )  B_SPLINE_CURVE ( 2, ( #37191, #8236, #57757, #48083, #47770, #27838, #17572, #47460, #23346 ),
 .UNSPECIFIED., .F., .F. ) 
 B_SPLINE_CURVE_WITH_KNOTS ( ( 3, 2, 2, 2, 3 ),
 ( 0.5946428571428571397, 0.5952380952380952328, 0.5964285714285714191, 0.5976190476190476053, 0.5982142857142856984 ),
 .UNSPECIFIED. ) 
 CURVE ( )  GEOMETRIC_REPRESENTATION_ITEM ( )  RATIONAL_B_SPLINE_CURVE ( ( 0.9330127018922194093, 0.9330127018922194093, 1.000000000000000000, 0.8660254037844387076, 1.000000000000000000, 0.8660254037844387076, 1.000000000000000000, 0.9330127018922194093, 0.9330127018922194093 ) ) 
 REPRESENTATION_ITEM ( '' )  );
#41911=CARTESIAN_POINT ( 'NONE',  ( 2.229367062500001939, -18.22916666530106866, 3.861377020970579999 ) ) ;
#41917=AXIS2_PLACEMENT_3D ( 'NONE', #60503, #37871, #16745 ) ;
#41921=ORIENTED_EDGE ( 'NONE', *, *, #17799, .T. ) ;
#41923=ORIENTED_EDGE ( 'NONE', *, *, #51925, .T. ) ;
#41924=CARTESIAN_POINT ( 'NONE',  ( -2.229367062500000163, -62.72916666530106511, -3.861377020970580443 ) ) ;
#41925=CARTESIAN_POINT ( 'NONE',  ( 2.499999999999998668, -7.208333330602150646, -4.330127018922193649 ) ) ;
#41928=VERTEX_POINT ( 'NONE', #43335 ) ;
#41929=CARTESIAN_POINT ( 'NONE',  ( -2.500000000000000444, 26.95833333606451632, -4.330127018922193649 ) ) ;
#41933=EDGE_LOOP ( 'NONE', ( #27827, #27245, #40779, #12039 ) ) ;
#41935=CYLINDRICAL_SURFACE ( 'NONE', #47069, 5.000000000000000000 ) ;
#41936=CARTESIAN_POINT ( 'NONE',  ( 4.458734124999998549, 8.270833334698926009, -2.574251347313721627 ) ) ;
#41939=CARTESIAN_POINT ( 'NONE',  ( 2.499999999999998668, -77.33333333333334281, -4.330127018922193649 ) ) ;
#41942=CARTESIAN_POINT ( 'NONE',  ( -3.152548672688508926E-16, -69.56249999863439371, -5.148502694627439702 ) ) ;
#41943=CARTESIAN_POINT ( 'NONE',  ( 4.458734124999999437, 6.187500001365593860, -5.460374474430324690E-16 ) ) ;
#41945=CARTESIAN_POINT ( 'NONE',  ( -3.152548672688508926E-16, -60.81249999863440081, -5.148502694627439702 ) ) ;
#41946=CARTESIAN_POINT ( 'NONE',  ( -5.000000000000000000, -16.87499999726881583, 0.000000000000000000 ) ) ;
#41947=CARTESIAN_POINT ( 'NONE',  ( -1.339745962155610925, -99.79465819873853150, 5.000000000000000000 ) ) ;
#41948=CARTESIAN_POINT ( 'NONE',  ( -2.500000000000000444, -45.04166666393547303, -4.330127018922193649 ) ) ;
#41950=CARTESIAN_POINT ( 'NONE',  ( -3.152548672688508926E-16, -33.56249999863440792, -5.148502694627439702 ) ) ;
#41951=CARTESIAN_POINT ( 'NONE',  ( 4.458734124999999437, -24.06249999863440436, -5.460374474430324690E-16 ) ) ;
#41955=CARTESIAN_POINT ( 'NONE',  ( -2.229367062499996610, -107.1458333319677365, 3.861377020970582219 ) ) ;
#41957=EDGE_LOOP ( 'NONE', ( #2601, #8163, #13263, #2766 ) ) ;
#41958=CARTESIAN_POINT ( 'NONE',  ( 4.458734124999998549, -100.9791666653010509, -2.574251347313721627 ) ) ;
#41961=CARTESIAN_POINT ( 'NONE',  ( -4.458734124999998549, -33.22916666530107221, 2.574251347313722516 ) ) ;
#41962=CARTESIAN_POINT ( 'NONE',  ( 5.000000000000000888, -62.45833333060214443, 2.886751345948126879 ) ) ;
#41965=CARTESIAN_POINT ( 'NONE',  ( -4.458734124999999437, -31.39583333196773296, -2.574251347313719407 ) ) ;
#41966=CARTESIAN_POINT ( 'NONE',  ( -4.458734124999997661, -70.47916666530107932, 2.574251347313722516 ) ) ;
#41967=DIRECTION ( 'NONE',  ( -0.000000000000000000, 1.000000000000000000, -0.000000000000000000 ) ) ;
#41971=CARTESIAN_POINT ( 'NONE',  ( -5.000000000000000000, -17.00000000000000000, 0.000000000000000000 ) ) ;
#41976=CARTESIAN_POINT ( 'NONE',  ( -2.499999999999996447, -86.70833333060214443, 4.330127018922195425 ) ) ;
#41977=FACE_OUTER_BOUND ( 'NONE', #44916, .T. ) ;
#41979=AXIS2_PLACEMENT_3D ( 'NONE', #60023, #15946, #6307 ) ;
#41985=DIRECTION ( 'NONE',  ( 0.000000000000000000, 0.000000000000000000, 1.000000000000000000 ) ) ;
#41989=EDGE_LOOP ( 'NONE', ( #53411, #39060, #21664, #25468 ) ) ;
#41991=ORIENTED_EDGE ( 'NONE', *, *, #3325, .T. ) ;
#41996=ORIENTED_EDGE ( 'NONE', *, *, #2963, .F. ) ;
#41998=ORIENTED_EDGE ( 'NONE', *, *, #14576, .T. ) ;
#42001=CARTESIAN_POINT ( 'NONE',  ( -5.000000000000000000, -50.87499999726881583, 0.000000000000000000 ) ) ;
#42005=ORIENTED_EDGE ( 'NONE', *, *, #44419, .T. ) ;
#42007=CARTESIAN_POINT ( 'NONE',  ( 9.457646018065525792E-16, -81.06249999863440792, 5.148502694627439702 ) ) ;
#42008=CARTESIAN_POINT ( 'NONE',  ( 2.229367062499998831, 24.35416666803225993, -3.861377020970580887 ) ) ;
#42015=CARTESIAN_POINT ( 'NONE',  ( 2.500000000000002220, -27.66666666666666430, 4.330127018922192761 ) ) ;
#42016=CARTESIAN_POINT ( 'NONE',  ( 1.975475456537005874E-15, -82.74999999999998579, 5.000000000000000000 ) ) ;
#42018=CARTESIAN_POINT ( 'NONE',  ( 2.229367062500001939, -52.97916666530107221, 3.861377020970579999 ) ) ;
#42019=LINE ( 'NONE', #37837, #5837 ) ;
#42020=CARTESIAN_POINT ( 'NONE',  ( -4.458734124999999437, 27.68750000136559208, 0.000000000000000000 ) ) ;
#42022=CARTESIAN_POINT ( 'NONE',  ( -4.999999999999999112, -104.9166666666666572, 2.886751345948131764 ) ) ;
#42024=CARTESIAN_POINT ( 'NONE',  ( -3.152548672688508926E-16, -38.81249999863440081, -5.148502694627439702 ) ) ;
#42025=CARTESIAN_POINT ( 'NONE',  ( -5.000000000000000000, 1.125000002731184390, 0.000000000000000000 ) ) ;
#42029=CARTESIAN_POINT ( 'NONE',  ( -4.458734124999999437, -102.3958333319677365, -2.574251347313719407 ) ) ;
#42030=CARTESIAN_POINT ( 'NONE',  ( 4.458734124999998549, -4.979166665301071326, -2.574251347313721627 ) ) ;
#42032=CARTESIAN_POINT ( 'NONE',  ( 4.458734124999998549, -94.72916666530106511, -2.574251347313721627 ) ) ;
#42034=CARTESIAN_POINT ( 'NONE',  ( 4.458734124999998549, -88.97916666530107932, -2.574251347313721627 ) ) ;
#42037=CARTESIAN_POINT ( 'NONE',  ( 2.499999999999998668, -2.208333330602146205, -4.330127018922193649 ) ) ;
#42040=CARTESIAN_POINT ( 'NONE',  ( -4.458734124999999437, -11.31249999863440792, 0.000000000000000000 ) ) ;
#42041=CARTESIAN_POINT ( 'NONE',  ( 2.229367062499998831, 18.10416666803225993, -3.861377020970580887 ) ) ;
#42042=CARTESIAN_POINT ( 'NONE',  ( -2.229367062499996610, -53.39583333196773651, 3.861377020970582219 ) ) ;
#42043=CARTESIAN_POINT ( 'NONE',  ( -1.339745962155625802, 17.33034180399266688, 4.999999999999991118 ) ) ;
#42049=CARTESIAN_POINT ( 'NONE',  ( 3.044556291839386294E-14, 11.87500000273118417, -5.000000000000000000 ) ) ;
#42050=EDGE_CURVE ( 'NONE', #62343, #47452, #49543, .T. ) ;
#42051=CARTESIAN_POINT ( 'NONE',  ( 2.229367062499998831, -78.64583333196773651, -3.861377020970580887 ) ) ;
#42052=CARTESIAN_POINT ( 'NONE',  ( -4.458734124999999437, 22.43750000136559564, 0.000000000000000000 ) ) ;
#42056=ADVANCED_FACE ( 'NONE', ( #49431 ), #40092, .T. ) ;
#42057=DIRECTION ( 'NONE',  ( -0.000000000000000000, 1.000000000000000000, -0.000000000000000000 ) ) ;
#42059=CARTESIAN_POINT ( 'NONE',  ( 2.499999999999998668, -62.33333333333333570, -4.330127018922193649 ) ) ;
#42062=EDGE_LOOP ( 'NONE', ( #9241, #57788, #3662, #46044 ) ) ;
#42065=CARTESIAN_POINT ( 'NONE',  ( 7.204675194429079505E-15, 27.74999999999999645, -5.000000000000000000 ) ) ;
#42069=DIRECTION ( 'NONE',  ( 0.000000000000000000, 0.000000000000000000, 1.000000000000000000 ) ) ;
#42078=CARTESIAN_POINT ( 'NONE',  ( -2.229367062500000163, -53.72916666530107221, -3.861377020970580443 ) ) ;
#42080=CARTESIAN_POINT ( 'NONE',  ( -2.500000000000000444, -55.04166666393548013, -4.330127018922193649 ) ) ;
#42081=ORIENTED_EDGE ( 'NONE', *, *, #9423, .F. ) ;
#42083=ADVANCED_FACE ( 'NONE', ( #34632 ), #10198, .T. ) ;
#42088=CARTESIAN_POINT ( 'NONE',  ( 2.229367062500001939, -101.2291666653010651, 3.861377020970579999 ) ) ;
#42093=VECTOR ( 'NONE', #20788, 1000.000000000000000 ) ;
#42094=CARTESIAN_POINT ( 'NONE',  ( -4.458734124999998549, -8.229166665301073991, 2.574251347313722516 ) ) ;
#42095=CARTESIAN_POINT ( 'NONE',  ( -2.229367062499996610, -95.39583333196773651, 3.861377020970582219 ) ) ;
#42097=CARTESIAN_POINT ( 'NONE',  ( -2.229367062499996610, -22.39583333196773651, 3.861377020970582219 ) ) ;
#42100=CARTESIAN_POINT ( 'NONE',  ( 1.975475456537005874E-15, -22.74999999999999645, 5.000000000000000000 ) ) ;
#42103=CARTESIAN_POINT ( 'NONE',  ( 4.458734125000000326, 12.85416666803226171, 2.574251347313718519 ) ) ;
#42105=ORIENTED_EDGE ( 'NONE', *, *, #38170, .F. ) ;
#42106=CARTESIAN_POINT ( 'NONE',  ( -5.000000000000000000, -81.08333333333332860, -2.886751345948128211 ) ) ;
#42107=FACE_OUTER_BOUND ( 'NONE', #55599, .T. ) ;
#42108=CARTESIAN_POINT ( 'NONE',  ( 5.000000000000000000, -91.41666666666665719, -2.886751345948129988 ) ) ;
#42109=CARTESIAN_POINT ( 'NONE',  ( 4.458734125000001214, -24.89583333196773651, 2.574251347313718519 ) ) ;
#42111=CARTESIAN_POINT ( 'NONE',  ( -2.229367062500000163, -71.72916666530107932, -3.861377020970580443 ) ) ;
#42117=CARTESIAN_POINT ( 'NONE',  ( -2.229367062499996610, 8.854166668032261711, 3.861377020970582219 ) ) ;
#42118=CARTESIAN_POINT ( 'NONE',  ( -6.972266317189433020E-16, -63.12499999726880162, -5.000000000000000000 ) ) ;
#42119=CARTESIAN_POINT ( 'NONE',  ( 0.000000000000000000, -120.0000000000000000, 0.000000000000000000 ) ) ;
#42122=CARTESIAN_POINT ( 'NONE',  ( 4.458734124999998549, -71.72916666530107932, -2.574251347313721627 ) ) ;
#42124=CARTESIAN_POINT ( 'NONE',  ( -3.535250795749689387E-16, -2.250000000000001776, -5.773502691896257311 ) ) ;
#42127=CARTESIAN_POINT ( 'NONE',  ( 4.458734124999998549, -64.72916666530106511, -2.574251347313721627 ) ) ;
#42128=CARTESIAN_POINT ( 'NONE',  ( 5.000000000000000888, -99.45833333060213022, 2.886751345948126879 ) ) ;
#42130=CARTESIAN_POINT ( 'NONE',  ( 5.000000000000000000, -41.41666666666667140, -2.886751345948130876 ) ) ;
#42132=ADVANCED_FACE ( 'NONE', ( #16614 ), #50707, .T. ) ;
#42133=CARTESIAN_POINT ( 'NONE',  ( 9.457646018065525792E-16, -107.3124999986343937, 5.148502694627439702 ) ) ;
#42135=CARTESIAN_POINT ( 'NONE',  ( 2.499999999999998668, -47.33333333333333570, -4.330127018922193649 ) ) ;
#42136=CARTESIAN_POINT ( 'NONE',  ( -2.500000000000000444, -23.16666666666666785, -4.330127018922193649 ) ) ;
#42138=CARTESIAN_POINT ( 'NONE',  ( -2.499999999999996447, 16.16666666666666430, 4.330127018922195425 ) ) ;
#42141=VECTOR ( 'NONE', #52879, 1000.000000000000000 ) ;
#42145=EDGE_CURVE ( 'NONE', #63665, #19571, #56178, .T. ) ;
#42148=CARTESIAN_POINT ( 'NONE',  ( -6.972266317189433020E-16, -6.249999999999999112, -5.000000000000000000 ) ) ;
#42151=VERTEX_POINT ( 'NONE', #60376 ) ;
#42152=CARTESIAN_POINT ( 'NONE',  ( 5.000000000000000000, -81.50000000000000000, -6.123233995736766282E-16 ) ) ;
#42154=ORIENTED_EDGE ( 'NONE', *, *, #58181, .T. ) ;
#42158=CARTESIAN_POINT ( 'NONE',  ( 2.229367062500001939, -34.22916666530107221, 3.861377020970579999 ) ) ;
#42159=CARTESIAN_POINT ( 'NONE',  ( -5.000000000000000000, -87.00000000000000000, 0.000000000000000000 ) ) ;
#42167=CARTESIAN_POINT ( 'NONE',  ( 4.458734124999999437, -82.06249999863440792, -5.460374474430324690E-16 ) ) ;
#42173=CARTESIAN_POINT ( 'NONE',  ( 4.458734125000000326, -40.89583333196773651, 2.574251347313718519 ) ) ;
#42174=CARTESIAN_POINT ( 'NONE',  ( -4.458734124999999437, -9.645833331967738289, -2.574251347313719407 ) ) ;
#42177=CARTESIAN_POINT ( 'NONE',  ( 1.339745962155612702, 2.830341803992664662, -5.000000000000000000 ) ) ;
#42178=CARTESIAN_POINT ( 'NONE',  ( 2.229367062500001939, -4.229166665301070438, 3.861377020970579999 ) ) ;
#42179=DIRECTION ( 'NONE',  ( -0.000000000000000000, 1.000000000000000000, -0.000000000000000000 ) ) ;
#42182=CARTESIAN_POINT ( 'NONE',  ( -2.499999999999996447, -95.70833333060213022, 4.330127018922195425 ) ) ;
#42184=CARTESIAN_POINT ( 'NONE',  ( -4.458734124999999437, 26.35416666803225993, -2.574251347313719407 ) ) ;
#42186=CARTESIAN_POINT ( 'NONE',  ( 9.457646018065525792E-16, -84.06249999863439371, 5.148502694627439702 ) ) ;
#42188=CARTESIAN_POINT ( 'NONE',  ( 9.457646018065525792E-16, -11.06249999863440969, 5.148502694627439702 ) ) ;
#42189=CARTESIAN_POINT ( 'NONE',  ( -6.972266317189433020E-16, 19.75000000000000000, -5.000000000000000000 ) ) ;
#42190=CARTESIAN_POINT ( 'NONE',  ( 1.339745962155612702, -48.29465819873851729, -5.000000000000000000 ) ) ;
#42192=CARTESIAN_POINT ( 'NONE',  ( -5.000000000000000000, -33.95833333060213732, -2.886751345948128211 ) ) ;
#42194=CARTESIAN_POINT ( 'NONE',  ( 4.458734124999999437, 24.18750000136559564, -5.460374474430324690E-16 ) ) ;
#42197=CARTESIAN_POINT ( 'NONE',  ( -4.458734124999999437, -59.31249999863440081, 0.000000000000000000 ) ) ;
#42200=CARTESIAN_POINT ( 'NONE',  ( 1.060575238724906964E-15, 17.25000000000000000, 5.773502691896257311 ) ) ;
#42202=CARTESIAN_POINT ( 'NONE',  ( -2.500000000000000444, -46.16666666666666430, -4.330127018922193649 ) ) ;
#42203=CARTESIAN_POINT ( 'NONE',  ( 4.458734125000001214, -47.89583333196775072, 2.574251347313718519 ) ) ;
#42204=CARTESIAN_POINT ( 'NONE',  ( -5.000000000000000000, -84.87499999726880162, 0.000000000000000000 ) ) ;
#42206=CARTESIAN_POINT ( 'NONE',  ( 6.123233995736766282E-16, -120.0000000000000000, -5.000000000000000000 ) ) ;
#42207=CARTESIAN_POINT ( 'NONE',  ( 9.457646018065525792E-16, -87.31249999863440792, 5.148502694627439702 ) ) ;
#42209=CARTESIAN_POINT ( 'NONE',  ( 5.000000000000000000, -30.50000000000000000, -6.123233995736766282E-16 ) ) ;
#42210=CYLINDRICAL_SURFACE ( 'NONE', #11011, 5.000000000000000000 ) ;
#42214=VERTEX_POINT ( 'NONE', #1842 ) ;
#42215=CARTESIAN_POINT ( 'NONE',  ( -2.229367062499996610, -95.14583333196773651, 3.861377020970582219 ) ) ;
#42216=CARTESIAN_POINT ( 'NONE',  ( -2.229367062500000163, 16.27083333469892779, -3.861377020970580443 ) ) ;
#42217=CARTESIAN_POINT ( 'NONE',  ( 5.000000000000000888, 17.54166666939785557, 2.886751345948126879 ) ) ;
#42220=( BOUNDED_CURVE ( )  B_SPLINE_CURVE ( 2, ( #34569, #35548, #55173, #6287, #5965, #54530, #60323, #45508, #39713 ),
 .UNSPECIFIED., .F., .F. ) 
 B_SPLINE_CURVE_WITH_KNOTS ( ( 3, 2, 2, 2, 3 ),
 ( 0.9910714285714286031, 0.9916666666666666963, 0.9928571428571428825, 0.9940476190476190688, 0.9946428571428571619 ),
 .UNSPECIFIED. ) 
 CURVE ( )  GEOMETRIC_REPRESENTATION_ITEM ( )  RATIONAL_B_SPLINE_CURVE ( ( 0.9330127018922194093, 0.9330127018922194093, 1.000000000000000000, 0.8660254037844387076, 1.000000000000000000, 0.8660254037844387076, 1.000000000000000000, 0.9330127018922194093, 0.9330127018922194093 ) ) 
 REPRESENTATION_ITEM ( '' )  );
#42223=CARTESIAN_POINT ( 'NONE',  ( 5.000000000000000000, -82.50000000000000000, -6.123233995736766282E-16 ) ) ;
#42227=CARTESIAN_POINT ( 'NONE',  ( -2.499999999999996447, -25.70833333060214798, 4.330127018922195425 ) ) ;
#42231=CARTESIAN_POINT ( 'NONE',  ( -6.972266317189433020E-16, -43.25000000000000000, -5.000000000000000000 ) ) ;
#42232=CARTESIAN_POINT ( 'NONE',  ( 2.229367062499998831, -21.89583333196774007, -3.861377020970580887 ) ) ;
#42240=( BOUNDED_CURVE ( )  B_SPLINE_CURVE ( 2, ( #32461, #11885, #62380, #17361, #36661, #7402, #37294, #56923, #47266 ),
 .UNSPECIFIED., .F., .F. ) 
 B_SPLINE_CURVE_WITH_KNOTS ( ( 3, 2, 2, 2, 3 ),
 ( 0.6803571428571428825, 0.6809523809523809756, 0.6821428571428571619, 0.6833333333333333481, 0.6839285714285714413 ),
 .UNSPECIFIED. ) 
 CURVE ( )  GEOMETRIC_REPRESENTATION_ITEM ( )  RATIONAL_B_SPLINE_CURVE ( ( 0.9330127018922194093, 0.9330127018922194093, 1.000000000000000000, 0.8660254037844387076, 1.000000000000000000, 0.8660254037844387076, 1.000000000000000000, 0.9330127018922194093, 0.9330127018922194093 ) ) 
 REPRESENTATION_ITEM ( '' )  );
#42242=ORIENTED_EDGE ( 'NONE', *, *, #32238, .T. ) ;
#42245=CARTESIAN_POINT ( 'NONE',  ( -4.458734124999999437, -68.64583333196773651, -2.574251347313719407 ) ) ;
#42248=VERTEX_POINT ( 'NONE', #6650 ) ;
#42251=CYLINDRICAL_SURFACE ( 'NONE', #38075, 5.000000000000000000 ) ;
#42254=CARTESIAN_POINT ( 'NONE',  ( 2.499999999999998668, -45.33333333333333570, -4.330127018922193649 ) ) ;
#42255=CARTESIAN_POINT ( 'NONE',  ( -2.229367062500000163, 8.520833334698926009, -3.861377020970580443 ) ) ;
#42259=DIRECTION ( 'NONE',  ( 0.000000000000000000, 0.000000000000000000, 1.000000000000000000 ) ) ;
#42260=VERTEX_POINT ( 'NONE', #35601 ) ;
#42261=CARTESIAN_POINT ( 'NONE',  ( 2.229367062500001939, -71.97916666530107932, 3.861377020970579999 ) ) ;
#42262=CARTESIAN_POINT ( 'NONE',  ( 1.339745962155615144, 14.41965820146970323, 4.999999999999999112 ) ) ;
#42263=CARTESIAN_POINT ( 'NONE',  ( 4.458734124999998549, 9.270833334698927786, -2.574251347313721627 ) ) ;
#42264=EDGE_CURVE ( 'NONE', #58314, #483, #36032, .T. ) ;
#42266=CARTESIAN_POINT ( 'NONE',  ( -2.229367062499996610, -61.39583333196774362, 3.861377020970582219 ) ) ;
#42267=CARTESIAN_POINT ( 'NONE',  ( 2.499999999999998668, -21.20833333060214798, -4.330127018922193649 ) ) ;
#42268=CARTESIAN_POINT ( 'NONE',  ( -2.499999999999996447, -18.83333333333333215, 4.330127018922195425 ) ) ;
#42270=CARTESIAN_POINT ( 'NONE',  ( 1.339745962155612702, 19.83034180399266688, -5.000000000000000000 ) ) ;
#42272=CARTESIAN_POINT ( 'NONE',  ( 4.458734124999999437, -42.81249999863440081, -5.460374474430324690E-16 ) ) ;
#42273=CARTESIAN_POINT ( 'NONE',  ( 2.229367062500001939, -24.22916666530107577, 3.861377020970579999 ) ) ;
#42276=CARTESIAN_POINT ( 'NONE',  ( 4.458734125000001214, -107.8958333319677365, 2.574251347313718519 ) ) ;
#42278=EDGE_LOOP ( 'NONE', ( #2268, #52544, #55867, #59137 ) ) ;
#42279=CARTESIAN_POINT ( 'NONE',  ( 4.458734124999999437, -106.0624999986344221, -5.460374474430324690E-16 ) ) ;
#42280=VECTOR ( 'NONE', #42591, 1000.000000000000114 ) ;
#42281=CARTESIAN_POINT ( 'NONE',  ( 2.229367062500001939, -29.97916666530107221, 3.861377020970579999 ) ) ;
#42282=CARTESIAN_POINT ( 'NONE',  ( 1.060575238724906964E-15, -65.62499999726881583, 5.773502691896257311 ) ) ;
#42285=CARTESIAN_POINT ( 'NONE',  ( -2.229367062499996610, -28.14583333196774007, 3.861377020970582219 ) ) ;
#42286=CARTESIAN_POINT ( 'NONE',  ( 4.458734124999998549, -68.97916666530107932, -2.574251347313721627 ) ) ;
#42290=CARTESIAN_POINT ( 'NONE',  ( 2.499999999999998668, -14.33333333333333037, -4.330127018922193649 ) ) ;
#42292=ORIENTED_EDGE ( 'NONE', *, *, #53534, .T. ) ;
#42293=CARTESIAN_POINT ( 'NONE',  ( -5.000000000000000000, -82.00000000000000000, 0.000000000000000000 ) ) ;
#42295=( BOUNDED_CURVE ( )  B_SPLINE_CURVE ( 2, ( #2599, #2925, #22856, #33129, #3548, #22540, #42136, #27346, #31857 ),
 .UNSPECIFIED., .F., .F. ) 
 B_SPLINE_CURVE_WITH_KNOTS ( ( 3, 2, 2, 2, 3 ),
 ( 0.3767857142857142794, 0.3773809523809523725, 0.3785714285714285587, 0.3797619047619047450, 0.3803571428571428381 ),
 .UNSPECIFIED. ) 
 CURVE ( )  GEOMETRIC_REPRESENTATION_ITEM ( )  RATIONAL_B_SPLINE_CURVE ( ( 0.9330127018922194093, 0.9330127018922194093, 1.000000000000000000, 0.8660254037844387076, 1.000000000000000000, 0.8660254037844387076, 1.000000000000000000, 0.9330127018922194093, 0.9330127018922194093 ) ) 
 REPRESENTATION_ITEM ( '' )  );
#42299=CARTESIAN_POINT ( 'NONE',  ( -1.336351044127974539E-14, 25.24999999999999645, 5.000000000000000000 ) ) ;
#42307=EDGE_LOOP ( 'NONE', ( #16915, #10053, #1311, #14555 ) ) ;
#42308=CARTESIAN_POINT ( 'NONE',  ( -6.972266317189433020E-16, -33.24999999999999289, -5.000000000000000000 ) ) ;
#42314=ORIENTED_EDGE ( 'NONE', *, *, #20787, .F. ) ;
#42317=CARTESIAN_POINT ( 'NONE',  ( -6.972266317189433020E-16, -95.25000000000000000, -5.000000000000000000 ) ) ;
#42321=CARTESIAN_POINT ( 'NONE',  ( -5.000000000000000000, 23.04166666939784847, -2.886751345948128211 ) ) ;
#42322=VERTEX_POINT ( 'NONE', #22403 ) ;
#42323=CARTESIAN_POINT ( 'NONE',  ( 9.457646018065525792E-16, -84.06249999863439371, 5.148502694627439702 ) ) ;
#42324=CARTESIAN_POINT ( 'NONE',  ( 9.457646018065525792E-16, 25.93750000136559564, 5.148502694627439702 ) ) ;
#42327=CARTESIAN_POINT ( 'NONE',  ( 2.500000000000002220, 14.33333333333333393, 4.330127018922192761 ) ) ;
#42333=( BOUNDED_CURVE ( )  B_SPLINE_CURVE ( 2, ( #38535, #13483, #4760, #24078, #48195, #62695, #53340, #29510, #43989 ),
 .UNSPECIFIED., .F., .F. ) 
 B_SPLINE_CURVE_WITH_KNOTS ( ( 3, 2, 2, 2, 3 ),
 ( 0.1982142857142857040, 0.1988095238095237971, 0.2000000000000000111, 0.2011904761904761973, 0.2017857142857142905 ),
 .UNSPECIFIED. ) 
 CURVE ( )  GEOMETRIC_REPRESENTATION_ITEM ( )  RATIONAL_B_SPLINE_CURVE ( ( 0.9330127018922194093, 0.9330127018922194093, 1.000000000000000000, 0.8660254037844387076, 1.000000000000000000, 0.8660254037844387076, 1.000000000000000000, 0.9330127018922194093, 0.9330127018922194093 ) ) 
 REPRESENTATION_ITEM ( '' )  );
#42335=CARTESIAN_POINT ( 'NONE',  ( 4.458734124999999437, -52.81249999863440792, -5.460374474430324690E-16 ) ) ;
#42336=CARTESIAN_POINT ( 'NONE',  ( 2.500000000000002220, 10.33333333333333393, 4.330127018922192761 ) ) ;
#42337=CARTESIAN_POINT ( 'NONE',  ( -2.229367062499996610, 20.85416666803226349, 3.861377020970582219 ) ) ;
#42338=CARTESIAN_POINT ( 'NONE',  ( 2.500000000000002220, -105.6666666666666572, 4.330127018922192761 ) ) ;
#42340=CARTESIAN_POINT ( 'NONE',  ( 2.229367062499998831, -41.89583333196773651, -3.861377020970580887 ) ) ;
#42341=CARTESIAN_POINT ( 'NONE',  ( 5.000000000000000000, -4.374999997268816720, -6.123233995736766282E-16 ) ) ;
#42346=CARTESIAN_POINT ( 'NONE',  ( 9.457646018065525792E-16, -100.0624999986344221, 5.148502694627439702 ) ) ;
#42347=CARTESIAN_POINT ( 'NONE',  ( 4.458734125000000326, -3.145833331967738289, 2.574251347313718519 ) ) ;
#42350=CARTESIAN_POINT ( 'NONE',  ( 4.458734124999998549, -93.72916666530105090, -2.574251347313721627 ) ) ;
#42352=CARTESIAN_POINT ( 'NONE',  ( -4.458734124999998549, -92.47916666530106511, 2.574251347313722516 ) ) ;
#42354=DIRECTION ( 'NONE',  ( -0.000000000000000000, 1.000000000000000000, -0.000000000000000000 ) ) ;
#42356=CARTESIAN_POINT ( 'NONE',  ( 2.229367062499998831, -14.64583333196773474, -3.861377020970580887 ) ) ;
#42357=CARTESIAN_POINT ( 'NONE',  ( -4.458734124999998549, 14.52083333469892779, 2.574251347313722516 ) ) ;
#42358=CARTESIAN_POINT ( 'NONE',  ( 4.458734125000000326, -52.14583333196773651, 2.574251347313718519 ) ) ;
#42359=FACE_OUTER_BOUND ( 'NONE', #32276, .T. ) ;
#42362=CARTESIAN_POINT ( 'NONE',  ( 5.000000000000000000, -106.2916666639354730, -2.886751345948130876 ) ) ;
#42363=VERTEX_POINT ( 'NONE', #22720 ) ;
#42367=CARTESIAN_POINT ( 'NONE',  ( 9.457646018065525792E-16, -80.06249999863439371, 5.148502694627439702 ) ) ;
#42368=CARTESIAN_POINT ( 'NONE',  ( 4.458734124999998549, 22.02083333469892779, -2.574251347313721627 ) ) ;
#42370=CARTESIAN_POINT ( 'NONE',  ( -1.339745962155610925, 7.205341801261477386, 5.000000000000000000 ) ) ;
#42373=CARTESIAN_POINT ( 'NONE',  ( 5.000000000000000000, -69.49999999999998579, -6.123233995736766282E-16 ) ) ;
#42374=CARTESIAN_POINT ( 'NONE',  ( 1.975475456537005874E-15, -63.62499999726880873, 5.000000000000000000 ) ) ;
#42376=VERTEX_POINT ( 'NONE', #3728 ) ;
#42378=CARTESIAN_POINT ( 'NONE',  ( 5.000000000000000000, 7.583333333333333925, -2.886751345948130876 ) ) ;
#42385=ORIENTED_EDGE ( 'NONE', *, *, #3416, .F. ) ;
#42391=CARTESIAN_POINT ( 'NONE',  ( 2.229367062499998831, -53.89583333196773651, -3.861377020970580887 ) ) ;
#42396=ADVANCED_FACE ( 'NONE', ( #62276 ), #62896, .T. ) ;
#42401=CARTESIAN_POINT ( 'NONE',  ( 4.458734124999999437, -99.06249999863440792, -5.460374474430324690E-16 ) ) ;
#42402=VERTEX_POINT ( 'NONE', #42317 ) ;
#42406=CARTESIAN_POINT ( 'NONE',  ( 4.458734124999999437, -6.812499998634404363, -5.460374474430324690E-16 ) ) ;
#42407=( BOUNDED_CURVE ( )  B_SPLINE_CURVE ( 2, ( #20911, #5472, #44377, #44696, #39868, #40516, #60158, #30872, #15121 ),
 .UNSPECIFIED., .F., .F. ) 
 B_SPLINE_CURVE_WITH_KNOTS ( ( 3, 2, 2, 2, 3 ),
 ( 0.9267857142857143238, 0.9273809523809524169, 0.9285714285714286031, 0.9297619047619047894, 0.9303571428571428825 ),
 .UNSPECIFIED. ) 
 CURVE ( )  GEOMETRIC_REPRESENTATION_ITEM ( )  RATIONAL_B_SPLINE_CURVE ( ( 0.9330127018922194093, 0.9330127018922194093, 1.000000000000000000, 0.8660254037844387076, 1.000000000000000000, 0.8660254037844387076, 1.000000000000000000, 0.9330127018922194093, 0.9330127018922194093 ) ) 
 REPRESENTATION_ITEM ( '' )  );
#42408=CARTESIAN_POINT ( 'NONE',  ( 4.458734124999999437, -93.06249999863440792, -5.460374474430324690E-16 ) ) ;
#42410=CARTESIAN_POINT ( 'NONE',  ( 4.458734124999998549, -27.97916666530107577, -2.574251347313721627 ) ) ;
#42411=EDGE_CURVE ( 'NONE', #5841, #34951, #14220, .T. ) ;
#42416=CYLINDRICAL_SURFACE ( 'NONE', #35685, 5.000000000000000000 ) ;
#42418=CARTESIAN_POINT ( 'NONE',  ( -4.458734124999999437, 10.43750000136559386, 0.000000000000000000 ) ) ;
#42421=CARTESIAN_POINT ( 'NONE',  ( 5.000000000000000888, -61.58333333333333570, 2.886751345948126879 ) ) ;
#42422=CARTESIAN_POINT ( 'NONE',  ( -3.535250795749689387E-16, -90.24999999999998579, -5.773502691896257311 ) ) ;
#42423=CARTESIAN_POINT ( 'NONE',  ( 9.457646018065525792E-16, -22.06249999863440436, 5.148502694627439702 ) ) ;
#42424=CARTESIAN_POINT ( 'NONE',  ( 0.000000000000000000, -120.0000000000000000, 5.000000000000000000 ) ) ;
#42425=CARTESIAN_POINT ( 'NONE',  ( 4.458734124999999437, -70.06249999863439371, -5.460374474430324690E-16 ) ) ;
#42430=CARTESIAN_POINT ( 'NONE',  ( -4.458734124999999437, 2.687500001365593860, 0.000000000000000000 ) ) ;
#42431=CARTESIAN_POINT ( 'NONE',  ( 6.123233995736766282E-16, -120.0000000000000000, -5.000000000000000000 ) ) ;
#42432=DIRECTION ( 'NONE',  ( 0.000000000000000000, 0.000000000000000000, 1.000000000000000000 ) ) ;
#42434=CARTESIAN_POINT ( 'NONE',  ( -4.458734124999999437, -74.31249999863440792, 0.000000000000000000 ) ) ;
#42436=CARTESIAN_POINT ( 'NONE',  ( -3.535250795749689387E-16, -5.249999999999997335, -5.773502691896257311 ) ) ;
#42439=CARTESIAN_POINT ( 'NONE',  ( -2.229367062500000163, -62.47916666530106511, -3.861377020970580443 ) ) ;
#42440=CARTESIAN_POINT ( 'NONE',  ( 5.000000000000000888, -100.4583333306021444, 2.886751345948126879 ) ) ;
#42444=CARTESIAN_POINT ( 'NONE',  ( -4.458734124999999437, -107.5624999986343937, 0.000000000000000000 ) ) ;
#42446=CARTESIAN_POINT ( 'NONE',  ( 5.000000000000000888, -48.58333333333332149, 2.886751345948126879 ) ) ;
#42451=CARTESIAN_POINT ( 'NONE',  ( -2.500000000000000444, -100.0416666639354588, -4.330127018922193649 ) ) ;
#42459=CARTESIAN_POINT ( 'NONE',  ( 6.123233995736766282E-16, -120.0000000000000000, -5.000000000000000000 ) ) ;
#42466=CARTESIAN_POINT ( 'NONE',  ( 2.229367062500001939, -38.22916666530107221, 3.861377020970579999 ) ) ;
#42470=CARTESIAN_POINT ( 'NONE',  ( 0.000000000000000000, -120.0000000000000000, 0.000000000000000000 ) ) ;
#42472=ADVANCED_FACE ( 'NONE', ( #13054 ), #18198, .T. ) ;
#42479=CARTESIAN_POINT ( 'NONE',  ( 9.457646018065525792E-16, -84.31249999863437949, 5.148502694627439702 ) ) ;
#42482=CARTESIAN_POINT ( 'NONE',  ( -4.999999999999998224, -94.79166666393547303, 2.886751345948131764 ) ) ;
#42486=EDGE_LOOP ( 'NONE', ( #34422, #31872, #54971, #5159 ) ) ;
#42487=EDGE_CURVE ( 'NONE', #24623, #40250, #29805, .T. ) ;
#42489=CARTESIAN_POINT ( 'NONE',  ( 5.000000000000000000, 17.58333333333333215, -2.886751345948130876 ) ) ;
#42490=CARTESIAN_POINT ( 'NONE',  ( -2.229367062499996610, -5.395833331967740953, 3.861377020970582219 ) ) ;
#42494=CARTESIAN_POINT ( 'NONE',  ( -5.000000000000000000, -95.95833333060213022, -2.886751345948128211 ) ) ;
#42496=CARTESIAN_POINT ( 'NONE',  ( -4.458734124999999437, 27.43750000136559208, 0.000000000000000000 ) ) ;
#42497=ORIENTED_EDGE ( 'NONE', *, *, #21676, .T. ) ;
#42498=CARTESIAN_POINT ( 'NONE',  ( -4.458734124999997661, -93.22916666530107932, 2.574251347313722516 ) ) ;
#42499=CARTESIAN_POINT ( 'NONE',  ( -4.999999999999998224, -67.91666666666667140, 2.886751345948131764 ) ) ;
#42500=CARTESIAN_POINT ( 'NONE',  ( -4.999999999999998224, -69.79166666393547303, 2.886751345948131764 ) ) ;
#42501=CARTESIAN_POINT ( 'NONE',  ( -2.229367062500000163, -7.479166665301073991, -3.861377020970580443 ) ) ;
#42502=CARTESIAN_POINT ( 'NONE',  ( 0.000000000000000000, -120.0000000000000000, 5.000000000000000000 ) ) ;
#42503=CARTESIAN_POINT ( 'NONE',  ( 1.339745962155615144, -48.70534180126148271, 4.999999999999999112 ) ) ;
#42505=CARTESIAN_POINT ( 'NONE',  ( 2.500000000000002220, -33.54166666393547303, 4.330127018922192761 ) ) ;
#42507=CARTESIAN_POINT ( 'NONE',  ( -3.152548672688508926E-16, 20.43750000136559208, -5.148502694627439702 ) ) ;
#42508=CARTESIAN_POINT ( 'NONE',  ( -5.000000000000000000, -97.95833333060214443, -2.886751345948128211 ) ) ;
#42510=CARTESIAN_POINT ( 'NONE',  ( 4.458734124999999437, -54.81249999863440081, -5.460374474430324690E-16 ) ) ;
#42512=( BOUNDED_CURVE ( )  B_SPLINE_CURVE ( 2, ( #51369, #56515, #27229, #46850, #2797, #18527, #18824, #58070, #13694 ),
 .UNSPECIFIED., .F., .F. ) 
 B_SPLINE_CURVE_WITH_KNOTS ( ( 3, 2, 2, 2, 3 ),
 ( 0.7375000000000000444, 0.7380952380952381375, 0.7392857142857143238, 0.7404761904761905100, 0.7410714285714286031 ),
 .UNSPECIFIED. ) 
 CURVE ( )  GEOMETRIC_REPRESENTATION_ITEM ( )  RATIONAL_B_SPLINE_CURVE ( ( 0.9330127018922194093, 0.9330127018922194093, 1.000000000000000000, 0.8660254037844387076, 1.000000000000000000, 0.8660254037844387076, 1.000000000000000000, 0.9330127018922194093, 0.9330127018922194093 ) ) 
 REPRESENTATION_ITEM ( '' )  );
#42514=CARTESIAN_POINT ( 'NONE',  ( -5.000000000000000000, 15.91666666666666430, -2.886751345948128211 ) ) ;
#42517=CARTESIAN_POINT ( 'NONE',  ( -2.229367062499996610, -46.14583333196774362, 3.861377020970582219 ) ) ;
#42518=CARTESIAN_POINT ( 'NONE',  ( -2.499999999999996447, -84.70833333060214443, 4.330127018922195425 ) ) ;
#42520=VECTOR ( 'NONE', #38530, 1000.000000000000000 ) ;
#42522=CARTESIAN_POINT ( 'NONE',  ( 1.975475456537005874E-15, -104.6249999972688016, 5.000000000000000000 ) ) ;
#42523=CARTESIAN_POINT ( 'NONE',  ( 4.458734124999998549, -83.97916666530106511, -2.574251347313721627 ) ) ;
#42525=CARTESIAN_POINT ( 'NONE',  ( -3.535250795749689387E-16, -35.25000000000000000, -5.773502691896257311 ) ) ;
#42526=DIRECTION ( 'NONE',  ( -0.000000000000000000, 1.000000000000000000, -0.000000000000000000 ) ) ;
#42527=ORIENTED_EDGE ( 'NONE', *, *, #33478, .F. ) ;
#42529=ORIENTED_EDGE ( 'NONE', *, *, #34705, .F. ) ;
#42530=CARTESIAN_POINT ( 'NONE',  ( -4.458734124999998549, -98.22916666530105090, 2.574251347313722516 ) ) ;
#42531=CARTESIAN_POINT ( 'NONE',  ( -4.458734124999998549, 7.520833334698926009, 2.574251347313722516 ) ) ;
#42532=CARTESIAN_POINT ( 'NONE',  ( -3.535250795749689387E-16, 12.87500000273118417, -5.773502691896257311 ) ) ;
#42533=LINE ( 'NONE', #11997, #48332 ) ;
#42537=CARTESIAN_POINT ( 'NONE',  ( 1.060575238724906964E-15, -80.75000000000000000, 5.773502691896257311 ) ) ;
#42539=LINE ( 'NONE', #12334, #24510 ) ;
#42541=CARTESIAN_POINT ( 'NONE',  ( 1.339745962155612702, -109.2946581987385315, -5.000000000000000000 ) ) ;
#42544=CARTESIAN_POINT ( 'NONE',  ( -1.339745962155610925, 14.20534180126148094, 5.000000000000000000 ) ) ;
#42545=CARTESIAN_POINT ( 'NONE',  ( 2.229367062499998831, -20.89583333196774007, -3.861377020970580887 ) ) ;
#42546=CARTESIAN_POINT ( 'NONE',  ( -2.499999999999996447, -57.83333333333333570, 4.330127018922195425 ) ) ;
#42555=CYLINDRICAL_SURFACE ( 'NONE', #30248, 5.000000000000000000 ) ;
#42556=ORIENTED_EDGE ( 'NONE', *, *, #49250, .F. ) ;
#42557=CARTESIAN_POINT ( 'NONE',  ( 4.458734124999998549, -69.97916666530107932, -2.574251347313721627 ) ) ;
#42559=DIRECTION ( 'NONE',  ( 0.8660254037844385966, 0.5000000000000001110, 0.000000000000000000 ) ) ;
#42567=CARTESIAN_POINT ( 'NONE',  ( 2.500000000000002220, -45.66666666666666430, 4.330127018922192761 ) ) ;
#42568=CARTESIAN_POINT ( 'NONE',  ( 2.229367062500001939, 10.02083333469892779, 3.861377020970579999 ) ) ;
#42569=ADVANCED_FACE ( 'NONE', ( #39062 ), #59331, .T. ) ;
#42572=CARTESIAN_POINT ( 'NONE',  ( -2.500000000000000444, 5.958333336064519870, -4.330127018922193649 ) ) ;
#42575=EDGE_CURVE ( 'NONE', #28956, #23230, #43878, .T. ) ;
#42576=CARTESIAN_POINT ( 'NONE',  ( 2.229367062499998831, -72.64583333196773651, -3.861377020970580887 ) ) ;
#42577=LINE ( 'NONE', #32935, #34603 ) ;
#42578=CARTESIAN_POINT ( 'NONE',  ( -4.458734124999999437, 8.687500001365595637, 0.000000000000000000 ) ) ;
#42579=EDGE_CURVE ( 'NONE', #4978, #29860, #5592, .T. ) ;
#42581=CARTESIAN_POINT ( 'NONE',  ( 2.229367062500001939, -62.22916666530106511, 3.861377020970579999 ) ) ;
#42582=CARTESIAN_POINT ( 'NONE',  ( -2.499999999999996447, -17.70833333060214443, 4.330127018922195425 ) ) ;
#42583=CARTESIAN_POINT ( 'NONE',  ( -5.000000000000000000, -32.87499999726880873, 0.000000000000000000 ) ) ;
#42588=CARTESIAN_POINT ( 'NONE',  ( 4.458734125000001214, -42.89583333196773651, 2.574251347313718519 ) ) ;
#42589=CARTESIAN_POINT ( 'NONE',  ( -3.152548672688508926E-16, -25.81249999863440792, -5.148502694627439702 ) ) ;
#42591=DIRECTION ( 'NONE',  ( -0.8660254037844410391, 0.4999999999999958367, 0.000000000000000000 ) ) ;
#42592=CARTESIAN_POINT ( 'NONE',  ( -4.458734124999999437, -108.3124999986343937, 0.000000000000000000 ) ) ;
#42594=VERTEX_POINT ( 'NONE', #14619 ) ;
#42595=CARTESIAN_POINT ( 'NONE',  ( 2.229367062499998831, -109.8958333319677365, -3.861377020970580887 ) ) ;
#42596=CARTESIAN_POINT ( 'NONE',  ( -2.229367062499996610, -31.14583333196773651, 3.861377020970582219 ) ) ;
#42597=CARTESIAN_POINT ( 'NONE',  ( -2.500000000000000444, -68.04166666393547303, -4.330127018922193649 ) ) ;
#42601=CARTESIAN_POINT ( 'NONE',  ( 2.229367062500001939, -28.97916666530107221, 3.861377020970579999 ) ) ;
#42602=CARTESIAN_POINT ( 'NONE',  ( 4.458734124999998549, -70.97916666530107932, -2.574251347313721627 ) ) ;
#42606=FACE_OUTER_BOUND ( 'NONE', #31501, .T. ) ;
#42607=CARTESIAN_POINT ( 'NONE',  ( -3.535250795749689387E-16, -18.25000000000000355, -5.773502691896257311 ) ) ;
#42610=FACE_OUTER_BOUND ( 'NONE', #20902, .T. ) ;
#42612=CARTESIAN_POINT ( 'NONE',  ( 5.000000000000000000, 28.62500000273118417, -6.123233995736766282E-16 ) ) ;
#42613=DIRECTION ( 'NONE',  ( 0.000000000000000000, 0.000000000000000000, 1.000000000000000000 ) ) ;
#42615=CARTESIAN_POINT ( 'NONE',  ( 1.975475456537005874E-15, 8.375000002731187720, 5.000000000000000000 ) ) ;
#42619=LINE ( 'NONE', #13353, #39924 ) ;
#42621=EDGE_LOOP ( 'NONE', ( #27555, #38508, #38801, #11281 ) ) ;
#42623=ORIENTED_EDGE ( 'NONE', *, *, #57131, .T. ) ;
#42628=VERTEX_POINT ( 'NONE', #34231 ) ;
#42630=ORIENTED_EDGE ( 'NONE', *, *, #29400, .T. ) ;
#42631=CARTESIAN_POINT ( 'NONE',  ( 2.499999999999998668, -34.33333333333332860, -4.330127018922193649 ) ) ;
#42637=EDGE_LOOP ( 'NONE', ( #44766, #50496, #53304, #30215, #17187, #6499, #49350, #5976, #59401, #42005, #56229, #12815, #52817, #17410, #8309, #8388, #31769, #21049, #11822, #48550, #1829, #13690, #17504, #4028, #37996, #51211, #29750, #53422, #59729, #50307, #16190, #14386, #55643, #51502, #16619, #18279, #18366, #21827, #24917, #8224, #55466, #58467, #19846, #6867, #28213, #34114, #49605, #59956, #23332, #22957, #43851, #52538, #17244, #39555, #28446, #17199, #12968, #26580, #24425, #26370, #30453, #18341, #3969, #46191, #39919, #22143, #45255, #43250, #15769, #28054, #8096, #18119, #5431, #30663, #15082, #24743, #33824, #8627, #50314, #43437, #60860, #11993, #48376, #3870, #31344, #62361, #52313, #62104, #36179, #29783, #55800, #58207, #18581, #31890, #53157, #35264, #45094, #3419, #31979, #32885, #62600, #488, #51521, #38499, #42709, #15268, #4511, #20528, #60153, #47567, #13058, #6182, #16259, #8248, #24092, #55648, #26975, #41998, #5127, #38681, #50055, #34670, #55143, #12214, #51253, #4872, #10429, #47459, #49741, #43306, #63587, #1847, #21520, #38664, #25425, #2308, #16450, #7986, #16981, #51040, #14411, #13311, #57929, #48017, #7620, #16145, #51749, #1801, #5614, #50756, #10359, #24045, #8677, #1349, #17203, #3343, #58193, #45814, #10627, #46176, #15846, #4661, #15662, #37153, #10492, #60130, #11456, #45750, #17169, #49252, #17510, #19842, #39226, #8232, #26842, #36472, #29573, #27709, #41042, #34790, #27204, #4389, #50788, #51758, #17864, #46870, #63237, #36057, #9551, #47203, #2712, #8817, #20155, #742, #63138, #632, #58103, #23508, #9328, #48023, #47766, #36209, #31795, #7328, #21480, #14627, #23600, #31085, #19447, #57833, #11290, #58909, #13708, #12088, #20242, #55375, #38296, #31254, #36397, #1456, #61, #19556, #48467, #31753, #26660, #43611, #39169, #59726, #52556, #58119, #52613, #52382, #59011, #23358, #10753, #5202, #15934, #32501, #24984, #6096, #245, #53397, #4374, #25772, #58383, #59579, #49704, #23710, #33264, #2831, #8798, #42870, #52882, #8004, #1195, #37807, #41282, #63606, #60550, #7109, #37757, #53905, #41208, #41847, #36831, #31717, #2297, #10695, #54431, #13365, #2455, #54872, #61355, #42886, #59987, #31469, #12661, #61318, #49744, #38573, #12379, #43181, #28924, #15233 ) ) ;
#42638=CARTESIAN_POINT ( 'NONE',  ( 4.458734125000001214, -79.89583333196773651, 2.574251347313718519 ) ) ;
#42639=CARTESIAN_POINT ( 'NONE',  ( 4.458734124999998549, 26.27083333469893134, -2.574251347313721627 ) ) ;
#42640=CARTESIAN_POINT ( 'NONE',  ( 1.975475456537005874E-15, -12.62499999726881050, 5.000000000000000000 ) ) ;
#42642=AXIS2_PLACEMENT_3D ( 'NONE', #23662, #8009, #33620 ) ;
#42650=CARTESIAN_POINT ( 'NONE',  ( 4.458734124999999437, -54.81249999863440081, -5.460374474430324690E-16 ) ) ;
#42651=CARTESIAN_POINT ( 'NONE',  ( 5.000000000000000000, 10.58333333333333393, -2.886751345948130876 ) ) ;
#42652=CARTESIAN_POINT ( 'NONE',  ( -4.458734124999999437, 22.60416666803225993, -2.574251347313719407 ) ) ;
#42653=CARTESIAN_POINT ( 'NONE',  ( 5.000000000000000888, -109.5833333333333286, 2.886751345948126879 ) ) ;
#42654=AXIS2_PLACEMENT_3D ( 'NONE', #52610, #28157, #43256 ) ;
#42656=CARTESIAN_POINT ( 'NONE',  ( -4.458734124999998549, -42.47916666530107932, 2.574251347313722516 ) ) ;
#42657=CARTESIAN_POINT ( 'NONE',  ( -2.500000000000000444, -5.041666663935480130, -4.330127018922193649 ) ) ;
#42661=CARTESIAN_POINT ( 'NONE',  ( -4.458734124999997661, -100.2291666653010509, 2.574251347313722516 ) ) ;
#42662=CARTESIAN_POINT ( 'NONE',  ( 2.229367062500001939, -7.229166665301073103, 3.861377020970579999 ) ) ;
#42663=( BOUNDED_CURVE ( )  B_SPLINE_CURVE ( 2, ( #53132, #58896, #4246, #692, #14825, #20305, #13886, #48921, #9064 ),
 .UNSPECIFIED., .F., .F. ) 
 B_SPLINE_CURVE_WITH_KNOTS ( ( 3, 2, 2, 2, 3 ),
 ( 0.3482142857142856984, 0.3488095238095237915, 0.3499999999999999778, 0.3511904761904761640, 0.3517857142857143127 ),
 .UNSPECIFIED. ) 
 CURVE ( )  GEOMETRIC_REPRESENTATION_ITEM ( )  RATIONAL_B_SPLINE_CURVE ( ( 0.9330127018922194093, 0.9330127018922194093, 1.000000000000000000, 0.8660254037844387076, 1.000000000000000000, 0.8660254037844387076, 1.000000000000000000, 0.9330127018922163007, 0.9330127018922194093 ) ) 
 REPRESENTATION_ITEM ( '' )  );
#42665=CARTESIAN_POINT ( 'NONE',  ( -3.152548672688508926E-16, -92.56249999863439371, -5.148502694627439702 ) ) ;
#42667=CARTESIAN_POINT ( 'NONE',  ( 4.458734125000001214, -94.14583333196773651, 2.574251347313718519 ) ) ;
#42670=CARTESIAN_POINT ( 'NONE',  ( -4.458734124999997661, -13.22916666530107399, 2.574251347313722516 ) ) ;
#42671=CARTESIAN_POINT ( 'NONE',  ( 2.229367062500001939, 10.77083333469892956, 3.861377020970579999 ) ) ;
#42672=CARTESIAN_POINT ( 'NONE',  ( -4.458734124999997661, -54.47916666530107932, 2.574251347313722516 ) ) ;
#42679=CARTESIAN_POINT ( 'NONE',  ( 1.339745962155615144, -76.70534180126148271, 4.999999999999999112 ) ) ;
#42681=CARTESIAN_POINT ( 'NONE',  ( 4.458734125000001214, -81.89583333196773651, 2.574251347313718519 ) ) ;
#42682=CARTESIAN_POINT ( 'NONE',  ( -4.458734124999999437, 24.35416666803225993, -2.574251347313719407 ) ) ;
#42684=DIRECTION ( 'NONE',  ( -0.000000000000000000, 1.000000000000000000, -0.000000000000000000 ) ) ;
#42687=CARTESIAN_POINT ( 'NONE',  ( -5.000000000000000000, -69.08333333333332860, -2.886751345948128211 ) ) ;
#42691=( BOUNDED_CURVE ( )  B_SPLINE_CURVE ( 2, ( #21350, #1114, #788, #56082, #55765, #50616, #20721, #10739, #26169 ),
 .UNSPECIFIED., .F., .F. ) 
 B_SPLINE_CURVE_WITH_KNOTS ( ( 3, 2, 2, 2, 3 ),
 ( 0.09464285714285713969, 0.09523809523809523281, 0.09642857142857143293, 0.09761904761904761918, 0.09821428571428571230 ),
 .UNSPECIFIED. ) 
 CURVE ( )  GEOMETRIC_REPRESENTATION_ITEM ( )  RATIONAL_B_SPLINE_CURVE ( ( 0.9330127018922194093, 0.9330127018922194093, 1.000000000000000000, 0.8660254037844387076, 1.000000000000000000, 0.8660254037844387076, 1.000000000000000000, 0.9330127018922194093, 0.9330127018922194093 ) ) 
 REPRESENTATION_ITEM ( '' )  );
#42692=DIRECTION ( 'NONE',  ( 0.000000000000000000, 0.000000000000000000, 1.000000000000000000 ) ) ;
#42693=CARTESIAN_POINT ( 'NONE',  ( -1.339745962155727277, -108.6696581960073331, 4.999999999999933387 ) ) ;
#42699=EDGE_LOOP ( 'NONE', ( #19114, #7047, #39943, #60929 ) ) ;
#42705=CARTESIAN_POINT ( 'NONE',  ( -2.229367062500000163, -52.72916666530107221, -3.861377020970580443 ) ) ;
#42709=ORIENTED_EDGE ( 'NONE', *, *, #14593, .T. ) ;
#42713=ORIENTED_EDGE ( 'NONE', *, *, #21285, .F. ) ;
#42716=CARTESIAN_POINT ( 'NONE',  ( 4.458734125000001214, -98.14583333196773651, 2.574251347313718519 ) ) ;
#42722=CARTESIAN_POINT ( 'NONE',  ( 2.229367062500001939, -5.979166665301072214, 3.861377020970579999 ) ) ;
#42723=CARTESIAN_POINT ( 'NONE',  ( 4.458734124999998549, -95.97916666530107932, -2.574251347313721627 ) ) ;
#42725=CARTESIAN_POINT ( 'NONE',  ( 4.458734124999999437, -29.06249999863440436, -5.460374474430324690E-16 ) ) ;
#42729=CARTESIAN_POINT ( 'NONE',  ( -2.500000000000000444, -91.16666666666665719, -4.330127018922193649 ) ) ;
#42730=CARTESIAN_POINT ( 'NONE',  ( 2.500000000000002220, -88.54166666393548724, 4.330127018922192761 ) ) ;
#42732=CARTESIAN_POINT ( 'NONE',  ( 2.229367062499998831, 8.104166668032261711, -3.861377020970580887 ) ) ;
#42735=LINE ( 'NONE', #51463, #21267 ) ;
#42737=CARTESIAN_POINT ( 'NONE',  ( 5.000000000000000000, -90.50000000000000000, -6.123233995736766282E-16 ) ) ;
#42738=CARTESIAN_POINT ( 'NONE',  ( 4.458734124999999437, -25.81249999863440792, -5.460374474430324690E-16 ) ) ;
#42740=CARTESIAN_POINT ( 'NONE',  ( -3.152548672688508926E-16, -78.81249999863440792, -5.148502694627439702 ) ) ;
#42744=VECTOR ( 'NONE', #36665, 1000.000000000000000 ) ;
#42746=CARTESIAN_POINT ( 'NONE',  ( -4.458734124999999437, 4.687500001365595637, 0.000000000000000000 ) ) ;
#42747=LINE ( 'NONE', #14106, #63321 ) ;
#42748=CARTESIAN_POINT ( 'NONE',  ( 2.229367062500001939, -36.22916666530107221, 3.861377020970579999 ) ) ;
#42749=CARTESIAN_POINT ( 'NONE',  ( -2.500000000000000444, -4.041666663935479242, -4.330127018922193649 ) ) ;
#42751=CARTESIAN_POINT ( 'NONE',  ( -4.458734124999998549, -71.22916666530106511, 2.574251347313722516 ) ) ;
#42753=CARTESIAN_POINT ( 'NONE',  ( -2.500000000000000444, -8.166666666666669627, -4.330127018922193649 ) ) ;
#42756=CARTESIAN_POINT ( 'NONE',  ( -3.152548672688508926E-16, -65.56249999863440792, -5.148502694627439702 ) ) ;
#42757=CARTESIAN_POINT ( 'NONE',  ( 5.000000000000000888, -98.45833333060213022, 2.886751345948126879 ) ) ;
#42758=EDGE_CURVE ( 'NONE', #16611, #15979, #42968, .T. ) ;
#42762=CARTESIAN_POINT ( 'NONE',  ( -2.229367062500000163, -103.7291666653010651, -3.861377020970580443 ) ) ;
#42764=CARTESIAN_POINT ( 'NONE',  ( 2.499999999999998668, -53.33333333333332860, -4.330127018922193649 ) ) ;
#42766=DIRECTION ( 'NONE',  ( 1.000000000000000000, 0.000000000000000000, 3.614007241618347908E-17 ) ) ;
#42769=CARTESIAN_POINT ( 'NONE',  ( -2.916731409357579869E-14, 13.25000000000000178, 5.000000000000000888 ) ) ;
#42773=CARTESIAN_POINT ( 'NONE',  ( -6.972266317189433020E-16, 19.87500000273118417, -5.000000000000000000 ) ) ;
#42777=ORIENTED_EDGE ( 'NONE', *, *, #51450, .T. ) ;
#42785=CARTESIAN_POINT ( 'NONE',  ( -4.458734124999998549, -34.47916666530107221, 2.574251347313722516 ) ) ;
#42787=AXIS2_PLACEMENT_3D ( 'NONE', #49697, #5641, #8111 ) ;
#42797=CARTESIAN_POINT ( 'NONE',  ( -1.339745962155613812, -25.08034179853028789, -5.000000000000000000 ) ) ;
#42798=CARTESIAN_POINT ( 'NONE',  ( 9.457646018065525792E-16, -86.31249999863440792, 5.148502694627439702 ) ) ;
#42799=CARTESIAN_POINT ( 'NONE',  ( -6.972266317189433020E-16, -108.2499999999999858, -5.000000000000000000 ) ) ;
#42800=VERTEX_POINT ( 'NONE', #16856 ) ;
#42801=CARTESIAN_POINT ( 'NONE',  ( 1.975475456537005874E-15, -94.62499999726880162, 5.000000000000000000 ) ) ;
#42805=ORIENTED_EDGE ( 'NONE', *, *, #12741, .T. ) ;
#42807=CARTESIAN_POINT ( 'NONE',  ( 4.458734125000001214, -11.14583333196774007, 2.574251347313718519 ) ) ;
#42808=DIRECTION ( 'NONE',  ( 0.000000000000000000, 0.000000000000000000, 1.000000000000000000 ) ) ;
#42812=CARTESIAN_POINT ( 'NONE',  ( 4.458734124999998549, 28.02083333469893134, -2.574251347313721627 ) ) ;
#42814=CARTESIAN_POINT ( 'NONE',  ( 2.229367062499998831, -94.64583333196773651, -3.861377020970580887 ) ) ;
#42815=CARTESIAN_POINT ( 'NONE',  ( -5.000000000000000000, -31.08333333333332860, -2.886751345948128211 ) ) ;
#42816=CARTESIAN_POINT ( 'NONE',  ( -5.000000000000000000, -63.00000000000000000, 0.000000000000000000 ) ) ;
#42817=CARTESIAN_POINT ( 'NONE',  ( 2.229367062500001939, -7.979166665301073991, 3.861377020970579999 ) ) ;
#42818=CARTESIAN_POINT ( 'NONE',  ( 5.000000000000000000, -51.50000000000000711, -6.123233995736766282E-16 ) ) ;
#42819=CARTESIAN_POINT ( 'NONE',  ( -6.972266317189433020E-16, 14.74999999999999822, -5.000000000000000000 ) ) ;
#42820=CARTESIAN_POINT ( 'NONE',  ( 5.000000000000000000, -34.37499999726881583, -6.123233995736766282E-16 ) ) ;
#42822=CARTESIAN_POINT ( 'NONE',  ( 2.229367062499998831, 20.35416666803225993, -3.861377020970580887 ) ) ;
#42823=CARTESIAN_POINT ( 'NONE',  ( -1.339745962155610925, -97.66965819600733312, 5.000000000000000000 ) ) ;
#42825=CARTESIAN_POINT ( 'NONE',  ( 4.458734124999999437, -58.81249999863440081, -5.460374474430324690E-16 ) ) ;
#42827=AXIS2_PLACEMENT_3D ( 'NONE', #1410, #21010, #55741 ) ;
#42829=CARTESIAN_POINT ( 'NONE',  ( 5.000000000000000888, 7.416666666666665186, 2.886751345948126879 ) ) ;
#42832=CARTESIAN_POINT ( 'NONE',  ( 9.457646018065525792E-16, -49.06249999863440792, 5.148502694627439702 ) ) ;
#42833=CARTESIAN_POINT ( 'NONE',  ( 5.000000000000000000, -86.29166666393547303, -2.886751345948129988 ) ) ;
#42834=EDGE_CURVE ( 'NONE', #800, #22037, #49165, .T. ) ;
#42837=CARTESIAN_POINT ( 'NONE',  ( -4.999999999999998224, -16.91666666666666430, 2.886751345948131764 ) ) ;
#42839=AXIS2_PLACEMENT_3D ( 'NONE', #53590, #48131, #18852 ) ;
#42840=CARTESIAN_POINT ( 'NONE',  ( 4.458734124999999437, -89.06249999863439371, -5.460374474430324690E-16 ) ) ;
#42843=CARTESIAN_POINT ( 'NONE',  ( -4.999999999999999112, -38.91666666666667140, 2.886751345948131764 ) ) ;
#42847=CARTESIAN_POINT ( 'NONE',  ( 9.457646018065525792E-16, -97.06249999863439371, 5.148502694627439702 ) ) ;
#42848=CARTESIAN_POINT ( 'NONE',  ( -3.152548672688508926E-16, 6.187500001365593860, -5.148502694627439702 ) ) ;
#42849=CARTESIAN_POINT ( 'NONE',  ( 5.000000000000000000, 9.625000002731184168, -6.123233995736766282E-16 ) ) ;
#42850=CARTESIAN_POINT ( 'NONE',  ( -2.500000000000000444, -35.04166666393547303, -4.330127018922193649 ) ) ;
#42855=EDGE_CURVE ( 'NONE', #721, #53022, #31508, .T. ) ;
#42858=CARTESIAN_POINT ( 'NONE',  ( -6.972266317189433020E-16, 5.749999999999999112, -5.000000000000000000 ) ) ;
#42860=CARTESIAN_POINT ( 'NONE',  ( -2.229367062500000163, -19.72916666530107221, -3.861377020970580443 ) ) ;
#42870=ORIENTED_EDGE ( 'NONE', *, *, #3233, .T. ) ;
#42871=CARTESIAN_POINT ( 'NONE',  ( -3.152548672688508926E-16, -68.81249999863439371, -5.148502694627439702 ) ) ;
#42873=CARTESIAN_POINT ( 'NONE',  ( -1.339745962155610925, -5.669658196007334006, 5.000000000000000000 ) ) ;
#42877=VECTOR ( 'NONE', #17064, 1000.000000000000000 ) ;
#42878=CARTESIAN_POINT ( 'NONE',  ( -4.458734124999999437, -0.5624999986344053626, 0.000000000000000000 ) ) ;
#42879=ORIENTED_EDGE ( 'NONE', *, *, #10976, .T. ) ;
#42881=CARTESIAN_POINT ( 'NONE',  ( -4.458734124999999437, 4.604166668032261711, -2.574251347313719407 ) ) ;
#42886=ORIENTED_EDGE ( 'NONE', *, *, #9170, .T. ) ;
#42887=CARTESIAN_POINT ( 'NONE',  ( 4.458734124999999437, -74.81249999863440792, -5.460374474430324690E-16 ) ) ;
#42889=CARTESIAN_POINT ( 'NONE',  ( -4.458734124999999437, 9.687500001365593860, 0.000000000000000000 ) ) ;
#42890=CARTESIAN_POINT ( 'NONE',  ( -2.499999999999996447, -88.83333333333332860, 4.330127018922195425 ) ) ;
#42891=CARTESIAN_POINT ( 'NONE',  ( -3.152548672688508926E-16, -57.81249999863440081, -5.148502694627439702 ) ) ;
#42892=CARTESIAN_POINT ( 'NONE',  ( 2.500000000000002220, -20.54166666393548013, 4.330127018922192761 ) ) ;
#42893=CARTESIAN_POINT ( 'NONE',  ( -6.972266317189433020E-16, -96.12499999726880162, -5.000000000000000000 ) ) ;
#42897=FACE_OUTER_BOUND ( 'NONE', #20160, .T. ) ;
#42898=CARTESIAN_POINT ( 'NONE',  ( -2.229367062500000163, -40.47916666530107221, -3.861377020970580443 ) ) ;
#42899=CARTESIAN_POINT ( 'NONE',  ( -2.229367062499996610, -25.39583333196773651, 3.861377020970582219 ) ) ;
#42901=CARTESIAN_POINT ( 'NONE',  ( -3.535250795749689387E-16, 26.75000000000000000, -5.773502691896257311 ) ) ;
#42903=ORIENTED_EDGE ( 'NONE', *, *, #753, .F. ) ;
#42904=CARTESIAN_POINT ( 'NONE',  ( -4.458734124999999437, -108.6458333319677365, -2.574251347313719407 ) ) ;
#42905=CARTESIAN_POINT ( 'NONE',  ( 4.458734124999998549, -34.72916666530107221, -2.574251347313721627 ) ) ;
#42906=CARTESIAN_POINT ( 'NONE',  ( 1.060575238724906964E-15, -70.62499999726881583, 5.773502691896257311 ) ) ;
#42911=CARTESIAN_POINT ( 'NONE',  ( 9.457646018065525792E-16, -28.06249999863440081, 5.148502694627439702 ) ) ;
#42912=CARTESIAN_POINT ( 'NONE',  ( -4.458734124999997661, -75.47916666530106511, 2.574251347313722516 ) ) ;
#42916=FACE_OUTER_BOUND ( 'NONE', #27886, .T. ) ;
#42918=CARTESIAN_POINT ( 'NONE',  ( 5.000000000000000888, -15.58333333333333215, 2.886751345948126879 ) ) ;
#42920=ORIENTED_EDGE ( 'NONE', *, *, #47530, .T. ) ;
#42923=EDGE_CURVE ( 'NONE', #8886, #4102, #12173, .T. ) ;
#42924=CARTESIAN_POINT ( 'NONE',  ( 2.499999999999998668, 25.79166666939785202, -4.330127018922193649 ) ) ;
#42925=CARTESIAN_POINT ( 'NONE',  ( 0.000000000000000000, -120.0000000000000000, 0.000000000000000000 ) ) ;
#42928=EDGE_CURVE ( 'NONE', #38937, #33932, #33946, .T. ) ;
#42933=CARTESIAN_POINT ( 'NONE',  ( -4.999999999999998224, -80.79166666393547303, 2.886751345948131764 ) ) ;
#42936=CARTESIAN_POINT ( 'NONE',  ( 2.500000000000002220, -12.66666666666666607, 4.330127018922192761 ) ) ;
#42937=VERTEX_POINT ( 'NONE', #58225 ) ;
#42943=VERTEX_POINT ( 'NONE', #51603 ) ;
#42945=EDGE_LOOP ( 'NONE', ( #16569, #20085, #55718, #45733 ) ) ;
#42947=CARTESIAN_POINT ( 'NONE',  ( -6.972266317189433020E-16, -103.1249999972688158, -5.000000000000000000 ) ) ;
#42953=ORIENTED_EDGE ( 'NONE', *, *, #57558, .T. ) ;
#42954=CARTESIAN_POINT ( 'NONE',  ( 4.458734125000001214, -82.89583333196772230, 2.574251347313718519 ) ) ;
#42955=CARTESIAN_POINT ( 'NONE',  ( 4.458734124999999437, 19.18750000136559564, -5.460374474430324690E-16 ) ) ;
#42956=CARTESIAN_POINT ( 'NONE',  ( -5.000000000000000000, -17.87499999726881583, 0.000000000000000000 ) ) ;
#42961=CARTESIAN_POINT ( 'NONE',  ( 2.499999999999998668, -4.208333330602147981, -4.330127018922193649 ) ) ;
#42963=CARTESIAN_POINT ( 'NONE',  ( 1.339745962155615144, -13.58034179853029322, 4.999999999999999112 ) ) ;
#42964=CARTESIAN_POINT ( 'NONE',  ( -4.458734124999999437, -61.39583333196774362, -2.574251347313719407 ) ) ;
#42966=CARTESIAN_POINT ( 'NONE',  ( -4.458734124999998549, 24.77083333469893134, 2.574251347313722516 ) ) ;
#42967=VECTOR ( 'NONE', #3642, 1000.000000000000000 ) ;
#42968=( BOUNDED_CURVE ( )  B_SPLINE_CURVE ( 2, ( #53857, #9787, #5621, #10434, #4974, #44203, #19767, #54178, #39376 ),
 .UNSPECIFIED., .F., .F. ) 
 B_SPLINE_CURVE_WITH_KNOTS ( ( 3, 2, 2, 2, 3 ),
 ( 0.1339285714285714246, 0.1345238095238095177, 0.1357142857142857040, 0.1369047619047619180, 0.1375000000000000111 ),
 .UNSPECIFIED. ) 
 CURVE ( )  GEOMETRIC_REPRESENTATION_ITEM ( )  RATIONAL_B_SPLINE_CURVE ( ( 0.9330127018922194093, 0.9330127018922194093, 1.000000000000000000, 0.8660254037844387076, 1.000000000000000000, 0.8660254037844387076, 1.000000000000000000, 0.9330127018922194093, 0.9330127018922194093 ) ) 
 REPRESENTATION_ITEM ( '' )  );
#42969=CARTESIAN_POINT ( 'NONE',  ( 2.500000000000002220, -97.66666666666665719, 4.330127018922192761 ) ) ;
#42971=CARTESIAN_POINT ( 'NONE',  ( 4.458734124999999437, -44.06249999863440081, -5.460374474430324690E-16 ) ) ;
#42972=CARTESIAN_POINT ( 'NONE',  ( 5.000000000000000888, -2.458333330602146205, 2.886751345948126879 ) ) ;
#42976=CARTESIAN_POINT ( 'NONE',  ( -4.458734124999997661, -101.2291666653010651, 2.574251347313722516 ) ) ;
#42977=CARTESIAN_POINT ( 'NONE',  ( -2.229367062500000163, -12.72916666530107044, -3.861377020970580443 ) ) ;
#42980=CARTESIAN_POINT ( 'NONE',  ( -2.229367062499996610, -98.14583333196773651, 3.861377020970582219 ) ) ;
#42982=CARTESIAN_POINT ( 'NONE',  ( -4.458734124999999437, -91.64583333196773651, -2.574251347313719407 ) ) ;
#42983=CARTESIAN_POINT ( 'NONE',  ( 5.000000000000000888, -53.45833333060213732, 2.886751345948126879 ) ) ;
#42984=CARTESIAN_POINT ( 'NONE',  ( 1.975475456537005874E-15, 19.37500000273118772, 5.000000000000000000 ) ) ;
#42988=CARTESIAN_POINT ( 'NONE',  ( -2.229367062499996610, -15.14583333196773474, 3.861377020970582219 ) ) ;
#42989=CARTESIAN_POINT ( 'NONE',  ( 4.458734124999998549, 11.02083333469892779, -2.574251347313721627 ) ) ;
#42990=CARTESIAN_POINT ( 'NONE',  ( -4.458734124999999437, -58.56249999863440081, 0.000000000000000000 ) ) ;
#42994=CARTESIAN_POINT ( 'NONE',  ( 1.975475456537005874E-15, -24.62499999726881583, 5.000000000000000000 ) ) ;
#42997=DIRECTION ( 'NONE',  ( 0.000000000000000000, 0.000000000000000000, 1.000000000000000000 ) ) ;
#43000=CARTESIAN_POINT ( 'NONE',  ( 4.458734124999998549, -86.72916666530107932, -2.574251347313721627 ) ) ;
#43001=CARTESIAN_POINT ( 'NONE',  ( -2.229367062499996610, 24.60416666803225993, 3.861377020970582219 ) ) ;
#43003=CARTESIAN_POINT ( 'NONE',  ( -1.339745962155610925, -47.79465819873851729, 5.000000000000000000 ) ) ;
#43006=CARTESIAN_POINT ( 'NONE',  ( 5.000000000000000000, -68.41666666666667140, -2.886751345948129988 ) ) ;
#43009=ORIENTED_EDGE ( 'NONE', *, *, #38840, .F. ) ;
#43014=CARTESIAN_POINT ( 'NONE',  ( 1.975475456537005874E-15, -71.75000000000000000, 5.000000000000000000 ) ) ;
#43017=CARTESIAN_POINT ( 'NONE',  ( 1.339745962155600711, 18.29465819873852084, 5.000000000000007994 ) ) ;
#43018=EDGE_CURVE ( 'NONE', #41687, #15898, #4206, .T. ) ;
#43024=ORIENTED_EDGE ( 'NONE', *, *, #10605, .F. ) ;
#43027=CARTESIAN_POINT ( 'NONE',  ( 9.457646018065525792E-16, -58.31249999863440792, 5.148502694627439702 ) ) ;
#43034=ORIENTED_EDGE ( 'NONE', *, *, #7875, .F. ) ;
#43037=CARTESIAN_POINT ( 'NONE',  ( -3.152548672688508926E-16, -97.81249999863439371, -5.148502694627439702 ) ) ;
#43038=CARTESIAN_POINT ( 'NONE',  ( -1.339745962155613812, -27.08034179853029499, -5.000000000000000000 ) ) ;
#43039=ORIENTED_EDGE ( 'NONE', *, *, #19611, .F. ) ;
#43042=( BOUNDED_CURVE ( )  B_SPLINE_CURVE ( 2, ( #62957, #14050, #15000, #19187, #29461, #24023, #43627, #14366, #33990 ),
 .UNSPECIFIED., .F., .F. ) 
 B_SPLINE_CURVE_WITH_KNOTS ( ( 3, 2, 2, 2, 3 ),
 ( 0.9446428571428571175, 0.9452380952380952106, 0.9464285714285713969, 0.9476190476190475831, 0.9482142857142856762 ),
 .UNSPECIFIED. ) 
 CURVE ( )  GEOMETRIC_REPRESENTATION_ITEM ( )  RATIONAL_B_SPLINE_CURVE ( ( 0.9330127018922194093, 0.9330127018922194093, 1.000000000000000000, 0.8660254037844387076, 1.000000000000000000, 0.8660254037844387076, 1.000000000000000000, 0.9330127018922194093, 0.9330127018922194093 ) ) 
 REPRESENTATION_ITEM ( '' )  );
#43043=CARTESIAN_POINT ( 'NONE',  ( -1.339745962155613812, 0.9196582014697067819, -5.000000000000000000 ) ) ;
#43044=CARTESIAN_POINT ( 'NONE',  ( 9.457646018065525792E-16, -10.06249999863440792, 5.148502694627439702 ) ) ;
#43045=CARTESIAN_POINT ( 'NONE',  ( 2.229367062500001939, -102.2291666653010651, 3.861377020970579999 ) ) ;
#43047=CARTESIAN_POINT ( 'NONE',  ( -2.229367062500000163, -29.72916666530107221, -3.861377020970580443 ) ) ;
#43048=CARTESIAN_POINT ( 'NONE',  ( -6.972266317189433020E-16, -80.24999999999998579, -5.000000000000000000 ) ) ;
#43051=CARTESIAN_POINT ( 'NONE',  ( 0.000000000000000000, -120.0000000000000000, 5.000000000000000000 ) ) ;
#43052=CARTESIAN_POINT ( 'NONE',  ( -6.972266317189433020E-16, -22.12499999726881228, -5.000000000000000000 ) ) ;
#43054=AXIS2_PLACEMENT_3D ( 'NONE', #62200, #38367, #13919 ) ;
#43055=CARTESIAN_POINT ( 'NONE',  ( -4.458734124999999437, 4.437500001365595637, 0.000000000000000000 ) ) ;
#43056=ORIENTED_EDGE ( 'NONE', *, *, #4706, .F. ) ;
#43059=CARTESIAN_POINT ( 'NONE',  ( 5.000000000000000000, -91.50000000000000000, -6.123233995736766282E-16 ) ) ;
#43060=CARTESIAN_POINT ( 'NONE',  ( 4.458734124999999437, -30.81249999863440436, -5.460374474430324690E-16 ) ) ;
#43062=CARTESIAN_POINT ( 'NONE',  ( -4.458734124999998549, -76.47916666530105090, 2.574251347313722516 ) ) ;
#43066=CARTESIAN_POINT ( 'NONE',  ( -2.229367062499996610, 4.854166668032261711, 3.861377020970582219 ) ) ;
#43067=CARTESIAN_POINT ( 'NONE',  ( 2.229367062500001939, 26.77083333469892423, 3.861377020970579999 ) ) ;
#43068=CARTESIAN_POINT ( 'NONE',  ( 4.458734124999999437, -40.06249999863440081, -5.460374474430324690E-16 ) ) ;
#43072=( BOUNDED_CURVE ( )  B_SPLINE_CURVE ( 2, ( #6555, #1749, #45468, #21674, #11682 ),
 .UNSPECIFIED., .F., .F. ) 
 B_SPLINE_CURVE_WITH_KNOTS ( ( 3, 2, 3 ),
 ( 0.9982142857142857206, 0.9988095238095238138, 1.000000000000000000 ),
 .UNSPECIFIED. ) 
 CURVE ( )  GEOMETRIC_REPRESENTATION_ITEM ( )  RATIONAL_B_SPLINE_CURVE ( ( 0.9330127018922194093, 0.9330127018922194093, 1.000000000000000000, 0.8660254037844387076, 1.000000000000000000 ) ) 
 REPRESENTATION_ITEM ( '' )  );
#43074=CARTESIAN_POINT ( 'NONE',  ( -2.229367062499996610, -67.14583333196773651, 3.861377020970582219 ) ) ;
#43075=CARTESIAN_POINT ( 'NONE',  ( -4.999999999999999112, -99.79166666393545881, 2.886751345948131764 ) ) ;
#43077=CARTESIAN_POINT ( 'NONE',  ( 1.339745962155615144, 9.419658201469706782, 4.999999999999999112 ) ) ;
#43078=CARTESIAN_POINT ( 'NONE',  ( 2.229367062500001939, -106.2291666653010651, 3.861377020970579999 ) ) ;
#43080=CARTESIAN_POINT ( 'NONE',  ( 2.500000000000002220, -51.66666666666666430, 4.330127018922192761 ) ) ;
#43084=CARTESIAN_POINT ( 'NONE',  ( 4.458734125000001214, -109.8958333319677365, 2.574251347313718519 ) ) ;
#43092=ORIENTED_EDGE ( 'NONE', *, *, #46502, .F. ) ;
#43093=FACE_OUTER_BOUND ( 'NONE', #10762, .T. ) ;
#43099=CARTESIAN_POINT ( 'NONE',  ( -2.229367062500000163, -35.72916666530107221, -3.861377020970580443 ) ) ;
#43101=DIRECTION ( 'NONE',  ( -0.000000000000000000, 1.000000000000000000, -0.000000000000000000 ) ) ;
#43107=CARTESIAN_POINT ( 'NONE',  ( 1.339745962155615144, -54.70534180126148271, 4.999999999999999112 ) ) ;
#43109=CARTESIAN_POINT ( 'NONE',  ( 2.229367062499998831, -81.89583333196773651, -3.861377020970580887 ) ) ;
#43113=CARTESIAN_POINT ( 'NONE',  ( -6.972266317189433020E-16, -44.25000000000000000, -5.000000000000000000 ) ) ;
#43115=EDGE_CURVE ( 'NONE', #16789, #49905, #44651, .T. ) ;
#43116=EDGE_LOOP ( 'NONE', ( #43243, #309, #2528, #6926 ) ) ;
#43118=CARTESIAN_POINT ( 'NONE',  ( 4.458734125000001214, -13.14583333196774184, 2.574251347313718519 ) ) ;
#43119=DIRECTION ( 'NONE',  ( -0.000000000000000000, 1.000000000000000000, -0.000000000000000000 ) ) ;
#43121=CARTESIAN_POINT ( 'NONE',  ( 5.000000000000000888, -77.45833333060213022, 2.886751345948126879 ) ) ;
#43123=CARTESIAN_POINT ( 'NONE',  ( 4.458734125000000326, 23.85416666803225993, 2.574251347313718519 ) ) ;
#43124=VERTEX_POINT ( 'NONE', #30536 ) ;
#43125=CARTESIAN_POINT ( 'NONE',  ( 4.458734124999999437, -91.81249999863440792, -5.460374474430324690E-16 ) ) ;
#43126=CARTESIAN_POINT ( 'NONE',  ( 2.499999999999998668, -47.33333333333333570, -4.330127018922193649 ) ) ;
#43127=CARTESIAN_POINT ( 'NONE',  ( 1.975475456537005874E-15, -103.6249999972687874, 5.000000000000000000 ) ) ;
#43128=CARTESIAN_POINT ( 'NONE',  ( -2.229367062499996610, -8.145833331967736513, 3.861377020970582219 ) ) ;
#43129=CARTESIAN_POINT ( 'NONE',  ( -1.339745962155610925, -84.66965819600731891, 5.000000000000000000 ) ) ;
#43130=CARTESIAN_POINT ( 'NONE',  ( 4.769696007084728073, -120.0000000000000000, 1.500000000000000000 ) ) ;
#43132=CARTESIAN_POINT ( 'NONE',  ( -2.499999999999996447, -34.70833333060213732, 4.330127018922195425 ) ) ;
#43134=CARTESIAN_POINT ( 'NONE',  ( -4.458734124999999437, 20.60416666803225993, -2.574251347313719407 ) ) ;
#43137=CARTESIAN_POINT ( 'NONE',  ( 4.458734125000001214, -56.89583333196774362, 2.574251347313718519 ) ) ;
#43140=CARTESIAN_POINT ( 'NONE',  ( 2.500000000000002220, 8.333333333333332149, 4.330127018922192761 ) ) ;
#43144=CARTESIAN_POINT ( 'NONE',  ( -2.229367062499996610, -47.14583333196774362, 3.861377020970582219 ) ) ;
#43145=CARTESIAN_POINT ( 'NONE',  ( -3.535250795749689387E-16, -83.12499999726880162, -5.773502691896257311 ) ) ;
#43147=CARTESIAN_POINT ( 'NONE',  ( -2.500000000000000444, -17.16666666666666430, -4.330127018922193649 ) ) ;
#43148=CARTESIAN_POINT ( 'NONE',  ( 0.000000000000000000, -120.0000000000000000, 5.000000000000000000 ) ) ;
#43149=CARTESIAN_POINT ( 'NONE',  ( 4.458734125000000326, -89.14583333196773651, 2.574251347313718519 ) ) ;
#43151=CARTESIAN_POINT ( 'NONE',  ( 2.499999999999998668, -37.33333333333332860, -4.330127018922193649 ) ) ;
#43153=ORIENTED_EDGE ( 'NONE', *, *, #54428, .F. ) ;
#43154=CARTESIAN_POINT ( 'NONE',  ( 5.000000000000000000, -22.41666666666666785, -2.886751345948130876 ) ) ;
#43156=CARTESIAN_POINT ( 'NONE',  ( 4.458734124999998549, -96.72916666530105090, -2.574251347313721627 ) ) ;
#43157=CARTESIAN_POINT ( 'NONE',  ( 2.229367062500001939, 10.77083333469892956, 3.861377020970579999 ) ) ;
#43158=CARTESIAN_POINT ( 'NONE',  ( 5.000000000000000000, 12.70833333606451809, -2.886751345948129988 ) ) ;
#43168=CARTESIAN_POINT ( 'NONE',  ( 5.000000000000000000, -19.41666666666666785, -2.886751345948130876 ) ) ;
#43171=CARTESIAN_POINT ( 'NONE',  ( 4.458734124999998549, -20.97916666530107221, -2.574251347313721627 ) ) ;
#43181=ORIENTED_EDGE ( 'NONE', *, *, #62273, .T. ) ;
#43182=CARTESIAN_POINT ( 'NONE',  ( -2.229367062499996610, -70.39583333196773651, 3.861377020970582219 ) ) ;
#43184=CARTESIAN_POINT ( 'NONE',  ( -1.339745962155613812, -6.080341798530292330, -5.000000000000000000 ) ) ;
#43190=CARTESIAN_POINT ( 'NONE',  ( 4.458734124999998549, 1.020833334698927120, -2.574251347313721627 ) ) ;
#43191=ORIENTED_EDGE ( 'NONE', *, *, #39783, .T. ) ;
#43192=CARTESIAN_POINT ( 'NONE',  ( -2.500000000000000444, -55.16666666666667140, -4.330127018922193649 ) ) ;
#43198=CARTESIAN_POINT ( 'NONE',  ( 2.229367062499998831, -73.64583333196773651, -3.861377020970580887 ) ) ;
#43199=EDGE_CURVE ( 'NONE', #25684, #10189, #54672, .T. ) ;
#43201=CARTESIAN_POINT ( 'NONE',  ( 2.229367062499998831, 8.354166668032261711, -3.861377020970580887 ) ) ;
#43202=CARTESIAN_POINT ( 'NONE',  ( -2.229367062500000163, -59.72916666530106511, -3.861377020970580443 ) ) ;
#43203=CARTESIAN_POINT ( 'NONE',  ( -5.000000000000000000, -19.95833333060214798, -2.886751345948128211 ) ) ;
#43206=FACE_OUTER_BOUND ( 'NONE', #37058, .T. ) ;
#43208=( BOUNDED_CURVE ( )  B_SPLINE_CURVE ( 2, ( #16779, #56353, #56027, #11944, #17098, #57301, #12584, #51204, #37039 ),
 .UNSPECIFIED., .F., .F. ) 
 B_SPLINE_CURVE_WITH_KNOTS ( ( 3, 2, 2, 2, 3 ),
 ( 0.1875000000000000000, 0.1880952380952380931, 0.1892857142857142794, 0.1904761904761904656, 0.1910714285714285865 ),
 .UNSPECIFIED. ) 
 CURVE ( )  GEOMETRIC_REPRESENTATION_ITEM ( )  RATIONAL_B_SPLINE_CURVE ( ( 0.9330127018922194093, 0.9330127018922194093, 1.000000000000000000, 0.8660254037844387076, 1.000000000000000000, 0.8660254037844387076, 1.000000000000000000, 0.9330127018922178550, 0.9330127018922194093 ) ) 
 REPRESENTATION_ITEM ( '' )  );
#43210=CARTESIAN_POINT ( 'NONE',  ( 6.123233995736766282E-16, -120.0000000000000000, -5.000000000000000000 ) ) ;
#43211=CARTESIAN_POINT ( 'NONE',  ( 9.457646018065525792E-16, -38.06249999863441502, 5.148502694627439702 ) ) ;
#43212=CARTESIAN_POINT ( 'NONE',  ( -4.458734124999997661, -26.47916666530107221, 2.574251347313722516 ) ) ;
#43215=CARTESIAN_POINT ( 'NONE',  ( 2.499999999999998668, 26.66666666666666430, -4.330127018922193649 ) ) ;
#43218=CARTESIAN_POINT ( 'NONE',  ( -4.458734124999999437, -106.5624999986343937, 0.000000000000000000 ) ) ;
#43219=CARTESIAN_POINT ( 'NONE',  ( 9.457646018065525792E-16, -31.06249999863440436, 5.148502694627439702 ) ) ;
#43220=CARTESIAN_POINT ( 'NONE',  ( -5.000000000000000000, -69.87499999726880162, 0.000000000000000000 ) ) ;
#43223=CARTESIAN_POINT ( 'NONE',  ( 2.229367062499998831, -72.89583333196773651, -3.861377020970580887 ) ) ;
#43226=CARTESIAN_POINT ( 'NONE',  ( -5.000000000000000000, -27.95833333060214798, -2.886751345948128211 ) ) ;
#43227=DIRECTION ( 'NONE',  ( -0.000000000000000000, 1.000000000000000000, -0.000000000000000000 ) ) ;
#43228=CARTESIAN_POINT ( 'NONE',  ( -5.000000000000000000, -19.99999999999999645, 0.000000000000000000 ) ) ;
#43230=ORIENTED_EDGE ( 'NONE', *, *, #30367, .F. ) ;
#43232=CARTESIAN_POINT ( 'NONE',  ( -5.000000000000000000, 27.12500000273118772, 0.000000000000000000 ) ) ;
#43235=FACE_OUTER_BOUND ( 'NONE', #59394, .T. ) ;
#43237=CARTESIAN_POINT ( 'NONE',  ( -6.972266317189433020E-16, 7.750000000000000000, -5.000000000000000000 ) ) ;
#43238=EDGE_CURVE ( 'NONE', #48396, #41928, #57826, .T. ) ;
#43241=( BOUNDED_CURVE ( )  B_SPLINE_CURVE ( 2, ( #8841, #61941, #13666, #22704, #23643, #18496, #61623, #62879, #18791 ),
 .UNSPECIFIED., .F., .F. ) 
 B_SPLINE_CURVE_WITH_KNOTS ( ( 3, 2, 2, 2, 3 ),
 ( 0.008928571428571429811, 0.009523809523809524669, 0.01071428571428571438, 0.01190476190476190410, 0.01250000000000000069 ),
 .UNSPECIFIED. ) 
 CURVE ( )  GEOMETRIC_REPRESENTATION_ITEM ( )  RATIONAL_B_SPLINE_CURVE ( ( 0.9330127018922192983, 0.9330127018922194093, 1.000000000000000000, 0.8660254037844387076, 1.000000000000000000, 0.8660254037844387076, 1.000000000000000000, 0.9330127018922191873, 0.9330127018922192983 ) ) 
 REPRESENTATION_ITEM ( '' )  );
#43243=ORIENTED_EDGE ( 'NONE', *, *, #7490, .F. ) ;
#43244=CARTESIAN_POINT ( 'NONE',  ( 5.000000000000000000, 0.5000000000000004441, -6.123233995736766282E-16 ) ) ;
#43250=ORIENTED_EDGE ( 'NONE', *, *, #10696, .T. ) ;
#43251=CARTESIAN_POINT ( 'NONE',  ( 1.975475456537005874E-15, -87.75000000000001421, 5.000000000000000000 ) ) ;
#43252=CARTESIAN_POINT ( 'NONE',  ( -1.339745962155613812, -103.0803417985302843, -5.000000000000000000 ) ) ;
#43255=( BOUNDED_CURVE ( )  B_SPLINE_CURVE ( 2, ( #31366, #47131, #41976, #3079, #7583, #41647, #51007, #46498, #22698 ),
 .UNSPECIFIED., .F., .F. ) 
 B_SPLINE_CURVE_WITH_KNOTS ( ( 3, 2, 2, 2, 3 ),
 ( 0.8267857142857142350, 0.8273809523809523281, 0.8285714285714286254, 0.8297619047619048116, 0.8303571428571429047 ),
 .UNSPECIFIED. ) 
 CURVE ( )  GEOMETRIC_REPRESENTATION_ITEM ( )  RATIONAL_B_SPLINE_CURVE ( ( 0.9330127018922194093, 0.9330127018922194093, 1.000000000000000000, 0.8660254037844387076, 1.000000000000000000, 0.8660254037844387076, 1.000000000000000000, 0.9330127018922194093, 0.9330127018922194093 ) ) 
 REPRESENTATION_ITEM ( '' )  );
#43256=DIRECTION ( 'NONE',  ( 0.000000000000000000, 0.000000000000000000, 1.000000000000000000 ) ) ;
#43258=CARTESIAN_POINT ( 'NONE',  ( 1.339745962155612702, -53.16965819600733312, -5.000000000000000000 ) ) ;
#43262=EDGE_CURVE ( 'NONE', #9578, #20024, #40147, .T. ) ;
#43263=CARTESIAN_POINT ( 'NONE',  ( 4.458734125000001214, -83.89583333196773651, 2.574251347313718519 ) ) ;
#43264=CARTESIAN_POINT ( 'NONE',  ( 9.457646018065525792E-16, 16.93750000136559564, 5.148502694627439702 ) ) ;
#43266=ADVANCED_FACE ( 'NONE', ( #34730 ), #25727, .T. ) ;
#43271=CARTESIAN_POINT ( 'NONE',  ( 1.975475456537005874E-15, -4.624999997268815832, 5.000000000000000000 ) ) ;
#43273=CARTESIAN_POINT ( 'NONE',  ( 5.000000000000000000, -13.29166666393548191, -2.886751345948130876 ) ) ;
#43274=CARTESIAN_POINT ( 'NONE',  ( -4.458734124999997661, -62.22916666530105090, 2.574251347313722516 ) ) ;
#43276=AXIS2_PLACEMENT_3D ( 'NONE', #48479, #4416, #38814 ) ;
#43277=CARTESIAN_POINT ( 'NONE',  ( 4.458734125000001214, 23.10416666803225993, 2.574251347313718519 ) ) ;
#43279=CARTESIAN_POINT ( 'NONE',  ( 1.339745962155615144, -42.70534180126148982, 4.999999999999999112 ) ) ;
#43281=CARTESIAN_POINT ( 'NONE',  ( -4.458734124999998549, -45.47916666530105800, 2.574251347313722516 ) ) ;
#43282=CARTESIAN_POINT ( 'NONE',  ( -2.499999999999996447, -6.708333330602149758, 4.330127018922195425 ) ) ;
#43284=EDGE_CURVE ( 'NONE', #60011, #51908, #41632, .T. ) ;
#43287=CARTESIAN_POINT ( 'NONE',  ( -4.458734124999999437, -105.3958333319677365, -2.574251347313719407 ) ) ;
#43288=CARTESIAN_POINT ( 'NONE',  ( 4.458734124999998549, -8.979166665301075767, -2.574251347313721627 ) ) ;
#43290=CARTESIAN_POINT ( 'NONE',  ( 1.339745962155615144, -52.70534180126147561, 4.999999999999999112 ) ) ;
#43291=CARTESIAN_POINT ( 'NONE',  ( 9.457646018065525792E-16, -99.06249999863440792, 5.148502694627439702 ) ) ;
#43292=EDGE_CURVE ( 'NONE', #58774, #9375, #18735, .T. ) ;
#43294=CARTESIAN_POINT ( 'NONE',  ( -4.458734124999999437, -89.56249999863440792, 0.000000000000000000 ) ) ;
#43295=CARTESIAN_POINT ( 'NONE',  ( 5.000000000000000888, -54.45833333060214443, 2.886751345948126879 ) ) ;
#43299=CARTESIAN_POINT ( 'NONE',  ( -2.229367062499996610, -13.14583333196774007, 3.861377020970582219 ) ) ;
#43300=CARTESIAN_POINT ( 'NONE',  ( 9.457646018065525792E-16, 13.68750000136559208, 5.148502694627439702 ) ) ;
#43301=CARTESIAN_POINT ( 'NONE',  ( 4.458734125000000326, -58.14583333196773651, 2.574251347313718519 ) ) ;
#43303=DIRECTION ( 'NONE',  ( -0.000000000000000000, 1.000000000000000000, -0.000000000000000000 ) ) ;
#43306=ORIENTED_EDGE ( 'NONE', *, *, #57454, .T. ) ;
#43309=CARTESIAN_POINT ( 'NONE',  ( 1.975475456537005874E-15, -37.74999999999999289, 5.000000000000000000 ) ) ;
#43310=CARTESIAN_POINT ( 'NONE',  ( 2.499999999999998668, -66.33333333333332860, -4.330127018922193649 ) ) ;
#43311=CARTESIAN_POINT ( 'NONE',  ( -5.000000000000000000, -66.95833333060214443, -2.886751345948128211 ) ) ;
#43312=CARTESIAN_POINT ( 'NONE',  ( 4.458734124999998549, -87.72916666530107932, -2.574251347313721627 ) ) ;
#43313=CARTESIAN_POINT ( 'NONE',  ( -3.152548672688508926E-16, 18.18750000136559564, -5.148502694627439702 ) ) ;
#43315=CARTESIAN_POINT ( 'NONE',  ( -5.000000000000000000, -48.08333333333332860, -2.886751345948128211 ) ) ;
#43318=CARTESIAN_POINT ( 'NONE',  ( 5.000000000000000000, -69.41666666666667140, -2.886751345948129988 ) ) ;
#43321=CARTESIAN_POINT ( 'NONE',  ( 1.975475456537005874E-15, -79.74999999999998579, 5.000000000000000000 ) ) ;
#43327=VERTEX_POINT ( 'NONE', #30211 ) ;
#43333=CARTESIAN_POINT ( 'NONE',  ( -4.458734124999999437, -57.56249999863440081, 0.000000000000000000 ) ) ;
#43335=CARTESIAN_POINT ( 'NONE',  ( 1.975475456537005874E-15, -19.62499999726881228, 5.000000000000000000 ) ) ;
#43341=( BOUNDED_CURVE ( )  B_SPLINE_CURVE ( 2, ( #61871, #3013, #42227, #8460, #37105, #17484, #52525, #56724, #7514 ),
 .UNSPECIFIED., .F., .F. ) 
 B_SPLINE_CURVE_WITH_KNOTS ( ( 3, 2, 2, 2, 3 ),
 ( 0.3910714285714285698, 0.3916666666666666630, 0.3928571428571428492, 0.3940476190476190355, 0.3946428571428571286 ),
 .UNSPECIFIED. ) 
 CURVE ( )  GEOMETRIC_REPRESENTATION_ITEM ( )  RATIONAL_B_SPLINE_CURVE ( ( 0.9330127018922194093, 0.9330127018922194093, 1.000000000000000000, 0.8660254037844387076, 1.000000000000000000, 0.8660254037844387076, 1.000000000000000000, 0.9330127018922194093, 0.9330127018922194093 ) ) 
 REPRESENTATION_ITEM ( '' )  );
#43345=CARTESIAN_POINT ( 'NONE',  ( -3.152548672688508926E-16, -104.8124999986344079, -5.148502694627439702 ) ) ;
#43347=ORIENTED_EDGE ( 'NONE', *, *, #15409, .F. ) ;
#43350=CARTESIAN_POINT ( 'NONE',  ( 4.458734124999998549, -39.72916666530107221, -2.574251347313721627 ) ) ;
#43352=CARTESIAN_POINT ( 'NONE',  ( -4.458734124999998549, -14.22916666530107221, 2.574251347313722516 ) ) ;
#43353=CARTESIAN_POINT ( 'NONE',  ( 2.229367062500001939, -99.22916666530105090, 3.861377020970579999 ) ) ;
#43356=CARTESIAN_POINT ( 'NONE',  ( -3.152548672688508926E-16, -25.81249999863440792, -5.148502694627439702 ) ) ;
#43360=EDGE_CURVE ( 'NONE', #59975, #22959, #41452, .T. ) ;
#43361=DIRECTION ( 'NONE',  ( -0.000000000000000000, 1.000000000000000000, -0.000000000000000000 ) ) ;
#43364=CARTESIAN_POINT ( 'NONE',  ( -4.458734124999999437, 5.437500001365592972, 0.000000000000000000 ) ) ;
#43365=VERTEX_POINT ( 'NONE', #31484 ) ;
#43368=CARTESIAN_POINT ( 'NONE',  ( -6.972266317189433020E-16, 15.87500000273118417, -5.000000000000000000 ) ) ;
#43369=CARTESIAN_POINT ( 'NONE',  ( -2.500000000000000444, -97.16666666666665719, -4.330127018922193649 ) ) ;
#43370=CARTESIAN_POINT ( 'NONE',  ( 4.458734124999998549, -31.72916666530107577, -2.574251347313721627 ) ) ;
#43371=CARTESIAN_POINT ( 'NONE',  ( -4.999999999999998224, -76.79166666393547303, 2.886751345948131764 ) ) ;
#43372=CARTESIAN_POINT ( 'NONE',  ( 4.458734125000001214, -74.14583333196773651, 2.574251347313718519 ) ) ;
#43377=CARTESIAN_POINT ( 'NONE',  ( -3.152548672688508926E-16, 3.437500001365594748, -5.148502694627439702 ) ) ;
#43378=CARTESIAN_POINT ( 'NONE',  ( -4.458734124999999437, 28.43750000136559208, 0.000000000000000000 ) ) ;
#43379=CARTESIAN_POINT ( 'NONE',  ( 4.458734124999998549, -43.97916666530106511, -2.574251347313721627 ) ) ;
#43384=CARTESIAN_POINT ( 'NONE',  ( 9.457646018065525792E-16, -68.06249999863440792, 5.148502694627439702 ) ) ;
#43385=CARTESIAN_POINT ( 'NONE',  ( -4.999999999999999112, -106.7916666639354730, 2.886751345948131764 ) ) ;
#43387=DIRECTION ( 'NONE',  ( 0.000000000000000000, 0.000000000000000000, 1.000000000000000000 ) ) ;
#43388=CARTESIAN_POINT ( 'NONE',  ( 4.458734124999999437, -104.0624999986344079, -5.460374474430324690E-16 ) ) ;
#43390=CARTESIAN_POINT ( 'NONE',  ( -2.500000000000000444, -55.16666666666667140, -4.330127018922193649 ) ) ;
#43393=ORIENTED_EDGE ( 'NONE', *, *, #28841, .F. ) ;
#43395=CARTESIAN_POINT ( 'NONE',  ( -6.972266317189433020E-16, -27.12499999726881228, -5.000000000000000000 ) ) ;
#43402=ORIENTED_EDGE ( 'NONE', *, *, #31536, .T. ) ;
#43409=CARTESIAN_POINT ( 'NONE',  ( -4.458734124999998549, -40.47916666530107221, 2.574251347313722516 ) ) ;
#43411=( BOUNDED_CURVE ( )  B_SPLINE_CURVE ( 2, ( #21241, #1010, #15465, #35083, #19956, #45364, #49859, #55349, #11263 ),
 .UNSPECIFIED., .F., .F. ) 
 B_SPLINE_CURVE_WITH_KNOTS ( ( 3, 2, 2, 2, 3 ),
 ( 0.2696428571428571286, 0.2702380952380952217, 0.2714285714285714080, 0.2726190476190475942, 0.2732142857142857428 ),
 .UNSPECIFIED. ) 
 CURVE ( )  GEOMETRIC_REPRESENTATION_ITEM ( )  RATIONAL_B_SPLINE_CURVE ( ( 0.9330127018922194093, 0.9330127018922194093, 1.000000000000000000, 0.8660254037844387076, 1.000000000000000000, 0.8660254037844387076, 1.000000000000000000, 0.9330127018922163007, 0.9330127018922194093 ) ) 
 REPRESENTATION_ITEM ( '' )  );
#43417=EDGE_CURVE ( 'NONE', #58830, #39750, #2253, .T. ) ;
#43418=CARTESIAN_POINT ( 'NONE',  ( -4.999999999999998224, -24.79166666393548368, 2.886751345948131764 ) ) ;
#43420=CARTESIAN_POINT ( 'NONE',  ( 4.458734124999998549, -90.97916666530106511, -2.574251347313721627 ) ) ;
#43421=CARTESIAN_POINT ( 'NONE',  ( 1.339745962155615144, -108.7053418012614543, 4.999999999999999112 ) ) ;
#43423=CARTESIAN_POINT ( 'NONE',  ( -2.499999999999996447, 27.29166666939785202, 4.330127018922195425 ) ) ;
#43429=FACE_OUTER_BOUND ( 'NONE', #37041, .T. ) ;
#43430=CARTESIAN_POINT ( 'NONE',  ( 4.458734124999999437, -13.06249999863440259, -5.460374474430324690E-16 ) ) ;
#43436=CARTESIAN_POINT ( 'NONE',  ( -3.152548672688508926E-16, 21.18750000136559208, -5.148502694627439702 ) ) ;
#43437=ORIENTED_EDGE ( 'NONE', *, *, #21651, .T. ) ;
#43438=CARTESIAN_POINT ( 'NONE',  ( 2.229367062499998831, -93.64583333196772230, -3.861377020970580887 ) ) ;
#43439=CARTESIAN_POINT ( 'NONE',  ( 1.975475456537005874E-15, -47.74999999999999289, 5.000000000000000000 ) ) ;
#43441=CARTESIAN_POINT ( 'NONE',  ( 2.229367062500001939, -15.97916666530107399, 3.861377020970579999 ) ) ;
#43442=CARTESIAN_POINT ( 'NONE',  ( -2.500000000000000444, -85.04166666393547303, -4.330127018922193649 ) ) ;
#43443=CARTESIAN_POINT ( 'NONE',  ( -4.999999999999998224, -72.91666666666667140, 2.886751345948131764 ) ) ;
#43445=CARTESIAN_POINT ( 'NONE',  ( -5.000000000000000000, -42.87499999726880873, 0.000000000000000000 ) ) ;
#43447=CARTESIAN_POINT ( 'NONE',  ( -2.229367062499996610, 17.85416666803225993, 3.861377020970582219 ) ) ;
#43448=CARTESIAN_POINT ( 'NONE',  ( 2.499999999999998668, -51.20833333060213732, -4.330127018922193649 ) ) ;
#43450=CARTESIAN_POINT ( 'NONE',  ( 2.229367062500001939, -58.97916666530106511, 3.861377020970579999 ) ) ;
#43453=CARTESIAN_POINT ( 'NONE',  ( 5.000000000000000000, 9.499999999999998224, -6.123233995736766282E-16 ) ) ;
#43456=CARTESIAN_POINT ( 'NONE',  ( 4.458734124999999437, -52.81249999863440792, -5.460374474430324690E-16 ) ) ;
#43457=CARTESIAN_POINT ( 'NONE',  ( -4.999999999999999112, -83.79166666393547303, 2.886751345948131764 ) ) ;
#43459=CARTESIAN_POINT ( 'NONE',  ( 1.975475456537005874E-15, -33.62499999726880873, 5.000000000000000000 ) ) ;
#43461=CARTESIAN_POINT ( 'NONE',  ( -2.229367062500000163, -92.72916666530106511, -3.861377020970580443 ) ) ;
#43463=CARTESIAN_POINT ( 'NONE',  ( 5.000000000000000000, -38.49999999999999289, -6.123233995736766282E-16 ) ) ;
#43467=CARTESIAN_POINT ( 'NONE',  ( 4.458734125000001214, -102.8958333319677365, 2.574251347313718519 ) ) ;
#43468=CARTESIAN_POINT ( 'NONE',  ( -4.458734124999999437, 9.354166668032261711, -2.574251347313719407 ) ) ;
#43469=CARTESIAN_POINT ( 'NONE',  ( 5.000000000000000888, 13.54166666939785202, 2.886751345948126879 ) ) ;
#43474=VECTOR ( 'NONE', #58149, 1000.000000000000000 ) ;
#43482=CARTESIAN_POINT ( 'NONE',  ( 2.499999999999998668, 6.791666669397851130, -4.330127018922193649 ) ) ;
#43483=CARTESIAN_POINT ( 'NONE',  ( -3.152548672688508926E-16, -26.81249999863440436, -5.148502694627439702 ) ) ;
#43491=ORIENTED_EDGE ( 'NONE', *, *, #6627, .T. ) ;
#43492=CARTESIAN_POINT ( 'NONE',  ( 5.000000000000000000, -93.29166666393547303, -2.886751345948130876 ) ) ;
#43493=VERTEX_POINT ( 'NONE', #17482 ) ;
#43494=CARTESIAN_POINT ( 'NONE',  ( -2.229367062500000163, -69.72916666530107932, -3.861377020970580443 ) ) ;
#43496=VERTEX_POINT ( 'NONE', #2068 ) ;
#43497=PLANE ( 'NONE',  #13517 ) ;
#43500=CARTESIAN_POINT ( 'NONE',  ( 4.458734125000001214, 3.854166668032260823, 2.574251347313718519 ) ) ;
#43505=CARTESIAN_POINT ( 'NONE',  ( -6.972266317189433020E-16, -92.12499999726878741, -5.000000000000000000 ) ) ;
#43507=ORIENTED_EDGE ( 'NONE', *, *, #32707, .T. ) ;
#43508=CARTESIAN_POINT ( 'NONE',  ( 4.458734124999998549, -76.72916666530106511, -2.574251347313721627 ) ) ;
#43510=CARTESIAN_POINT ( 'NONE',  ( -2.229367062499996610, 2.854166668032259935, 3.861377020970582219 ) ) ;
#43512=CARTESIAN_POINT ( 'NONE',  ( 4.458734124999998549, -62.97916666530107221, -2.574251347313721627 ) ) ;
#43513=CARTESIAN_POINT ( 'NONE',  ( 5.000000000000000000, -18.29166666393548013, -2.886751345948129988 ) ) ;
#43514=CARTESIAN_POINT ( 'NONE',  ( 1.975475456537005874E-15, 20.24999999999999645, 5.000000000000000000 ) ) ;
#43515=DIRECTION ( 'NONE',  ( -0.000000000000000000, 1.000000000000000000, -0.000000000000000000 ) ) ;
#43516=CARTESIAN_POINT ( 'NONE',  ( -5.000000000000000000, -59.00000000000000000, 0.000000000000000000 ) ) ;
#43518=CARTESIAN_POINT ( 'NONE',  ( 5.000000000000000000, -43.29166666393548013, -2.886751345948130876 ) ) ;
#43519=CARTESIAN_POINT ( 'NONE',  ( 9.457646018065525792E-16, -41.06249999863440792, 5.148502694627439702 ) ) ;
#43521=CARTESIAN_POINT ( 'NONE',  ( 2.229367062499998831, -26.89583333196774007, -3.861377020970580887 ) ) ;
#43524=CARTESIAN_POINT ( 'NONE',  ( -2.500000000000000444, 27.83333333333333215, -4.330127018922193649 ) ) ;
#43526=CARTESIAN_POINT ( 'NONE',  ( 4.458734125000001214, -108.1458333319677365, 2.574251347313718519 ) ) ;
#43527=CARTESIAN_POINT ( 'NONE',  ( 4.458734124999998549, -35.72916666530107221, -2.574251347313721627 ) ) ;
#43528=CARTESIAN_POINT ( 'NONE',  ( -2.499999999999996447, -69.70833333060214443, 4.330127018922195425 ) ) ;
#43532=CARTESIAN_POINT ( 'NONE',  ( -4.458734124999999437, -73.56249999863439371, 0.000000000000000000 ) ) ;
#43536=CARTESIAN_POINT ( 'NONE',  ( 1.975475456537005874E-15, -107.6249999972687874, 5.000000000000000000 ) ) ;
#43537=CARTESIAN_POINT ( 'NONE',  ( 5.000000000000000000, -21.50000000000000000, -6.123233995736766282E-16 ) ) ;
#43539=ORIENTED_EDGE ( 'NONE', *, *, #28390, .T. ) ;
#43541=CARTESIAN_POINT ( 'NONE',  ( -1.339745962155610925, -78.66965819600731891, 5.000000000000000000 ) ) ;
#43543=CARTESIAN_POINT ( 'NONE',  ( -2.500000000000000444, 28.95833333606451987, -4.330127018922193649 ) ) ;
#43546=EDGE_CURVE ( 'NONE', #27379, #942, #40904, .T. ) ;
#43552=CARTESIAN_POINT ( 'NONE',  ( 4.458734124999998549, -19.72916666530107221, -2.574251347313721627 ) ) ;
#43561=VERTEX_POINT ( 'NONE', #7512 ) ;
#43564=ORIENTED_EDGE ( 'NONE', *, *, #37702, .F. ) ;
#43565=CARTESIAN_POINT ( 'NONE',  ( 5.000000000000000888, -23.45833333060214443, 2.886751345948126879 ) ) ;
#43567=CARTESIAN_POINT ( 'NONE',  ( 5.000000000000000000, -53.37499999726881583, -6.123233995736766282E-16 ) ) ;
#43569=VERTEX_POINT ( 'NONE', #61869 ) ;
#43570=EDGE_CURVE ( 'NONE', #31695, #6727, #27380, .T. ) ;
#43572=CARTESIAN_POINT ( 'NONE',  ( 4.458734124999999437, 20.18750000136559208, -5.460374474430324690E-16 ) ) ;
#43578=CARTESIAN_POINT ( 'NONE',  ( 1.339745962155612702, -4.169658196007335782, -5.000000000000000000 ) ) ;
#43580=( BOUNDED_CURVE ( )  B_SPLINE_CURVE ( 2, ( #37884, #47222, #3165, #57515, #33058, #28216, #22146, #47830, #22784 ),
 .UNSPECIFIED., .F., .F. ) 
 B_SPLINE_CURVE_WITH_KNOTS ( ( 3, 2, 2, 2, 3 ),
 ( 0.5017857142857142794, 0.5023809523809523725, 0.5035714285714285587, 0.5047619047619047450, 0.5053571428571428381 ),
 .UNSPECIFIED. ) 
 CURVE ( )  GEOMETRIC_REPRESENTATION_ITEM ( )  RATIONAL_B_SPLINE_CURVE ( ( 0.9330127018922194093, 0.9330127018922194093, 1.000000000000000000, 0.8660254037844387076, 1.000000000000000000, 0.8660254037844387076, 1.000000000000000000, 0.9330127018922194093, 0.9330127018922194093 ) ) 
 REPRESENTATION_ITEM ( '' )  );
#43581=CARTESIAN_POINT ( 'NONE',  ( -1.339745962155613812, -103.2053418012614969, -5.000000000000000000 ) ) ;
#43582=CARTESIAN_POINT ( 'NONE',  ( -4.458734124999999437, -58.39583333196773651, -2.574251347313719407 ) ) ;
#43584=CARTESIAN_POINT ( 'NONE',  ( -4.458734124999999437, 21.68750000136559208, 0.000000000000000000 ) ) ;
#43587=CARTESIAN_POINT ( 'NONE',  ( -2.229367062500000163, -46.72916666530106511, -3.861377020970580443 ) ) ;
#43589=CARTESIAN_POINT ( 'NONE',  ( 5.000000000000000888, -3.458333330602147093, 2.886751345948126879 ) ) ;
#43591=LINE ( 'NONE', #63233, #36851 ) ;
#43593=CARTESIAN_POINT ( 'NONE',  ( -4.458734124999999437, -11.64583333196774184, -2.574251347313719407 ) ) ;
#43594=ORIENTED_EDGE ( 'NONE', *, *, #4348, .T. ) ;
#43596=CARTESIAN_POINT ( 'NONE',  ( 2.229367062500001939, -96.97916666530105090, 3.861377020970579999 ) ) ;
#43598=CARTESIAN_POINT ( 'NONE',  ( -2.229367062500000163, -92.72916666530106511, -3.861377020970580443 ) ) ;
#43599=CARTESIAN_POINT ( 'NONE',  ( 5.000000000000000000, -54.29166666393549434, -2.886751345948129988 ) ) ;
#43600=DIRECTION ( 'NONE',  ( 0.000000000000000000, 0.000000000000000000, 1.000000000000000000 ) ) ;
#43603=CARTESIAN_POINT ( 'NONE',  ( 2.229367062500001939, -16.97916666530106866, 3.861377020970579999 ) ) ;
#43604=CARTESIAN_POINT ( 'NONE',  ( 2.229367062500001939, 8.770833334698927786, 3.861377020970579999 ) ) ;
#43606=CARTESIAN_POINT ( 'NONE',  ( 4.458734124999999437, -57.06249999863440081, -5.460374474430324690E-16 ) ) ;
#43607=DIRECTION ( 'NONE',  ( -0.000000000000000000, 1.000000000000000000, -0.000000000000000000 ) ) ;
#43609=CARTESIAN_POINT ( 'NONE',  ( 1.975475456537005874E-15, -8.624999997268812280, 5.000000000000000000 ) ) ;
#43611=ORIENTED_EDGE ( 'NONE', *, *, #62887, .T. ) ;
#43615=CARTESIAN_POINT ( 'NONE',  ( -1.339745962155613812, -25.20534180126147561, -5.000000000000000000 ) ) ;
#43616=CARTESIAN_POINT ( 'NONE',  ( 4.458734124999998549, -83.72916666530107932, -2.574251347313721627 ) ) ;
#43617=CARTESIAN_POINT ( 'NONE',  ( 9.457646018065525792E-16, 16.68750000136559564, 5.148502694627439702 ) ) ;
#43620=EDGE_CURVE ( 'NONE', #10332, #27379, #47480, .T. ) ;
#43621=EDGE_CURVE ( 'NONE', #1553, #30363, #31911, .T. ) ;
#43622=DIRECTION ( 'NONE',  ( -0.000000000000000000, 1.000000000000000000, -0.000000000000000000 ) ) ;
#43624=CARTESIAN_POINT ( 'NONE',  ( -3.535250795749689387E-16, -68.25000000000000000, -5.773502691896257311 ) ) ;
#43627=CARTESIAN_POINT ( 'NONE',  ( 2.500000000000002220, -102.6666666666666572, 4.330127018922192761 ) ) ;
#43631=CARTESIAN_POINT ( 'NONE',  ( -6.972266317189433020E-16, 4.875000002731184168, -5.000000000000000000 ) ) ;
#43639=EDGE_CURVE ( 'NONE', #20419, #54097, #18380, .T. ) ;
#43644=CARTESIAN_POINT ( 'NONE',  ( -4.458734124999999437, -59.56249999863440081, 0.000000000000000000 ) ) ;
#43647=ORIENTED_EDGE ( 'NONE', *, *, #58246, .F. ) ;
#43652=CARTESIAN_POINT ( 'NONE',  ( 4.458734124999998549, -105.9791666653010651, -2.574251347313721627 ) ) ;
#43657=CARTESIAN_POINT ( 'NONE',  ( 2.229367062500001939, -38.97916666530107221, 3.861377020970579999 ) ) ;
#43658=CARTESIAN_POINT ( 'NONE',  ( 1.975475456537005874E-15, -83.74999999999998579, 5.000000000000000000 ) ) ;
#43659=CARTESIAN_POINT ( 'NONE',  ( 0.000000000000000000, -120.0000000000000000, 0.000000000000000000 ) ) ;
#43660=CARTESIAN_POINT ( 'NONE',  ( 4.458734125000001214, -13.89583333196774007, 2.574251347313718519 ) ) ;
#43661=CARTESIAN_POINT ( 'NONE',  ( -4.458734124999999437, -102.6458333319677365, -2.574251347313719407 ) ) ;
#43662=ORIENTED_EDGE ( 'NONE', *, *, #2413, .F. ) ;
#43664=CARTESIAN_POINT ( 'NONE',  ( -2.229367062499996610, -30.39583333196773651, 3.861377020970582219 ) ) ;
#43668=CARTESIAN_POINT ( 'NONE',  ( -6.972266317189433020E-16, -47.12499999726880873, -5.000000000000000000 ) ) ;
#43671=CARTESIAN_POINT ( 'NONE',  ( 2.229367062500001939, 2.770833334698928674, 3.861377020970579999 ) ) ;
#43674=CARTESIAN_POINT ( 'NONE',  ( 6.158835246850667461E-14, 9.749999999999996447, -4.999999999999999112 ) ) ;
#43675=CARTESIAN_POINT ( 'NONE',  ( 2.499999999999998668, -94.33333333333332860, -4.330127018922193649 ) ) ;
#43676=CARTESIAN_POINT ( 'NONE',  ( 2.229367062499998831, -29.64583333196773296, -3.861377020970580887 ) ) ;
#43677=CARTESIAN_POINT ( 'NONE',  ( 2.500000000000002220, -73.66666666666665719, 4.330127018922192761 ) ) ;
#43678=CARTESIAN_POINT ( 'NONE',  ( 4.458734124999999437, -76.06249999863440792, -5.460374474430324690E-16 ) ) ;
#43682=CARTESIAN_POINT ( 'NONE',  ( -4.458734124999999437, -2.312499998634407028, 0.000000000000000000 ) ) ;
#43683=CARTESIAN_POINT ( 'NONE',  ( 2.229367062499998831, 29.10416666803225993, -3.861377020970580887 ) ) ;
#43684=CARTESIAN_POINT ( 'NONE',  ( -4.458734124999999437, -44.56249999863440081, 0.000000000000000000 ) ) ;
#43687=ORIENTED_EDGE ( 'NONE', *, *, #58688, .T. ) ;
#43690=CARTESIAN_POINT ( 'NONE',  ( -2.229367062500000163, -71.47916666530107932, -3.861377020970580443 ) ) ;
#43691=CARTESIAN_POINT ( 'NONE',  ( 5.000000000000000000, -103.2916666639354730, -2.886751345948129988 ) ) ;
#43695=CARTESIAN_POINT ( 'NONE',  ( -2.229367062499996610, -110.3958333319677507, 3.861377020970582219 ) ) ;
#43697=CARTESIAN_POINT ( 'NONE',  ( -2.499999999999996447, -53.83333333333332860, 4.330127018922195425 ) ) ;
#43702=EDGE_CURVE ( 'NONE', #26835, #22293, #52491, .T. ) ;
#43706=ADVANCED_FACE ( 'NONE', ( #21945 ), #57001, .T. ) ;
#43708=EDGE_CURVE ( 'NONE', #39400, #52308, #28026, .T. ) ;
#43713=ORIENTED_EDGE ( 'NONE', *, *, #24049, .F. ) ;
#43721=CARTESIAN_POINT ( 'NONE',  ( 2.229367062499998831, -38.89583333196773651, -3.861377020970580887 ) ) ;
#43725=CARTESIAN_POINT ( 'NONE',  ( -2.499999999999996447, -29.83333333333332860, 4.330127018922195425 ) ) ;
#43729=( BOUNDED_CURVE ( )  B_SPLINE_CURVE ( 2, ( #27742, #8140, #47371, #3319, #13268, #46422, #2371, #4552, #63116 ),
 .UNSPECIFIED., .F., .F. ) 
 B_SPLINE_CURVE_WITH_KNOTS ( ( 3, 2, 2, 2, 3 ),
 ( 0.5196428571428571841, 0.5202380952380952772, 0.5214285714285714635, 0.5226190476190476497, 0.5232142857142857428 ),
 .UNSPECIFIED. ) 
 CURVE ( )  GEOMETRIC_REPRESENTATION_ITEM ( )  RATIONAL_B_SPLINE_CURVE ( ( 0.9330127018922194093, 0.9330127018922194093, 1.000000000000000000, 0.8660254037844387076, 1.000000000000000000, 0.8660254037844387076, 1.000000000000000000, 0.9330127018922194093, 0.9330127018922194093 ) ) 
 REPRESENTATION_ITEM ( '' )  );
#43733=CARTESIAN_POINT ( 'NONE',  ( 9.457646018065525792E-16, -88.31249999863439371, 5.148502694627439702 ) ) ;
#43735=ORIENTED_EDGE ( 'NONE', *, *, #38543, .F. ) ;
#43739=CARTESIAN_POINT ( 'NONE',  ( 2.499999999999998668, -43.33333333333333570, -4.330127018922193649 ) ) ;
#43740=EDGE_LOOP ( 'NONE', ( #34368, #22805, #26507, #34859 ) ) ;
#43741=DIRECTION ( 'NONE',  ( 0.000000000000000000, 0.000000000000000000, 1.000000000000000000 ) ) ;
#43742=CARTESIAN_POINT ( 'NONE',  ( -3.152548672688508926E-16, -10.81249999863440792, -5.148502694627439702 ) ) ;
#43743=FACE_OUTER_BOUND ( 'NONE', #4727, .T. ) ;
#43745=CARTESIAN_POINT ( 'NONE',  ( 2.500000000000002220, -55.54166666393548013, 4.330127018922192761 ) ) ;
#43747=CARTESIAN_POINT ( 'NONE',  ( 2.229367062500001939, 20.77083333469892779, 3.861377020970579999 ) ) ;
#43749=CARTESIAN_POINT ( 'NONE',  ( -4.458734124999999437, -94.31249999863440792, 0.000000000000000000 ) ) ;
#43752=CARTESIAN_POINT ( 'NONE',  ( -4.458734124999999437, -11.39583333196774007, -2.574251347313719407 ) ) ;
#43754=DIRECTION ( 'NONE',  ( 0.000000000000000000, 0.000000000000000000, 1.000000000000000000 ) ) ;
#43755=CARTESIAN_POINT ( 'NONE',  ( -1.339745962155613812, -88.20534180126146850, -5.000000000000000000 ) ) ;
#43756=CARTESIAN_POINT ( 'NONE',  ( -2.500000000000000444, -42.04166666393548013, -4.330127018922193649 ) ) ;
#43757=CARTESIAN_POINT ( 'NONE',  ( 1.975475456537005874E-15, -29.74999999999999645, 5.000000000000000000 ) ) ;
#43758=CARTESIAN_POINT ( 'NONE',  ( 4.458734124999998549, 20.27083333469892779, -2.574251347313721627 ) ) ;
#43762=CARTESIAN_POINT ( 'NONE',  ( -4.458734124999998549, -62.22916666530106511, 2.574251347313722516 ) ) ;
#43765=CARTESIAN_POINT ( 'NONE',  ( -5.000000000000000000, 8.916666666666666075, -2.886751345948128211 ) ) ;
#43767=CARTESIAN_POINT ( 'NONE',  ( -2.500000000000000444, -60.04166666393547303, -4.330127018922193649 ) ) ;
#43768=CARTESIAN_POINT ( 'NONE',  ( 4.458734125000001214, -51.89583333196773651, 2.574251347313718519 ) ) ;
#43769=CARTESIAN_POINT ( 'NONE',  ( -5.000000000000000000, -87.87499999726880162, 0.000000000000000000 ) ) ;
#43771=CARTESIAN_POINT ( 'NONE',  ( 5.000000000000000000, -14.29166666393548013, -2.886751345948130876 ) ) ;
#43773=CARTESIAN_POINT ( 'NONE',  ( 4.458734124999998549, -90.97916666530106511, -2.574251347313721627 ) ) ;
#43775=CARTESIAN_POINT ( 'NONE',  ( -2.499999999999996447, -36.83333333333332860, 4.330127018922195425 ) ) ;
#43777=CARTESIAN_POINT ( 'NONE',  ( -6.972266317189433020E-16, -96.12499999726880162, -5.000000000000000000 ) ) ;
#43779=CARTESIAN_POINT ( 'NONE',  ( 9.457646018065525792E-16, -104.0624999986344221, 5.148502694627439702 ) ) ;
#43780=CARTESIAN_POINT ( 'NONE',  ( -2.229367062499996610, 9.604166668032261711, 3.861377020970582219 ) ) ;
#43784=VECTOR ( 'NONE', #31202, 1000.000000000000000 ) ;
#43789=VERTEX_POINT ( 'NONE', #4525 ) ;
#43792=CARTESIAN_POINT ( 'NONE',  ( -1.339745962155618253, 25.20534180126147916, 4.999999999999996447 ) ) ;
#43794=CARTESIAN_POINT ( 'NONE',  ( -2.499999999999996447, 24.29166666939785202, 4.330127018922195425 ) ) ;
#43795=CARTESIAN_POINT ( 'NONE',  ( 4.458734124999998549, -24.97916666530106511, -2.574251347313721627 ) ) ;
#43806=VERTEX_POINT ( 'NONE', #57943 ) ;
#43807=CARTESIAN_POINT ( 'NONE',  ( 4.458734124999999437, -75.06249999863440792, -5.460374474430324690E-16 ) ) ;
#43808=( NAMED_UNIT ( * ) PLANE_ANGLE_UNIT ( ) SI_UNIT ( $, .RADIAN. ) );
#43811=( BOUNDED_SURFACE ( )  B_SPLINE_SURFACE ( 1, 2, ( 
 ( #12754, #36255, #41066, #40748, #31743, #6670, #32053, #6995, #21467, #51689, #2802, #50416, #46221, #2486, #26277, #16953, #16634, #55883, #51375, #25965, #45900, #11794, #26605, #22422, #42020, #45582, #61028, #2184, #17595, #60396, #16321, #21788, #22099, #31412, #37211, #35942, #31105, #1861, #36566, #61661, #56197, #12118, #7316, #26927, #46544, #23048, #28489, #8561, #32376, #23368, #48107, #52323, #27545, #19141, #18829, #13698, #27860, #37517, #52938, #42966, #23678, #62609, #58075, #8875, #57777, #47176, #38153, #3746, #38448, #13389, #9189, #53253, #32691, #18532, #33634, #28173, #8257, #47478, #4060, #43277, #62916, #33319, #14007, #28802, #3433, #42652, #48418, #47788, #4361, #57158, #23980, #62293, #3119, #13072, #33011, #37838, #43584, #18215, #63226, #38758, #57470, #52628, #58396, #7941, #52000, #22739, #42337, #61975, #17895, #35223, #40355, #14324, #39708, #39391, #498, #25247, #30062, #49372, #30384, #54843, #43894, #5317, #24934, #20102, #50007, #25569, #53877, #5636, #44862, #5958, #10448, #45184, #39079, #59023, #34565, #53567, #44542, #59348, #33945, #15280, #34903, #825, #10134, #1150, #63543, #20431, #49045, #40031, #54525, #48727, #49690, #20750, #24292, #9491, #184, #4991, #4668, #59674, #34248, #15605, #54195, #24613, #10774, #29102, #19464, #29740, #58708, #14634, #9803, #44219, #19784, #29412, #14954, #55490, #6590, #1788, #6281, #56118, #55168, #12042, #7550, #30709, #36816, #40673, #50974, #26853, #7239, #46465, #26205, #16873, #17190, #45824, #35865, #56447, #36491, #6916, #60638, #50334, #50652, #51617, #22023, #11405, #1466, #12368, #31337, #51304, #40994, #11087, #2408, #21068, #59996, #21388, #25887, #31667, #55803, #41616, #61267, #46778, #31983, #27162, #2724, #60318, #45503, #22346, #2111, #16245, #15919, #35541, #31025, #16558, #36182, #11720, #26528, #46147, #21712, #41304, #60954, #3984, #7865, #22977, #42889, #38077, #18134, #58008, #8801, #42263, #62842, #28414, #32936, #33248, #48345, #48033, #42578, #23603, #3360, #32615, #43201, #37760, #52868, #56761, #18757, #3047, #12683, #38382, #61904, #62533, #52241, #13934, #33559, #8492, #57078, #53181, #52559, #32297, #37447, #22665, #4291, #18455, #9114, #57393, #28722, #51924, #41943, #17823, #27470, #61586, #12992, #57704, #8182, #17520, #37140, #28100, #27785, #47098, #47718, #47410, #62217, #13314, #3674, #13630, #23287, #59601, #33872, #30308, #9734, #14558, #58323, #5240, #43826, #49621, #44142, #58639, #10379, #20355, #23909, #19708, #39632, #24219, #54118, #53800, #29338, #24863, #43510, #19390, #34177, #48968, #53490, #20027, #19066, #59271, #35154, #14249, #744, #4596, #14875, #54451, #34828, #29988, #4920, #44464, #44783, #24539, #63471, #39953, #423, #34484, #114, #9419, #39317, #15534, #5557, #39008, #29030, #54769, #58945, #15203, #10056, #38684, #25169, #48654, #63156, #29668, #49300, #10700, #49928, #2029, #41226, #56371, #41542, #46391, #2338, #6202, #1076, #7162, #11643, #25817, #60873, #45111, #12293, #20682, #11328, #45753, #40915, #16162, #31263, #56047, #11963, #31591, #35469, #50578, #6841, #21634, #1707, #21944, #36417, #45430, #26770, #51225, #60560, #16799, #31910, #61194, #6521, #17116, #30952, #60245, #16482, #36103, #55728, #20995, #35789, #36740, #21312, #5882, #11010, #25489, #55411, #40288, #30632, #26133, #50898, #59926, #40600, #26449, #46070, #15848, #55087, #50254, #1395, #52164, #32860, #3599, #12914, #37061, #8727, #13860, #51538, #13237, #32536, #37678, #62459, #23204, #22905, #3908, #28339, #17443, #42501, #62137, #57320, #23527, #62768, #27392, #42817, #18379, #43128, #47644, #18688, #12604, #8108, #27712, #27085, #18057, #52489, #7474, #8422, #28025, #38000, #47339, #38314, #56688, #57632, #22591, #13561, #33179, #22267, #3289, #52794, #57942, #46700, #47955, #2648, #41867, #61514, #32217, #51846, #7789, #61828, #47025, #2974, #42188, #17752, #37368, #57000, #43752, #33484, #44387, #54042, #4224, #24149, #29592, #9660, #53105, #24462, #49223, #53415, #28651, #20278, #19948, #14800, #28960, #38610, #9980, #44067, #24782, #33, #59201, #5163, #58869, #48266, #39243, #4842, #39559, #14483, #10302, #54377, #33797, #19632, #34750, #29268, #9345, #48583, #347, #15129, #29913, #63396, #25096, #49540, #4524, #58243, #5481, #34413, #44704, #34104, #23838, #669, #14171, #9040, #58563, #43441, #39879, #48898, #59524, #63085, #18995, #19314, #38929, #53729, #15772, #10616, #16728, #21234, #35389, #50824, #54694, #2272, #30228, #20920, #55340, #50508, #25743, #40840, #1958, #21559, #41155, #45035, #60167, #16411, #11575, #11256, #31505, #45992, #55008, #36344, #60801, #6451, #6761, #21876, #55975, #16088, #11887, #40523, #6129, #51150, #30881, #26374, #49852, #7084, #40211, #5799, #26698, #10934, #36029, #45357, #46315, #41471, #45675, #30551, #15458, #26060, #25417, #50177, #59847, #35075, #55661, #31195, #1003, #20607, #1323, #35712, #1633, #60484, #42423, #17363, #23132, #17681, #32142, #47571, #57561, #61122, #56925, #13163, #61437, #27639, #27324, #2901, #62066, #17046, #56613, #7721, #22514, #7404, #57247, #56290, #32786, #8651, #31835, #37928, #41793, #52095, #27948, #8350, #3522, #46954, #17979, #18304, #42109, #36985, #13486, #37604, #8034, #61754, #51466, #12530, #22192, #23455, #52417, #42738, #33103, #27011, #3837, #37296, #51776, #46631, #62382, #12844, #52717, #32463, #47268, #28264, #47877, #36663, #3213, #12218, #22833, #2576, #9276, #48513, #24390, #62698, #38538, #53342, #4452, #53027, #39172, #38246, #58797, #54293, #13788, #19876, #23770, #34037, #9903, #53975, #29513, #28892, #63639, #278, #24081, #18923, #39490, #19560, #53658, #43676, #33411, #33724, #34674, #5089, #58167, #48198, #59126, #14414, #34347, #63318, #57867, #49144, #4152, #43060, #19238, #8967, #14728, #38854, #24710, #44314, #29837, #15059, #10232, #49470, #43370, #28578, #5409, #48825, #63016, #18623, #14098, #58490, #9592, #29200, #4763, #43992, #35317, #30805, #12377, #31990, #51624, #54618, #6060, #25983, #21159, #1246, #41950, #56455, #25343, #46786, #7558, #16012, #17197, #32304, #27170, #25670, #2733, #50103, #15697, #22353, #20846, #36824, #39807, #61595, #49783, #59449, #17529, #44966, #45598, #54937, #37147, #56771, #55265, #40130, #12691, #35637, #15379, #35003, #50436, #60090, #51933, #45280, #25025, #44636, #928, #11183, #596, #40449, #20532, #59771, #40765, #60412, #20203, #6377, #1557, #10543, #10863, #30479, #30154, #5729, #43211, #13004, #53190, #18144, #3055, #32624, #52568, #13324, #3991, #22986, #23298, #62546, #37772, #57403, #57713, #47106, #8501, #52877, #23615, #32944, #57085, #28731, #33880, #7874, #33258, #28111, #13638, #18765, #62852, #42898, #23918, #48357, #37454, #18466, #38087, #8812, #43519, #19075, #47418, #38391, #58016, #63164, #13944, #38695, #52251, #47727, #3684, #22673, #28427, #48041, #27478, #33571, #9123, #4301, #58332, #14258, #8191, #42272, #42588, #61912, #17832, #27793, #3370, #62226, #45119, #59935, #44473, #29678, #20692, #43833, #9430, #54127, #5566, #123, #40297, #63479, #29040, #53810, #10065, #10710, #19717, #53500, #758, #10388, #24227, #44152, #49630, #49308, #48663, #432, #25180, #9741, #4604, #15857, #39964, #34837, #48980, #58646, #29998, #20038, #44794, #39642, #15543, #20366, #15212, #19398, #59611, #14566, #39017, #14885, #34188, #35163, #5249, #54779, #30317, #29346, #25500, #49938, #5893, #4929, #24547, #1084, #59281, #39326, #58958, #34492, #24872, #54462, #40923, #11651, #6847, #45760, #41234, #21954, #41550, #61201, #1403, #16491, #36426, #31600, #31271, #51545, #2346, #35798, #56379, #17123, #26461, #26779, #41876, #36749, #36112, #12303, #60566, #26141, #31918, #50905, #46397, #50264, #7481, #60254, #6212, #27094, #55421, #56054, #1714, #46711, #2656, #2036, #50587, #22275, #46078, #25825, #30962, #16173, #61523, #11970, #51234, #35479, #45440, #55095, #21322, #55735, #21004, #16806, #11339, #11021, #21641, #6527, #30642, #40610, #60881, #7170, #33188, #17760, #47654, #47348, #22918, #62470, #37075, #12925, #27721, #42510, #27402, #13570, #12613, #52803, #28660, #51857, #57951, #61840, #8432, #47964, #28347, #3919, #3297, #38009, #38322, #62148, #57010, #13872, #57642, #28036, #18066, #7800, #8117, #9050, #43137, #32547, #22600, #33497, #52498, #8740, #37688, #53114, #48276, #4232, #37377, #32226, #18697, #23215, #52173, #23538, #56697, #23847, #47033, #57330, #13246, #3607, #32869, #42825, #62777, #43450, #17453, #2983, #18390, #42197, #59210, #39253, #15468, #29925, #63407, #20288, #49550, #54053, #54387, #5810, #5492, #43, #25106, #24473, #53737, #679, #58879, #10312, #14181, #44716, #24159, #33808, #39889, #19325, #19959, #9670, #35086, #59535, #29603, #14494, #54706, #9990, #53424, #58575, #43762, #25427, #39570, #15139, #10626, #9358, #63095, #48908, #29278, #28970, #44398, #38939, #30239, #19643, #34116, #49862, #19007, #38620, #14810, #34761, #4853, #49233, #44080, #34424, #357, #58257, #5175, #24792, #48593, #4534, #41165, #40223, #60812, #56303, #15783, #21886, #25753, #36040, #11899, #55985, #31519, #11266, #1968, #2282, #30890, #20931, #41482, #21569, #55671, #45688, #35399, #35722, #36673, #7095, #40536, #50187, #61133, #16422, #36355, #26070, #59858, #51162, #6139, #45046, #6461, #55021, #16738, #40851, #26709, #46324, #31845, #17056, #50835, #45367, #12231, #20616, #51477, #10943, #50521, #21244, #11586, #55352, #6775, #7414, #1013, #30562, #1334, #1645, #46003, #60177, #60494, #16099, #31205, #26386, #18315, #47583, #47277, #8359, #28276, #3534, #12856, #23143, #37306, #22526, #62394, #52104, #27960, #22206, #42751, #12539, #41805, #37940, #7730, #37616, #42122, #13498, #57572, #22844, #46966, #33114, #3226, #61449, #27335, #32152, #47890, #13174, #32798, #52731, #17378, #27024, #17691, #61764, #36999, #57257, #2911, #8663, #32475, #56935, #46642, #2587, #56625, #52427, #51788, #8045, #27650, #42434, #62076, #17990, #40418, #16308, #31091, #26264, #30777, #16939, #15982, #36553, #32040, #55233, #61331, #1526, #11781, #51361, #6657, #50713, #7302, #55868, #36877, #17255, #50398, #31399, #51037, #26591, #56507, #51677, #60382, #12104, #31731, #12429, #56184, #7617, #45569, #1848, #41054, #60058, #6980, #46208, #20818, #2170, #21776, #26914, #16620, #27222, #6347, #46531, #55557, #2472, #41368, #11155, #60700, #61014, #35607, #22085, #41683, #46842, #36241, #25953, #21130, #40735, #11471, #35929, #45886, #21454, #42638, #13687, #58064, #9178, #57456, #62281, #33624, #56823, #22408, #3420, #18519, #13059, #53242, #12742, #42007, #3108, #23036, #23666, #32678, #2788, #33306, #23355, #37198, #57144, #62597, #18202, #61647, #13376, #38139, #22725, #17581, #28790, #52926, #47777, #61963, #7929, #42954, #32998, #57765, #52614, #28478, #8863, #28162, #32362, #8549, #37823, #48093, #47466, #43263, #62902, #42323, #3734, #4048, #18817, #17884, #37505, #38437, #13996, #51986, #27531, #47164, #52309, #8245, #27845, #41081, #54617, #40129, #1878, #11810, #15378, #11182, #31120, #15696, #45597, #45279, #20845, #60411, #35002, #10862, #25669, #40448, #25342, #11504, #10542, #50742, #26618, #49782, #55897, #59770, #6376, #45916, #1245, #6686, #35959, #60727, #36273, #60089, #54936, #31427, #55584, #25982, #16011, #5728, #6059, #7009, #16649, #30478, #20531, #51065, #50435, #26292, #35636, #30153, #21483, #55264, #21158, #46235, #2198, #21802, #44965, #30804, #16337, #41397, #1556, #927, #35316, #50102, #40764, #27872, #52014, #52335, #3758, #47492, #61674, #3445, #22437, #51703, #62304, #56849, #8269, #12134, #23060, #22116, #31756, #37853, #17280, #17908, #7643, #33024, #57485, #27557, #12455, #42665, #7956, #51389, #56534, #41709, #23381, #37529, #13086, #52640, #7331, #61047, #46873, #27247, #26942, #42350, #2816, #18226, #36580, #61358, #13403, #8574, #16969, #12766, #32706, #36904, #47190, #42032, #17607, #61988, #56212, #32066, #37223, #32389, #46558, #57170, #2499, #28185, #47801, #3132, #22752, #23692, #33958, #9814, #53266, #58719, #63557, #5005, #196, #9201, #18842, #39402, #19475, #53579, #43596, #33332, #33647, #34576, #24625, #38460, #48120, #59038, #14337, #34262, #23992, #57790, #49057, #4072, #42980, #4375, #13709, #14645, #38771, #39089, #53890, #29752, #14968, #19794, #54208, #43291, #38167, #44231, #48737, #62927, #29425, #18545, #49385, #52951, #48433, #19153, #9507, #10145, #29116, #5330, #62623, #8888, #63239, #28501, #58409, #28813, #58088, #4681, #14019, #24303, #43908, #49702, #39721, #1799, #44878, #45516, #15618, #60648, #21402, #55179, #40043, #55505, #15932, #59358, #20444, #5646, #50989, #1477, #40685, #16571, #34915, #31346, #10787, #35235, #15293, #6294, #54854, #50663, #509, #25259, #11419, #41006, #24947, #20762, #60330, #841, #11100, #30397, #50020, #25899, #44553, #59685, #5974, #25583, #54537, #21080, #20119, #16257, #36193, #10458, #55814, #45196, #35555, #31038, #1163, #35876, #6603, #26217, #45837, #40368, #60009, #11730, #30072, #30724, #50347, #60966, #61280, #62229, #32628, #2423, #12054, #22991, #41955, #61916, #51628, #21723, #13008, #31678, #6928, #31994, #41318, #42276, #2737, #3059, #17836, #57407, #42592, #47422, #3374, #7252, #2122, #8195, #12695, #26864, #37459, #46160, #13327, #16886, #12381, #46791, #61598, #17201, #32308, #57089, #52256, #27797, #36502, #7562, #7879, #22677, #22357 ),
 ( #36829, #18147, #56131, #51314, #37775, #32948, #26538, #17533, #46477, #22035, #37151, #56459, #27174, #51937, #41626, #56776, #27482, #47111, #62550, #48668, #47731, #4608, #127, #23301, #29350, #33262, #43524, #19405, #62855, #24231, #9434, #14570, #9745, #18768, #28431, #48984, #29043, #63168, #53194, #42901, #43215, #44157, #34192, #48044, #57716, #4933, #23923, #43837, #33573, #3687, #58649, #13641, #52571, #13947, #18470, #63483, #48360, #39021, #53815, #39330, #24553, #19721, #58963, #52880, #38090, #14890, #58336, #8815, #8504, #28114, #3996, #23618, #58019, #28734, #19079, #38395, #14264, #9127, #4304, #38699, #33884, #53504, #35483, #30647, #10714, #50591, #30966, #11025, #25504, #35168, #24876, #25184, #26145, #60259, #30002, #39647, #6531, #5898, #25828, #15547, #49312, #40614, #59285, #34497, #59615, #5254, #6216, #30321, #50269, #45444, #21326, #45764, #11343, #1719, #34843, #29683, #35802, #40301, #54466, #1408, #10069, #40926, #44477, #39970, #49943, #45123, #44799, #59939, #21008, #16177, #55426, #436, #54783, #55100, #60572, #1088, #54131, #20042, #10393, #15216, #49633, #20696, #5570, #762, #20370, #15861, #47037, #41554, #7174, #17763, #12308, #7803, #31275, #42200, #41238, #50909, #57013, #36430, #37078, #22279, #60885, #16809, #61525, #31604, #2986, #7485, #6851, #11975, #56059, #42514, #56700, #32229, #52176, #26465, #22921, #2350, #26782, #46082, #17456, #46401, #61843, #55739, #51238, #22603, #12928, #16494, #31922, #51860, #21958, #46714, #61205, #17129, #12617, #36116, #36753, #56383, #51550, #2041, #27405, #11655, #37380, #27724, #21646, #32551, #27098, #2659, #8121, #41879, #47351, #3300, #24162, #19328, #28350, #38013, #9361, #53741, #4857, #53118, #38325, #29281, #52501, #18069, #62781, #14184, #8742, #48911, #8435, #37691, #62473, #18700, #38942, #47967, #62151, #28974, #19010, #32872, #52806, #58261, #57954, #57333, #9053, #33811, #18393, #13249, #24477, #48596, #43453, #57645, #3611, #38623, #28663, #53428, #48279, #43765, #4536, #23850, #3922, #63411, #28039, #58578, #43140, #14497, #34118, #13573, #4235, #9673, #13875, #33191, #23541, #47657, #23218, #42829, #33501, #63098, #10629, #59213, #47, #19646, #19964, #34428, #49237, #25757, #54390, #39257, #5179, #25109, #49553, #40227, #15143, #59538, #35090, #10317, #29928, #30242, #58883, #44720, #25431, #59862, #5495, #29607, #1336, #6464, #44082, #5813, #54056, #682, #20291, #30566, #15473, #60179, #20934, #9994, #54709, #49865, #45049, #16101, #55354, #39574, #35402, #55024, #35725, #15786, #11268, #24797, #39892, #1016, #14814, #20620, #10947, #44402, #50190, #6142, #45370, #40538, #30893, #361, #50523, #34764, #37001, #31847, #60496, #2285, #52106, #2589, #41807, #61766, #36043, #32477, #11902, #16740, #16424, #7417, #36357, #51790, #1647, #50837, #12541, #22528, #26072, #21888, #61452, #26388, #56307, #55987, #31522, #27026, #45690, #21571, #51164, #7097, #55673, #22209, #21246, #17382, #37308, #11588, #2915, #6778, #17058, #56628, #26712, #32154, #46644, #7732, #46968, #46326, #1971, #42124, #27337, #36675, #41484, #31208, #61136, #17694, #56937, #41168, #46006, #12858, #12233, #40853, #51479, #60815, #14984, #13178, #8048, #33116, #22846, #44247, #4696, #5021, #211, #59375, #44568, #49401, #5345, #8361, #3228, #10162, #14660, #27962, #19809, #47279, #15309, #42436, #13500, #48754, #43925, #18317, #34279, #59056, #34593, #54224, #37618, #52733, #9830, #24640, #24318, #24963, #39418, #47585, #29767, #526, #63572, #20135, #34931, #39735, #9524, #27652, #29131, #62396, #62079, #19491, #17992, #57259, #32800, #52429, #3536, #23145, #42753, #29441, #53904, #37942, #57575, #49073, #39106, #58734, #45531, #25276, #50037, #15634, #25913, #45851, #35570, #5663, #60663, #59702, #54552, #15948, #44897, #26231, #50361, #50676, #1813, #41333, #26554, #31362, #51003, #54870, #49718, #55829, #60344, #10801, #21417, #30088, #60980, #857, #60025, #30740, #1492, #1179, #16272, #41020, #16587, #36207, #20460, #55194, #55521, #6618, #6309, #6943, #11744, #30413, #46174, #2135, #21095, #21738, #16901, #10475, #11114, #40059, #40699, #45213, #35250, #35891, #5995, #25600, #20779, #40384, #11435, #31053, #56473, #57107, #42290, #61294, #17216, #17850, #51643, #3389, #27497, #7266, #32009, #36843, #62565, #13024, #52272, #8518, #46492, #42918, #22371, #27189, #26878, #37472, #46805, #62245, #12068, #12394, #23006, #32962, #36517, #32324, #8209, #7577, #3074, #2752, #41971, #32641, #56147, #61613, #17547, #37167, #2440, #27812, #31693, #47437, #47746, #22049, #13342, #56790, #47126, #42607, #12708, #18164, #37791, #57421, #52586, #51954, #7892, #28128, #3702, #22691, #61931, #41642, #23317, #51328, #44172, #13960, #23633, #34513, #58030, #8831, #43228, #139, #28749, #13656, #62869, #63181, #23936, #14584, #33587, #33896, #9447, #48374, #4316, #4620, #57730, #19092, #63495, #34204, #43537, #4012, #39347, #44490, #18484, #43849, #28444, #38710, #58349, #4944, #53519, #54144, #58977, #48059, #29056, #48680, #24245, #10083, #29694, #53206, #9757, #29364, #49325, #53828, #5268, #18781, #14277, #19420, #33276, #39034, #58661, #38106, #48997, #24567, #19733, #14904, #24889, #38408, #52895, #9140, #11354, #6229, #34857, #40314, #30977, #55750, #6863, #55113, #59952, #31286, #54478, #20056, #1100, #16188, #10726, #50921, #10405, #39660, #775, #20709, #21337, #30333, #452, #50601, #21020, #30017, #54798, #60270, #15875, #59297, #11038, #35815, #20382, #15229, #26478, #6542, #45456, #59627, #5582, #40627, #30661, #55439, #50282, #26156, #45775, #25839, #5911, #1734, #49645, #40937, #45136, #60587, #16507, #39982, #1421, #36128, #35495, #15560, #35180, #11667, #25199, #44813, #49959, #25518, #12627, #61216, #2052, #21660, #42209, #18082, #7186, #27111, #2669, #41251, #32243, #51873, #46092, #17468, #47047, #32564, #41890, #57343, #31615, #52186, #17141, #57026, #7814, #16821, #22291, #12941, #37705, #52511, #37090, #61536, #13259, #36440, #60898, #46724, #61855, #56394, #32883, #56070, #11989, #46414, #56708, #3310, #12321, #51251, #8131, #2997, #26794, #36765, #17772, #27416, #2363, #22614, #37391, #21972, #41565, #8446, #27734, #47363, #31932, #51560, #22931, #42525, #62162, #7499, #53750, #4546, #53440, #33513, #48607, #38024, #29291, #9063, #4869, #48920, #28359, #14195, #24488, #4245, #47980, #3934, #43775, #63421, #38951, #63109, #58276, #33821, #43151, #47669, #3621, #23553, #18403, #33201, #9683, #38336, #23228, #52816, #28673, #53131, #24171, #62791, #43463, #19020, #57964, #13885, #9373, #42843, #48293, #28984, #19339, #23860, #13582, #44094, #54067, #28049, #58589, #57656, #38633, #14507, #34129, #58, #19655, #39267, #8754, #58895, #14824, #34438, #62485, #18710, #49565, #1346, #20948, #1657, #19977, #11278, #54721, #50531, #30904, #10328, #59875, #6474, #49877, #29939, #5503, #25769, #45381, #40550, #45061, #40238, #15797, #25119, #29618, #49248, #44731, #372, #15154, #55364, #20304, #5191, #34775, #10641, #15484, #6153, #691, #25441, #1027, #39904, #59549, #35414, #24808, #30254, #55035, #60191, #35103, #59222, #26082, #36054, #10006, #10959, #39585, #5826, #20632, #16111, #30581, #45702, #21256, #54399, #50203, #35737, #40863, #60507, #16434, #44411, #46976, #2924, #47289, #51799, #27661, #16749, #36687, #12243, #31217, #22218, #61462, #55682, #27036, #56638, #42135, #51489, #3239, #41179, #61776, #26721, #22539, #17394, #26397, #31856, #17703, #22855, #62088, #46653, #7427, #42446, #46017, #11596, #56320, #7741, #2294, #18005, #1979, #50847, #55997, #2598, #12868, #21896, #6788, #37317, #12552, #21581, #46337, #27345, #41815, #60824, #37009, #56947, #11912, #36366, #31534, #32486, #32165, #51174, #7107, #52115, #8059, #41493, #61146, #17068, #14119, #63035, #43080, #58190, #28600, #4474, #47900, #53362, #33745, #63345, #58510, #3856, #13512, #34057, #9296, #48218, #38265, #27974, #28288, #29219, #19259, #33128, #42764, #53679, #8988, #28912, #18643, #52439, #43697, #62406, #37628, #62718, #8373, #48535, #33432, #24101, #38876, #24413, #9612, #14434, #48845, #37952, #32810, #4786, #43390, #57585, #44014, #13187, #63662, #47595, #57887, #13813, #4173, #23477, #18943, #57269, #3547, #23155, #18328, #53051, #38561, #52745, #23788, #8674, #50125, #19895, #40473, #6082, #10564, #10887, #26008, #25692, #20227, #45302, #44656, #10256, #20871, #15403, #30503, #34365, #1269, #44332, #53995, #60113, #39510, #40154, #25367, #298, #59147, #953, #34692, #16034, #30174, #9922, #15079, #54317, #45626, #59798, #35338, #55288, #29534, #19579, #5428, #29857, #49171, #20553, #49490, #35663, #58818, #25045, #11208, #30831, #39193, #35028, #54957, #617, #49804, #39827, #59470, #15719, #14748, #54640, #5749, #44987, #5111, #50460, #24730, #6400, #12792, #35981, #42059, #45938, #60435, #2842, #7354, #1901, #36932, #40788, #52044, #16360, #7031, #41422, #36608, #11833, #26964, #51728, #7668, #27275, #31142, #46261, #2525, #61385, #61071, #17630, #32092, #21508, #22462, #46901, #56240, #56558, #7983, #61701, #2220, #37247, #26642, #55919, #56874, #16992, #12479, #55610, #32413, #26319, #11526, #27581, #41105, #22140, #46583, #60750, #16675, #41735, #36296, #1581, #12161, #50768, #31453, #51094, #21181, #17305, #6711, #21823, #31780, #51411, #33053, #37879, #17930, #28529, #57511, #9226, #22778, #8296, #33671, #43624, #47216, #43006, #62953, #47520, #13739, #13427, #52667, #48147, #3159, #42687, #8601, #28211, #57194, #43318, #42373, #18871, #58435, #37554, #24020, #27899, #38192, #14047, #47825, #38488, #4099, #28839, #4400, #3784, #23084, #63266, #23722, #57817, #23407, #13114, #62652, #38797, #48463, #62331, #52358, #19184, #18571, #58115, #33360, #62012, #53290, #3471, #32731, #52975, #18252, #14363, #8916, #33987, #53607, #9541, #1193, #6010, #25612, #29458, #44260, #44583, #20151, #39431, #59072, #15323, #4712, #29781, #10488, #44913, #54237, #14674, #50052, #55210, #29145, #54566, #19506, #14997, #34610, #15646, #540, #45226, #20793, #58746, #39748, #59390, #34947, #40395, #60036, #5035, #20472, #40074, #15961, #25288, #35583, #53917, #10178, #49413, #24337, #30101, #49732, #48767, #5677, #869, #35262, #24976, #43938, #34295, #54883, #224, #59717, #10813, #63585, #5357, #30425, #39119, #9843, #49089, #24654, #19822, #45545, #30754, #61549, #17784, #27123, #57354, #1505, #50374, #16284, #17480, #47375, #46737, #11127, #8146, #37403, #21106, #2683, #12953, #32255, #6321, #47060, #32577, #6633, #40711, #25926, #37719, #52199, #37102, #22303, #27746, #57039, #42537, #3324, #13273, #22943, #62173, #51885, #18095, #31066, #32897, #27428, #60360, #35902, #56721, #55537, #11447, #50690, #3010, #22626, #41902, #12638, #7826, #42223, #61868, #36028, #20029, #24540, #44144, #44466, #58949, #10057, #51149, #15204, #115, #29669, #49622, #10380, #1957, #55974, #11886, #31504, #34485, #5559, #6760, #21558, #44786, #21875, #36343, #5241, #26697, #7083, #59604, #60800, #12217, #46314, #25171, #2271, #29989, #59273, #41470, #747, #16727, #19709, #61121, #49301, #39318, #17045, #24864, #26373, #11574, #424, #39633, #50823, #34829, #36662, #15536, #14876, #54454, #20358, #31834, #45991, #41154, #56289, #54119, #4921, #39956, #55660, #31194, #32785, #61753, #13485, #27010, #12529, #37927, #47876, #51465, #47267, #3521, #51775, #17978, #17680, #56924, #52416, #7403, #46953, #37295, #12843, #61436, #47570, #46630, #23131, #62697, #22191, #28263, #32141, #42422, #18303, #32462, #42737, #8349, #33102, #8650, #52094, #27323, #3836, #27947, #62065, #8033, #41792, #42108, #43059, #52716, #2900, #56612, #23454, #22832, #62381, #27638, #2575, #57560, #7720, #17362, #3212, #36984, #18622, #37603, #38245, #57866, #13787, #22513, #57246, #13162, #33723, #28577, #34673, #39171, #53341, #5088, #8966, #20202, #48197, #38853, #9591, #4762, #43675, #58796, #5408, #44635, #9275, #24709, #44313, #25024, #29512, #595, #58166, #14413, #53657, #4151, #63638, #14727, #33410, #24389, #34346, #19875, #29199, #39806, #18922, #39489, #4451, #277, #53974, #23769, #48824, #59125, #59448, #53026, #43991, #19559, #43369, #63015, #38537, #34036, #49143, #63317, #14097, #28891, #48512, #24080, #9902, #54292, #19237, #58489, #15058, #10231, #29836, #49469, #16324, #60399, #26279, #45901, #50420, #20516, #6364, #44951, #10525, #21145, #15682, #11169, #34657, #45584, #44620, #54277, #35944, #39790, #40434, #25653, #580, #20189, #1233, #34988, #25968, #10848, #10216, #15365, #59436, #19860, #60073, #35622, #55573, #29820, #39473, #5714, #30139, #49452, #20832, #49768, #1541, #59110, #54603, #40750, #11490, #15039, #35300, #55250, #25328, #50091, #911, #40115, #15998, #5394, #59756, #54921, #30463, #25011, #30792, #6045, #31107, #50728, #45266, #6671, #46222, #56522, #32377, #12121, #17596, #22424, #27546, #22741, #31745, #41383, #61976, #42022, #12442, #7317, #11796, #61663, #60713, #37212, #13073, #36258, #42338, #2185, #32054, #52002, #51376, #56838, #12755, #47177, #17896, #26928, #61032, #37518, #7943, #51690, #2487, #55884, #56198, #57159, #3120, #16954, #6996, #32694, #36893, #52324, #46545, #16635, #8258, #26606, #1864, #22102, #31413, #27861, #61344, #21468, #41067, #51052, #21789, #36567, #41697, #17268, #7631, #27235, #46859, #2803, #19143, #23049, #35150, #42653, #52939, #23679, #18830, #57778, #53255 ) ),
 .UNSPECIFIED., .F., .F., .F. ) 
 B_SPLINE_SURFACE_WITH_KNOTS ( ( 2, 2 ),
 ( 3, 2, 2, 2, 2, 2, 2, 2, 2, 2, 2, 2, 2, 2, 2, 2, 2, 2, 2, 2, 2, 2, 2, 2, 2, 2, 2, 2, 2, 2, 2, 2, 2, 2, 2, 2, 2, 2, 2, 2, 2, 2, 2, 2, 2, 2, 2, 2, 2, 2, 2, 2, 2, 2, 2, 2, 2, 2, 2, 2, 2, 2, 2, 2, 2, 2, 2, 2, 2, 2, 2, 2, 2, 2, 2, 2, 2, 2, 2, 2, 2, 2, 2, 2, 2, 2, 2, 2, 2, 2, 2, 2, 2, 2, 2, 2, 2, 2, 2, 2, 2, 2, 2, 2, 2, 2, 2, 2, 2, 2, 2, 2, 2, 2, 2, 2, 2, 2, 2, 2, 2, 2, 2, 2, 2, 2, 2, 2, 2, 2, 2, 2, 2, 2, 2, 2, 2, 2, 2, 2, 2, 2, 2, 2, 2, 2, 2, 2, 2, 2, 2, 2, 2, 2, 2, 2, 2, 2, 2, 2, 2, 2, 2, 2, 2, 2, 2, 2, 2, 2, 2, 2, 2, 2, 2, 2, 2, 2, 2, 2, 2, 2, 2, 2, 2, 2, 2, 2, 2, 2, 2, 2, 2, 2, 2, 2, 2, 2, 2, 2, 2, 2, 2, 2, 2, 2, 2, 2, 2, 2, 2, 2, 2, 2, 2, 2, 2, 2, 2, 2, 2, 2, 2, 2, 2, 2, 2, 2, 2, 2, 2, 2, 2, 2, 2, 2, 2, 2, 2, 2, 2, 2, 2, 2, 2, 2, 2, 2, 2, 2, 2, 2, 2, 2, 2, 2, 2, 2, 2, 2, 2, 2, 2, 2, 2, 2, 2, 2, 2, 2, 2, 2, 2, 2, 2, 2, 2, 2, 2, 2, 2, 2, 2, 2, 2, 2, 2, 2, 2, 2, 2, 2, 2, 2, 2, 2, 2, 2, 2, 2, 2, 2, 2, 2, 2, 2, 2, 2, 2, 2, 2, 2, 2, 2, 2, 2, 2, 2, 2, 2, 2, 2, 2, 2, 2, 2, 2, 2, 2, 2, 2, 2, 2, 2, 2, 2, 2, 2, 2, 2, 2, 2, 2, 2, 2, 2, 2, 2, 2, 2, 2, 2, 2, 2, 2, 2, 2, 2, 2, 2, 2, 2, 2, 2, 2, 2, 2, 2, 2, 2, 2, 2, 2, 2, 2, 2, 2, 2, 2, 2, 2, 2, 2, 2, 2, 2, 2, 2, 2, 2, 2, 2, 2, 2, 2, 2, 2, 2, 2, 2, 2, 2, 2, 2, 2, 2, 2, 2, 2, 2, 2, 2, 2, 2, 2, 2, 2, 2, 2, 2, 2, 2, 2, 2, 2, 2, 2, 2, 2, 2, 2, 2, 2, 2, 2, 2, 2, 2, 2, 2, 2, 2, 2, 2, 2, 2, 2, 2, 2, 2, 2, 2, 2, 2, 2, 2, 2, 2, 2, 2, 2, 2, 2, 2, 2, 2, 2, 2, 2, 2, 2, 2, 2, 2, 2, 2, 2, 2, 2, 2, 2, 2, 2, 2, 2, 2, 2, 2, 2, 2, 2, 2, 2, 2, 2, 2, 2, 2, 2, 2, 2, 2, 2, 2, 2, 2, 2, 2, 2, 2, 2, 2, 2, 2, 2, 2, 2, 2, 2, 2, 2, 2, 2, 2, 2, 2, 2, 2, 2, 2, 2, 2, 2, 2, 2, 2, 2, 2, 2, 2, 2, 2, 2, 2, 2, 2, 2, 2, 2, 2, 2, 2, 2, 2, 2, 2, 2, 2, 2, 2, 2, 2, 2, 2, 2, 2, 2, 2, 2, 2, 2, 2, 2, 2, 2, 2, 2, 2, 2, 2, 2, 2, 2, 2, 2, 2, 2, 2, 2, 2, 2, 2, 2, 2, 2, 2, 2, 2, 2, 2, 2, 2, 2, 2, 2, 2, 2, 2, 2, 2, 2, 2, 2, 2, 2, 2, 2, 2, 2, 2, 2, 2, 2, 2, 2, 2, 2, 2, 2, 2, 2, 2, 2, 2, 2, 2, 2, 2, 2, 2, 2, 2, 2, 2, 2, 2, 2, 2, 2, 2, 2, 2, 2, 2, 2, 2, 2, 2, 2, 2, 2, 2, 2, 2, 2, 2, 2, 2, 2, 2, 2, 2, 2, 2, 2, 2, 2, 2, 2, 2, 2, 2, 2, 2, 2, 2, 2, 2, 2, 2, 2, 2, 2, 2, 2, 2, 2, 2, 2, 2, 2, 2, 2, 2, 2, 2, 2, 2, 2, 2, 2, 2, 2, 2, 2, 2, 2, 2, 2, 2, 2, 2, 2, 2, 2, 2, 2, 2, 2, 2, 2, 2, 2, 2, 2, 2, 2, 2, 2, 2, 2, 2, 2, 2, 2, 2, 2, 2, 2, 2, 2, 2, 2, 2, 2, 2, 2, 2, 2, 2, 2, 2, 2, 2, 2, 2, 2, 2, 2, 2, 2, 2, 2, 2, 2, 2, 2, 2, 2, 2, 2, 2, 2, 2, 2, 2, 2, 2, 2, 2, 2, 2, 2, 2, 2, 2, 2, 2, 2, 2, 2, 2, 2, 2, 2, 2, 2, 2, 2, 2, 2, 2, 2, 2, 2, 2, 2, 2, 2, 2, 2, 2, 2, 2, 2, 2, 2, 2, 2, 2, 2, 2, 2, 2, 2, 2, 2, 2, 2, 2, 3 ),
 ( 0.000000000000000000, 1.000000000000000000 ),
 ( 0.000000000000000000, 0.001190476190476190584, 0.002380952380952381167, 0.003571428571428571317, 0.004761904761904762334, 0.005952380952380952051, 0.007142857142857142634, 0.008333333333333333218, 0.009523809523809524669, 0.01071428571428571438, 0.01190476190476190410, 0.01309523809523809555, 0.01428571428571428527, 0.01547619047619047672, 0.01666666666666666644, 0.01785714285714285615, 0.01904761904761904934, 0.02023809523809523905, 0.02142857142857142877, 0.02261904761904761849, 0.02380952380952380820, 0.02500000000000000139, 0.02619047619047619110, 0.02738095238095238082, 0.02857142857142857054, 0.02976190476190476025, 0.03095238095238095344, 0.03214285714285713969, 0.03333333333333333287, 0.03452380952380952606, 0.03571428571428571230, 0.03690476190476190549, 0.03809523809523809867, 0.03928571428571428492, 0.04047619047619047811, 0.04166666666666666435, 0.04285714285714285754, 0.04404761904761905073, 0.04523809523809523697, 0.04642857142857143016, 0.04761904761904761640, 0.04880952380952380959, 0.05000000000000000278, 0.05119047619047618902, 0.05238095238095238221, 0.05357142857142856845, 0.05476190476190476164, 0.05595238095238095483, 0.05714285714285714107, 0.05833333333333333426, 0.05952380952380952051, 0.06071428571428571369, 0.06190476190476190688, 0.06309523809523809312, 0.06428571428571427937, 0.06547619047619047949, 0.06666666666666666574, 0.06785714285714285199, 0.06904761904761905211, 0.07023809523809523836, 0.07142857142857142461, 0.07261904761904762473, 0.07380952380952381098, 0.07499999999999999722, 0.07619047619047619735, 0.07738095238095238360, 0.07857142857142856984, 0.07976190476190475609, 0.08095238095238095621, 0.08214285714285714246, 0.08333333333333332871, 0.08452380952380952883, 0.08571428571428571508, 0.08690476190476190133, 0.08809523809523810145, 0.08928571428571428770, 0.09047619047619047394, 0.09166666666666666019, 0.09285714285714286031, 0.09404761904761904656, 0.09523809523809523281, 0.09642857142857143293, 0.09761904761904761918, 0.09880952380952380543, 0.1000000000000000056, 0.1011904761904761918, 0.1023809523809523780, 0.1035714285714285782, 0.1047619047619047644, 0.1059523809523809507, 0.1071428571428571369, 0.1083333333333333370, 0.1095238095238095233, 0.1107142857142857095, 0.1119047619047619097, 0.1130952380952380959, 0.1142857142857142821, 0.1154761904761904823, 0.1166666666666666685, 0.1178571428571428548, 0.1190476190476190410, 0.1202380952380952411, 0.1214285714285714274, 0.1226190476190476136, 0.1238095238095238138, 0.1250000000000000000, 0.1261904761904761862, 0.1273809523809523725, 0.1285714285714285587, 0.1297619047619047727, 0.1309523809523809590, 0.1321428571428571452, 0.1333333333333333315, 0.1345238095238095177, 0.1357142857142857040, 0.1369047619047619180, 0.1380952380952381042, 0.1392857142857142905, 0.1404761904761904767, 0.1416666666666666630, 0.1428571428571428492, 0.1440476190476190355, 0.1452380952380952495, 0.1464285714285714357, 0.1476190476190476220, 0.1488095238095238082, 0.1499999999999999944, 0.1511904761904761807, 0.1523809523809523947, 0.1535714285714285809, 0.1547619047619047672, 0.1559523809523809534, 0.1571428571428571397, 0.1583333333333333259, 0.1595238095238095122, 0.1607142857142857262, 0.1619047619047619124, 0.1630952380952380987, 0.1642857142857142849, 0.1654761904761904712, 0.1666666666666666574, 0.1678571428571428437, 0.1690476190476190577, 0.1702380952380952439, 0.1714285714285714302, 0.1726190476190476164, 0.1738095238095238027, 0.1749999999999999889, 0.1761904761904762029, 0.1773809523809523891, 0.1785714285714285754, 0.1797619047619047616, 0.1809523809523809479, 0.1821428571428571341, 0.1833333333333333204, 0.1845238095238095344, 0.1857142857142857206, 0.1869047619047619069, 0.1880952380952380931, 0.1892857142857142794, 0.1904761904761904656, 0.1916666666666666796, 0.1928571428571428659, 0.1940476190476190521, 0.1952380952380952384, 0.1964285714285714246, 0.1976190476190476109, 0.1988095238095237971, 0.2000000000000000111, 0.2011904761904761973, 0.2023809523809523836, 0.2035714285714285698, 0.2047619047619047561, 0.2059523809523809423, 0.2071428571428571563, 0.2083333333333333426, 0.2095238095238095288, 0.2107142857142857151, 0.2119047619047619013, 0.2130952380952380876, 0.2142857142857142738, 0.2154761904761904878, 0.2166666666666666741, 0.2178571428571428603, 0.2190476190476190466, 0.2202380952380952328, 0.2214285714285714191, 0.2226190476190476053, 0.2238095238095238193, 0.2250000000000000056, 0.2261904761904761918, 0.2273809523809523780, 0.2285714285714285643, 0.2297619047619047505, 0.2309523809523809645, 0.2321428571428571508, 0.2333333333333333370, 0.2345238095238095233, 0.2357142857142857095, 0.2369047619047618958, 0.2380952380952380820, 0.2392857142857142960, 0.2404761904761904823, 0.2416666666666666685, 0.2428571428571428548, 0.2440476190476190410, 0.2452380952380952273, 0.2464285714285714413, 0.2476190476190476275, 0.2488095238095238138, 0.2500000000000000000, 0.2511904761904761862, 0.2523809523809523725, 0.2535714285714285587, 0.2547619047619047450, 0.2559523809523809312, 0.2571428571428571175, 0.2583333333333333592, 0.2595238095238095455, 0.2607142857142857317, 0.2619047619047619180, 0.2630952380952381042, 0.2642857142857142905, 0.2654761904761904767, 0.2666666666666666630, 0.2678571428571428492, 0.2690476190476190355, 0.2702380952380952217, 0.2714285714285714080, 0.2726190476190475942, 0.2738095238095238360, 0.2750000000000000222, 0.2761904761904762085, 0.2773809523809523947, 0.2785714285714285809, 0.2797619047619047672, 0.2809523809523809534, 0.2821428571428571397, 0.2833333333333333259, 0.2845238095238095122, 0.2857142857142856984, 0.2869047619047618847, 0.2880952380952380709, 0.2892857142857143127, 0.2904761904761904989, 0.2916666666666666852, 0.2928571428571428714, 0.2940476190476190577, 0.2952380952380952439, 0.2964285714285714302, 0.2976190476190476164, 0.2988095238095238027, 0.2999999999999999889, 0.3011904761904761751, 0.3023809523809523614, 0.3035714285714285476, 0.3047619047619047894, 0.3059523809523809756, 0.3071428571428571619, 0.3083333333333333481, 0.3095238095238095344, 0.3107142857142857206, 0.3119047619047619069, 0.3130952380952380931, 0.3142857142857142794, 0.3154761904761904656, 0.3166666666666666519, 0.3178571428571428381, 0.3190476190476190244, 0.3202380952380952106, 0.3214285714285714524, 0.3226190476190476386, 0.3238095238095238249, 0.3250000000000000111, 0.3261904761904761973, 0.3273809523809523836, 0.3285714285714285698, 0.3297619047619047561, 0.3309523809523809423, 0.3321428571428571286, 0.3333333333333333148, 0.3345238095238095011, 0.3357142857142856873, 0.3369047619047619291, 0.3380952380952381153, 0.3392857142857143016, 0.3404761904761904878, 0.3416666666666666741, 0.3428571428571428603, 0.3440476190476190466, 0.3452380952380952328, 0.3464285714285714191, 0.3476190476190476053, 0.3488095238095237915, 0.3499999999999999778, 0.3511904761904761640, 0.3523809523809524058, 0.3535714285714285920, 0.3547619047619047783, 0.3559523809523809645, 0.3571428571428571508, 0.3583333333333333370, 0.3595238095238095233, 0.3607142857142857095, 0.3619047619047618958, 0.3630952380952380820, 0.3642857142857142683, 0.3654761904761904545, 0.3666666666666666408, 0.3678571428571428825, 0.3690476190476190688, 0.3702380952380952550, 0.3714285714285714413, 0.3726190476190476275, 0.3738095238095238138, 0.3750000000000000000, 0.3761904761904761862, 0.3773809523809523725, 0.3785714285714285587, 0.3797619047619047450, 0.3809523809523809312, 0.3821428571428571175, 0.3833333333333333592, 0.3845238095238095455, 0.3857142857142857317, 0.3869047619047619180, 0.3880952380952381042, 0.3892857142857142905, 0.3904761904761904767, 0.3916666666666666630, 0.3928571428571428492, 0.3940476190476190355, 0.3952380952380952217, 0.3964285714285714080, 0.3976190476190475942, 0.3988095238095238360, 0.4000000000000000222, 0.4011904761904762085, 0.4023809523809523947, 0.4035714285714285809, 0.4047619047619047672, 0.4059523809523809534, 0.4071428571428571397, 0.4083333333333333259, 0.4095238095238095122, 0.4107142857142856984, 0.4119047619047618847, 0.4130952380952380709, 0.4142857142857143127, 0.4154761904761904989, 0.4166666666666666852, 0.4178571428571428714, 0.4190476190476190577, 0.4202380952380952439, 0.4214285714285714302, 0.4226190476190476164, 0.4238095238095238027, 0.4249999999999999889, 0.4261904761904761751, 0.4273809523809523614, 0.4285714285714285476, 0.4297619047619047894, 0.4309523809523809756, 0.4321428571428571619, 0.4333333333333333481, 0.4345238095238095344, 0.4357142857142857206, 0.4369047619047619069, 0.4380952380952380931, 0.4392857142857142794, 0.4404761904761904656, 0.4416666666666666519, 0.4428571428571428381, 0.4440476190476190244, 0.4452380952380952106, 0.4464285714285714524, 0.4476190476190476386, 0.4488095238095238249, 0.4500000000000000111, 0.4511904761904761973, 0.4523809523809523836, 0.4535714285714285698, 0.4547619047619047561, 0.4559523809523809423, 0.4571428571428571286, 0.4583333333333333148, 0.4595238095238095011, 0.4607142857142856873, 0.4619047619047619291, 0.4630952380952381153, 0.4642857142857143016, 0.4654761904761904878, 0.4666666666666666741, 0.4678571428571428603, 0.4690476190476190466, 0.4702380952380952328, 0.4714285714285714191, 0.4726190476190476053, 0.4738095238095237915, 0.4749999999999999778, 0.4761904761904761640, 0.4773809523809524058, 0.4785714285714285920, 0.4797619047619047783, 0.4809523809523809645, 0.4821428571428571508, 0.4833333333333333370, 0.4845238095238095233, 0.4857142857142857095, 0.4869047619047618958, 0.4880952380952380820, 0.4892857142857142683, 0.4904761904761904545, 0.4916666666666666408, 0.4928571428571428825, 0.4940476190476190688, 0.4952380952380952550, 0.4964285714285714413, 0.4976190476190476275, 0.4988095238095238138, 0.5000000000000000000, 0.5011904761904761862, 0.5023809523809523725, 0.5035714285714285587, 0.5047619047619047450, 0.5059523809523809312, 0.5071428571428571175, 0.5083333333333333037, 0.5095238095238094900, 0.5107142857142856762, 0.5119047619047618625, 0.5130952380952380487, 0.5142857142857142350, 0.5154761904761904212, 0.5166666666666667185, 0.5178571428571429047, 0.5190476190476190910, 0.5202380952380952772, 0.5214285714285714635, 0.5226190476190476497, 0.5238095238095238360, 0.5250000000000000222, 0.5261904761904762085, 0.5273809523809523947, 0.5285714285714285809, 0.5297619047619047672, 0.5309523809523809534, 0.5321428571428571397, 0.5333333333333333259, 0.5345238095238095122, 0.5357142857142856984, 0.5369047619047618847, 0.5380952380952380709, 0.5392857142857142572, 0.5404761904761904434, 0.5416666666666666297, 0.5428571428571428159, 0.5440476190476190022, 0.5452380952380951884, 0.5464285714285713746, 0.5476190476190476719, 0.5488095238095238582, 0.5500000000000000444, 0.5511904761904762307, 0.5523809523809524169, 0.5535714285714286031, 0.5547619047619047894, 0.5559523809523809756, 0.5571428571428571619, 0.5583333333333333481, 0.5595238095238095344, 0.5607142857142857206, 0.5619047619047619069, 0.5630952380952380931, 0.5642857142857142794, 0.5654761904761904656, 0.5666666666666666519, 0.5678571428571428381, 0.5690476190476190244, 0.5702380952380952106, 0.5714285714285713969, 0.5726190476190475831, 0.5738095238095237693, 0.5749999999999999556, 0.5761904761904761418, 0.5773809523809523281, 0.5785714285714286254, 0.5797619047619048116, 0.5809523809523809978, 0.5821428571428571841, 0.5833333333333333703, 0.5845238095238095566, 0.5857142857142857428, 0.5869047619047619291, 0.5880952380952381153, 0.5892857142857143016, 0.5904761904761904878, 0.5916666666666666741, 0.5928571428571428603, 0.5940476190476190466, 0.5952380952380952328, 0.5964285714285714191, 0.5976190476190476053, 0.5988095238095237915, 0.5999999999999999778, 0.6011904761904761640, 0.6023809523809523503, 0.6035714285714285365, 0.6047619047619047228, 0.6059523809523809090, 0.6071428571428570953, 0.6083333333333332815, 0.6095238095238095788, 0.6107142857142857650, 0.6119047619047619513, 0.6130952380952381375, 0.6142857142857143238, 0.6154761904761905100, 0.6166666666666666963, 0.6178571428571428825, 0.6190476190476190688, 0.6202380952380952550, 0.6214285714285714413, 0.6226190476190476275, 0.6238095238095238138, 0.6250000000000000000, 0.6261904761904761862, 0.6273809523809523725, 0.6285714285714285587, 0.6297619047619047450, 0.6309523809523809312, 0.6321428571428571175, 0.6333333333333333037, 0.6345238095238094900, 0.6357142857142856762, 0.6369047619047618625, 0.6380952380952380487, 0.6392857142857142350, 0.6404761904761904212, 0.6416666666666667185, 0.6428571428571429047, 0.6440476190476190910, 0.6452380952380952772, 0.6464285714285714635, 0.6476190476190476497, 0.6488095238095238360, 0.6500000000000000222, 0.6511904761904762085, 0.6523809523809523947, 0.6535714285714285809, 0.6547619047619047672, 0.6559523809523809534, 0.6571428571428571397, 0.6583333333333333259, 0.6595238095238095122, 0.6607142857142856984, 0.6619047619047618847, 0.6630952380952380709, 0.6642857142857142572, 0.6654761904761904434, 0.6666666666666666297, 0.6678571428571428159, 0.6690476190476190022, 0.6702380952380951884, 0.6714285714285713746, 0.6726190476190476719, 0.6738095238095238582, 0.6750000000000000444, 0.6761904761904762307, 0.6773809523809524169, 0.6785714285714286031, 0.6797619047619047894, 0.6809523809523809756, 0.6821428571428571619, 0.6833333333333333481, 0.6845238095238095344, 0.6857142857142857206, 0.6869047619047619069, 0.6880952380952380931, 0.6892857142857142794, 0.6904761904761904656, 0.6916666666666666519, 0.6928571428571428381, 0.6940476190476190244, 0.6952380952380952106, 0.6964285714285713969, 0.6976190476190475831, 0.6988095238095237693, 0.6999999999999999556, 0.7011904761904761418, 0.7023809523809523281, 0.7035714285714286254, 0.7047619047619048116, 0.7059523809523809978, 0.7071428571428571841, 0.7083333333333333703, 0.7095238095238095566, 0.7107142857142857428, 0.7119047619047619291, 0.7130952380952381153, 0.7142857142857143016, 0.7154761904761904878, 0.7166666666666666741, 0.7178571428571428603, 0.7190476190476190466, 0.7202380952380952328, 0.7214285714285714191, 0.7226190476190476053, 0.7238095238095237915, 0.7249999999999999778, 0.7261904761904761640, 0.7273809523809523503, 0.7285714285714285365, 0.7297619047619047228, 0.7309523809523809090, 0.7321428571428570953, 0.7333333333333332815, 0.7345238095238095788, 0.7357142857142857650, 0.7369047619047619513, 0.7380952380952381375, 0.7392857142857143238, 0.7404761904761905100, 0.7416666666666666963, 0.7428571428571428825, 0.7440476190476190688, 0.7452380952380952550, 0.7464285714285714413, 0.7476190476190476275, 0.7488095238095238138, 0.7500000000000000000, 0.7511904761904761862, 0.7523809523809523725, 0.7535714285714285587, 0.7547619047619047450, 0.7559523809523809312, 0.7571428571428571175, 0.7583333333333333037, 0.7595238095238094900, 0.7607142857142856762, 0.7619047619047618625, 0.7630952380952380487, 0.7642857142857142350, 0.7654761904761904212, 0.7666666666666667185, 0.7678571428571429047, 0.7690476190476190910, 0.7702380952380952772, 0.7714285714285714635, 0.7726190476190476497, 0.7738095238095238360, 0.7750000000000000222, 0.7761904761904762085, 0.7773809523809523947, 0.7785714285714285809, 0.7797619047619047672, 0.7809523809523809534, 0.7821428571428571397, 0.7833333333333333259, 0.7845238095238095122, 0.7857142857142856984, 0.7869047619047618847, 0.7880952380952380709, 0.7892857142857142572, 0.7904761904761904434, 0.7916666666666666297, 0.7928571428571428159, 0.7940476190476190022, 0.7952380952380951884, 0.7964285714285713746, 0.7976190476190476719, 0.7988095238095238582, 0.8000000000000000444, 0.8011904761904762307, 0.8023809523809524169, 0.8035714285714286031, 0.8047619047619047894, 0.8059523809523809756, 0.8071428571428571619, 0.8083333333333333481, 0.8095238095238095344, 0.8107142857142857206, 0.8119047619047619069, 0.8130952380952380931, 0.8142857142857142794, 0.8154761904761904656, 0.8166666666666666519, 0.8178571428571428381, 0.8190476190476190244, 0.8202380952380952106, 0.8214285714285713969, 0.8226190476190475831, 0.8238095238095237693, 0.8249999999999999556, 0.8261904761904761418, 0.8273809523809523281, 0.8285714285714286254, 0.8297619047619048116, 0.8309523809523809978, 0.8321428571428571841, 0.8333333333333333703, 0.8345238095238095566, 0.8357142857142857428, 0.8369047619047619291, 0.8380952380952381153, 0.8392857142857143016, 0.8404761904761904878, 0.8416666666666666741, 0.8428571428571428603, 0.8440476190476190466, 0.8452380952380952328, 0.8464285714285714191, 0.8476190476190476053, 0.8488095238095237915, 0.8499999999999999778, 0.8511904761904761640, 0.8523809523809523503, 0.8535714285714285365, 0.8547619047619047228, 0.8559523809523809090, 0.8571428571428570953, 0.8583333333333332815, 0.8595238095238095788, 0.8607142857142857650, 0.8619047619047619513, 0.8630952380952381375, 0.8642857142857143238, 0.8654761904761905100, 0.8666666666666666963, 0.8678571428571428825, 0.8690476190476190688, 0.8702380952380952550, 0.8714285714285714413, 0.8726190476190476275, 0.8738095238095238138, 0.8750000000000000000, 0.8761904761904761862, 0.8773809523809523725, 0.8785714285714285587, 0.8797619047619047450, 0.8809523809523809312, 0.8821428571428571175, 0.8833333333333333037, 0.8845238095238094900, 0.8857142857142856762, 0.8869047619047618625, 0.8880952380952380487, 0.8892857142857142350, 0.8904761904761904212, 0.8916666666666667185, 0.8928571428571429047, 0.8940476190476190910, 0.8952380952380952772, 0.8964285714285714635, 0.8976190476190476497, 0.8988095238095238360, 0.9000000000000000222, 0.9011904761904762085, 0.9023809523809523947, 0.9035714285714285809, 0.9047619047619047672, 0.9059523809523809534, 0.9071428571428571397, 0.9083333333333333259, 0.9095238095238095122, 0.9107142857142856984, 0.9119047619047618847, 0.9130952380952380709, 0.9142857142857142572, 0.9154761904761904434, 0.9166666666666666297, 0.9178571428571428159, 0.9190476190476190022, 0.9202380952380951884, 0.9214285714285713746, 0.9226190476190476719, 0.9238095238095238582, 0.9250000000000000444, 0.9261904761904762307, 0.9273809523809524169, 0.9285714285714286031, 0.9297619047619047894, 0.9309523809523809756, 0.9321428571428571619, 0.9333333333333333481, 0.9345238095238095344, 0.9357142857142857206, 0.9369047619047619069, 0.9380952380952380931, 0.9392857142857142794, 0.9404761904761904656, 0.9416666666666666519, 0.9428571428571428381, 0.9440476190476190244, 0.9452380952380952106, 0.9464285714285713969, 0.9476190476190475831, 0.9488095238095237693, 0.9499999999999999556, 0.9511904761904761418, 0.9523809523809523281, 0.9535714285714286254, 0.9547619047619048116, 0.9559523809523809978, 0.9571428571428571841, 0.9583333333333333703, 0.9595238095238095566, 0.9607142857142857428, 0.9619047619047619291, 0.9630952380952381153, 0.9642857142857143016, 0.9654761904761904878, 0.9666666666666666741, 0.9678571428571428603, 0.9690476190476190466, 0.9702380952380952328, 0.9714285714285714191, 0.9726190476190476053, 0.9738095238095237915, 0.9749999999999999778, 0.9761904761904761640, 0.9773809523809523503, 0.9785714285714285365, 0.9797619047619047228, 0.9809523809523809090, 0.9821428571428570953, 0.9833333333333332815, 0.9845238095238095788, 0.9857142857142857650, 0.9869047619047619513, 0.9880952380952381375, 0.9892857142857143238, 0.9904761904761905100, 0.9916666666666666963, 0.9928571428571428825, 0.9940476190476190688, 0.9952380952380952550, 0.9964285714285714413, 0.9976190476190476275, 0.9988095238095238138, 1.000000000000000000 ),
 .UNSPECIFIED. ) 
 GEOMETRIC_REPRESENTATION_ITEM ( )  RATIONAL_B_SPLINE_SURFACE ( (
 ( 1.000000000000000000, 0.8660254037844387076, 1.000000000000000000, 0.8660254037844387076, 1.000000000000000000, 0.8660254037844387076, 1.000000000000000000, 0.8660254037844387076, 1.000000000000000000, 0.8660254037844387076, 1.000000000000000000, 0.8660254037844387076, 1.000000000000000000, 0.8660254037844387076, 1.000000000000000000, 0.8660254037844387076, 1.000000000000000000, 0.8660254037844387076, 1.000000000000000000, 0.8660254037844387076, 1.000000000000000000, 0.8660254037844387076, 1.000000000000000000, 0.8660254037844387076, 1.000000000000000000, 0.8660254037844387076, 1.000000000000000000, 0.8660254037844387076, 1.000000000000000000, 0.8660254037844387076, 1.000000000000000000, 0.8660254037844387076, 1.000000000000000000, 0.8660254037844387076, 1.000000000000000000, 0.8660254037844387076, 1.000000000000000000, 0.8660254037844387076, 1.000000000000000000, 0.8660254037844387076, 1.000000000000000000, 0.8660254037844387076, 1.000000000000000000, 0.8660254037844387076, 1.000000000000000000, 0.8660254037844387076, 1.000000000000000000, 0.8660254037844387076, 1.000000000000000000, 0.8660254037844387076, 1.000000000000000000, 0.8660254037844387076, 1.000000000000000000, 0.8660254037844387076, 1.000000000000000000, 0.8660254037844387076, 1.000000000000000000, 0.8660254037844387076, 1.000000000000000000, 0.8660254037844387076, 1.000000000000000000, 0.8660254037844387076, 1.000000000000000000, 0.8660254037844387076, 1.000000000000000000, 0.8660254037844387076, 1.000000000000000000, 0.8660254037844387076, 1.000000000000000000, 0.8660254037844387076, 1.000000000000000000, 0.8660254037844387076, 1.000000000000000000, 0.8660254037844387076, 1.000000000000000000, 0.8660254037844387076, 1.000000000000000000, 0.8660254037844387076, 1.000000000000000000, 0.8660254037844387076, 1.000000000000000000, 0.8660254037844387076, 1.000000000000000000, 0.8660254037844387076, 1.000000000000000000, 0.8660254037844387076, 1.000000000000000000, 0.8660254037844387076, 1.000000000000000000, 0.8660254037844387076, 1.000000000000000000, 0.8660254037844387076, 1.000000000000000000, 0.8660254037844387076, 1.000000000000000000, 0.8660254037844387076, 1.000000000000000000, 0.8660254037844387076, 1.000000000000000000, 0.8660254037844387076, 1.000000000000000000, 0.8660254037844387076, 1.000000000000000000, 0.8660254037844387076, 1.000000000000000000, 0.8660254037844387076, 1.000000000000000000, 0.8660254037844387076, 1.000000000000000000, 0.8660254037844387076, 1.000000000000000000, 0.8660254037844387076, 1.000000000000000000, 0.8660254037844387076, 1.000000000000000000, 0.8660254037844387076, 1.000000000000000000, 0.8660254037844387076, 1.000000000000000000, 0.8660254037844387076, 1.000000000000000000, 0.8660254037844387076, 1.000000000000000000, 0.8660254037844387076, 1.000000000000000000, 0.8660254037844387076, 1.000000000000000000, 0.8660254037844387076, 1.000000000000000000, 0.8660254037844387076, 1.000000000000000000, 0.8660254037844387076, 1.000000000000000000, 0.8660254037844387076, 1.000000000000000000, 0.8660254037844387076, 1.000000000000000000, 0.8660254037844387076, 1.000000000000000000, 0.8660254037844387076, 1.000000000000000000, 0.8660254037844387076, 1.000000000000000000, 0.8660254037844387076, 1.000000000000000000, 0.8660254037844387076, 1.000000000000000000, 0.8660254037844387076, 1.000000000000000000, 0.8660254037844387076, 1.000000000000000000, 0.8660254037844387076, 1.000000000000000000, 0.8660254037844387076, 1.000000000000000000, 0.8660254037844387076, 1.000000000000000000, 0.8660254037844387076, 1.000000000000000000, 0.8660254037844387076, 1.000000000000000000, 0.8660254037844387076, 1.000000000000000000, 0.8660254037844387076, 1.000000000000000000, 0.8660254037844387076, 1.000000000000000000, 0.8660254037844387076, 1.000000000000000000, 0.8660254037844387076, 1.000000000000000000, 0.8660254037844387076, 1.000000000000000000, 0.8660254037844387076, 1.000000000000000000, 0.8660254037844387076, 1.000000000000000000, 0.8660254037844387076, 1.000000000000000000, 0.8660254037844387076, 1.000000000000000000, 0.8660254037844387076, 1.000000000000000000, 0.8660254037844387076, 1.000000000000000000, 0.8660254037844387076, 1.000000000000000000, 0.8660254037844387076, 1.000000000000000000, 0.8660254037844387076, 1.000000000000000000, 0.8660254037844387076, 1.000000000000000000, 0.8660254037844387076, 1.000000000000000000, 0.8660254037844387076, 1.000000000000000000, 0.8660254037844387076, 1.000000000000000000, 0.8660254037844387076, 1.000000000000000000, 0.8660254037844387076, 1.000000000000000000, 0.8660254037844387076, 1.000000000000000000, 0.8660254037844387076, 1.000000000000000000, 0.8660254037844387076, 1.000000000000000000, 0.8660254037844387076, 1.000000000000000000, 0.8660254037844387076, 1.000000000000000000, 0.8660254037844387076, 1.000000000000000000, 0.8660254037844387076, 1.000000000000000000, 0.8660254037844387076, 1.000000000000000000, 0.8660254037844387076, 1.000000000000000000, 0.8660254037844387076, 1.000000000000000000, 0.8660254037844387076, 1.000000000000000000, 0.8660254037844387076, 1.000000000000000000, 0.8660254037844387076, 1.000000000000000000, 0.8660254037844387076, 1.000000000000000000, 0.8660254037844387076, 1.000000000000000000, 0.8660254037844387076, 1.000000000000000000, 0.8660254037844387076, 1.000000000000000000, 0.8660254037844387076, 1.000000000000000000, 0.8660254037844387076, 1.000000000000000000, 0.8660254037844387076, 1.000000000000000000, 0.8660254037844387076, 1.000000000000000000, 0.8660254037844387076, 1.000000000000000000, 0.8660254037844387076, 1.000000000000000000, 0.8660254037844387076, 1.000000000000000000, 0.8660254037844387076, 1.000000000000000000, 0.8660254037844387076, 1.000000000000000000, 0.8660254037844387076, 1.000000000000000000, 0.8660254037844387076, 1.000000000000000000, 0.8660254037844387076, 1.000000000000000000, 0.8660254037844387076, 1.000000000000000000, 0.8660254037844387076, 1.000000000000000000, 0.8660254037844387076, 1.000000000000000000, 0.8660254037844387076, 1.000000000000000000, 0.8660254037844387076, 1.000000000000000000, 0.8660254037844387076, 1.000000000000000000, 0.8660254037844387076, 1.000000000000000000, 0.8660254037844387076, 1.000000000000000000, 0.8660254037844387076, 1.000000000000000000, 0.8660254037844387076, 1.000000000000000000, 0.8660254037844387076, 1.000000000000000000, 0.8660254037844387076, 1.000000000000000000, 0.8660254037844387076, 1.000000000000000000, 0.8660254037844387076, 1.000000000000000000, 0.8660254037844387076, 1.000000000000000000, 0.8660254037844387076, 1.000000000000000000, 0.8660254037844387076, 1.000000000000000000, 0.8660254037844387076, 1.000000000000000000, 0.8660254037844387076, 1.000000000000000000, 0.8660254037844387076, 1.000000000000000000, 0.8660254037844387076, 1.000000000000000000, 0.8660254037844387076, 1.000000000000000000, 0.8660254037844387076, 1.000000000000000000, 0.8660254037844387076, 1.000000000000000000, 0.8660254037844387076, 1.000000000000000000, 0.8660254037844387076, 1.000000000000000000, 0.8660254037844387076, 1.000000000000000000, 0.8660254037844387076, 1.000000000000000000, 0.8660254037844387076, 1.000000000000000000, 0.8660254037844387076, 1.000000000000000000, 0.8660254037844387076, 1.000000000000000000, 0.8660254037844387076, 1.000000000000000000, 0.8660254037844387076, 1.000000000000000000, 0.8660254037844387076, 1.000000000000000000, 0.8660254037844387076, 1.000000000000000000, 0.8660254037844387076, 1.000000000000000000, 0.8660254037844387076, 1.000000000000000000, 0.8660254037844387076, 1.000000000000000000, 0.8660254037844387076, 1.000000000000000000, 0.8660254037844387076, 1.000000000000000000, 0.8660254037844387076, 1.000000000000000000, 0.8660254037844387076, 1.000000000000000000, 0.8660254037844387076, 1.000000000000000000, 0.8660254037844387076, 1.000000000000000000, 0.8660254037844387076, 1.000000000000000000, 0.8660254037844387076, 1.000000000000000000, 0.8660254037844387076, 1.000000000000000000, 0.8660254037844387076, 1.000000000000000000, 0.8660254037844387076, 1.000000000000000000, 0.8660254037844387076, 1.000000000000000000, 0.8660254037844387076, 1.000000000000000000, 0.8660254037844387076, 1.000000000000000000, 0.8660254037844387076, 1.000000000000000000, 0.8660254037844387076, 1.000000000000000000, 0.8660254037844387076, 1.000000000000000000, 0.8660254037844387076, 1.000000000000000000, 0.8660254037844387076, 1.000000000000000000, 0.8660254037844387076, 1.000000000000000000, 0.8660254037844387076, 1.000000000000000000, 0.8660254037844387076, 1.000000000000000000, 0.8660254037844387076, 1.000000000000000000, 0.8660254037844387076, 1.000000000000000000, 0.8660254037844387076, 1.000000000000000000, 0.8660254037844387076, 1.000000000000000000, 0.8660254037844387076, 1.000000000000000000, 0.8660254037844387076, 1.000000000000000000, 0.8660254037844387076, 1.000000000000000000, 0.8660254037844387076, 1.000000000000000000, 0.8660254037844387076, 1.000000000000000000, 0.8660254037844387076, 1.000000000000000000, 0.8660254037844387076, 1.000000000000000000, 0.8660254037844387076, 1.000000000000000000, 0.8660254037844387076, 1.000000000000000000, 0.8660254037844387076, 1.000000000000000000, 0.8660254037844387076, 1.000000000000000000, 0.8660254037844387076, 1.000000000000000000, 0.8660254037844387076, 1.000000000000000000, 0.8660254037844387076, 1.000000000000000000, 0.8660254037844387076, 1.000000000000000000, 0.8660254037844387076, 1.000000000000000000, 0.8660254037844387076, 1.000000000000000000, 0.8660254037844387076, 1.000000000000000000, 0.8660254037844387076, 1.000000000000000000, 0.8660254037844387076, 1.000000000000000000, 0.8660254037844387076, 1.000000000000000000, 0.8660254037844387076, 1.000000000000000000, 0.8660254037844387076, 1.000000000000000000, 0.8660254037844387076, 1.000000000000000000, 0.8660254037844387076, 1.000000000000000000, 0.8660254037844387076, 1.000000000000000000, 0.8660254037844387076, 1.000000000000000000, 0.8660254037844387076, 1.000000000000000000, 0.8660254037844387076, 1.000000000000000000, 0.8660254037844387076, 1.000000000000000000, 0.8660254037844387076, 1.000000000000000000, 0.8660254037844387076, 1.000000000000000000, 0.8660254037844387076, 1.000000000000000000, 0.8660254037844387076, 1.000000000000000000, 0.8660254037844387076, 1.000000000000000000, 0.8660254037844387076, 1.000000000000000000, 0.8660254037844387076, 1.000000000000000000, 0.8660254037844387076, 1.000000000000000000, 0.8660254037844387076, 1.000000000000000000, 0.8660254037844387076, 1.000000000000000000, 0.8660254037844387076, 1.000000000000000000, 0.8660254037844387076, 1.000000000000000000, 0.8660254037844387076, 1.000000000000000000, 0.8660254037844387076, 1.000000000000000000, 0.8660254037844387076, 1.000000000000000000, 0.8660254037844387076, 1.000000000000000000, 0.8660254037844387076, 1.000000000000000000, 0.8660254037844387076, 1.000000000000000000, 0.8660254037844387076, 1.000000000000000000, 0.8660254037844387076, 1.000000000000000000, 0.8660254037844387076, 1.000000000000000000, 0.8660254037844387076, 1.000000000000000000, 0.8660254037844387076, 1.000000000000000000, 0.8660254037844387076, 1.000000000000000000, 0.8660254037844387076, 1.000000000000000000, 0.8660254037844387076, 1.000000000000000000, 0.8660254037844387076, 1.000000000000000000, 0.8660254037844387076, 1.000000000000000000, 0.8660254037844387076, 1.000000000000000000, 0.8660254037844387076, 1.000000000000000000, 0.8660254037844387076, 1.000000000000000000, 0.8660254037844387076, 1.000000000000000000, 0.8660254037844387076, 1.000000000000000000, 0.8660254037844387076, 1.000000000000000000, 0.8660254037844387076, 1.000000000000000000, 0.8660254037844387076, 1.000000000000000000, 0.8660254037844387076, 1.000000000000000000, 0.8660254037844387076, 1.000000000000000000, 0.8660254037844387076, 1.000000000000000000, 0.8660254037844387076, 1.000000000000000000, 0.8660254037844387076, 1.000000000000000000, 0.8660254037844387076, 1.000000000000000000, 0.8660254037844387076, 1.000000000000000000, 0.8660254037844387076, 1.000000000000000000, 0.8660254037844387076, 1.000000000000000000, 0.8660254037844387076, 1.000000000000000000, 0.8660254037844387076, 1.000000000000000000, 0.8660254037844387076, 1.000000000000000000, 0.8660254037844387076, 1.000000000000000000, 0.8660254037844387076, 1.000000000000000000, 0.8660254037844387076, 1.000000000000000000, 0.8660254037844387076, 1.000000000000000000, 0.8660254037844387076, 1.000000000000000000, 0.8660254037844387076, 1.000000000000000000, 0.8660254037844387076, 1.000000000000000000, 0.8660254037844387076, 1.000000000000000000, 0.8660254037844387076, 1.000000000000000000, 0.8660254037844387076, 1.000000000000000000, 0.8660254037844387076, 1.000000000000000000, 0.8660254037844387076, 1.000000000000000000, 0.8660254037844387076, 1.000000000000000000, 0.8660254037844387076, 1.000000000000000000, 0.8660254037844387076, 1.000000000000000000, 0.8660254037844387076, 1.000000000000000000, 0.8660254037844387076, 1.000000000000000000, 0.8660254037844387076, 1.000000000000000000, 0.8660254037844387076, 1.000000000000000000, 0.8660254037844387076, 1.000000000000000000, 0.8660254037844387076, 1.000000000000000000, 0.8660254037844387076, 1.000000000000000000, 0.8660254037844387076, 1.000000000000000000, 0.8660254037844387076, 1.000000000000000000, 0.8660254037844387076, 1.000000000000000000, 0.8660254037844387076, 1.000000000000000000, 0.8660254037844387076, 1.000000000000000000, 0.8660254037844387076, 1.000000000000000000, 0.8660254037844387076, 1.000000000000000000, 0.8660254037844387076, 1.000000000000000000, 0.8660254037844387076, 1.000000000000000000, 0.8660254037844387076, 1.000000000000000000, 0.8660254037844387076, 1.000000000000000000, 0.8660254037844387076, 1.000000000000000000, 0.8660254037844387076, 1.000000000000000000, 0.8660254037844387076, 1.000000000000000000, 0.8660254037844387076, 1.000000000000000000, 0.8660254037844387076, 1.000000000000000000, 0.8660254037844387076, 1.000000000000000000, 0.8660254037844387076, 1.000000000000000000, 0.8660254037844387076, 1.000000000000000000, 0.8660254037844387076, 1.000000000000000000, 0.8660254037844387076, 1.000000000000000000, 0.8660254037844387076, 1.000000000000000000, 0.8660254037844387076, 1.000000000000000000, 0.8660254037844387076, 1.000000000000000000, 0.8660254037844387076, 1.000000000000000000, 0.8660254037844387076, 1.000000000000000000, 0.8660254037844387076, 1.000000000000000000, 0.8660254037844387076, 1.000000000000000000, 0.8660254037844387076, 1.000000000000000000, 0.8660254037844387076, 1.000000000000000000, 0.8660254037844387076, 1.000000000000000000, 0.8660254037844387076, 1.000000000000000000, 0.8660254037844387076, 1.000000000000000000, 0.8660254037844387076, 1.000000000000000000, 0.8660254037844387076, 1.000000000000000000, 0.8660254037844387076, 1.000000000000000000, 0.8660254037844387076, 1.000000000000000000, 0.8660254037844387076, 1.000000000000000000, 0.8660254037844387076, 1.000000000000000000, 0.8660254037844387076, 1.000000000000000000, 0.8660254037844387076, 1.000000000000000000, 0.8660254037844387076, 1.000000000000000000, 0.8660254037844387076, 1.000000000000000000, 0.8660254037844387076, 1.000000000000000000, 0.8660254037844387076, 1.000000000000000000, 0.8660254037844387076, 1.000000000000000000, 0.8660254037844387076, 1.000000000000000000, 0.8660254037844387076, 1.000000000000000000, 0.8660254037844387076, 1.000000000000000000, 0.8660254037844387076, 1.000000000000000000, 0.8660254037844387076, 1.000000000000000000, 0.8660254037844387076, 1.000000000000000000, 0.8660254037844387076, 1.000000000000000000, 0.8660254037844387076, 1.000000000000000000, 0.8660254037844387076, 1.000000000000000000, 0.8660254037844387076, 1.000000000000000000, 0.8660254037844387076, 1.000000000000000000, 0.8660254037844387076, 1.000000000000000000, 0.8660254037844387076, 1.000000000000000000, 0.8660254037844387076, 1.000000000000000000, 0.8660254037844387076, 1.000000000000000000, 0.8660254037844387076, 1.000000000000000000, 0.8660254037844387076, 1.000000000000000000, 0.8660254037844387076, 1.000000000000000000, 0.8660254037844387076, 1.000000000000000000, 0.8660254037844387076, 1.000000000000000000, 0.8660254037844387076, 1.000000000000000000, 0.8660254037844387076, 1.000000000000000000, 0.8660254037844387076, 1.000000000000000000, 0.8660254037844387076, 1.000000000000000000, 0.8660254037844387076, 1.000000000000000000, 0.8660254037844387076, 1.000000000000000000, 0.8660254037844387076, 1.000000000000000000, 0.8660254037844387076, 1.000000000000000000, 0.8660254037844387076, 1.000000000000000000, 0.8660254037844387076, 1.000000000000000000, 0.8660254037844387076, 1.000000000000000000, 0.8660254037844387076, 1.000000000000000000, 0.8660254037844387076, 1.000000000000000000, 0.8660254037844387076, 1.000000000000000000, 0.8660254037844387076, 1.000000000000000000, 0.8660254037844387076, 1.000000000000000000, 0.8660254037844387076, 1.000000000000000000, 0.8660254037844387076, 1.000000000000000000, 0.8660254037844387076, 1.000000000000000000, 0.8660254037844387076, 1.000000000000000000, 0.8660254037844387076, 1.000000000000000000, 0.8660254037844387076, 1.000000000000000000, 0.8660254037844387076, 1.000000000000000000, 0.8660254037844387076, 1.000000000000000000, 0.8660254037844387076, 1.000000000000000000, 0.8660254037844387076, 1.000000000000000000, 0.8660254037844387076, 1.000000000000000000, 0.8660254037844387076, 1.000000000000000000, 0.8660254037844387076, 1.000000000000000000, 0.8660254037844387076, 1.000000000000000000, 0.8660254037844387076, 1.000000000000000000, 0.8660254037844387076, 1.000000000000000000, 0.8660254037844387076, 1.000000000000000000, 0.8660254037844387076, 1.000000000000000000, 0.8660254037844387076, 1.000000000000000000, 0.8660254037844387076, 1.000000000000000000, 0.8660254037844387076, 1.000000000000000000, 0.8660254037844387076, 1.000000000000000000, 0.8660254037844387076, 1.000000000000000000, 0.8660254037844387076, 1.000000000000000000, 0.8660254037844387076, 1.000000000000000000, 0.8660254037844387076, 1.000000000000000000, 0.8660254037844387076, 1.000000000000000000, 0.8660254037844387076, 1.000000000000000000, 0.8660254037844387076, 1.000000000000000000, 0.8660254037844387076, 1.000000000000000000, 0.8660254037844387076, 1.000000000000000000, 0.8660254037844387076, 1.000000000000000000, 0.8660254037844387076, 1.000000000000000000, 0.8660254037844387076, 1.000000000000000000, 0.8660254037844387076, 1.000000000000000000, 0.8660254037844387076, 1.000000000000000000, 0.8660254037844387076, 1.000000000000000000, 0.8660254037844387076, 1.000000000000000000, 0.8660254037844387076, 1.000000000000000000, 0.8660254037844387076, 1.000000000000000000, 0.8660254037844387076, 1.000000000000000000, 0.8660254037844387076, 1.000000000000000000, 0.8660254037844387076, 1.000000000000000000, 0.8660254037844387076, 1.000000000000000000, 0.8660254037844387076, 1.000000000000000000, 0.8660254037844387076, 1.000000000000000000, 0.8660254037844387076, 1.000000000000000000, 0.8660254037844387076, 1.000000000000000000, 0.8660254037844387076, 1.000000000000000000, 0.8660254037844387076, 1.000000000000000000, 0.8660254037844387076, 1.000000000000000000, 0.8660254037844387076, 1.000000000000000000, 0.8660254037844387076, 1.000000000000000000, 0.8660254037844387076, 1.000000000000000000, 0.8660254037844387076, 1.000000000000000000, 0.8660254037844387076, 1.000000000000000000, 0.8660254037844387076, 1.000000000000000000, 0.8660254037844387076, 1.000000000000000000, 0.8660254037844387076, 1.000000000000000000, 0.8660254037844387076, 1.000000000000000000, 0.8660254037844387076, 1.000000000000000000, 0.8660254037844387076, 1.000000000000000000, 0.8660254037844387076, 1.000000000000000000, 0.8660254037844387076, 1.000000000000000000, 0.8660254037844387076, 1.000000000000000000, 0.8660254037844387076, 1.000000000000000000, 0.8660254037844387076, 1.000000000000000000, 0.8660254037844387076, 1.000000000000000000, 0.8660254037844387076, 1.000000000000000000, 0.8660254037844387076, 1.000000000000000000, 0.8660254037844387076, 1.000000000000000000, 0.8660254037844387076, 1.000000000000000000, 0.8660254037844387076, 1.000000000000000000, 0.8660254037844387076, 1.000000000000000000, 0.8660254037844387076, 1.000000000000000000, 0.8660254037844387076, 1.000000000000000000, 0.8660254037844387076, 1.000000000000000000, 0.8660254037844387076, 1.000000000000000000, 0.8660254037844387076, 1.000000000000000000, 0.8660254037844387076, 1.000000000000000000, 0.8660254037844387076, 1.000000000000000000, 0.8660254037844387076, 1.000000000000000000, 0.8660254037844387076, 1.000000000000000000, 0.8660254037844387076, 1.000000000000000000, 0.8660254037844387076, 1.000000000000000000, 0.8660254037844387076, 1.000000000000000000, 0.8660254037844387076, 1.000000000000000000, 0.8660254037844387076, 1.000000000000000000, 0.8660254037844387076, 1.000000000000000000, 0.8660254037844387076, 1.000000000000000000, 0.8660254037844387076, 1.000000000000000000, 0.8660254037844387076, 1.000000000000000000, 0.8660254037844387076, 1.000000000000000000, 0.8660254037844387076, 1.000000000000000000, 0.8660254037844387076, 1.000000000000000000, 0.8660254037844387076, 1.000000000000000000, 0.8660254037844387076, 1.000000000000000000, 0.8660254037844387076, 1.000000000000000000, 0.8660254037844387076, 1.000000000000000000, 0.8660254037844387076, 1.000000000000000000, 0.8660254037844387076, 1.000000000000000000, 0.8660254037844387076, 1.000000000000000000, 0.8660254037844387076, 1.000000000000000000, 0.8660254037844387076, 1.000000000000000000, 0.8660254037844387076, 1.000000000000000000, 0.8660254037844387076, 1.000000000000000000, 0.8660254037844387076, 1.000000000000000000, 0.8660254037844387076, 1.000000000000000000, 0.8660254037844387076, 1.000000000000000000, 0.8660254037844387076, 1.000000000000000000, 0.8660254037844387076, 1.000000000000000000, 0.8660254037844387076, 1.000000000000000000, 0.8660254037844387076, 1.000000000000000000, 0.8660254037844387076, 1.000000000000000000, 0.8660254037844387076, 1.000000000000000000, 0.8660254037844387076, 1.000000000000000000, 0.8660254037844387076, 1.000000000000000000, 0.8660254037844387076, 1.000000000000000000, 0.8660254037844387076, 1.000000000000000000, 0.8660254037844387076, 1.000000000000000000, 0.8660254037844387076, 1.000000000000000000, 0.8660254037844387076, 1.000000000000000000, 0.8660254037844387076, 1.000000000000000000, 0.8660254037844387076, 1.000000000000000000, 0.8660254037844387076, 1.000000000000000000, 0.8660254037844387076, 1.000000000000000000, 0.8660254037844387076, 1.000000000000000000, 0.8660254037844387076, 1.000000000000000000, 0.8660254037844387076, 1.000000000000000000, 0.8660254037844387076, 1.000000000000000000, 0.8660254037844387076, 1.000000000000000000, 0.8660254037844387076, 1.000000000000000000, 0.8660254037844387076, 1.000000000000000000, 0.8660254037844387076, 1.000000000000000000, 0.8660254037844387076, 1.000000000000000000, 0.8660254037844387076, 1.000000000000000000, 0.8660254037844387076, 1.000000000000000000, 0.8660254037844387076, 1.000000000000000000, 0.8660254037844387076, 1.000000000000000000, 0.8660254037844387076, 1.000000000000000000, 0.8660254037844387076, 1.000000000000000000, 0.8660254037844387076, 1.000000000000000000, 0.8660254037844387076, 1.000000000000000000, 0.8660254037844387076, 1.000000000000000000, 0.8660254037844387076, 1.000000000000000000, 0.8660254037844387076, 1.000000000000000000, 0.8660254037844387076, 1.000000000000000000, 0.8660254037844387076, 1.000000000000000000, 0.8660254037844387076, 1.000000000000000000, 0.8660254037844387076, 1.000000000000000000, 0.8660254037844387076, 1.000000000000000000, 0.8660254037844387076, 1.000000000000000000, 0.8660254037844387076, 1.000000000000000000, 0.8660254037844387076, 1.000000000000000000, 0.8660254037844387076, 1.000000000000000000, 0.8660254037844387076, 1.000000000000000000, 0.8660254037844387076, 1.000000000000000000, 0.8660254037844387076, 1.000000000000000000, 0.8660254037844387076, 1.000000000000000000, 0.8660254037844387076, 1.000000000000000000, 0.8660254037844387076, 1.000000000000000000, 0.8660254037844387076, 1.000000000000000000, 0.8660254037844387076, 1.000000000000000000, 0.8660254037844387076, 1.000000000000000000, 0.8660254037844387076, 1.000000000000000000, 0.8660254037844387076, 1.000000000000000000, 0.8660254037844387076, 1.000000000000000000, 0.8660254037844387076, 1.000000000000000000, 0.8660254037844387076, 1.000000000000000000, 0.8660254037844387076, 1.000000000000000000, 0.8660254037844387076, 1.000000000000000000, 0.8660254037844387076, 1.000000000000000000, 0.8660254037844387076, 1.000000000000000000, 0.8660254037844387076, 1.000000000000000000, 0.8660254037844387076, 1.000000000000000000, 0.8660254037844387076, 1.000000000000000000, 0.8660254037844387076, 1.000000000000000000, 0.8660254037844387076, 1.000000000000000000, 0.8660254037844387076, 1.000000000000000000, 0.8660254037844387076, 1.000000000000000000, 0.8660254037844387076, 1.000000000000000000, 0.8660254037844387076, 1.000000000000000000, 0.8660254037844387076, 1.000000000000000000, 0.8660254037844387076, 1.000000000000000000, 0.8660254037844387076, 1.000000000000000000, 0.8660254037844387076, 1.000000000000000000, 0.8660254037844387076, 1.000000000000000000, 0.8660254037844387076, 1.000000000000000000, 0.8660254037844387076, 1.000000000000000000, 0.8660254037844387076, 1.000000000000000000, 0.8660254037844387076, 1.000000000000000000, 0.8660254037844387076, 1.000000000000000000, 0.8660254037844387076, 1.000000000000000000, 0.8660254037844387076, 1.000000000000000000, 0.8660254037844387076, 1.000000000000000000, 0.8660254037844387076, 1.000000000000000000, 0.8660254037844387076, 1.000000000000000000, 0.8660254037844387076, 1.000000000000000000, 0.8660254037844387076, 1.000000000000000000, 0.8660254037844387076, 1.000000000000000000, 0.8660254037844387076, 1.000000000000000000, 0.8660254037844387076, 1.000000000000000000, 0.8660254037844387076, 1.000000000000000000, 0.8660254037844387076, 1.000000000000000000, 0.8660254037844387076, 1.000000000000000000, 0.8660254037844387076, 1.000000000000000000, 0.8660254037844387076, 1.000000000000000000, 0.8660254037844387076, 1.000000000000000000, 0.8660254037844387076, 1.000000000000000000, 0.8660254037844387076, 1.000000000000000000, 0.8660254037844387076, 1.000000000000000000, 0.8660254037844387076, 1.000000000000000000, 0.8660254037844387076, 1.000000000000000000, 0.8660254037844387076, 1.000000000000000000, 0.8660254037844387076, 1.000000000000000000, 0.8660254037844387076, 1.000000000000000000, 0.8660254037844387076, 1.000000000000000000, 0.8660254037844387076, 1.000000000000000000, 0.8660254037844387076, 1.000000000000000000, 0.8660254037844387076, 1.000000000000000000, 0.8660254037844387076, 1.000000000000000000, 0.8660254037844387076, 1.000000000000000000, 0.8660254037844387076, 1.000000000000000000, 0.8660254037844387076, 1.000000000000000000, 0.8660254037844387076, 1.000000000000000000, 0.8660254037844387076, 1.000000000000000000, 0.8660254037844387076, 1.000000000000000000, 0.8660254037844387076, 1.000000000000000000, 0.8660254037844387076, 1.000000000000000000, 0.8660254037844387076, 1.000000000000000000, 0.8660254037844387076, 1.000000000000000000, 0.8660254037844387076, 1.000000000000000000, 0.8660254037844387076, 1.000000000000000000, 0.8660254037844387076, 1.000000000000000000, 0.8660254037844387076, 1.000000000000000000, 0.8660254037844387076, 1.000000000000000000, 0.8660254037844387076, 1.000000000000000000, 0.8660254037844387076, 1.000000000000000000, 0.8660254037844387076, 1.000000000000000000, 0.8660254037844387076, 1.000000000000000000, 0.8660254037844387076, 1.000000000000000000, 0.8660254037844387076, 1.000000000000000000, 0.8660254037844387076, 1.000000000000000000, 0.8660254037844387076, 1.000000000000000000, 0.8660254037844387076, 1.000000000000000000, 0.8660254037844387076, 1.000000000000000000, 0.8660254037844387076, 1.000000000000000000, 0.8660254037844387076, 1.000000000000000000, 0.8660254037844387076, 1.000000000000000000, 0.8660254037844387076, 1.000000000000000000, 0.8660254037844387076, 1.000000000000000000, 0.8660254037844387076, 1.000000000000000000, 0.8660254037844387076, 1.000000000000000000, 0.8660254037844387076, 1.000000000000000000, 0.8660254037844387076, 1.000000000000000000, 0.8660254037844387076, 1.000000000000000000, 0.8660254037844387076, 1.000000000000000000, 0.8660254037844387076, 1.000000000000000000, 0.8660254037844387076, 1.000000000000000000, 0.8660254037844387076, 1.000000000000000000, 0.8660254037844387076, 1.000000000000000000, 0.8660254037844387076, 1.000000000000000000, 0.8660254037844387076, 1.000000000000000000, 0.8660254037844387076, 1.000000000000000000, 0.8660254037844387076, 1.000000000000000000, 0.8660254037844387076, 1.000000000000000000, 0.8660254037844387076, 1.000000000000000000, 0.8660254037844387076, 1.000000000000000000, 0.8660254037844387076, 1.000000000000000000, 0.8660254037844387076, 1.000000000000000000, 0.8660254037844387076, 1.000000000000000000, 0.8660254037844387076, 1.000000000000000000, 0.8660254037844387076, 1.000000000000000000, 0.8660254037844387076, 1.000000000000000000, 0.8660254037844387076, 1.000000000000000000, 0.8660254037844387076, 1.000000000000000000, 0.8660254037844387076, 1.000000000000000000, 0.8660254037844387076, 1.000000000000000000, 0.8660254037844387076, 1.000000000000000000, 0.8660254037844387076, 1.000000000000000000, 0.8660254037844387076, 1.000000000000000000, 0.8660254037844387076, 1.000000000000000000, 0.8660254037844387076, 1.000000000000000000, 0.8660254037844387076, 1.000000000000000000, 0.8660254037844387076, 1.000000000000000000, 0.8660254037844387076, 1.000000000000000000, 0.8660254037844387076, 1.000000000000000000, 0.8660254037844387076, 1.000000000000000000, 0.8660254037844387076, 1.000000000000000000, 0.8660254037844387076, 1.000000000000000000, 0.8660254037844387076, 1.000000000000000000, 0.8660254037844387076, 1.000000000000000000, 0.8660254037844387076, 1.000000000000000000, 0.8660254037844387076, 1.000000000000000000, 0.8660254037844387076, 1.000000000000000000, 0.8660254037844387076, 1.000000000000000000, 0.8660254037844387076, 1.000000000000000000, 0.8660254037844387076, 1.000000000000000000, 0.8660254037844387076, 1.000000000000000000, 0.8660254037844387076, 1.000000000000000000, 0.8660254037844387076, 1.000000000000000000, 0.8660254037844387076, 1.000000000000000000, 0.8660254037844387076, 1.000000000000000000, 0.8660254037844387076, 1.000000000000000000, 0.8660254037844387076, 1.000000000000000000, 0.8660254037844387076, 1.000000000000000000, 0.8660254037844387076, 1.000000000000000000, 0.8660254037844387076, 1.000000000000000000, 0.8660254037844387076, 1.000000000000000000, 0.8660254037844387076, 1.000000000000000000, 0.8660254037844387076, 1.000000000000000000, 0.8660254037844387076, 1.000000000000000000, 0.8660254037844387076, 1.000000000000000000, 0.8660254037844387076, 1.000000000000000000, 0.8660254037844387076, 1.000000000000000000, 0.8660254037844387076, 1.000000000000000000, 0.8660254037844387076, 1.000000000000000000, 0.8660254037844387076, 1.000000000000000000, 0.8660254037844387076, 1.000000000000000000, 0.8660254037844387076, 1.000000000000000000, 0.8660254037844387076, 1.000000000000000000, 0.8660254037844387076, 1.000000000000000000, 0.8660254037844387076, 1.000000000000000000, 0.8660254037844387076, 1.000000000000000000, 0.8660254037844387076, 1.000000000000000000, 0.8660254037844387076, 1.000000000000000000, 0.8660254037844387076, 1.000000000000000000, 0.8660254037844387076, 1.000000000000000000, 0.8660254037844387076, 1.000000000000000000, 0.8660254037844387076, 1.000000000000000000, 0.8660254037844387076, 1.000000000000000000, 0.8660254037844387076, 1.000000000000000000, 0.8660254037844387076, 1.000000000000000000, 0.8660254037844387076, 1.000000000000000000, 0.8660254037844387076, 1.000000000000000000, 0.8660254037844387076, 1.000000000000000000, 0.8660254037844387076, 1.000000000000000000, 0.8660254037844387076, 1.000000000000000000, 0.8660254037844387076, 1.000000000000000000, 0.8660254037844387076, 1.000000000000000000, 0.8660254037844387076, 1.000000000000000000, 0.8660254037844387076, 1.000000000000000000, 0.8660254037844387076, 1.000000000000000000, 0.8660254037844387076, 1.000000000000000000, 0.8660254037844387076, 1.000000000000000000, 0.8660254037844387076, 1.000000000000000000, 0.8660254037844387076, 1.000000000000000000, 0.8660254037844387076, 1.000000000000000000, 0.8660254037844387076, 1.000000000000000000, 0.8660254037844387076, 1.000000000000000000, 0.8660254037844387076, 1.000000000000000000, 0.8660254037844387076, 1.000000000000000000, 0.8660254037844387076, 1.000000000000000000, 0.8660254037844387076, 1.000000000000000000, 0.8660254037844387076, 1.000000000000000000, 0.8660254037844387076, 1.000000000000000000, 0.8660254037844387076, 1.000000000000000000, 0.8660254037844387076, 1.000000000000000000, 0.8660254037844387076, 1.000000000000000000, 0.8660254037844387076, 1.000000000000000000, 0.8660254037844387076, 1.000000000000000000, 0.8660254037844387076, 1.000000000000000000, 0.8660254037844387076, 1.000000000000000000, 0.8660254037844387076, 1.000000000000000000, 0.8660254037844387076, 1.000000000000000000, 0.8660254037844387076, 1.000000000000000000, 0.8660254037844387076, 1.000000000000000000, 0.8660254037844387076, 1.000000000000000000, 0.8660254037844387076, 1.000000000000000000, 0.8660254037844387076, 1.000000000000000000, 0.8660254037844387076, 1.000000000000000000, 0.8660254037844387076, 1.000000000000000000, 0.8660254037844387076, 1.000000000000000000, 0.8660254037844387076, 1.000000000000000000, 0.8660254037844387076, 1.000000000000000000, 0.8660254037844387076, 1.000000000000000000, 0.8660254037844387076, 1.000000000000000000, 0.8660254037844387076, 1.000000000000000000, 0.8660254037844387076, 1.000000000000000000, 0.8660254037844387076, 1.000000000000000000, 0.8660254037844387076, 1.000000000000000000, 0.8660254037844387076, 1.000000000000000000, 0.8660254037844387076, 1.000000000000000000, 0.8660254037844387076, 1.000000000000000000, 0.8660254037844387076, 1.000000000000000000, 0.8660254037844387076, 1.000000000000000000, 0.8660254037844387076, 1.000000000000000000, 0.8660254037844387076, 1.000000000000000000, 0.8660254037844387076, 1.000000000000000000, 0.8660254037844387076, 1.000000000000000000, 0.8660254037844387076, 1.000000000000000000, 0.8660254037844387076, 1.000000000000000000, 0.8660254037844387076, 1.000000000000000000, 0.8660254037844387076, 1.000000000000000000, 0.8660254037844387076, 1.000000000000000000, 0.8660254037844387076, 1.000000000000000000, 0.8660254037844387076, 1.000000000000000000, 0.8660254037844387076, 1.000000000000000000, 0.8660254037844387076, 1.000000000000000000, 0.8660254037844387076, 1.000000000000000000, 0.8660254037844387076, 1.000000000000000000, 0.8660254037844387076, 1.000000000000000000, 0.8660254037844387076, 1.000000000000000000, 0.8660254037844387076, 1.000000000000000000, 0.8660254037844387076, 1.000000000000000000, 0.8660254037844387076, 1.000000000000000000, 0.8660254037844387076, 1.000000000000000000, 0.8660254037844387076, 1.000000000000000000, 0.8660254037844387076, 1.000000000000000000, 0.8660254037844387076, 1.000000000000000000, 0.8660254037844387076, 1.000000000000000000, 0.8660254037844387076, 1.000000000000000000, 0.8660254037844387076, 1.000000000000000000, 0.8660254037844387076, 1.000000000000000000, 0.8660254037844387076, 1.000000000000000000, 0.8660254037844387076, 1.000000000000000000, 0.8660254037844387076, 1.000000000000000000, 0.8660254037844387076, 1.000000000000000000, 0.8660254037844387076, 1.000000000000000000, 0.8660254037844387076, 1.000000000000000000, 0.8660254037844387076, 1.000000000000000000, 0.8660254037844387076, 1.000000000000000000, 0.8660254037844387076, 1.000000000000000000, 0.8660254037844387076, 1.000000000000000000, 0.8660254037844387076, 1.000000000000000000, 0.8660254037844387076, 1.000000000000000000, 0.8660254037844387076, 1.000000000000000000, 0.8660254037844387076, 1.000000000000000000, 0.8660254037844387076, 1.000000000000000000, 0.8660254037844387076, 1.000000000000000000, 0.8660254037844387076, 1.000000000000000000, 0.8660254037844387076, 1.000000000000000000, 0.8660254037844387076, 1.000000000000000000, 0.8660254037844387076, 1.000000000000000000, 0.8660254037844387076, 1.000000000000000000, 0.8660254037844387076, 1.000000000000000000, 0.8660254037844387076, 1.000000000000000000, 0.8660254037844387076, 1.000000000000000000, 0.8660254037844387076, 1.000000000000000000, 0.8660254037844387076, 1.000000000000000000, 0.8660254037844387076, 1.000000000000000000, 0.8660254037844387076, 1.000000000000000000, 0.8660254037844387076, 1.000000000000000000, 0.8660254037844387076, 1.000000000000000000, 0.8660254037844387076, 1.000000000000000000, 0.8660254037844387076, 1.000000000000000000, 0.8660254037844387076, 1.000000000000000000, 0.8660254037844387076, 1.000000000000000000, 0.8660254037844387076, 1.000000000000000000, 0.8660254037844387076, 1.000000000000000000, 0.8660254037844387076, 1.000000000000000000, 0.8660254037844387076, 1.000000000000000000, 0.8660254037844387076, 1.000000000000000000, 0.8660254037844387076, 1.000000000000000000, 0.8660254037844387076, 1.000000000000000000, 0.8660254037844387076, 1.000000000000000000, 0.8660254037844387076, 1.000000000000000000, 0.8660254037844387076, 1.000000000000000000, 0.8660254037844387076, 1.000000000000000000, 0.8660254037844387076, 1.000000000000000000, 0.8660254037844387076, 1.000000000000000000, 0.8660254037844387076, 1.000000000000000000, 0.8660254037844387076, 1.000000000000000000, 0.8660254037844387076, 1.000000000000000000),
 ( 1.000000000000000000, 0.8660254037844387076, 1.000000000000000000, 0.8660254037844387076, 1.000000000000000000, 0.8660254037844387076, 1.000000000000000000, 0.8660254037844387076, 1.000000000000000000, 0.8660254037844387076, 1.000000000000000000, 0.8660254037844387076, 1.000000000000000000, 0.8660254037844387076, 1.000000000000000000, 0.8660254037844387076, 1.000000000000000000, 0.8660254037844387076, 1.000000000000000000, 0.8660254037844387076, 1.000000000000000000, 0.8660254037844387076, 1.000000000000000000, 0.8660254037844387076, 1.000000000000000000, 0.8660254037844387076, 1.000000000000000000, 0.8660254037844387076, 1.000000000000000000, 0.8660254037844387076, 1.000000000000000000, 0.8660254037844387076, 1.000000000000000000, 0.8660254037844387076, 1.000000000000000000, 0.8660254037844387076, 1.000000000000000000, 0.8660254037844387076, 1.000000000000000000, 0.8660254037844387076, 1.000000000000000000, 0.8660254037844387076, 1.000000000000000000, 0.8660254037844387076, 1.000000000000000000, 0.8660254037844387076, 1.000000000000000000, 0.8660254037844387076, 1.000000000000000000, 0.8660254037844387076, 1.000000000000000000, 0.8660254037844387076, 1.000000000000000000, 0.8660254037844387076, 1.000000000000000000, 0.8660254037844387076, 1.000000000000000000, 0.8660254037844387076, 1.000000000000000000, 0.8660254037844387076, 1.000000000000000000, 0.8660254037844387076, 1.000000000000000000, 0.8660254037844387076, 1.000000000000000000, 0.8660254037844387076, 1.000000000000000000, 0.8660254037844387076, 1.000000000000000000, 0.8660254037844387076, 1.000000000000000000, 0.8660254037844387076, 1.000000000000000000, 0.8660254037844387076, 1.000000000000000000, 0.8660254037844387076, 1.000000000000000000, 0.8660254037844387076, 1.000000000000000000, 0.8660254037844387076, 1.000000000000000000, 0.8660254037844387076, 1.000000000000000000, 0.8660254037844387076, 1.000000000000000000, 0.8660254037844387076, 1.000000000000000000, 0.8660254037844387076, 1.000000000000000000, 0.8660254037844387076, 1.000000000000000000, 0.8660254037844387076, 1.000000000000000000, 0.8660254037844387076, 1.000000000000000000, 0.8660254037844387076, 1.000000000000000000, 0.8660254037844387076, 1.000000000000000000, 0.8660254037844387076, 1.000000000000000000, 0.8660254037844387076, 1.000000000000000000, 0.8660254037844387076, 1.000000000000000000, 0.8660254037844387076, 1.000000000000000000, 0.8660254037844387076, 1.000000000000000000, 0.8660254037844387076, 1.000000000000000000, 0.8660254037844387076, 1.000000000000000000, 0.8660254037844387076, 1.000000000000000000, 0.8660254037844387076, 1.000000000000000000, 0.8660254037844387076, 1.000000000000000000, 0.8660254037844387076, 1.000000000000000000, 0.8660254037844387076, 1.000000000000000000, 0.8660254037844387076, 1.000000000000000000, 0.8660254037844387076, 1.000000000000000000, 0.8660254037844387076, 1.000000000000000000, 0.8660254037844387076, 1.000000000000000000, 0.8660254037844387076, 1.000000000000000000, 0.8660254037844387076, 1.000000000000000000, 0.8660254037844387076, 1.000000000000000000, 0.8660254037844387076, 1.000000000000000000, 0.8660254037844387076, 1.000000000000000000, 0.8660254037844387076, 1.000000000000000000, 0.8660254037844387076, 1.000000000000000000, 0.8660254037844387076, 1.000000000000000000, 0.8660254037844387076, 1.000000000000000000, 0.8660254037844387076, 1.000000000000000000, 0.8660254037844387076, 1.000000000000000000, 0.8660254037844387076, 1.000000000000000000, 0.8660254037844387076, 1.000000000000000000, 0.8660254037844387076, 1.000000000000000000, 0.8660254037844387076, 1.000000000000000000, 0.8660254037844387076, 1.000000000000000000, 0.8660254037844387076, 1.000000000000000000, 0.8660254037844387076, 1.000000000000000000, 0.8660254037844387076, 1.000000000000000000, 0.8660254037844387076, 1.000000000000000000, 0.8660254037844387076, 1.000000000000000000, 0.8660254037844387076, 1.000000000000000000, 0.8660254037844387076, 1.000000000000000000, 0.8660254037844387076, 1.000000000000000000, 0.8660254037844387076, 1.000000000000000000, 0.8660254037844387076, 1.000000000000000000, 0.8660254037844387076, 1.000000000000000000, 0.8660254037844387076, 1.000000000000000000, 0.8660254037844387076, 1.000000000000000000, 0.8660254037844387076, 1.000000000000000000, 0.8660254037844387076, 1.000000000000000000, 0.8660254037844387076, 1.000000000000000000, 0.8660254037844387076, 1.000000000000000000, 0.8660254037844387076, 1.000000000000000000, 0.8660254037844387076, 1.000000000000000000, 0.8660254037844387076, 1.000000000000000000, 0.8660254037844387076, 1.000000000000000000, 0.8660254037844387076, 1.000000000000000000, 0.8660254037844387076, 1.000000000000000000, 0.8660254037844387076, 1.000000000000000000, 0.8660254037844387076, 1.000000000000000000, 0.8660254037844387076, 1.000000000000000000, 0.8660254037844387076, 1.000000000000000000, 0.8660254037844387076, 1.000000000000000000, 0.8660254037844387076, 1.000000000000000000, 0.8660254037844387076, 1.000000000000000000, 0.8660254037844387076, 1.000000000000000000, 0.8660254037844387076, 1.000000000000000000, 0.8660254037844387076, 1.000000000000000000, 0.8660254037844387076, 1.000000000000000000, 0.8660254037844387076, 1.000000000000000000, 0.8660254037844387076, 1.000000000000000000, 0.8660254037844387076, 1.000000000000000000, 0.8660254037844387076, 1.000000000000000000, 0.8660254037844387076, 1.000000000000000000, 0.8660254037844387076, 1.000000000000000000, 0.8660254037844387076, 1.000000000000000000, 0.8660254037844387076, 1.000000000000000000, 0.8660254037844387076, 1.000000000000000000, 0.8660254037844387076, 1.000000000000000000, 0.8660254037844387076, 1.000000000000000000, 0.8660254037844387076, 1.000000000000000000, 0.8660254037844387076, 1.000000000000000000, 0.8660254037844387076, 1.000000000000000000, 0.8660254037844387076, 1.000000000000000000, 0.8660254037844387076, 1.000000000000000000, 0.8660254037844387076, 1.000000000000000000, 0.8660254037844387076, 1.000000000000000000, 0.8660254037844387076, 1.000000000000000000, 0.8660254037844387076, 1.000000000000000000, 0.8660254037844387076, 1.000000000000000000, 0.8660254037844387076, 1.000000000000000000, 0.8660254037844387076, 1.000000000000000000, 0.8660254037844387076, 1.000000000000000000, 0.8660254037844387076, 1.000000000000000000, 0.8660254037844387076, 1.000000000000000000, 0.8660254037844387076, 1.000000000000000000, 0.8660254037844387076, 1.000000000000000000, 0.8660254037844387076, 1.000000000000000000, 0.8660254037844387076, 1.000000000000000000, 0.8660254037844387076, 1.000000000000000000, 0.8660254037844387076, 1.000000000000000000, 0.8660254037844387076, 1.000000000000000000, 0.8660254037844387076, 1.000000000000000000, 0.8660254037844387076, 1.000000000000000000, 0.8660254037844387076, 1.000000000000000000, 0.8660254037844387076, 1.000000000000000000, 0.8660254037844387076, 1.000000000000000000, 0.8660254037844387076, 1.000000000000000000, 0.8660254037844387076, 1.000000000000000000, 0.8660254037844387076, 1.000000000000000000, 0.8660254037844387076, 1.000000000000000000, 0.8660254037844387076, 1.000000000000000000, 0.8660254037844387076, 1.000000000000000000, 0.8660254037844387076, 1.000000000000000000, 0.8660254037844387076, 1.000000000000000000, 0.8660254037844387076, 1.000000000000000000, 0.8660254037844387076, 1.000000000000000000, 0.8660254037844387076, 1.000000000000000000, 0.8660254037844387076, 1.000000000000000000, 0.8660254037844387076, 1.000000000000000000, 0.8660254037844387076, 1.000000000000000000, 0.8660254037844387076, 1.000000000000000000, 0.8660254037844387076, 1.000000000000000000, 0.8660254037844387076, 1.000000000000000000, 0.8660254037844387076, 1.000000000000000000, 0.8660254037844387076, 1.000000000000000000, 0.8660254037844387076, 1.000000000000000000, 0.8660254037844387076, 1.000000000000000000, 0.8660254037844387076, 1.000000000000000000, 0.8660254037844387076, 1.000000000000000000, 0.8660254037844387076, 1.000000000000000000, 0.8660254037844387076, 1.000000000000000000, 0.8660254037844387076, 1.000000000000000000, 0.8660254037844387076, 1.000000000000000000, 0.8660254037844387076, 1.000000000000000000, 0.8660254037844387076, 1.000000000000000000, 0.8660254037844387076, 1.000000000000000000, 0.8660254037844387076, 1.000000000000000000, 0.8660254037844387076, 1.000000000000000000, 0.8660254037844387076, 1.000000000000000000, 0.8660254037844387076, 1.000000000000000000, 0.8660254037844387076, 1.000000000000000000, 0.8660254037844387076, 1.000000000000000000, 0.8660254037844387076, 1.000000000000000000, 0.8660254037844387076, 1.000000000000000000, 0.8660254037844387076, 1.000000000000000000, 0.8660254037844387076, 1.000000000000000000, 0.8660254037844387076, 1.000000000000000000, 0.8660254037844387076, 1.000000000000000000, 0.8660254037844387076, 1.000000000000000000, 0.8660254037844387076, 1.000000000000000000, 0.8660254037844387076, 1.000000000000000000, 0.8660254037844387076, 1.000000000000000000, 0.8660254037844387076, 1.000000000000000000, 0.8660254037844387076, 1.000000000000000000, 0.8660254037844387076, 1.000000000000000000, 0.8660254037844387076, 1.000000000000000000, 0.8660254037844387076, 1.000000000000000000, 0.8660254037844387076, 1.000000000000000000, 0.8660254037844387076, 1.000000000000000000, 0.8660254037844387076, 1.000000000000000000, 0.8660254037844387076, 1.000000000000000000, 0.8660254037844387076, 1.000000000000000000, 0.8660254037844387076, 1.000000000000000000, 0.8660254037844387076, 1.000000000000000000, 0.8660254037844387076, 1.000000000000000000, 0.8660254037844387076, 1.000000000000000000, 0.8660254037844387076, 1.000000000000000000, 0.8660254037844387076, 1.000000000000000000, 0.8660254037844387076, 1.000000000000000000, 0.8660254037844387076, 1.000000000000000000, 0.8660254037844387076, 1.000000000000000000, 0.8660254037844387076, 1.000000000000000000, 0.8660254037844387076, 1.000000000000000000, 0.8660254037844387076, 1.000000000000000000, 0.8660254037844387076, 1.000000000000000000, 0.8660254037844387076, 1.000000000000000000, 0.8660254037844387076, 1.000000000000000000, 0.8660254037844387076, 1.000000000000000000, 0.8660254037844387076, 1.000000000000000000, 0.8660254037844387076, 1.000000000000000000, 0.8660254037844387076, 1.000000000000000000, 0.8660254037844387076, 1.000000000000000000, 0.8660254037844387076, 1.000000000000000000, 0.8660254037844387076, 1.000000000000000000, 0.8660254037844387076, 1.000000000000000000, 0.8660254037844387076, 1.000000000000000000, 0.8660254037844387076, 1.000000000000000000, 0.8660254037844387076, 1.000000000000000000, 0.8660254037844387076, 1.000000000000000000, 0.8660254037844387076, 1.000000000000000000, 0.8660254037844387076, 1.000000000000000000, 0.8660254037844387076, 1.000000000000000000, 0.8660254037844387076, 1.000000000000000000, 0.8660254037844387076, 1.000000000000000000, 0.8660254037844387076, 1.000000000000000000, 0.8660254037844387076, 1.000000000000000000, 0.8660254037844387076, 1.000000000000000000, 0.8660254037844387076, 1.000000000000000000, 0.8660254037844387076, 1.000000000000000000, 0.8660254037844387076, 1.000000000000000000, 0.8660254037844387076, 1.000000000000000000, 0.8660254037844387076, 1.000000000000000000, 0.8660254037844387076, 1.000000000000000000, 0.8660254037844387076, 1.000000000000000000, 0.8660254037844387076, 1.000000000000000000, 0.8660254037844387076, 1.000000000000000000, 0.8660254037844387076, 1.000000000000000000, 0.8660254037844387076, 1.000000000000000000, 0.8660254037844387076, 1.000000000000000000, 0.8660254037844387076, 1.000000000000000000, 0.8660254037844387076, 1.000000000000000000, 0.8660254037844387076, 1.000000000000000000, 0.8660254037844387076, 1.000000000000000000, 0.8660254037844387076, 1.000000000000000000, 0.8660254037844387076, 1.000000000000000000, 0.8660254037844387076, 1.000000000000000000, 0.8660254037844387076, 1.000000000000000000, 0.8660254037844387076, 1.000000000000000000, 0.8660254037844387076, 1.000000000000000000, 0.8660254037844387076, 1.000000000000000000, 0.8660254037844387076, 1.000000000000000000, 0.8660254037844387076, 1.000000000000000000, 0.8660254037844387076, 1.000000000000000000, 0.8660254037844387076, 1.000000000000000000, 0.8660254037844387076, 1.000000000000000000, 0.8660254037844387076, 1.000000000000000000, 0.8660254037844387076, 1.000000000000000000, 0.8660254037844387076, 1.000000000000000000, 0.8660254037844387076, 1.000000000000000000, 0.8660254037844387076, 1.000000000000000000, 0.8660254037844387076, 1.000000000000000000, 0.8660254037844387076, 1.000000000000000000, 0.8660254037844387076, 1.000000000000000000, 0.8660254037844387076, 1.000000000000000000, 0.8660254037844387076, 1.000000000000000000, 0.8660254037844387076, 1.000000000000000000, 0.8660254037844387076, 1.000000000000000000, 0.8660254037844387076, 1.000000000000000000, 0.8660254037844387076, 1.000000000000000000, 0.8660254037844387076, 1.000000000000000000, 0.8660254037844387076, 1.000000000000000000, 0.8660254037844387076, 1.000000000000000000, 0.8660254037844387076, 1.000000000000000000, 0.8660254037844387076, 1.000000000000000000, 0.8660254037844387076, 1.000000000000000000, 0.8660254037844387076, 1.000000000000000000, 0.8660254037844387076, 1.000000000000000000, 0.8660254037844387076, 1.000000000000000000, 0.8660254037844387076, 1.000000000000000000, 0.8660254037844387076, 1.000000000000000000, 0.8660254037844387076, 1.000000000000000000, 0.8660254037844387076, 1.000000000000000000, 0.8660254037844387076, 1.000000000000000000, 0.8660254037844387076, 1.000000000000000000, 0.8660254037844387076, 1.000000000000000000, 0.8660254037844387076, 1.000000000000000000, 0.8660254037844387076, 1.000000000000000000, 0.8660254037844387076, 1.000000000000000000, 0.8660254037844387076, 1.000000000000000000, 0.8660254037844387076, 1.000000000000000000, 0.8660254037844387076, 1.000000000000000000, 0.8660254037844387076, 1.000000000000000000, 0.8660254037844387076, 1.000000000000000000, 0.8660254037844387076, 1.000000000000000000, 0.8660254037844387076, 1.000000000000000000, 0.8660254037844387076, 1.000000000000000000, 0.8660254037844387076, 1.000000000000000000, 0.8660254037844387076, 1.000000000000000000, 0.8660254037844387076, 1.000000000000000000, 0.8660254037844387076, 1.000000000000000000, 0.8660254037844387076, 1.000000000000000000, 0.8660254037844387076, 1.000000000000000000, 0.8660254037844387076, 1.000000000000000000, 0.8660254037844387076, 1.000000000000000000, 0.8660254037844387076, 1.000000000000000000, 0.8660254037844387076, 1.000000000000000000, 0.8660254037844387076, 1.000000000000000000, 0.8660254037844387076, 1.000000000000000000, 0.8660254037844387076, 1.000000000000000000, 0.8660254037844387076, 1.000000000000000000, 0.8660254037844387076, 1.000000000000000000, 0.8660254037844387076, 1.000000000000000000, 0.8660254037844387076, 1.000000000000000000, 0.8660254037844387076, 1.000000000000000000, 0.8660254037844387076, 1.000000000000000000, 0.8660254037844387076, 1.000000000000000000, 0.8660254037844387076, 1.000000000000000000, 0.8660254037844387076, 1.000000000000000000, 0.8660254037844387076, 1.000000000000000000, 0.8660254037844387076, 1.000000000000000000, 0.8660254037844387076, 1.000000000000000000, 0.8660254037844387076, 1.000000000000000000, 0.8660254037844387076, 1.000000000000000000, 0.8660254037844387076, 1.000000000000000000, 0.8660254037844387076, 1.000000000000000000, 0.8660254037844387076, 1.000000000000000000, 0.8660254037844387076, 1.000000000000000000, 0.8660254037844387076, 1.000000000000000000, 0.8660254037844387076, 1.000000000000000000, 0.8660254037844387076, 1.000000000000000000, 0.8660254037844387076, 1.000000000000000000, 0.8660254037844387076, 1.000000000000000000, 0.8660254037844387076, 1.000000000000000000, 0.8660254037844387076, 1.000000000000000000, 0.8660254037844387076, 1.000000000000000000, 0.8660254037844387076, 1.000000000000000000, 0.8660254037844387076, 1.000000000000000000, 0.8660254037844387076, 1.000000000000000000, 0.8660254037844387076, 1.000000000000000000, 0.8660254037844387076, 1.000000000000000000, 0.8660254037844387076, 1.000000000000000000, 0.8660254037844387076, 1.000000000000000000, 0.8660254037844387076, 1.000000000000000000, 0.8660254037844387076, 1.000000000000000000, 0.8660254037844387076, 1.000000000000000000, 0.8660254037844387076, 1.000000000000000000, 0.8660254037844387076, 1.000000000000000000, 0.8660254037844387076, 1.000000000000000000, 0.8660254037844387076, 1.000000000000000000, 0.8660254037844387076, 1.000000000000000000, 0.8660254037844387076, 1.000000000000000000, 0.8660254037844387076, 1.000000000000000000, 0.8660254037844387076, 1.000000000000000000, 0.8660254037844387076, 1.000000000000000000, 0.8660254037844387076, 1.000000000000000000, 0.8660254037844387076, 1.000000000000000000, 0.8660254037844387076, 1.000000000000000000, 0.8660254037844387076, 1.000000000000000000, 0.8660254037844387076, 1.000000000000000000, 0.8660254037844387076, 1.000000000000000000, 0.8660254037844387076, 1.000000000000000000, 0.8660254037844387076, 1.000000000000000000, 0.8660254037844387076, 1.000000000000000000, 0.8660254037844387076, 1.000000000000000000, 0.8660254037844387076, 1.000000000000000000, 0.8660254037844387076, 1.000000000000000000, 0.8660254037844387076, 1.000000000000000000, 0.8660254037844387076, 1.000000000000000000, 0.8660254037844387076, 1.000000000000000000, 0.8660254037844387076, 1.000000000000000000, 0.8660254037844387076, 1.000000000000000000, 0.8660254037844387076, 1.000000000000000000, 0.8660254037844387076, 1.000000000000000000, 0.8660254037844387076, 1.000000000000000000, 0.8660254037844387076, 1.000000000000000000, 0.8660254037844387076, 1.000000000000000000, 0.8660254037844387076, 1.000000000000000000, 0.8660254037844387076, 1.000000000000000000, 0.8660254037844387076, 1.000000000000000000, 0.8660254037844387076, 1.000000000000000000, 0.8660254037844387076, 1.000000000000000000, 0.8660254037844387076, 1.000000000000000000, 0.8660254037844387076, 1.000000000000000000, 0.8660254037844387076, 1.000000000000000000, 0.8660254037844387076, 1.000000000000000000, 0.8660254037844387076, 1.000000000000000000, 0.8660254037844387076, 1.000000000000000000, 0.8660254037844387076, 1.000000000000000000, 0.8660254037844387076, 1.000000000000000000, 0.8660254037844387076, 1.000000000000000000, 0.8660254037844387076, 1.000000000000000000, 0.8660254037844387076, 1.000000000000000000, 0.8660254037844387076, 1.000000000000000000, 0.8660254037844387076, 1.000000000000000000, 0.8660254037844387076, 1.000000000000000000, 0.8660254037844387076, 1.000000000000000000, 0.8660254037844387076, 1.000000000000000000, 0.8660254037844387076, 1.000000000000000000, 0.8660254037844387076, 1.000000000000000000, 0.8660254037844387076, 1.000000000000000000, 0.8660254037844387076, 1.000000000000000000, 0.8660254037844387076, 1.000000000000000000, 0.8660254037844387076, 1.000000000000000000, 0.8660254037844387076, 1.000000000000000000, 0.8660254037844387076, 1.000000000000000000, 0.8660254037844387076, 1.000000000000000000, 0.8660254037844387076, 1.000000000000000000, 0.8660254037844387076, 1.000000000000000000, 0.8660254037844387076, 1.000000000000000000, 0.8660254037844387076, 1.000000000000000000, 0.8660254037844387076, 1.000000000000000000, 0.8660254037844387076, 1.000000000000000000, 0.8660254037844387076, 1.000000000000000000, 0.8660254037844387076, 1.000000000000000000, 0.8660254037844387076, 1.000000000000000000, 0.8660254037844387076, 1.000000000000000000, 0.8660254037844387076, 1.000000000000000000, 0.8660254037844387076, 1.000000000000000000, 0.8660254037844387076, 1.000000000000000000, 0.8660254037844387076, 1.000000000000000000, 0.8660254037844387076, 1.000000000000000000, 0.8660254037844387076, 1.000000000000000000, 0.8660254037844387076, 1.000000000000000000, 0.8660254037844387076, 1.000000000000000000, 0.8660254037844387076, 1.000000000000000000, 0.8660254037844387076, 1.000000000000000000, 0.8660254037844387076, 1.000000000000000000, 0.8660254037844387076, 1.000000000000000000, 0.8660254037844387076, 1.000000000000000000, 0.8660254037844387076, 1.000000000000000000, 0.8660254037844387076, 1.000000000000000000, 0.8660254037844387076, 1.000000000000000000, 0.8660254037844387076, 1.000000000000000000, 0.8660254037844387076, 1.000000000000000000, 0.8660254037844387076, 1.000000000000000000, 0.8660254037844387076, 1.000000000000000000, 0.8660254037844387076, 1.000000000000000000, 0.8660254037844387076, 1.000000000000000000, 0.8660254037844387076, 1.000000000000000000, 0.8660254037844387076, 1.000000000000000000, 0.8660254037844387076, 1.000000000000000000, 0.8660254037844387076, 1.000000000000000000, 0.8660254037844387076, 1.000000000000000000, 0.8660254037844387076, 1.000000000000000000, 0.8660254037844387076, 1.000000000000000000, 0.8660254037844387076, 1.000000000000000000, 0.8660254037844387076, 1.000000000000000000, 0.8660254037844387076, 1.000000000000000000, 0.8660254037844387076, 1.000000000000000000, 0.8660254037844387076, 1.000000000000000000, 0.8660254037844387076, 1.000000000000000000, 0.8660254037844387076, 1.000000000000000000, 0.8660254037844387076, 1.000000000000000000, 0.8660254037844387076, 1.000000000000000000, 0.8660254037844387076, 1.000000000000000000, 0.8660254037844387076, 1.000000000000000000, 0.8660254037844387076, 1.000000000000000000, 0.8660254037844387076, 1.000000000000000000, 0.8660254037844387076, 1.000000000000000000, 0.8660254037844387076, 1.000000000000000000, 0.8660254037844387076, 1.000000000000000000, 0.8660254037844387076, 1.000000000000000000, 0.8660254037844387076, 1.000000000000000000, 0.8660254037844387076, 1.000000000000000000, 0.8660254037844387076, 1.000000000000000000, 0.8660254037844387076, 1.000000000000000000, 0.8660254037844387076, 1.000000000000000000, 0.8660254037844387076, 1.000000000000000000, 0.8660254037844387076, 1.000000000000000000, 0.8660254037844387076, 1.000000000000000000, 0.8660254037844387076, 1.000000000000000000, 0.8660254037844387076, 1.000000000000000000, 0.8660254037844387076, 1.000000000000000000, 0.8660254037844387076, 1.000000000000000000, 0.8660254037844387076, 1.000000000000000000, 0.8660254037844387076, 1.000000000000000000, 0.8660254037844387076, 1.000000000000000000, 0.8660254037844387076, 1.000000000000000000, 0.8660254037844387076, 1.000000000000000000, 0.8660254037844387076, 1.000000000000000000, 0.8660254037844387076, 1.000000000000000000, 0.8660254037844387076, 1.000000000000000000, 0.8660254037844387076, 1.000000000000000000, 0.8660254037844387076, 1.000000000000000000, 0.8660254037844387076, 1.000000000000000000, 0.8660254037844387076, 1.000000000000000000, 0.8660254037844387076, 1.000000000000000000, 0.8660254037844387076, 1.000000000000000000, 0.8660254037844387076, 1.000000000000000000, 0.8660254037844387076, 1.000000000000000000, 0.8660254037844387076, 1.000000000000000000, 0.8660254037844387076, 1.000000000000000000, 0.8660254037844387076, 1.000000000000000000, 0.8660254037844387076, 1.000000000000000000, 0.8660254037844387076, 1.000000000000000000, 0.8660254037844387076, 1.000000000000000000, 0.8660254037844387076, 1.000000000000000000, 0.8660254037844387076, 1.000000000000000000, 0.8660254037844387076, 1.000000000000000000, 0.8660254037844387076, 1.000000000000000000, 0.8660254037844387076, 1.000000000000000000, 0.8660254037844387076, 1.000000000000000000, 0.8660254037844387076, 1.000000000000000000, 0.8660254037844387076, 1.000000000000000000, 0.8660254037844387076, 1.000000000000000000, 0.8660254037844387076, 1.000000000000000000, 0.8660254037844387076, 1.000000000000000000, 0.8660254037844387076, 1.000000000000000000, 0.8660254037844387076, 1.000000000000000000, 0.8660254037844387076, 1.000000000000000000, 0.8660254037844387076, 1.000000000000000000, 0.8660254037844387076, 1.000000000000000000, 0.8660254037844387076, 1.000000000000000000, 0.8660254037844387076, 1.000000000000000000, 0.8660254037844387076, 1.000000000000000000, 0.8660254037844387076, 1.000000000000000000, 0.8660254037844387076, 1.000000000000000000, 0.8660254037844387076, 1.000000000000000000, 0.8660254037844387076, 1.000000000000000000, 0.8660254037844387076, 1.000000000000000000, 0.8660254037844387076, 1.000000000000000000, 0.8660254037844387076, 1.000000000000000000, 0.8660254037844387076, 1.000000000000000000, 0.8660254037844387076, 1.000000000000000000, 0.8660254037844387076, 1.000000000000000000, 0.8660254037844387076, 1.000000000000000000, 0.8660254037844387076, 1.000000000000000000, 0.8660254037844387076, 1.000000000000000000, 0.8660254037844387076, 1.000000000000000000, 0.8660254037844387076, 1.000000000000000000, 0.8660254037844387076, 1.000000000000000000, 0.8660254037844387076, 1.000000000000000000, 0.8660254037844387076, 1.000000000000000000, 0.8660254037844387076, 1.000000000000000000, 0.8660254037844387076, 1.000000000000000000, 0.8660254037844387076, 1.000000000000000000, 0.8660254037844387076, 1.000000000000000000, 0.8660254037844387076, 1.000000000000000000, 0.8660254037844387076, 1.000000000000000000, 0.8660254037844387076, 1.000000000000000000, 0.8660254037844387076, 1.000000000000000000, 0.8660254037844387076, 1.000000000000000000, 0.8660254037844387076, 1.000000000000000000, 0.8660254037844387076, 1.000000000000000000, 0.8660254037844387076, 1.000000000000000000, 0.8660254037844387076, 1.000000000000000000, 0.8660254037844387076, 1.000000000000000000, 0.8660254037844387076, 1.000000000000000000, 0.8660254037844387076, 1.000000000000000000, 0.8660254037844387076, 1.000000000000000000, 0.8660254037844387076, 1.000000000000000000, 0.8660254037844387076, 1.000000000000000000, 0.8660254037844387076, 1.000000000000000000, 0.8660254037844387076, 1.000000000000000000, 0.8660254037844387076, 1.000000000000000000, 0.8660254037844387076, 1.000000000000000000, 0.8660254037844387076, 1.000000000000000000, 0.8660254037844387076, 1.000000000000000000, 0.8660254037844387076, 1.000000000000000000, 0.8660254037844387076, 1.000000000000000000, 0.8660254037844387076, 1.000000000000000000, 0.8660254037844387076, 1.000000000000000000, 0.8660254037844387076, 1.000000000000000000, 0.8660254037844387076, 1.000000000000000000, 0.8660254037844387076, 1.000000000000000000, 0.8660254037844387076, 1.000000000000000000, 0.8660254037844387076, 1.000000000000000000, 0.8660254037844387076, 1.000000000000000000, 0.8660254037844387076, 1.000000000000000000, 0.8660254037844387076, 1.000000000000000000, 0.8660254037844387076, 1.000000000000000000, 0.8660254037844387076, 1.000000000000000000, 0.8660254037844387076, 1.000000000000000000, 0.8660254037844387076, 1.000000000000000000, 0.8660254037844387076, 1.000000000000000000, 0.8660254037844387076, 1.000000000000000000, 0.8660254037844387076, 1.000000000000000000, 0.8660254037844387076, 1.000000000000000000, 0.8660254037844387076, 1.000000000000000000, 0.8660254037844387076, 1.000000000000000000, 0.8660254037844387076, 1.000000000000000000, 0.8660254037844387076, 1.000000000000000000, 0.8660254037844387076, 1.000000000000000000, 0.8660254037844387076, 1.000000000000000000, 0.8660254037844387076, 1.000000000000000000, 0.8660254037844387076, 1.000000000000000000, 0.8660254037844387076, 1.000000000000000000, 0.8660254037844387076, 1.000000000000000000, 0.8660254037844387076, 1.000000000000000000, 0.8660254037844387076, 1.000000000000000000, 0.8660254037844387076, 1.000000000000000000, 0.8660254037844387076, 1.000000000000000000, 0.8660254037844387076, 1.000000000000000000, 0.8660254037844387076, 1.000000000000000000, 0.8660254037844387076, 1.000000000000000000, 0.8660254037844387076, 1.000000000000000000, 0.8660254037844387076, 1.000000000000000000, 0.8660254037844387076, 1.000000000000000000, 0.8660254037844387076, 1.000000000000000000, 0.8660254037844387076, 1.000000000000000000, 0.8660254037844387076, 1.000000000000000000, 0.8660254037844387076, 1.000000000000000000, 0.8660254037844387076, 1.000000000000000000, 0.8660254037844387076, 1.000000000000000000, 0.8660254037844387076, 1.000000000000000000, 0.8660254037844387076, 1.000000000000000000, 0.8660254037844387076, 1.000000000000000000, 0.8660254037844387076, 1.000000000000000000, 0.8660254037844387076, 1.000000000000000000, 0.8660254037844387076, 1.000000000000000000, 0.8660254037844387076, 1.000000000000000000, 0.8660254037844387076, 1.000000000000000000, 0.8660254037844387076, 1.000000000000000000, 0.8660254037844387076, 1.000000000000000000, 0.8660254037844387076, 1.000000000000000000, 0.8660254037844387076, 1.000000000000000000, 0.8660254037844387076, 1.000000000000000000, 0.8660254037844387076, 1.000000000000000000, 0.8660254037844387076, 1.000000000000000000, 0.8660254037844387076, 1.000000000000000000, 0.8660254037844387076, 1.000000000000000000, 0.8660254037844387076, 1.000000000000000000, 0.8660254037844387076, 1.000000000000000000, 0.8660254037844387076, 1.000000000000000000, 0.8660254037844387076, 1.000000000000000000, 0.8660254037844387076, 1.000000000000000000, 0.8660254037844387076, 1.000000000000000000, 0.8660254037844387076, 1.000000000000000000, 0.8660254037844387076, 1.000000000000000000, 0.8660254037844387076, 1.000000000000000000, 0.8660254037844387076, 1.000000000000000000, 0.8660254037844387076, 1.000000000000000000, 0.8660254037844387076, 1.000000000000000000, 0.8660254037844387076, 1.000000000000000000, 0.8660254037844387076, 1.000000000000000000, 0.8660254037844387076, 1.000000000000000000, 0.8660254037844387076, 1.000000000000000000, 0.8660254037844387076, 1.000000000000000000, 0.8660254037844387076, 1.000000000000000000, 0.8660254037844387076, 1.000000000000000000, 0.8660254037844387076, 1.000000000000000000, 0.8660254037844387076, 1.000000000000000000, 0.8660254037844387076, 1.000000000000000000, 0.8660254037844387076, 1.000000000000000000, 0.8660254037844387076, 1.000000000000000000, 0.8660254037844387076, 1.000000000000000000, 0.8660254037844387076, 1.000000000000000000, 0.8660254037844387076, 1.000000000000000000, 0.8660254037844387076, 1.000000000000000000, 0.8660254037844387076, 1.000000000000000000, 0.8660254037844387076, 1.000000000000000000, 0.8660254037844387076, 1.000000000000000000, 0.8660254037844387076, 1.000000000000000000, 0.8660254037844387076, 1.000000000000000000, 0.8660254037844387076, 1.000000000000000000, 0.8660254037844387076, 1.000000000000000000, 0.8660254037844387076, 1.000000000000000000, 0.8660254037844387076, 1.000000000000000000, 0.8660254037844387076, 1.000000000000000000, 0.8660254037844387076, 1.000000000000000000, 0.8660254037844387076, 1.000000000000000000, 0.8660254037844387076, 1.000000000000000000, 0.8660254037844387076, 1.000000000000000000, 0.8660254037844387076, 1.000000000000000000, 0.8660254037844387076, 1.000000000000000000, 0.8660254037844387076, 1.000000000000000000, 0.8660254037844387076, 1.000000000000000000, 0.8660254037844387076, 1.000000000000000000, 0.8660254037844387076, 1.000000000000000000, 0.8660254037844387076, 1.000000000000000000, 0.8660254037844387076, 1.000000000000000000, 0.8660254037844387076, 1.000000000000000000, 0.8660254037844387076, 1.000000000000000000, 0.8660254037844387076, 1.000000000000000000, 0.8660254037844387076, 1.000000000000000000, 0.8660254037844387076, 1.000000000000000000, 0.8660254037844387076, 1.000000000000000000, 0.8660254037844387076, 1.000000000000000000, 0.8660254037844387076, 1.000000000000000000, 0.8660254037844387076, 1.000000000000000000, 0.8660254037844387076, 1.000000000000000000, 0.8660254037844387076, 1.000000000000000000, 0.8660254037844387076, 1.000000000000000000, 0.8660254037844387076, 1.000000000000000000, 0.8660254037844387076, 1.000000000000000000, 0.8660254037844387076, 1.000000000000000000, 0.8660254037844387076, 1.000000000000000000, 0.8660254037844387076, 1.000000000000000000, 0.8660254037844387076, 1.000000000000000000, 0.8660254037844387076, 1.000000000000000000, 0.8660254037844387076, 1.000000000000000000, 0.8660254037844387076, 1.000000000000000000, 0.8660254037844387076, 1.000000000000000000, 0.8660254037844387076, 1.000000000000000000, 0.8660254037844387076, 1.000000000000000000, 0.8660254037844387076, 1.000000000000000000, 0.8660254037844387076, 1.000000000000000000, 0.8660254037844387076, 1.000000000000000000, 0.8660254037844387076, 1.000000000000000000, 0.8660254037844387076, 1.000000000000000000, 0.8660254037844387076, 1.000000000000000000, 0.8660254037844387076, 1.000000000000000000, 0.8660254037844387076, 1.000000000000000000, 0.8660254037844387076, 1.000000000000000000, 0.8660254037844387076, 1.000000000000000000, 0.8660254037844387076, 1.000000000000000000, 0.8660254037844387076, 1.000000000000000000, 0.8660254037844387076, 1.000000000000000000, 0.8660254037844387076, 1.000000000000000000, 0.8660254037844387076, 1.000000000000000000, 0.8660254037844387076, 1.000000000000000000, 0.8660254037844387076, 1.000000000000000000, 0.8660254037844387076, 1.000000000000000000, 0.8660254037844387076, 1.000000000000000000, 0.8660254037844387076, 1.000000000000000000, 0.8660254037844387076, 1.000000000000000000, 0.8660254037844387076, 1.000000000000000000, 0.8660254037844387076, 1.000000000000000000, 0.8660254037844387076, 1.000000000000000000, 0.8660254037844387076, 1.000000000000000000, 0.8660254037844387076, 1.000000000000000000, 0.8660254037844387076, 1.000000000000000000, 0.8660254037844387076, 1.000000000000000000, 0.8660254037844387076, 1.000000000000000000, 0.8660254037844387076, 1.000000000000000000, 0.8660254037844387076, 1.000000000000000000, 0.8660254037844387076, 1.000000000000000000, 0.8660254037844387076, 1.000000000000000000, 0.8660254037844387076, 1.000000000000000000, 0.8660254037844387076, 1.000000000000000000, 0.8660254037844387076, 1.000000000000000000, 0.8660254037844387076, 1.000000000000000000, 0.8660254037844387076, 1.000000000000000000, 0.8660254037844387076, 1.000000000000000000, 0.8660254037844387076, 1.000000000000000000, 0.8660254037844387076, 1.000000000000000000, 0.8660254037844387076, 1.000000000000000000, 0.8660254037844387076, 1.000000000000000000, 0.8660254037844387076, 1.000000000000000000, 0.8660254037844387076, 1.000000000000000000, 0.8660254037844387076, 1.000000000000000000, 0.8660254037844387076, 1.000000000000000000, 0.8660254037844387076, 1.000000000000000000, 0.8660254037844387076, 1.000000000000000000, 0.8660254037844387076, 1.000000000000000000, 0.8660254037844387076, 1.000000000000000000, 0.8660254037844387076, 1.000000000000000000, 0.8660254037844387076, 1.000000000000000000, 0.8660254037844387076, 1.000000000000000000, 0.8660254037844387076, 1.000000000000000000, 0.8660254037844387076, 1.000000000000000000, 0.8660254037844387076, 1.000000000000000000, 0.8660254037844387076, 1.000000000000000000, 0.8660254037844387076, 1.000000000000000000, 0.8660254037844387076, 1.000000000000000000, 0.8660254037844387076, 1.000000000000000000, 0.8660254037844387076, 1.000000000000000000, 0.8660254037844387076, 1.000000000000000000, 0.8660254037844387076, 1.000000000000000000, 0.8660254037844387076, 1.000000000000000000, 0.8660254037844387076, 1.000000000000000000, 0.8660254037844387076, 1.000000000000000000, 0.8660254037844387076, 1.000000000000000000, 0.8660254037844387076, 1.000000000000000000, 0.8660254037844387076, 1.000000000000000000, 0.8660254037844387076, 1.000000000000000000, 0.8660254037844387076, 1.000000000000000000, 0.8660254037844387076, 1.000000000000000000, 0.8660254037844387076, 1.000000000000000000, 0.8660254037844387076, 1.000000000000000000, 0.8660254037844387076, 1.000000000000000000, 0.8660254037844387076, 1.000000000000000000, 0.8660254037844387076, 1.000000000000000000, 0.8660254037844387076, 1.000000000000000000, 0.8660254037844387076, 1.000000000000000000, 0.8660254037844387076, 1.000000000000000000, 0.8660254037844387076, 1.000000000000000000, 0.8660254037844387076, 1.000000000000000000, 0.8660254037844387076, 1.000000000000000000, 0.8660254037844387076, 1.000000000000000000, 0.8660254037844387076, 1.000000000000000000, 0.8660254037844387076, 1.000000000000000000, 0.8660254037844387076, 1.000000000000000000, 0.8660254037844387076, 1.000000000000000000, 0.8660254037844387076, 1.000000000000000000, 0.8660254037844387076, 1.000000000000000000, 0.8660254037844387076, 1.000000000000000000, 0.8660254037844387076, 1.000000000000000000, 0.8660254037844387076, 1.000000000000000000, 0.8660254037844387076, 1.000000000000000000, 0.8660254037844387076, 1.000000000000000000, 0.8660254037844387076, 1.000000000000000000, 0.8660254037844387076, 1.000000000000000000, 0.8660254037844387076, 1.000000000000000000, 0.8660254037844387076, 1.000000000000000000, 0.8660254037844387076, 1.000000000000000000, 0.8660254037844387076, 1.000000000000000000, 0.8660254037844387076, 1.000000000000000000, 0.8660254037844387076, 1.000000000000000000, 0.8660254037844387076, 1.000000000000000000, 0.8660254037844387076, 1.000000000000000000, 0.8660254037844387076, 1.000000000000000000, 0.8660254037844387076, 1.000000000000000000, 0.8660254037844387076, 1.000000000000000000, 0.8660254037844387076, 1.000000000000000000, 0.8660254037844387076, 1.000000000000000000, 0.8660254037844387076, 1.000000000000000000, 0.8660254037844387076, 1.000000000000000000, 0.8660254037844387076, 1.000000000000000000, 0.8660254037844387076, 1.000000000000000000, 0.8660254037844387076, 1.000000000000000000, 0.8660254037844387076, 1.000000000000000000, 0.8660254037844387076, 1.000000000000000000, 0.8660254037844387076, 1.000000000000000000, 0.8660254037844387076, 1.000000000000000000, 0.8660254037844387076, 1.000000000000000000, 0.8660254037844387076, 1.000000000000000000, 0.8660254037844387076, 1.000000000000000000, 0.8660254037844387076, 1.000000000000000000, 0.8660254037844387076, 1.000000000000000000, 0.8660254037844387076, 1.000000000000000000, 0.8660254037844387076, 1.000000000000000000, 0.8660254037844387076, 1.000000000000000000) ) ) 
 REPRESENTATION_ITEM ( '' )  SURFACE ( )  );
#43814=CARTESIAN_POINT ( 'NONE',  ( 4.458734125000001214, 0.8541666680322613781, 2.574251347313718519 ) ) ;
#43816=FACE_OUTER_BOUND ( 'NONE', #29368, .T. ) ;
#43817=CARTESIAN_POINT ( 'NONE',  ( -2.500000000000000444, 28.95833333606451987, -4.330127018922193649 ) ) ;
#43820=CARTESIAN_POINT ( 'NONE',  ( -2.499999999999996447, 6.291666669397851130, 4.330127018922195425 ) ) ;
#43824=CARTESIAN_POINT ( 'NONE',  ( 4.458734125000000326, -74.89583333196773651, 2.574251347313718519 ) ) ;
#43825=CARTESIAN_POINT ( 'NONE',  ( 1.339745962155612702, -0.1696581960073343942, -5.000000000000000000 ) ) ;
#43826=CARTESIAN_POINT ( 'NONE',  ( 2.229367062500001939, 4.020833334698926009, 3.861377020970579999 ) ) ;
#43828=CARTESIAN_POINT ( 'NONE',  ( -4.458734124999999437, -65.64583333196773651, -2.574251347313719407 ) ) ;
#43829=CARTESIAN_POINT ( 'NONE',  ( -5.000000000000000000, -26.95833333060214798, -2.886751345948128211 ) ) ;
#43833=CARTESIAN_POINT ( 'NONE',  ( 4.458734124999999437, -43.81249999863440081, -5.460374474430324690E-16 ) ) ;
#43834=CARTESIAN_POINT ( 'NONE',  ( -4.458734124999999437, -26.56249999863440792, 0.000000000000000000 ) ) ;
#43837=CARTESIAN_POINT ( 'NONE',  ( -4.999999999999999112, 26.08333333333333215, 2.886751345948131764 ) ) ;
#43839=CARTESIAN_POINT ( 'NONE',  ( 5.000000000000000000, -54.37499999726880162, -6.123233995736766282E-16 ) ) ;
#43840=CARTESIAN_POINT ( 'NONE',  ( 2.229367062500001939, -38.97916666530107221, 3.861377020970579999 ) ) ;
#43841=CARTESIAN_POINT ( 'NONE',  ( -5.000000000000000000, -70.95833333060214443, -2.886751345948128211 ) ) ;
#43844=CARTESIAN_POINT ( 'NONE',  ( -4.458734124999997661, -73.47916666530106511, 2.574251347313722516 ) ) ;
#43849=CARTESIAN_POINT ( 'NONE',  ( -4.999999999999999112, -21.91666666666666785, 2.886751345948131764 ) ) ;
#43851=ORIENTED_EDGE ( 'NONE', *, *, #6070, .T. ) ;
#43853=CARTESIAN_POINT ( 'NONE',  ( 5.000000000000000000, -16.29166666393548368, -2.886751345948130876 ) ) ;
#43855=CARTESIAN_POINT ( 'NONE',  ( 5.000000000000000888, 28.54166666939785202, 2.886751345948126879 ) ) ;
#43856=LINE ( 'NONE', #39039, #24738 ) ;
#43858=CARTESIAN_POINT ( 'NONE',  ( -2.500000000000000444, 7.958333336064518093, -4.330127018922193649 ) ) ;
#43860=CARTESIAN_POINT ( 'NONE',  ( -6.031010364368858512E-14, 4.249999999999995559, 5.000000000000000000 ) ) ;
#43862=CARTESIAN_POINT ( 'NONE',  ( 5.000000000000000888, -89.45833333060215864, 2.886751345948126879 ) ) ;
#43863=CARTESIAN_POINT ( 'NONE',  ( 1.339745962155615144, -12.70534180126147739, 4.999999999999999112 ) ) ;
#43864=CARTESIAN_POINT ( 'NONE',  ( -4.458734124999999437, -21.31249999863440436, 0.000000000000000000 ) ) ;
#43865=CARTESIAN_POINT ( 'NONE',  ( 1.975475456537005874E-15, 10.37500000273118417, 5.000000000000000000 ) ) ;
#43868=VECTOR ( 'NONE', #35104, 1000.000000000000000 ) ;
#43874=CARTESIAN_POINT ( 'NONE',  ( 5.000000000000000000, -87.41666666666667140, -2.886751345948130876 ) ) ;
#43875=CARTESIAN_POINT ( 'NONE',  ( -1.339745962155610925, -2.794658198738521726, 5.000000000000000000 ) ) ;
#43878=LINE ( 'NONE', #9475, #9766 ) ;
#43882=ORIENTED_EDGE ( 'NONE', *, *, #42575, .T. ) ;
#43884=CARTESIAN_POINT ( 'NONE',  ( 4.458734124999998549, 21.27083333469892779, -2.574251347313721627 ) ) ;
#43885=CARTESIAN_POINT ( 'NONE',  ( 0.000000000000000000, -120.0000000000000000, 0.000000000000000000 ) ) ;
#43886=ORIENTED_EDGE ( 'NONE', *, *, #7213, .T. ) ;
#43889=CARTESIAN_POINT ( 'NONE',  ( 5.000000000000000888, -88.58333333333332860, 2.886751345948126879 ) ) ;
#43892=CARTESIAN_POINT ( 'NONE',  ( 2.229367062499998831, -59.64583333196774362, -3.861377020970580887 ) ) ;
#43894=CARTESIAN_POINT ( 'NONE',  ( -4.458734124999999437, 19.68750000136559208, 0.000000000000000000 ) ) ;
#43895=ADVANCED_FACE ( 'NONE', ( #58245 ), #54043, .T. ) ;
#43896=( BOUNDED_CURVE ( )  B_SPLINE_CURVE ( 2, ( #20362, #25497, #11017, #39639, #11335, #39960, #35475, #59931, #21000 ),
 .UNSPECIFIED., .F., .F. ) 
 B_SPLINE_CURVE_WITH_KNOTS ( ( 3, 2, 2, 2, 3 ),
 ( 0.3196428571428571175, 0.3202380952380952106, 0.3214285714285714524, 0.3226190476190476386, 0.3232142857142857317 ),
 .UNSPECIFIED. ) 
 CURVE ( )  GEOMETRIC_REPRESENTATION_ITEM ( )  RATIONAL_B_SPLINE_CURVE ( ( 0.9330127018922194093, 0.9330127018922194093, 1.000000000000000000, 0.8660254037844387076, 1.000000000000000000, 0.8660254037844387076, 1.000000000000000000, 0.9330127018922194093, 0.9330127018922194093 ) ) 
 REPRESENTATION_ITEM ( '' )  );
#43898=CARTESIAN_POINT ( 'NONE',  ( 4.458734124999999437, -51.06249999863440792, -5.460374474430324690E-16 ) ) ;
#43899=CARTESIAN_POINT ( 'NONE',  ( 5.000000000000000000, -9.374999997268814056, -6.123233995736766282E-16 ) ) ;
#43900=CARTESIAN_POINT ( 'NONE',  ( -6.972266317189433020E-16, -31.24999999999999645, -5.000000000000000000 ) ) ;
#43903=CARTESIAN_POINT ( 'NONE',  ( -2.229367062499996610, -107.1458333319677365, 3.861377020970582219 ) ) ;
#43904=CARTESIAN_POINT ( 'NONE',  ( -2.229367062499996610, -9.395833331967736513, 3.861377020970582219 ) ) ;
#43905=ORIENTED_EDGE ( 'NONE', *, *, #53448, .T. ) ;
#43908=CARTESIAN_POINT ( 'NONE',  ( -2.229367062499996610, -101.1458333319677365, 3.861377020970582219 ) ) ;
#43910=CARTESIAN_POINT ( 'NONE',  ( -4.458734124999999437, -97.56249999863440792, 0.000000000000000000 ) ) ;
#43913=CARTESIAN_POINT ( 'NONE',  ( 2.499999999999998668, -51.20833333060213732, -4.330127018922193649 ) ) ;
#43918=CARTESIAN_POINT ( 'NONE',  ( -3.152548672688508926E-16, -18.56249999863440792, -5.148502694627439702 ) ) ;
#43919=CARTESIAN_POINT ( 'NONE',  ( -2.229367062499996610, 9.604166668032261711, 3.861377020970582219 ) ) ;
#43920=CARTESIAN_POINT ( 'NONE',  ( -2.229367062500000163, -57.72916666530107932, -3.861377020970580443 ) ) ;
#43925=CARTESIAN_POINT ( 'NONE',  ( 5.000000000000000000, -5.499999999999998224, -6.123233995736766282E-16 ) ) ;
#43926=EDGE_LOOP ( 'NONE', ( #58475, #59197, #10833, #17800 ) ) ;
#43929=CARTESIAN_POINT ( 'NONE',  ( 0.000000000000000000, -120.0000000000000000, 0.000000000000000000 ) ) ;
#43930=CARTESIAN_POINT ( 'NONE',  ( 4.458734124999998549, -85.72916666530106511, -2.574251347313721627 ) ) ;
#43931=CARTESIAN_POINT ( 'NONE',  ( -4.458734124999999437, 21.35416666803225993, -2.574251347313719407 ) ) ;
#43934=CARTESIAN_POINT ( 'NONE',  ( 1.975475456537005874E-15, -82.74999999999998579, 5.000000000000000000 ) ) ;
#43938=CARTESIAN_POINT ( 'NONE',  ( -5.000000000000000000, -77.00000000000000000, 0.000000000000000000 ) ) ;
#43940=ORIENTED_EDGE ( 'NONE', *, *, #32893, .T. ) ;
#43941=DIRECTION ( 'NONE',  ( -0.000000000000000000, 1.000000000000000000, -0.000000000000000000 ) ) ;
#43948=VERTEX_POINT ( 'NONE', #5164 ) ;
#43955=CARTESIAN_POINT ( 'NONE',  ( 4.458734125000001214, -55.14583333196772941, 2.574251347313718519 ) ) ;
#43959=VERTEX_POINT ( 'NONE', #19315 ) ;
#43963=ORIENTED_EDGE ( 'NONE', *, *, #57908, .F. ) ;
#43966=CARTESIAN_POINT ( 'NONE',  ( -4.458734124999999437, -105.6458333319677507, -2.574251347313719407 ) ) ;
#43967=CARTESIAN_POINT ( 'NONE',  ( 1.975475456537005874E-15, -68.62499999726881583, 5.000000000000000000 ) ) ;
#43971=CARTESIAN_POINT ( 'NONE',  ( 4.458734124999998549, -36.72916666530107221, -2.574251347313721627 ) ) ;
#43975=EDGE_CURVE ( 'NONE', #47768, #37487, #3169, .T. ) ;
#43976=CARTESIAN_POINT ( 'NONE',  ( -3.152548672688508926E-16, -13.56249999863440259, -5.148502694627439702 ) ) ;
#43977=CARTESIAN_POINT ( 'NONE',  ( -4.458734124999999437, -102.5624999986344079, 0.000000000000000000 ) ) ;
#43978=VERTEX_POINT ( 'NONE', #19633 ) ;
#43980=CARTESIAN_POINT ( 'NONE',  ( 2.229367062500001939, -31.22916666530107221, 3.861377020970579999 ) ) ;
#43981=CARTESIAN_POINT ( 'NONE',  ( 0.000000000000000000, -120.0000000000000000, 0.000000000000000000 ) ) ;
#43987=CARTESIAN_POINT ( 'NONE',  ( 4.458734125000000326, 4.854166668032262599, 2.574251347313718519 ) ) ;
#43989=CARTESIAN_POINT ( 'NONE',  ( -6.972266317189433020E-16, 1.750000000000000444, -5.000000000000000000 ) ) ;
#43991=CARTESIAN_POINT ( 'NONE',  ( -5.000000000000000000, -97.00000000000000000, 0.000000000000000000 ) ) ;
#43992=CARTESIAN_POINT ( 'NONE',  ( 2.229367062499998831, -32.64583333196773651, -3.861377020970580887 ) ) ;
#43993=EDGE_CURVE ( 'NONE', #34951, #51281, #718, .T. ) ;
#43995=CARTESIAN_POINT ( 'NONE',  ( 9.457646018065525792E-16, -78.31249999863442213, 5.148502694627439702 ) ) ;
#43999=CARTESIAN_POINT ( 'NONE',  ( 4.458734124999998549, -0.7291666653010709931, -2.574251347313721627 ) ) ;
#44000=CARTESIAN_POINT ( 'NONE',  ( -2.229367062499996610, 28.60416666803226349, 3.861377020970582219 ) ) ;
#44002=CARTESIAN_POINT ( 'NONE',  ( 4.458734124999998549, -44.97916666530107221, -2.574251347313721627 ) ) ;
#44008=CARTESIAN_POINT ( 'NONE',  ( -2.229367062500000163, -68.47916666530107932, -3.861377020970580443 ) ) ;
#44009=CARTESIAN_POINT ( 'NONE',  ( -2.499999999999996447, -104.7083333306021444, 4.330127018922195425 ) ) ;
#44011=CARTESIAN_POINT ( 'NONE',  ( 2.499999999999998668, -58.20833333060214443, -4.330127018922193649 ) ) ;
#44012=CARTESIAN_POINT ( 'NONE',  ( -3.152548672688508926E-16, -109.8124999986343795, -5.148502694627439702 ) ) ;
#44014=CARTESIAN_POINT ( 'NONE',  ( 2.499999999999998668, -55.33333333333332860, -4.330127018922193649 ) ) ;
#44015=FACE_OUTER_BOUND ( 'NONE', #53307, .T. ) ;
#44018=CARTESIAN_POINT ( 'NONE',  ( 1.975475456537005874E-15, -99.74999999999998579, 5.000000000000000000 ) ) ;
#44022=ADVANCED_FACE ( 'NONE', ( #34106 ), #28340, .T. ) ;
#44028=CARTESIAN_POINT ( 'NONE',  ( 1.339745962155612702, 5.705341801261479162, -5.000000000000000000 ) ) ;
#44029=CARTESIAN_POINT ( 'NONE',  ( 5.000000000000000000, -45.37499999726880873, -6.123233995736766282E-16 ) ) ;
#44035=CARTESIAN_POINT ( 'NONE',  ( 4.458734125000001214, -41.14583333196774362, 2.574251347313718519 ) ) ;
#44038=CARTESIAN_POINT ( 'NONE',  ( -6.972266317189433020E-16, -57.12499999726879452, -5.000000000000000000 ) ) ;
#44044=CARTESIAN_POINT ( 'NONE',  ( 2.229367062500001939, -91.22916666530106511, 3.861377020970579999 ) ) ;
#44046=EDGE_LOOP ( 'NONE', ( #39756, #10438, #11925, #56862 ) ) ;
#44047=CARTESIAN_POINT ( 'NONE',  ( 2.499999999999998668, -19.20833333060214798, -4.330127018922193649 ) ) ;
#44053=CARTESIAN_POINT ( 'NONE',  ( 9.457646018065525792E-16, 0.9375000013655959696, 5.148502694627439702 ) ) ;
#44057=CARTESIAN_POINT ( 'NONE',  ( 2.229367062499998831, -12.89583333196774007, -3.861377020970580887 ) ) ;
#44058=ADVANCED_FACE ( 'NONE', ( #55343 ), #30229, .T. ) ;
#44062=CARTESIAN_POINT ( 'NONE',  ( 9.457646018065525792E-16, 21.68750000136559208, 5.148502694627439702 ) ) ;
#44063=ORIENTED_EDGE ( 'NONE', *, *, #43620, .F. ) ;
#44064=CARTESIAN_POINT ( 'NONE',  ( 9.457646018065525792E-16, -99.06249999863440792, 5.148502694627439702 ) ) ;
#44065=CYLINDRICAL_SURFACE ( 'NONE', #51071, 5.000000000000000000 ) ;
#44067=CARTESIAN_POINT ( 'NONE',  ( 2.229367062500001939, -12.97916666530107221, 3.861377020970579999 ) ) ;
#44072=CARTESIAN_POINT ( 'NONE',  ( 2.500000000000002220, -40.54166666393548013, 4.330127018922192761 ) ) ;
#44073=DIRECTION ( 'NONE',  ( -0.000000000000000000, 1.000000000000000000, -0.000000000000000000 ) ) ;
#44074=CARTESIAN_POINT ( 'NONE',  ( -4.458734124999997661, 12.77083333469892779, 2.574251347313722516 ) ) ;
#44075=CARTESIAN_POINT ( 'NONE',  ( 1.339745962155612702, -46.16965819600732601, -5.000000000000000000 ) ) ;
#44079=ADVANCED_FACE ( 'NONE', ( #55663 ), #670, .T. ) ;
#44080=CARTESIAN_POINT ( 'NONE',  ( 9.457646018065525792E-16, -64.06249999863440792, 5.148502694627439702 ) ) ;
#44082=CARTESIAN_POINT ( 'NONE',  ( -2.500000000000000444, 4.833333333333332149, -4.330127018922193649 ) ) ;
#44085=EDGE_CURVE ( 'NONE', #13643, #41864, #31196, .T. ) ;
#44086=CARTESIAN_POINT ( 'NONE',  ( -2.229367062500000163, -52.47916666530107221, -3.861377020970580443 ) ) ;
#44087=CARTESIAN_POINT ( 'NONE',  ( -2.499999999999996447, -87.70833333060214443, 4.330127018922195425 ) ) ;
#44088=CARTESIAN_POINT ( 'NONE',  ( -4.458734124999999437, -26.39583333196774007, -2.574251347313719407 ) ) ;
#44090=CARTESIAN_POINT ( 'NONE',  ( 1.975475456537005874E-15, -16.74999999999999645, 5.000000000000000000 ) ) ;
#44091=CARTESIAN_POINT ( 'NONE',  ( 1.975475456537005874E-15, -28.62499999726881583, 5.000000000000000000 ) ) ;
#44094=CARTESIAN_POINT ( 'NONE',  ( 5.000000000000000000, -39.41666666666666430, -2.886751345948129988 ) ) ;
#44098=CARTESIAN_POINT ( 'NONE',  ( 4.458734124999998549, -102.7291666653010509, -2.574251347313721627 ) ) ;
#44099=CARTESIAN_POINT ( 'NONE',  ( -4.458734124999998549, 4.520833334698926009, 2.574251347313722516 ) ) ;
#44107=CYLINDRICAL_SURFACE ( 'NONE', #13219, 5.000000000000000000 ) ;
#44109=CARTESIAN_POINT ( 'NONE',  ( -6.972266317189433020E-16, -20.24999999999999289, -5.000000000000000000 ) ) ;
#44112=CARTESIAN_POINT ( 'NONE',  ( -3.152548672688508926E-16, -23.81249999863440792, -5.148502694627439702 ) ) ;
#44113=CARTESIAN_POINT ( 'NONE',  ( -2.500000000000000444, 21.95833333606451987, -4.330127018922193649 ) ) ;
#44120=EDGE_LOOP ( 'NONE', ( #42529, #19005, #4896, #60448 ) ) ;
#44123=CARTESIAN_POINT ( 'NONE',  ( 9.457646018065525792E-16, -74.31249999863440792, 5.148502694627439702 ) ) ;
#44124=CARTESIAN_POINT ( 'NONE',  ( -6.972266317189433020E-16, -103.2500000000000000, -5.000000000000000000 ) ) ;
#44131=CARTESIAN_POINT ( 'NONE',  ( 2.229367062500001939, -0.2291666653010705768, 3.861377020970579999 ) ) ;
#44133=DIRECTION ( 'NONE',  ( -0.000000000000000000, 1.000000000000000000, -0.000000000000000000 ) ) ;
#44140=CARTESIAN_POINT ( 'NONE',  ( -4.458734124999999437, -80.39583333196773651, -2.574251347313719407 ) ) ;
#44141=DIRECTION ( 'NONE',  ( 0.000000000000000000, 0.000000000000000000, 1.000000000000000000 ) ) ;
#44142=CARTESIAN_POINT ( 'NONE',  ( -2.229367062499996610, 3.854166668032260823, 3.861377020970582219 ) ) ;
#44144=CARTESIAN_POINT ( 'NONE',  ( -4.999999999999999112, -82.91666666666667140, 2.886751345948131764 ) ) ;
#44145=CARTESIAN_POINT ( 'NONE',  ( -2.229367062500000163, -65.72916666530106511, -3.861377020970580443 ) ) ;
#44146=CARTESIAN_POINT ( 'NONE',  ( -5.000000000000000000, -24.87499999726881583, 0.000000000000000000 ) ) ;
#44147=DIRECTION ( 'NONE',  ( 0.000000000000000000, 0.000000000000000000, 1.000000000000000000 ) ) ;
#44148=CARTESIAN_POINT ( 'NONE',  ( -1.339745962155613812, -1.080341798530293218, -5.000000000000000000 ) ) ;
#44149=CARTESIAN_POINT ( 'NONE',  ( -6.972266317189433020E-16, -49.24999999999999289, -5.000000000000000000 ) ) ;
#44150=DIRECTION ( 'NONE',  ( 0.5000000000000009992, 0.000000000000000000, 0.8660254037844380415 ) ) ;
#44152=CARTESIAN_POINT ( 'NONE',  ( -2.229367062499996610, -45.14583333196774362, 3.861377020970582219 ) ) ;
#44153=CARTESIAN_POINT ( 'NONE',  ( 4.458734125000000326, -31.14583333196773651, 2.574251347313718519 ) ) ;
#44156=CYLINDRICAL_SURFACE ( 'NONE', #12397, 5.000000000000000000 ) ;
#44157=CARTESIAN_POINT ( 'NONE',  ( 5.000000000000000000, 26.58333333333333570, -2.886751345948129988 ) ) ;
#44161=CARTESIAN_POINT ( 'NONE',  ( 4.458734124999999437, -36.81249999863440792, -5.460374474430324690E-16 ) ) ;
#44162=CARTESIAN_POINT ( 'NONE',  ( -5.000000000000000000, -70.87499999726880162, 0.000000000000000000 ) ) ;
#44167=CARTESIAN_POINT ( 'NONE',  ( 4.458734124999998549, -72.97916666530107932, -2.574251347313721627 ) ) ;
#44170=CARTESIAN_POINT ( 'NONE',  ( 2.500000000000002220, 18.45833333606451632, 4.330127018922192761 ) ) ;
#44172=CARTESIAN_POINT ( 'NONE',  ( 5.000000000000000000, -19.49999999999999645, -6.123233995736766282E-16 ) ) ;
#44174=VERTEX_POINT ( 'NONE', #30553 ) ;
#44178=CARTESIAN_POINT ( 'NONE',  ( -2.500000000000000444, 22.95833333606451632, -4.330127018922193649 ) ) ;
#44185=CARTESIAN_POINT ( 'NONE',  ( -1.339745962155497683, -77.20534180126146850, -5.000000000000066613 ) ) ;
#44188=( BOUNDED_CURVE ( )  B_SPLINE_CURVE ( 2, ( #3747, #33635, #48109, #4061, #48419, #37840, #62610, #43279, #62917 ),
 .UNSPECIFIED., .F., .F. ) 
 B_SPLINE_CURVE_WITH_KNOTS ( ( 3, 2, 2, 2, 3 ),
 ( 0.5160714285714286254, 0.5166666666666667185, 0.5178571428571429047, 0.5190476190476190910, 0.5196428571428571841 ),
 .UNSPECIFIED. ) 
 CURVE ( )  GEOMETRIC_REPRESENTATION_ITEM ( )  RATIONAL_B_SPLINE_CURVE ( ( 0.9330127018922194093, 0.9330127018922256266, 1.000000000000000000, 0.8660254037844387076, 1.000000000000000000, 0.8660254037844387076, 1.000000000000000000, 0.9330127018922194093, 0.9330127018922194093 ) ) 
 REPRESENTATION_ITEM ( '' )  );
#44189=CARTESIAN_POINT ( 'NONE',  ( 2.500000000000002220, 18.33333333333333215, 4.330127018922192761 ) ) ;
#44190=CARTESIAN_POINT ( 'NONE',  ( 4.458734125000001214, -22.89583333196773651, 2.574251347313718519 ) ) ;
#44196=CARTESIAN_POINT ( 'NONE',  ( -6.972266317189433020E-16, 24.87500000273118417, -5.000000000000000000 ) ) ;
#44200=CARTESIAN_POINT ( 'NONE',  ( -5.000000000000000000, -29.08333333333332860, -2.886751345948128211 ) ) ;
#44203=CARTESIAN_POINT ( 'NONE',  ( -5.000000000000000000, 10.91666666666666607, -2.886751345948128211 ) ) ;
#44205=CARTESIAN_POINT ( 'NONE',  ( 1.975475456537005874E-15, -53.62499999726880162, 5.000000000000000000 ) ) ;
#44207=VERTEX_POINT ( 'NONE', #20921 ) ;
#44208=LINE ( 'NONE', #53556, #44992 ) ;
#44209=CARTESIAN_POINT ( 'NONE',  ( 2.229367062500001939, 20.02083333469892779, 3.861377020970579999 ) ) ;
#44214=CARTESIAN_POINT ( 'NONE',  ( 1.339745962155600711, 12.41965820146970501, 5.000000000000007994 ) ) ;
#44217=CARTESIAN_POINT ( 'NONE',  ( 4.458734124999999437, -59.81249999863440081, -5.460374474430324690E-16 ) ) ;
#44219=CARTESIAN_POINT ( 'NONE',  ( -4.458734124999999437, 15.60416666803225993, -2.574251347313719407 ) ) ;
#44221=CARTESIAN_POINT ( 'NONE',  ( 2.229367062499998831, -51.89583333196773651, -3.861377020970580887 ) ) ;
#44222=CARTESIAN_POINT ( 'NONE',  ( -2.499999999999996447, -9.708333330602146205, 4.330127018922195425 ) ) ;
#44225=CARTESIAN_POINT ( 'NONE',  ( -4.999999999999998224, -73.91666666666667140, 2.886751345948131764 ) ) ;
#44226=CARTESIAN_POINT ( 'NONE',  ( 9.457646018065525792E-16, -109.0624999986344221, 5.148502694627439702 ) ) ;
#44228=CARTESIAN_POINT ( 'NONE',  ( -4.458734124999999437, -12.64583333196774007, -2.574251347313719407 ) ) ;
#44231=CARTESIAN_POINT ( 'NONE',  ( -4.458734124999998549, -99.22916666530105090, 2.574251347313722516 ) ) ;
#44233=CARTESIAN_POINT ( 'NONE',  ( 4.458734124999999437, -97.06249999863440792, -5.460374474430324690E-16 ) ) ;
#44236=CARTESIAN_POINT ( 'NONE',  ( 5.000000000000000000, -58.37499999726880873, -6.123233995736766282E-16 ) ) ;
#44240=CARTESIAN_POINT ( 'NONE',  ( -4.458734124999997661, -16.22916666530107577, 2.574251347313722516 ) ) ;
#44241=CARTESIAN_POINT ( 'NONE',  ( -2.229367062500000163, 4.270833334698926897, -3.861377020970580443 ) ) ;
#44242=CARTESIAN_POINT ( 'NONE',  ( 4.458734124999998549, -58.97916666530106511, -2.574251347313721627 ) ) ;
#44243=DIRECTION ( 'NONE',  ( -0.000000000000000000, 1.000000000000000000, -0.000000000000000000 ) ) ;
#44245=DIRECTION ( 'NONE',  ( -0.000000000000000000, 1.000000000000000000, -0.000000000000000000 ) ) ;
#44247=CARTESIAN_POINT ( 'NONE',  ( -4.999999999999999112, -3.916666666666665630, 2.886751345948131764 ) ) ;
#44248=VERTEX_POINT ( 'NONE', #27643 ) ;
#44253=CARTESIAN_POINT ( 'NONE',  ( -3.152548672688508926E-16, -84.56249999863439371, -5.148502694627439702 ) ) ;
#44254=CARTESIAN_POINT ( 'NONE',  ( -4.458734124999999437, 16.43750000136559564, 0.000000000000000000 ) ) ;
#44256=CARTESIAN_POINT ( 'NONE',  ( -2.499999999999996447, -88.70833333060214443, 4.330127018922195425 ) ) ;
#44258=CARTESIAN_POINT ( 'NONE',  ( 5.000000000000000000, 20.70833333606451987, -2.886751345948130876 ) ) ;
#44260=CARTESIAN_POINT ( 'NONE',  ( -2.500000000000000444, -73.16666666666665719, -4.330127018922193649 ) ) ;
#44263=DIRECTION ( 'NONE',  ( -0.000000000000000000, 1.000000000000000000, -0.000000000000000000 ) ) ;
#44264=ORIENTED_EDGE ( 'NONE', *, *, #51925, .F. ) ;
#44276=VERTEX_POINT ( 'NONE', #22195 ) ;
#44279=CARTESIAN_POINT ( 'NONE',  ( -2.229367062500000163, -55.72916666530107221, -3.861377020970580443 ) ) ;
#44281=CARTESIAN_POINT ( 'NONE',  ( 0.000000000000000000, -120.0000000000000000, 0.000000000000000000 ) ) ;
#44287=( BOUNDED_CURVE ( )  B_SPLINE_CURVE ( 2, ( #44863, #4995, #1151, #44543, #20104, #50008, #40357, #29742, #20434 ),
 .UNSPECIFIED., .F., .F. ) 
 B_SPLINE_CURVE_WITH_KNOTS ( ( 3, 2, 2, 2, 3 ),
 ( 0.08392857142857143571, 0.08452380952380952883, 0.08571428571428571508, 0.08690476190476190133, 0.08750000000000000833 ),
 .UNSPECIFIED. ) 
 CURVE ( )  GEOMETRIC_REPRESENTATION_ITEM ( )  RATIONAL_B_SPLINE_CURVE ( ( 0.9330127018922192983, 0.9330127018922200755, 1.000000000000000000, 0.8660254037844387076, 1.000000000000000000, 0.8660254037844387076, 1.000000000000000000, 0.9330127018922185211, 0.9330127018922192983 ) ) 
 REPRESENTATION_ITEM ( '' )  );
#44289=CARTESIAN_POINT ( 'NONE',  ( -4.458734124999999437, -106.6458333319677365, -2.574251347313719407 ) ) ;
#44291=ORIENTED_EDGE ( 'NONE', *, *, #15606, .F. ) ;
#44294=CARTESIAN_POINT ( 'NONE',  ( 2.229367062499998831, -36.64583333196773651, -3.861377020970580887 ) ) ;
#44297=CARTESIAN_POINT ( 'NONE',  ( -2.229367062500000163, -11.47916666530107044, -3.861377020970580443 ) ) ;
#44298=CARTESIAN_POINT ( 'NONE',  ( 2.229367062500001939, -103.2291666653010651, 3.861377020970579999 ) ) ;
#44301=CARTESIAN_POINT ( 'NONE',  ( 4.458734124999998549, -34.97916666530107221, -2.574251347313721627 ) ) ;
#44302=CARTESIAN_POINT ( 'NONE',  ( -2.500000000000000444, 4.958333336064518981, -4.330127018922193649 ) ) ;
#44309=CARTESIAN_POINT ( 'NONE',  ( 2.229367062500001939, 6.770833334698928674, 3.861377020970579999 ) ) ;
#44310=ORIENTED_EDGE ( 'NONE', *, *, #44508, .F. ) ;
#44312=CARTESIAN_POINT ( 'NONE',  ( -2.499999999999996447, 16.29166666939785202, 4.330127018922195425 ) ) ;
#44313=CARTESIAN_POINT ( 'NONE',  ( -2.499999999999996447, -94.83333333333332860, 4.330127018922195425 ) ) ;
#44314=CARTESIAN_POINT ( 'NONE',  ( -4.458734124999999437, -31.31249999863440436, 0.000000000000000000 ) ) ;
#44315=CARTESIAN_POINT ( 'NONE',  ( 1.339745962155615144, -95.70534180126146850, 4.999999999999999112 ) ) ;
#44316=CARTESIAN_POINT ( 'NONE',  ( 4.458734124999999437, -83.06249999863440792, -5.460374474430324690E-16 ) ) ;
#44318=CARTESIAN_POINT ( 'NONE',  ( -5.000000000000000000, -101.8749999972688158, 0.000000000000000000 ) ) ;
#44320=CARTESIAN_POINT ( 'NONE',  ( 2.229367062500001939, -2.979166665301069550, 3.861377020970579999 ) ) ;
#44321=CARTESIAN_POINT ( 'NONE',  ( -3.152548672688508926E-16, 21.18750000136559208, -5.148502694627439702 ) ) ;
#44322=CARTESIAN_POINT ( 'NONE',  ( 9.457646018065525792E-16, -41.31249999863440792, 5.148502694627439702 ) ) ;
#44327=CARTESIAN_POINT ( 'NONE',  ( 2.229367062499998831, -71.64583333196773651, -3.861377020970580887 ) ) ;
#44328=CARTESIAN_POINT ( 'NONE',  ( 2.500000000000002220, -105.5416666639354730, 4.330127018922192761 ) ) ;
#44330=CARTESIAN_POINT ( 'NONE',  ( -4.458734124999997661, -109.4791666653010651, 2.574251347313722516 ) ) ;
#44332=CARTESIAN_POINT ( 'NONE',  ( -3.535250795749689387E-16, -58.24999999999999289, -5.773502691896257311 ) ) ;
#44333=PLANE ( 'NONE',  #6904 ) ;
#44337=( BOUNDED_CURVE ( )  B_SPLINE_CURVE ( 2, ( #14196, #29940, #15155, #38952, #19021, #58590, #24809, #34439, #54068 ),
 .UNSPECIFIED., .F., .F. ) 
 B_SPLINE_CURVE_WITH_KNOTS ( ( 3, 2, 2, 2, 3 ),
 ( 0.9089285714285714191, 0.9095238095238095122, 0.9107142857142856984, 0.9119047619047618847, 0.9124999999999999778 ),
 .UNSPECIFIED. ) 
 CURVE ( )  GEOMETRIC_REPRESENTATION_ITEM ( )  RATIONAL_B_SPLINE_CURVE ( ( 0.9330127018922194093, 0.9330127018922194093, 1.000000000000000000, 0.8660254037844387076, 1.000000000000000000, 0.8660254037844387076, 1.000000000000000000, 0.9330127018922194093, 0.9330127018922194093 ) ) 
 REPRESENTATION_ITEM ( '' )  );
#44341=EDGE_CURVE ( 'NONE', #37188, #2754, #16729, .T. ) ;
#44348=CARTESIAN_POINT ( 'NONE',  ( -6.972266317189433020E-16, -98.24999999999998579, -5.000000000000000000 ) ) ;
#44354=CARTESIAN_POINT ( 'NONE',  ( -2.229367062500000163, -38.72916666530107221, -3.861377020970580443 ) ) ;
#44357=DIRECTION ( 'NONE',  ( 0.000000000000000000, 0.000000000000000000, 1.000000000000000000 ) ) ;
#44361=ADVANCED_FACE ( 'NONE', ( #17982 ), #3216, .T. ) ;
#44365=CARTESIAN_POINT ( 'NONE',  ( 2.229367062499998831, -87.89583333196773651, -3.861377020970580887 ) ) ;
#44368=DIRECTION ( 'NONE',  ( -1.000000000000000000, 0.000000000000000000, 3.305092117221761110E-15 ) ) ;
#44374=CARTESIAN_POINT ( 'NONE',  ( 4.458734125000001214, 2.104166668032262599, 2.574251347313718519 ) ) ;
#44376=CARTESIAN_POINT ( 'NONE',  ( 2.229367062499998831, -16.89583333196773651, -3.861377020970580887 ) ) ;
#44377=CARTESIAN_POINT ( 'NONE',  ( -2.499999999999996447, -100.7083333306021444, 4.330127018922195425 ) ) ;
#44379=CARTESIAN_POINT ( 'NONE',  ( 5.000000000000000888, -55.45833333060214443, 2.886751345948126879 ) ) ;
#44382=CARTESIAN_POINT ( 'NONE',  ( 2.229367062499998831, 22.10416666803225993, -3.861377020970580887 ) ) ;
#44383=ORIENTED_EDGE ( 'NONE', *, *, #43292, .F. ) ;
#44384=CARTESIAN_POINT ( 'NONE',  ( -3.152548672688508926E-16, -99.56249999863440792, -5.148502694627439702 ) ) ;
#44387=CARTESIAN_POINT ( 'NONE',  ( -3.152548672688508926E-16, -11.56249999863440792, -5.148502694627439702 ) ) ;
#44388=CARTESIAN_POINT ( 'NONE',  ( 1.339745962155615144, -39.58034179853028434, 4.999999999999999112 ) ) ;
#44389=CARTESIAN_POINT ( 'NONE',  ( -6.972266317189433020E-16, -97.24999999999998579, -5.000000000000000000 ) ) ;
#44390=CARTESIAN_POINT ( 'NONE',  ( -6.972266317189433020E-16, -67.25000000000000000, -5.000000000000000000 ) ) ;
#44391=EDGE_CURVE ( 'NONE', #57684, #248, #25315, .T. ) ;
#44392=CARTESIAN_POINT ( 'NONE',  ( 2.500000000000002220, -39.54166666393548013, 4.330127018922192761 ) ) ;
#44393=CARTESIAN_POINT ( 'NONE',  ( -1.339745962155613812, 20.91965820146970501, -5.000000000000000000 ) ) ;
#44394=CARTESIAN_POINT ( 'NONE',  ( -4.458734124999999437, 11.60416666803225993, -2.574251347313719407 ) ) ;
#44398=CARTESIAN_POINT ( 'NONE',  ( 9.457646018065525792E-16, -63.06249999863440081, 5.148502694627439702 ) ) ;
#44402=CARTESIAN_POINT ( 'NONE',  ( 5.000000000000000000, 2.583333333333333481, -2.886751345948129988 ) ) ;
#44404=CARTESIAN_POINT ( 'NONE',  ( 1.975475456537005874E-15, -59.62499999726880873, 5.000000000000000000 ) ) ;
#44405=CARTESIAN_POINT ( 'NONE',  ( 2.229367062500001939, -52.97916666530107221, 3.861377020970579999 ) ) ;
#44406=CARTESIAN_POINT ( 'NONE',  ( 5.000000000000000888, -89.45833333060215864, 2.886751345948126879 ) ) ;
#44407=CARTESIAN_POINT ( 'NONE',  ( -4.458734124999999437, -35.31249999863440792, 0.000000000000000000 ) ) ;
#44408=CARTESIAN_POINT ( 'NONE',  ( -1.339745962155610925, 20.33034180399266688, 5.000000000000000000 ) ) ;
#44411=CARTESIAN_POINT ( 'NONE',  ( -5.000000000000000000, -46.08333333333333570, -2.886751345948128211 ) ) ;
#44412=FACE_OUTER_BOUND ( 'NONE', #58320, .T. ) ;
#44414=VERTEX_POINT ( 'NONE', #25924 ) ;
#44415=CARTESIAN_POINT ( 'NONE',  ( -4.458734124999998549, -102.2291666653010651, 2.574251347313722516 ) ) ;
#44416=CARTESIAN_POINT ( 'NONE',  ( -2.229367062500000163, 3.270833334698929118, -3.861377020970580443 ) ) ;
#44419=EDGE_CURVE ( 'NONE', #50232, #50678, #27016, .T. ) ;
#44422=ADVANCED_FACE ( 'NONE', ( #1826 ), #31064, .F. ) ;
#44423=ADVANCED_FACE ( 'NONE', ( #40709 ), #34945, .T. ) ;
#44427=CARTESIAN_POINT ( 'NONE',  ( -2.499999999999996447, -10.83333333333333393, 4.330127018922195425 ) ) ;
#44428=CARTESIAN_POINT ( 'NONE',  ( 0.000000000000000000, -120.0000000000000000, 0.000000000000000000 ) ) ;
#44429=ORIENTED_EDGE ( 'NONE', *, *, #56317, .F. ) ;
#44430=CARTESIAN_POINT ( 'NONE',  ( 2.499999999999998668, -20.33333333333333570, -4.330127018922193649 ) ) ;
#44433=CARTESIAN_POINT ( 'NONE',  ( 2.229367062499998831, -22.89583333196773651, -3.861377020970580887 ) ) ;
#44442=VERTEX_POINT ( 'NONE', #49730 ) ;
#44443=CARTESIAN_POINT ( 'NONE',  ( -6.972266317189433020E-16, -41.24999999999999289, -5.000000000000000000 ) ) ;
#44445=ORIENTED_EDGE ( 'NONE', *, *, #33124, .F. ) ;
#44446=CARTESIAN_POINT ( 'NONE',  ( -4.458734124999999437, -73.56249999863439371, 0.000000000000000000 ) ) ;
#44450=CARTESIAN_POINT ( 'NONE',  ( 2.499999999999998668, 12.66666666666666607, -4.330127018922193649 ) ) ;
#44451=CARTESIAN_POINT ( 'NONE',  ( 1.339745962155612702, -31.16965819600732956, -5.000000000000000000 ) ) ;
#44453=CARTESIAN_POINT ( 'NONE',  ( 9.457646018065525792E-16, -4.312499998634408804, 5.148502694627439702 ) ) ;
#44454=EDGE_LOOP ( 'NONE', ( #20476, #11640, #31080, #13586 ) ) ;
#44456=LINE ( 'NONE', #30944, #35633 ) ;
#44462=CARTESIAN_POINT ( 'NONE',  ( -2.229367062500000163, -83.47916666530106511, -3.861377020970580443 ) ) ;
#44464=CARTESIAN_POINT ( 'NONE',  ( -3.152548672688508926E-16, 1.437500001365596525, -5.148502694627439702 ) ) ;
#44466=CARTESIAN_POINT ( 'NONE',  ( -5.000000000000000000, -82.99999999999998579, 0.000000000000000000 ) ) ;
#44468=CARTESIAN_POINT ( 'NONE',  ( 4.458734124999999437, -64.06249999863440792, -5.460374474430324690E-16 ) ) ;
#44469=CARTESIAN_POINT ( 'NONE',  ( -5.000000000000000000, -24.95833333060214798, -2.886751345948128211 ) ) ;
#44470=DIRECTION ( 'NONE',  ( 0.000000000000000000, 0.000000000000000000, 1.000000000000000000 ) ) ;
#44473=CARTESIAN_POINT ( 'NONE',  ( -3.152548672688508926E-16, -43.56249999863440081, -5.148502694627439702 ) ) ;
#44474=CARTESIAN_POINT ( 'NONE',  ( -3.152548672688508926E-16, -29.81249999863440436, -5.148502694627439702 ) ) ;
#44477=CARTESIAN_POINT ( 'NONE',  ( -2.500000000000000444, 19.83333333333333570, -4.330127018922193649 ) ) ;
#44479=CARTESIAN_POINT ( 'NONE',  ( -4.729367062499999719, -110.7187499979515906, 0.000000000000000000 ) ) ;
#44480=CARTESIAN_POINT ( 'NONE',  ( -4.458734124999998549, -35.22916666530107221, 2.574251347313722516 ) ) ;
#44481=CARTESIAN_POINT ( 'NONE',  ( -2.499999999999996447, -71.70833333060214443, 4.330127018922195425 ) ) ;
#44483=CARTESIAN_POINT ( 'NONE',  ( 1.975475456537005874E-15, -24.62499999726881583, 5.000000000000000000 ) ) ;
#44485=CARTESIAN_POINT ( 'NONE',  ( -4.458734124999999437, -78.56249999863440792, 0.000000000000000000 ) ) ;
#44490=CARTESIAN_POINT ( 'NONE',  ( 1.060575238724906964E-15, -21.75000000000000000, 5.773502691896257311 ) ) ;
#44496=CARTESIAN_POINT ( 'NONE',  ( -5.000000000000000000, 23.12500000273118417, 0.000000000000000000 ) ) ;
#44507=CARTESIAN_POINT ( 'NONE',  ( 2.229367062500001939, -18.97916666530106866, 3.861377020970579999 ) ) ;
#44508=EDGE_CURVE ( 'NONE', #62283, #20660, #1191, .T. ) ;
#44517=VERTEX_POINT ( 'NONE', #39746 ) ;
#44519=CARTESIAN_POINT ( 'NONE',  ( 2.499999999999998668, 11.79166666939785202, -4.330127018922193649 ) ) ;
#44526=CARTESIAN_POINT ( 'NONE',  ( 1.339745962155612702, -86.29465819873851729, -5.000000000000000000 ) ) ;
#44529=AXIS2_PLACEMENT_3D ( 'NONE', #20982, #50563, #54755 ) ;
#44532=CARTESIAN_POINT ( 'NONE',  ( 4.458734125000001214, 16.10416666803225993, 2.574251347313718519 ) ) ;
#44534=ORIENTED_EDGE ( 'NONE', *, *, #30204, .T. ) ;
#44537=CARTESIAN_POINT ( 'NONE',  ( 0.000000000000000000, -120.0000000000000000, 0.000000000000000000 ) ) ;
#44538=CARTESIAN_POINT ( 'NONE',  ( 1.339745962155612702, -39.29465819873851729, -5.000000000000000000 ) ) ;
#44540=CARTESIAN_POINT ( 'NONE',  ( 4.458734124999998549, -66.72916666530106511, -2.574251347313721627 ) ) ;
#44542=CARTESIAN_POINT ( 'NONE',  ( 2.229367062499998831, 18.35416666803225993, -3.861377020970580887 ) ) ;
#44543=CARTESIAN_POINT ( 'NONE',  ( -4.999999999999998224, 18.08333333333333215, 2.886751345948131764 ) ) ;
#44544=CARTESIAN_POINT ( 'NONE',  ( 9.457646018065525792E-16, -50.31249999863440792, 5.148502694627439702 ) ) ;
#44545=CARTESIAN_POINT ( 'NONE',  ( -5.000000000000000000, -11.87499999726881761, 0.000000000000000000 ) ) ;
#44547=CARTESIAN_POINT ( 'NONE',  ( -6.972266317189433020E-16, 18.87500000273118772, -5.000000000000000000 ) ) ;
#44548=DIRECTION ( 'NONE',  ( -0.000000000000000000, 1.000000000000000000, -0.000000000000000000 ) ) ;
#44549=CARTESIAN_POINT ( 'NONE',  ( 4.458734124999999437, -109.8124999986343937, -5.460374474430324690E-16 ) ) ;
#44550=CARTESIAN_POINT ( 'NONE',  ( 4.458734124999999437, -14.06249999863440436, -5.460374474430324690E-16 ) ) ;
#44551=ORIENTED_EDGE ( 'NONE', *, *, #22300, .F. ) ;
#44552=CARTESIAN_POINT ( 'NONE',  ( -4.999999999999998224, -46.79166666393547303, 2.886751345948131764 ) ) ;
#44553=CARTESIAN_POINT ( 'NONE',  ( -2.229367062500000163, -104.4791666653010651, -3.861377020970580443 ) ) ;
#44555=CARTESIAN_POINT ( 'NONE',  ( -2.229367062499996610, -98.39583333196773651, 3.861377020970582219 ) ) ;
#44556=DIRECTION ( 'NONE',  ( 0.000000000000000000, 0.000000000000000000, 1.000000000000000000 ) ) ;
#44557=CARTESIAN_POINT ( 'NONE',  ( 2.499999999999998668, -55.20833333060214443, -4.330127018922193649 ) ) ;
#44558=CARTESIAN_POINT ( 'NONE',  ( -5.000000000000000000, 19.04166666939784847, -2.886751345948128211 ) ) ;
#44561=CARTESIAN_POINT ( 'NONE',  ( 9.457646018065525792E-16, -18.06249999863440792, 5.148502694627439702 ) ) ;
#44562=CARTESIAN_POINT ( 'NONE',  ( -4.458734124999999437, 5.354166668032262599, -2.574251347313719407 ) ) ;
#44563=CARTESIAN_POINT ( 'NONE',  ( 2.229367062500001939, -64.22916666530106511, 3.861377020970579999 ) ) ;
#44568=CARTESIAN_POINT ( 'NONE',  ( 2.499999999999998668, -4.333333333333334814, -4.330127018922193649 ) ) ;
#44569=VERTEX_POINT ( 'NONE', #7905 ) ;
#44571=( BOUNDED_CURVE ( )  B_SPLINE_CURVE ( 2, ( #55002, #58556, #24142, #24454, #24776, #997, #14794, #4516, #15452 ),
 .UNSPECIFIED., .F., .F. ) 
 B_SPLINE_CURVE_WITH_KNOTS ( ( 3, 2, 2, 2, 3 ),
 ( 0.1767857142857142960, 0.1773809523809523891, 0.1785714285714285754, 0.1797619047619047616, 0.1803571428571428548 ),
 .UNSPECIFIED. ) 
 CURVE ( )  GEOMETRIC_REPRESENTATION_ITEM ( )  RATIONAL_B_SPLINE_CURVE ( ( 0.9330127018922194093, 0.9330127018922194093, 1.000000000000000000, 0.8660254037844387076, 1.000000000000000000, 0.8660254037844387076, 1.000000000000000000, 0.9330127018922194093, 0.9330127018922194093 ) ) 
 REPRESENTATION_ITEM ( '' )  );
#44572=DIRECTION ( 'NONE',  ( -0.000000000000000000, 1.000000000000000000, -0.000000000000000000 ) ) ;
#44573=DIRECTION ( 'NONE',  ( -0.000000000000000000, 1.000000000000000000, -0.000000000000000000 ) ) ;
#44575=CARTESIAN_POINT ( 'NONE',  ( 9.457646018065525792E-16, -93.06249999863440792, 5.148502694627439702 ) ) ;
#44576=CARTESIAN_POINT ( 'NONE',  ( -2.229367062499996610, 21.60416666803226349, 3.861377020970582219 ) ) ;
#44579=CARTESIAN_POINT ( 'NONE',  ( 2.499999999999998668, -82.33333333333332860, -4.330127018922193649 ) ) ;
#44583=CARTESIAN_POINT ( 'NONE',  ( -3.535250795749689387E-16, -73.25000000000000000, -5.773502691896257311 ) ) ;
#44585=EDGE_LOOP ( 'NONE', ( #48465, #29176, #47012 ) ) ;
#44586=CARTESIAN_POINT ( 'NONE',  ( 1.339745962155612702, -80.16965819600733312, -5.000000000000000000 ) ) ;
#44598=CARTESIAN_POINT ( 'NONE',  ( -3.152548672688508926E-16, -63.81249999863440792, -5.148502694627439702 ) ) ;
#44601=ORIENTED_EDGE ( 'NONE', *, *, #32342, .F. ) ;
#44608=CARTESIAN_POINT ( 'NONE',  ( 2.229367062500001939, -105.2291666653010651, 3.861377020970579999 ) ) ;
#44610=EDGE_LOOP ( 'NONE', ( #13357, #31456, #38310, #4430 ) ) ;
#44614=CARTESIAN_POINT ( 'NONE',  ( -4.458734124999999437, -46.31249999863440792, 0.000000000000000000 ) ) ;
#44617=CARTESIAN_POINT ( 'NONE',  ( -2.229367062499996610, -49.14583333196772941, 3.861377020970582219 ) ) ;
#44619=CARTESIAN_POINT ( 'NONE',  ( 2.229367062500001939, -11.97916666530107044, 3.861377020970579999 ) ) ;
#44620=CARTESIAN_POINT ( 'NONE',  ( -2.499999999999996447, -99.83333333333332860, 4.330127018922195425 ) ) ;
#44621=VECTOR ( 'NONE', #38278, 1000.000000000000000 ) ;
#44623=CARTESIAN_POINT ( 'NONE',  ( -3.152548672688508926E-16, -31.81249999863440792, -5.148502694627439702 ) ) ;
#44624=CARTESIAN_POINT ( 'NONE',  ( 5.000000000000000888, 4.541666669397852019, 2.886751345948126879 ) ) ;
#44625=CARTESIAN_POINT ( 'NONE',  ( 2.500000000000002220, -50.66666666666666430, 4.330127018922192761 ) ) ;
#44630=LINE ( 'NONE', #15374, #55207 ) ;
#44631=CARTESIAN_POINT ( 'NONE',  ( 2.229367062499998831, 0.1041666680322607397, -3.861377020970580887 ) ) ;
#44632=EDGE_LOOP ( 'NONE', ( #41748, #23557, #34972, #59786 ) ) ;
#44633=CARTESIAN_POINT ( 'NONE',  ( 5.000000000000000888, 16.54166666939785202, 2.886751345948126879 ) ) ;
#44634=CARTESIAN_POINT ( 'NONE',  ( 1.975475456537005874E-15, -57.74999999999999289, 5.000000000000000000 ) ) ;
#44635=CARTESIAN_POINT ( 'NONE',  ( 5.000000000000000888, -94.58333333333332860, 2.886751345948126879 ) ) ;
#44636=CARTESIAN_POINT ( 'NONE',  ( 2.229367062499998831, -36.64583333196773651, -3.861377020970580887 ) ) ;
#44637=CARTESIAN_POINT ( 'NONE',  ( -6.972266317189433020E-16, -71.25000000000000000, -5.000000000000000000 ) ) ;
#44638=CARTESIAN_POINT ( 'NONE',  ( -4.458734124999998549, -83.47916666530107932, 2.574251347313722516 ) ) ;
#44642=CARTESIAN_POINT ( 'NONE',  ( 2.229367062500001939, -3.979166665301070438, 3.861377020970579999 ) ) ;
#44643=CARTESIAN_POINT ( 'NONE',  ( -3.152548672688508926E-16, 22.18750000136559564, -5.148502694627439702 ) ) ;
#44644=CARTESIAN_POINT ( 'NONE',  ( 4.458734124999999437, -41.06249999863440081, -5.460374474430324690E-16 ) ) ;
#44649=CARTESIAN_POINT ( 'NONE',  ( 9.457646018065525792E-16, -73.06249999863440792, 5.148502694627439702 ) ) ;
#44650=CARTESIAN_POINT ( 'NONE',  ( 5.000000000000000888, -107.4583333306021302, 2.886751345948126879 ) ) ;
#44651=( BOUNDED_CURVE ( )  B_SPLINE_CURVE ( 2, ( #58546, #47085, #43423, #17175, #36800, #22328, #41929, #6112, #24764 ),
 .UNSPECIFIED., .F., .F. ) 
 B_SPLINE_CURVE_WITH_KNOTS ( ( 3, 2, 2, 2, 3 ),
 ( 0.01250000000000000069, 0.01309523809523809555, 0.01428571428571428527, 0.01547619047619047672, 0.01607142857142857331 ),
 .UNSPECIFIED. ) 
 CURVE ( )  GEOMETRIC_REPRESENTATION_ITEM ( )  RATIONAL_B_SPLINE_CURVE ( ( 0.9330127018922192983, 0.9330127018922194093, 1.000000000000000000, 0.8660254037844387076, 1.000000000000000000, 0.8660254037844387076, 1.000000000000000000, 0.9330127018922191873, 0.9330127018922194093 ) ) 
 REPRESENTATION_ITEM ( '' )  );
#44654=DIRECTION ( 'NONE',  ( -0.000000000000000000, 1.000000000000000000, -0.000000000000000000 ) ) ;
#44656=CARTESIAN_POINT ( 'NONE',  ( 2.500000000000002220, -57.66666666666667140, 4.330127018922192761 ) ) ;
#44658=ORIENTED_EDGE ( 'NONE', *, *, #33062, .T. ) ;
#44659=LINE ( 'NONE', #621, #1681 ) ;
#44660=ADVANCED_FACE ( 'NONE', ( #27510 ), #31375, .T. ) ;
#44672=ORIENTED_EDGE ( 'NONE', *, *, #7213, .F. ) ;
#44676=CARTESIAN_POINT ( 'NONE',  ( 4.458734124999998549, -45.97916666530106511, -2.574251347313721627 ) ) ;
#44679=LINE ( 'NONE', #50148, #7695 ) ;
#44683=CARTESIAN_POINT ( 'NONE',  ( 1.975475456537005874E-15, -110.6249999972688158, 5.000000000000000000 ) ) ;
#44685=CARTESIAN_POINT ( 'NONE',  ( -4.458734124999999437, -89.64583333196773651, -2.574251347313719407 ) ) ;
#44688=CARTESIAN_POINT ( 'NONE',  ( 1.975475456537005874E-15, -19.62499999726881228, 5.000000000000000000 ) ) ;
#44693=CARTESIAN_POINT ( 'NONE',  ( -4.458734124999999437, 4.687500001365595637, 0.000000000000000000 ) ) ;
#44695=CARTESIAN_POINT ( 'NONE',  ( -3.152548672688508926E-16, -19.81249999863440436, -5.148502694627439702 ) ) ;
#44696=CARTESIAN_POINT ( 'NONE',  ( -4.999999999999998224, -100.7916666639354588, 2.886751345948131764 ) ) ;
#44699=CARTESIAN_POINT ( 'NONE',  ( 4.458734124999998549, 22.02083333469892779, -2.574251347313721627 ) ) ;
#44701=CARTESIAN_POINT ( 'NONE',  ( -2.229367062500000163, -95.47916666530107932, -3.861377020970580443 ) ) ;
#44702=CARTESIAN_POINT ( 'NONE',  ( -4.999999999999998224, -18.79166666393547658, 2.886751345948131764 ) ) ;
#44704=CARTESIAN_POINT ( 'NONE',  ( -4.458734124999999437, -15.39583333196773474, -2.574251347313719407 ) ) ;
#44705=EDGE_CURVE ( 'NONE', #58314, #62422, #41346, .T. ) ;
#44710=CARTESIAN_POINT ( 'NONE',  ( -4.999999999999999112, -38.79166666393548013, 2.886751345948131764 ) ) ;
#44712=CARTESIAN_POINT ( 'NONE',  ( 4.458734124999999437, 11.18750000136559386, -5.460374474430324690E-16 ) ) ;
#44714=CARTESIAN_POINT ( 'NONE',  ( -4.999999999999998224, -47.79166666393547303, 2.886751345948131764 ) ) ;
#44716=CARTESIAN_POINT ( 'NONE',  ( 2.229367062500001939, -60.97916666530106511, 3.861377020970579999 ) ) ;
#44717=EDGE_LOOP ( 'NONE', ( #57135, #13006, #37924, #48168 ) ) ;
#44719=( BOUNDED_CURVE ( )  B_SPLINE_CURVE ( 2, ( #48608, #4547, #60825, #16750, #6154, #10642, #26398, #2295, #26722 ),
 .UNSPECIFIED., .F., .F. ) 
 B_SPLINE_CURVE_WITH_KNOTS ( ( 3, 2, 2, 2, 3 ),
 ( 0.07678571428571429047, 0.07738095238095238360, 0.07857142857142856984, 0.07976190476190475609, 0.08035714285714286309 ),
 .UNSPECIFIED. ) 
 CURVE ( )  GEOMETRIC_REPRESENTATION_ITEM ( )  RATIONAL_B_SPLINE_CURVE ( ( 0.9330127018922194093, 0.9330127018922194093, 1.000000000000000000, 0.8660254037844387076, 1.000000000000000000, 0.8660254037844387076, 1.000000000000000000, 0.9330127018922185211, 0.9330127018922192983 ) ) 
 REPRESENTATION_ITEM ( '' )  );
#44720=CARTESIAN_POINT ( 'NONE',  ( 5.000000000000000888, 5.416666666666666963, 2.886751345948126879 ) ) ;
#44723=CARTESIAN_POINT ( 'NONE',  ( -2.229367062499996610, -55.14583333196773651, 3.861377020970582219 ) ) ;
#44724=CARTESIAN_POINT ( 'NONE',  ( 2.499999999999998668, -88.20833333060214443, -4.330127018922193649 ) ) ;
#44725=CARTESIAN_POINT ( 'NONE',  ( 9.457646018065525792E-16, -35.06249999863440792, 5.148502694627439702 ) ) ;
#44729=EDGE_CURVE ( 'NONE', #59250, #16461, #38449, .T. ) ;
#44731=CARTESIAN_POINT ( 'NONE',  ( -2.499999999999996447, -42.83333333333333570, 4.330127018922195425 ) ) ;
#44733=CARTESIAN_POINT ( 'NONE',  ( 1.339745962155612702, -6.169658196007334894, -5.000000000000000000 ) ) ;
#44735=CARTESIAN_POINT ( 'NONE',  ( -2.229367062499996610, -102.1458333319677365, 3.861377020970582219 ) ) ;
#44736=CARTESIAN_POINT ( 'NONE',  ( -4.458734124999998549, 5.520833334698927786, 2.574251347313722516 ) ) ;
#44737=CARTESIAN_POINT ( 'NONE',  ( 5.000000000000000888, -59.58333333333335702, 2.886751345948126879 ) ) ;
#44741=CARTESIAN_POINT ( 'NONE',  ( 1.975475456537005874E-15, -67.74999999999998579, 5.000000000000000000 ) ) ;
#44744=VERTEX_POINT ( 'NONE', #27201 ) ;
#44746=CARTESIAN_POINT ( 'NONE',  ( -6.972266317189433020E-16, -74.12499999726878741, -5.000000000000000000 ) ) ;
#44748=CARTESIAN_POINT ( 'NONE',  ( -6.972266317189433020E-16, -101.1249999972688158, -5.000000000000000000 ) ) ;
#44751=CARTESIAN_POINT ( 'NONE',  ( 2.229367062500001939, -26.22916666530106866, 3.861377020970579999 ) ) ;
#44760=EDGE_CURVE ( 'NONE', #44442, #11139, #46819, .T. ) ;
#44763=CARTESIAN_POINT ( 'NONE',  ( 4.458734125000001214, -74.14583333196773651, 2.574251347313718519 ) ) ;
#44765=SHAPE_REPRESENTATION_RELATIONSHIP ( 'NONE' , 'NONE' ,  #3639, #23309 ) ;
#44766=ORIENTED_EDGE ( 'NONE', *, *, #27955, .T. ) ;
#44769=CARTESIAN_POINT ( 'NONE',  ( -6.972266317189433020E-16, 13.74999999999999822, -5.000000000000000000 ) ) ;
#44771=CARTESIAN_POINT ( 'NONE',  ( 2.229367062500001939, -6.229166665301072214, 3.861377020970579999 ) ) ;
#44773=FACE_OUTER_BOUND ( 'NONE', #50739, .T. ) ;
#44781=CARTESIAN_POINT ( 'NONE',  ( 4.458734124999999437, -83.81249999863439371, -5.460374474430324690E-16 ) ) ;
#44783=CARTESIAN_POINT ( 'NONE',  ( 2.229367062499998831, 1.354166668032261933, -3.861377020970580887 ) ) ;
#44786=CARTESIAN_POINT ( 'NONE',  ( 5.000000000000000000, -84.41666666666667140, -2.886751345948129988 ) ) ;
#44788=CARTESIAN_POINT ( 'NONE',  ( 2.229367062500001939, -67.22916666530106511, 3.861377020970579999 ) ) ;
#44789=CARTESIAN_POINT ( 'NONE',  ( -5.000000000000000000, -25.87499999726881583, 0.000000000000000000 ) ) ;
#44792=CARTESIAN_POINT ( 'NONE',  ( -4.999999999999998224, 23.08333333333333215, 2.886751345948131764 ) ) ;
#44793=DIRECTION ( 'NONE',  ( -0.8660254037844380415, 0.000000000000000000, 0.5000000000000009992 ) ) ;
#44794=CARTESIAN_POINT ( 'NONE',  ( -4.458734124999999437, -46.39583333196774362, -2.574251347313719407 ) ) ;
#44795=CARTESIAN_POINT ( 'NONE',  ( -4.458734124999999437, -34.64583333196772941, -2.574251347313719407 ) ) ;
#44799=CARTESIAN_POINT ( 'NONE',  ( 5.000000000000000000, 19.50000000000000000, -6.123233995736766282E-16 ) ) ;
#44802=CARTESIAN_POINT ( 'NONE',  ( 4.458734125000001214, -34.89583333196772941, 2.574251347313718519 ) ) ;
#44803=CARTESIAN_POINT ( 'NONE',  ( 5.000000000000000000, -71.29166666393547303, -2.886751345948129988 ) ) ;
#44809=CARTESIAN_POINT ( 'NONE',  ( 4.458734124999999437, -80.06249999863440792, -5.460374474430324690E-16 ) ) ;
#44813=CARTESIAN_POINT ( 'NONE',  ( -4.999999999999999112, -29.91666666666667140, 2.886751345948131764 ) ) ;
#44819=CARTESIAN_POINT ( 'NONE',  ( -5.000000000000000000, 20.04166666939785202, -2.886751345948128211 ) ) ;
#44820=CARTESIAN_POINT ( 'NONE',  ( 0.000000000000000000, -120.0000000000000000, 5.000000000000000000 ) ) ;
#44827=DIRECTION ( 'NONE',  ( -0.000000000000000000, 1.000000000000000000, -0.000000000000000000 ) ) ;
#44829=CARTESIAN_POINT ( 'NONE',  ( 1.975475456537005874E-15, -78.74999999999998579, 5.000000000000000000 ) ) ;
#44830=CARTESIAN_POINT ( 'NONE',  ( -4.458734124999998549, -21.22916666530107221, 2.574251347313722516 ) ) ;
#44843=ORIENTED_EDGE ( 'NONE', *, *, #60578, .T. ) ;
#44844=AXIS2_PLACEMENT_3D ( 'NONE', #41870, #17447, #37067 ) ;
#44847=CARTESIAN_POINT ( 'NONE',  ( 5.000000000000000000, 15.58333333333332860, -2.886751345948130876 ) ) ;
#44850=ORIENTED_EDGE ( 'NONE', *, *, #19251, .F. ) ;
#44852=( BOUNDED_CURVE ( )  B_SPLINE_CURVE ( 2, ( #41161, #55980, #11893, #31513, #51156, #34636, #40733, #34971, #44934 ),
 .UNSPECIFIED., .F., .F. ) 
 B_SPLINE_CURVE_WITH_KNOTS ( ( 3, 2, 2, 2, 3 ),
 ( 0.5017857142857142794, 0.5023809523809523725, 0.5035714285714285587, 0.5047619047619047450, 0.5053571428571428381 ),
 .UNSPECIFIED. ) 
 CURVE ( )  GEOMETRIC_REPRESENTATION_ITEM ( )  RATIONAL_B_SPLINE_CURVE ( ( 0.9330127018922194093, 0.9330127018922194093, 1.000000000000000000, 0.8660254037844387076, 1.000000000000000000, 0.8660254037844387076, 1.000000000000000000, 0.9330127018922194093, 0.9330127018922194093 ) ) 
 REPRESENTATION_ITEM ( '' )  );
#44853=DIRECTION ( 'NONE',  ( -0.4999999999999948375, 0.000000000000000000, 0.8660254037844415942 ) ) ;
#44854=CARTESIAN_POINT ( 'NONE',  ( -4.458734124999999437, 12.68750000136559564, 0.000000000000000000 ) ) ;
#44860=CARTESIAN_POINT ( 'NONE',  ( -2.229367062500000163, -65.47916666530106511, -3.861377020970580443 ) ) ;
#44862=CARTESIAN_POINT ( 'NONE',  ( 2.229367062500001939, 19.02083333469892779, 3.861377020970579999 ) ) ;
#44863=CARTESIAN_POINT ( 'NONE',  ( -2.916731409357579869E-14, 18.24999999999999645, 5.000000000000000888 ) ) ;
#44867=CARTESIAN_POINT ( 'NONE',  ( -2.229367062499996610, -50.39583333196772941, 3.861377020970582219 ) ) ;
#44868=CARTESIAN_POINT ( 'NONE',  ( -5.000000000000000000, -8.958333330602146205, -2.886751345948128211 ) ) ;
#44874=CARTESIAN_POINT ( 'NONE',  ( -4.458734124999999437, -14.56249999863440436, 0.000000000000000000 ) ) ;
#44878=CARTESIAN_POINT ( 'NONE',  ( -2.229367062500000163, -101.4791666653010651, -3.861377020970580443 ) ) ;
#44880=ORIENTED_EDGE ( 'NONE', *, *, #44760, .T. ) ;
#44881=CARTESIAN_POINT ( 'NONE',  ( 9.457646018065525792E-16, -95.31249999863440792, 5.148502694627439702 ) ) ;
#44883=CARTESIAN_POINT ( 'NONE',  ( 5.000000000000000000, -55.37499999726880162, -6.123233995736766282E-16 ) ) ;
#44885=CARTESIAN_POINT ( 'NONE',  ( -5.000000000000000000, 19.12500000273118772, 0.000000000000000000 ) ) ;
#44886=ADVANCED_FACE ( 'NONE', ( #11964 ), #5558, .T. ) ;
#44889=CARTESIAN_POINT ( 'NONE',  ( 9.457646018065525792E-16, -16.06249999863440436, 5.148502694627439702 ) ) ;
#44890=CARTESIAN_POINT ( 'NONE',  ( 2.229367062500001939, 7.770833334698926009, 3.861377020970579999 ) ) ;
#44892=CARTESIAN_POINT ( 'NONE',  ( -4.458734124999997661, -64.47916666530106511, 2.574251347313722516 ) ) ;
#44895=CYLINDRICAL_SURFACE ( 'NONE', #10152, 5.000000000000000000 ) ;
#44897=CARTESIAN_POINT ( 'NONE',  ( -2.499999999999996447, -9.833333333333332149, 4.330127018922195425 ) ) ;
#44900=VERTEX_POINT ( 'NONE', #3202 ) ;
#44903=CARTESIAN_POINT ( 'NONE',  ( 5.000000000000000000, -92.50000000000000000, -6.123233995736766282E-16 ) ) ;
#44904=EDGE_CURVE ( 'NONE', #27512, #38937, #29413, .T. ) ;
#44906=VECTOR ( 'NONE', #28265, 1000.000000000000000 ) ;
#44909=CARTESIAN_POINT ( 'NONE',  ( -2.500000000000000444, -89.04166666393547303, -4.330127018922193649 ) ) ;
#44910=VECTOR ( 'NONE', #5659, 1000.000000000000000 ) ;
#44913=CARTESIAN_POINT ( 'NONE',  ( -4.999999999999999112, -73.91666666666664298, 2.886751345948131764 ) ) ;
#44916=EDGE_LOOP ( 'NONE', ( #3653, #11562, #37349, #54070 ) ) ;
#44919=CYLINDRICAL_SURFACE ( 'NONE', #19364, 5.000000000000000000 ) ;
#44922=VERTEX_POINT ( 'NONE', #22179 ) ;
#44925=VERTEX_POINT ( 'NONE', #57547 ) ;
#44928=CARTESIAN_POINT ( 'NONE',  ( -4.458734124999999437, -62.64583333196774362, -2.574251347313719407 ) ) ;
#44930=CARTESIAN_POINT ( 'NONE',  ( 0.000000000000000000, -120.0000000000000000, 0.000000000000000000 ) ) ;
#44934=CARTESIAN_POINT ( 'NONE',  ( 1.975475456537005874E-15, -41.62499999726880162, 5.000000000000000000 ) ) ;
#44937=CARTESIAN_POINT ( 'NONE',  ( -2.229367062499996610, -108.3958333319677365, 3.861377020970582219 ) ) ;
#44939=ORIENTED_EDGE ( 'NONE', *, *, #40615, .F. ) ;
#44943=CARTESIAN_POINT ( 'NONE',  ( -4.458734124999999437, -45.39583333196773651, -2.574251347313719407 ) ) ;
#44947=CARTESIAN_POINT ( 'NONE',  ( 4.458734124999999437, -48.81249999863440792, -5.460374474430324690E-16 ) ) ;
#44949=CARTESIAN_POINT ( 'NONE',  ( 4.458734125000001214, -16.89583333196773651, 2.574251347313718519 ) ) ;
#44951=CARTESIAN_POINT ( 'NONE',  ( -3.535250795749689387E-16, -99.25000000000000000, -5.773502691896257311 ) ) ;
#44953=CARTESIAN_POINT ( 'NONE',  ( 4.458734124999998549, -31.97916666530107577, -2.574251347313721627 ) ) ;
#44954=CARTESIAN_POINT ( 'NONE',  ( -3.535250795749689387E-16, 8.875000002731184168, -5.773502691896257311 ) ) ;
#44955=CARTESIAN_POINT ( 'NONE',  ( 2.499999999999998668, -50.33333333333332860, -4.330127018922193649 ) ) ;
#44961=( BOUNDED_CURVE ( )  B_SPLINE_CURVE ( 2, ( #22341, #46140, #46461, #41611, #41299, #60948, #17185, #6585, #31662 ),
 .UNSPECIFIED., .F., .F. ) 
 B_SPLINE_CURVE_WITH_KNOTS ( ( 3, 2, 2, 2, 3 ),
 ( 0.3767857142857142794, 0.3773809523809523725, 0.3785714285714285587, 0.3797619047619047450, 0.3803571428571428381 ),
 .UNSPECIFIED. ) 
 CURVE ( )  GEOMETRIC_REPRESENTATION_ITEM ( )  RATIONAL_B_SPLINE_CURVE ( ( 0.9330127018922194093, 0.9330127018922194093, 1.000000000000000000, 0.8660254037844387076, 1.000000000000000000, 0.8660254037844387076, 1.000000000000000000, 0.9330127018922194093, 0.9330127018922194093 ) ) 
 REPRESENTATION_ITEM ( '' )  );
#44962=CARTESIAN_POINT ( 'NONE',  ( 9.457646018065525792E-16, -1.312499998634406140, 5.148502694627439702 ) ) ;
#44965=CARTESIAN_POINT ( 'NONE',  ( 4.458734124999999437, -89.81249999863440792, -5.460374474430324690E-16 ) ) ;
#44966=CARTESIAN_POINT ( 'NONE',  ( -4.458734124999999437, -35.31249999863440792, 0.000000000000000000 ) ) ;
#44967=CARTESIAN_POINT ( 'NONE',  ( 4.458734124999998549, -80.97916666530106511, -2.574251347313721627 ) ) ;
#44971=CARTESIAN_POINT ( 'NONE',  ( 4.458734125000000326, -0.8958333319677401763, 2.574251347313718519 ) ) ;
#44972=CARTESIAN_POINT ( 'NONE',  ( -4.458734124999998549, 19.52083333469893134, 2.574251347313722516 ) ) ;
#44973=CARTESIAN_POINT ( 'NONE',  ( -2.229367062499996610, -49.39583333196772941, 3.861377020970582219 ) ) ;
#44974=CARTESIAN_POINT ( 'NONE',  ( -6.972266317189433020E-16, -11.25000000000000178, -5.000000000000000000 ) ) ;
#44976=EDGE_CURVE ( 'NONE', #62207, #53065, #58186, .T. ) ;
#44977=VERTEX_POINT ( 'NONE', #52407 ) ;
#44980=CARTESIAN_POINT ( 'NONE',  ( 2.229367062500001939, -73.97916666530106511, 3.861377020970579999 ) ) ;
#44981=CARTESIAN_POINT ( 'NONE',  ( 2.499999999999998668, -110.2083333306021444, -4.330127018922193649 ) ) ;
#44983=ADVANCED_FACE ( 'NONE', ( #61110 ), #17035, .T. ) ;
#44985=CARTESIAN_POINT ( 'NONE',  ( 4.458734124999999437, -109.0624999986343937, -5.460374474430324690E-16 ) ) ;
#44987=CARTESIAN_POINT ( 'NONE',  ( 1.060575238724906964E-15, -61.75000000000000000, 5.773502691896257311 ) ) ;
#44990=ORIENTED_EDGE ( 'NONE', *, *, #59869, .F. ) ;
#44992=VECTOR ( 'NONE', #38747, 1000.000000000000000 ) ;
#44996=VECTOR ( 'NONE', #51735, 1000.000000000000000 ) ;
#45000=VERTEX_POINT ( 'NONE', #46942 ) ;
#45003=VERTEX_POINT ( 'NONE', #47257 ) ;
#45007=CARTESIAN_POINT ( 'NONE',  ( 4.458734124999998549, -48.97916666530107221, -2.574251347313721627 ) ) ;
#45016=CARTESIAN_POINT ( 'NONE',  ( -2.229367062499996610, -92.39583333196773651, 3.861377020970582219 ) ) ;
#45017=LINE ( 'NONE', #30534, #31727 ) ;
#45022=CARTESIAN_POINT ( 'NONE',  ( 5.000000000000000888, -82.45833333060214443, 2.886751345948126879 ) ) ;
#45023=VERTEX_POINT ( 'NONE', #57236 ) ;
#45024=CARTESIAN_POINT ( 'NONE',  ( -4.458734124999999437, 5.604166668032262599, -2.574251347313719407 ) ) ;
#45027=CARTESIAN_POINT ( 'NONE',  ( -4.458734124999998549, -19.47916666530107221, 2.574251347313722516 ) ) ;
#45028=CARTESIAN_POINT ( 'NONE',  ( -5.000000000000000000, -101.0833333333333286, -2.886751345948128211 ) ) ;
#45031=CARTESIAN_POINT ( 'NONE',  ( 9.457646018065525792E-16, 16.68750000136559564, 5.148502694627439702 ) ) ;
#45034=CARTESIAN_POINT ( 'NONE',  ( 1.975475456537005874E-15, -71.62499999726878741, 5.000000000000000000 ) ) ;
#45035=CARTESIAN_POINT ( 'NONE',  ( -2.229367062499996610, -18.14583333196773651, 3.861377020970582219 ) ) ;
#45040=CARTESIAN_POINT ( 'NONE',  ( 2.500000000000002220, -46.54166666393547303, 4.330127018922192761 ) ) ;
#45041=CARTESIAN_POINT ( 'NONE',  ( 5.000000000000000888, -67.45833333060214443, 2.886751345948126879 ) ) ;
#45042=CARTESIAN_POINT ( 'NONE',  ( -2.229367062499996610, 13.85416666803226171, 3.861377020970582219 ) ) ;
#45044=CYLINDRICAL_SURFACE ( 'NONE', #14044, 5.000000000000000000 ) ;
#45046=CARTESIAN_POINT ( 'NONE',  ( -2.229367062500000163, -67.47916666530106511, -3.861377020970580443 ) ) ;
#45047=ORIENTED_EDGE ( 'NONE', *, *, #6119, .F. ) ;
#45049=CARTESIAN_POINT ( 'NONE',  ( -2.500000000000000444, 3.833333333333334370, -4.330127018922193649 ) ) ;
#45051=CARTESIAN_POINT ( 'NONE',  ( -1.339745962155613812, -99.08034179853029855, -5.000000000000000000 ) ) ;
#45052=CARTESIAN_POINT ( 'NONE',  ( -4.458734124999998549, -59.22916666530106511, 2.574251347313722516 ) ) ;
#45053=CARTESIAN_POINT ( 'NONE',  ( 2.499999999999998668, -90.20833333060214443, -4.330127018922193649 ) ) ;
#45054=CARTESIAN_POINT ( 'NONE',  ( -2.229367062500000163, -34.47916666530107221, -3.861377020970580443 ) ) ;
#45055=CARTESIAN_POINT ( 'NONE',  ( 1.975475456537005874E-15, -41.62499999726880162, 5.000000000000000000 ) ) ;
#45056=( BOUNDED_CURVE ( )  B_SPLINE_CURVE ( 2, ( #43127, #19313, #346, #13859, #9979, #32, #33483, #34749, #9344 ),
 .UNSPECIFIED., .F., .F. ) 
 B_SPLINE_CURVE_WITH_KNOTS ( ( 3, 2, 2, 2, 3 ),
 ( 0.9482142857142856762, 0.9488095238095237693, 0.9499999999999999556, 0.9511904761904761418, 0.9517857142857142350 ),
 .UNSPECIFIED. ) 
 CURVE ( )  GEOMETRIC_REPRESENTATION_ITEM ( )  RATIONAL_B_SPLINE_CURVE ( ( 0.9330127018922194093, 0.9330127018922194093, 1.000000000000000000, 0.8660254037844387076, 1.000000000000000000, 0.8660254037844387076, 1.000000000000000000, 0.9330127018922194093, 0.9330127018922194093 ) ) 
 REPRESENTATION_ITEM ( '' )  );
#45059=CARTESIAN_POINT ( 'NONE',  ( -4.999999999999998224, -78.79166666393547303, 2.886751345948131764 ) ) ;
#45061=CARTESIAN_POINT ( 'NONE',  ( 2.499999999999998668, -42.33333333333333570, -4.330127018922193649 ) ) ;
#45065=CARTESIAN_POINT ( 'NONE',  ( -2.229367062499996610, -105.1458333319677365, 3.861377020970582219 ) ) ;
#45066=CARTESIAN_POINT ( 'NONE',  ( -4.458734124999999437, 2.437500001365593860, 0.000000000000000000 ) ) ;
#45070=CARTESIAN_POINT ( 'NONE',  ( 6.123233995736766282E-16, -120.0000000000000000, -5.000000000000000000 ) ) ;
#45075=CARTESIAN_POINT ( 'NONE',  ( 1.975475456537005874E-15, -16.62499999726881583, 5.000000000000000000 ) ) ;
#45077=CARTESIAN_POINT ( 'NONE',  ( 1.975475456537005874E-15, -55.62499999726880873, 5.000000000000000000 ) ) ;
#45080=CARTESIAN_POINT ( 'NONE',  ( 9.457646018065525792E-16, -30.31249999863440436, 5.148502694627439702 ) ) ;
#45082=CYLINDRICAL_SURFACE ( 'NONE', #32740, 5.000000000000000000 ) ;
#45089=ORIENTED_EDGE ( 'NONE', *, *, #3576, .T. ) ;
#45091=VERTEX_POINT ( 'NONE', #23122 ) ;
#45092=CARTESIAN_POINT ( 'NONE',  ( -4.458734124999998549, -71.47916666530107932, 2.574251347313722516 ) ) ;
#45094=ORIENTED_EDGE ( 'NONE', *, *, #38212, .T. ) ;
#45095=DIRECTION ( 'NONE',  ( -0.000000000000000000, 1.000000000000000000, -0.000000000000000000 ) ) ;
#45098=CARTESIAN_POINT ( 'NONE',  ( 4.458734125000001214, -2.145833331967737845, 2.574251347313718519 ) ) ;
#45104=CARTESIAN_POINT ( 'NONE',  ( 2.499999999999998668, -47.20833333060214443, -4.330127018922193649 ) ) ;
#45108=ORIENTED_EDGE ( 'NONE', *, *, #32681, .T. ) ;
#45109=CARTESIAN_POINT ( 'NONE',  ( -4.458734124999999437, -80.31249999863440792, 0.000000000000000000 ) ) ;
#45110=CARTESIAN_POINT ( 'NONE',  ( -6.972266317189433020E-16, -75.25000000000000000, -5.000000000000000000 ) ) ;
#45111=CARTESIAN_POINT ( 'NONE',  ( 4.458734124999998549, -1.729166665301068440, -2.574251347313721627 ) ) ;
#45114=CARTESIAN_POINT ( 'NONE',  ( 2.229367062499998831, -71.89583333196773651, -3.861377020970580887 ) ) ;
#45115=CARTESIAN_POINT ( 'NONE',  ( -5.000000000000000000, -27.87499999726880873, 0.000000000000000000 ) ) ;
#45119=CARTESIAN_POINT ( 'NONE',  ( -4.458734124999999437, -43.39583333196774362, -2.574251347313719407 ) ) ;
#45120=CARTESIAN_POINT ( 'NONE',  ( -3.152548672688508926E-16, -34.81249999863440792, -5.148502694627439702 ) ) ;
#45122=FACE_OUTER_BOUND ( 'NONE', #8935, .T. ) ;
#45123=CARTESIAN_POINT ( 'NONE',  ( 5.000000000000000000, 19.58333333333333215, -2.886751345948129988 ) ) ;
#45126=VECTOR ( 'NONE', #32089, 1000.000000000000000 ) ;
#45127=CARTESIAN_POINT ( 'NONE',  ( 4.458734125000001214, -43.89583333196775072, 2.574251347313718519 ) ) ;
#45128=CARTESIAN_POINT ( 'NONE',  ( 1.060575238724906964E-15, -71.62499999726880162, 5.773502691896257311 ) ) ;
#45130=CARTESIAN_POINT ( 'NONE',  ( 5.000000000000000000, -24.37499999726881228, -6.123233995736766282E-16 ) ) ;
#45131=CARTESIAN_POINT ( 'NONE',  ( 1.975475456537005874E-15, -15.62499999726881406, 5.000000000000000000 ) ) ;
#45132=CARTESIAN_POINT ( 'NONE',  ( 4.458734125000000326, -81.14583333196773651, 2.574251347313718519 ) ) ;
#45134=CARTESIAN_POINT ( 'NONE',  ( 6.123233995736766282E-16, -120.0000000000000000, -5.000000000000000000 ) ) ;
#45136=CARTESIAN_POINT ( 'NONE',  ( -5.000000000000000000, -28.99999999999999645, 0.000000000000000000 ) ) ;
#45140=ORIENTED_EDGE ( 'NONE', *, *, #12294, .T. ) ;
#45143=CARTESIAN_POINT ( 'NONE',  ( 1.060575238724906964E-15, 24.37500000273118417, 5.773502691896257311 ) ) ;
#45144=DIRECTION ( 'NONE',  ( -0.000000000000000000, 1.000000000000000000, -0.000000000000000000 ) ) ;
#45150=CARTESIAN_POINT ( 'NONE',  ( 1.975475456537005874E-15, -89.62499999726880162, 5.000000000000000000 ) ) ;
#45151=CARTESIAN_POINT ( 'NONE',  ( -6.972266317189433020E-16, -75.12499999726880162, -5.000000000000000000 ) ) ;
#45152=CARTESIAN_POINT ( 'NONE',  ( 5.000000000000000888, -56.45833333060214443, 2.886751345948126879 ) ) ;
#45153=CARTESIAN_POINT ( 'NONE',  ( -5.000000000000000000, -79.00000000000000000, 0.000000000000000000 ) ) ;
#45154=CARTESIAN_POINT ( 'NONE',  ( 4.458734125000001214, -15.14583333196773651, 2.574251347313718519 ) ) ;
#45161=CARTESIAN_POINT ( 'NONE',  ( 0.000000000000000000, 30.00000000000000000, 5.000000000000000000 ) ) ;
#45165=CARTESIAN_POINT ( 'NONE',  ( 5.000000000000000000, 11.62500000273118594, -6.123233995736766282E-16 ) ) ;
#45167=ORIENTED_EDGE ( 'NONE', *, *, #48287, .F. ) ;
#45168=CARTESIAN_POINT ( 'NONE',  ( 5.000000000000000888, 5.416666666666666963, 2.886751345948126879 ) ) ;
#45169=ADVANCED_FACE ( 'NONE', ( #37285 ), #12832, .T. ) ;
#45170=CARTESIAN_POINT ( 'NONE',  ( 5.000000000000000000, -99.41666666666665719, -2.886751345948130876 ) ) ;
#45172=CYLINDRICAL_SURFACE ( 'NONE', #4149, 5.000000000000000000 ) ;
#45177=CARTESIAN_POINT ( 'NONE',  ( -2.229367062499996610, 12.85416666803226171, 3.861377020970582219 ) ) ;
#45180=CARTESIAN_POINT ( 'NONE',  ( 5.000000000000000888, -25.58333333333333215, 2.886751345948126879 ) ) ;
#45182=CARTESIAN_POINT ( 'NONE',  ( -2.229367062500000163, -64.47916666530106511, -3.861377020970580443 ) ) ;
#45183=CARTESIAN_POINT ( 'NONE',  ( -4.999999999999998224, -49.79166666393547303, 2.886751345948131764 ) ) ;
#45184=CARTESIAN_POINT ( 'NONE',  ( -4.458734124999998549, 18.77083333469893134, 2.574251347313722516 ) ) ;
#45187=CARTESIAN_POINT ( 'NONE',  ( 2.229367062499998831, -47.89583333196774362, -3.861377020970580887 ) ) ;
#45188=CARTESIAN_POINT ( 'NONE',  ( -2.500000000000000444, -11.04166666393547835, -4.330127018922193649 ) ) ;
#45193=CARTESIAN_POINT ( 'NONE',  ( 2.229367062499998831, -17.89583333196773651, -3.861377020970580887 ) ) ;
#45195=CARTESIAN_POINT ( 'NONE',  ( -5.000000000000000000, -46.87499999726880873, 0.000000000000000000 ) ) ;
#45196=CARTESIAN_POINT ( 'NONE',  ( -4.458734124999999437, -105.3958333319677365, -2.574251347313719407 ) ) ;
#45199=CARTESIAN_POINT ( 'NONE',  ( -4.458734124999999437, -99.56249999863440792, 0.000000000000000000 ) ) ;
#45201=CARTESIAN_POINT ( 'NONE',  ( -5.000000000000000000, -54.95833333060213732, -2.886751345948128211 ) ) ;
#45202=CARTESIAN_POINT ( 'NONE',  ( 2.499999999999998668, -62.20833333060214443, -4.330127018922193649 ) ) ;
#45205=EDGE_CURVE ( 'NONE', #44248, #13925, #18609, .T. ) ;
#45206=CARTESIAN_POINT ( 'NONE',  ( 4.458734124999998549, -24.72916666530106866, -2.574251347313721627 ) ) ;
#45207=CARTESIAN_POINT ( 'NONE',  ( 2.229367062499998831, 8.104166668032261711, -3.861377020970580887 ) ) ;
#45208=CARTESIAN_POINT ( 'NONE',  ( 4.458734124999998549, -66.97916666530106511, -2.574251347313721627 ) ) ;
#45209=CYLINDRICAL_SURFACE ( 'NONE', #34661, 5.000000000000000000 ) ;
#45213=CARTESIAN_POINT ( 'NONE',  ( 5.000000000000000000, -13.41666666666666607, -2.886751345948129988 ) ) ;
#45216=VECTOR ( 'NONE', #58242, 1000.000000000000000 ) ;
#45218=LINE ( 'NONE', #1184, #19122 ) ;
#45219=CARTESIAN_POINT ( 'NONE',  ( 2.500000000000002220, -92.66666666666665719, 4.330127018922192761 ) ) ;
#45221=AXIS2_PLACEMENT_3D ( 'NONE', #32723, #28521, #8905 ) ;
#45223=CARTESIAN_POINT ( 'NONE',  ( 5.000000000000000888, -93.58333333333332860, 2.886751345948126879 ) ) ;
#45226=CARTESIAN_POINT ( 'NONE',  ( -4.999999999999999112, -74.91666666666665719, 2.886751345948131764 ) ) ;
#45230=ORIENTED_EDGE ( 'NONE', *, *, #57397, .F. ) ;
#45231=CARTESIAN_POINT ( 'NONE',  ( 5.000000000000000888, -85.58333333333332860, 2.886751345948126879 ) ) ;
#45233=( BOUNDED_CURVE ( )  B_SPLINE_CURVE ( 2, ( #8428, #14176, #9047, #18386, #37684, #33184, #4529, #13242, #53110 ),
 .UNSPECIFIED., .F., .F. ) 
 B_SPLINE_CURVE_WITH_KNOTS ( ( 3, 2, 2, 2, 3 ),
 ( 0.5589285714285714413, 0.5595238095238095344, 0.5607142857142857206, 0.5619047619047619069, 0.5625000000000000000 ),
 .UNSPECIFIED. ) 
 CURVE ( )  GEOMETRIC_REPRESENTATION_ITEM ( )  RATIONAL_B_SPLINE_CURVE ( ( 0.9330127018922194093, 0.9330127018922194093, 1.000000000000000000, 0.8660254037844387076, 1.000000000000000000, 0.8660254037844387076, 1.000000000000000000, 0.9330127018922194093, 0.9330127018922194093 ) ) 
 REPRESENTATION_ITEM ( '' )  );
#45237=ORIENTED_EDGE ( 'NONE', *, *, #59431, .F. ) ;
#45243=CARTESIAN_POINT ( 'NONE',  ( 2.499999999999998668, -55.33333333333332860, -4.330127018922193649 ) ) ;
#45248=EDGE_CURVE ( 'NONE', #20419, #23270, #1110, .T. ) ;
#45253=CARTESIAN_POINT ( 'NONE',  ( 2.229367062499998831, 27.35416666803225993, -3.861377020970580887 ) ) ;
#45255=ORIENTED_EDGE ( 'NONE', *, *, #15869, .T. ) ;
#45260=CARTESIAN_POINT ( 'NONE',  ( -4.458734124999999437, -42.31249999863440081, 0.000000000000000000 ) ) ;
#45262=CARTESIAN_POINT ( 'NONE',  ( 4.458734125000000326, -46.89583333196773651, 2.574251347313718519 ) ) ;
#45264=CARTESIAN_POINT ( 'NONE',  ( 5.000000000000000888, 29.41666666666666785, 2.886751345948126879 ) ) ;
#45265=CARTESIAN_POINT ( 'NONE',  ( -2.229367062499996610, -18.14583333196773651, 3.861377020970582219 ) ) ;
#45266=CARTESIAN_POINT ( 'NONE',  ( -2.499999999999996447, -103.8333333333333286, 4.330127018922195425 ) ) ;
#45268=CARTESIAN_POINT ( 'NONE',  ( -4.458734124999999437, -35.56249999863440792, 0.000000000000000000 ) ) ;
#45269=CARTESIAN_POINT ( 'NONE',  ( -3.535250795749689387E-16, 5.875000002731185056, -5.773502691896257311 ) ) ;
#45275=CARTESIAN_POINT ( 'NONE',  ( 4.458734125000000326, -2.145833331967737845, 2.574251347313718519 ) ) ;
#45276=VERTEX_POINT ( 'NONE', #43048 ) ;
#45279=CARTESIAN_POINT ( 'NONE',  ( 9.457646018065525792E-16, -86.06249999863439371, 5.148502694627439702 ) ) ;
#45280=CARTESIAN_POINT ( 'NONE',  ( -2.229367062500000163, -36.47916666530107221, -3.861377020970580443 ) ) ;
#45281=CARTESIAN_POINT ( 'NONE',  ( 5.000000000000000000, -95.41666666666667140, -2.886751345948130876 ) ) ;
#45282=CARTESIAN_POINT ( 'NONE',  ( 4.458734124999999437, -84.06249999863439371, -5.460374474430324690E-16 ) ) ;
#45286=CARTESIAN_POINT ( 'NONE',  ( 9.457646018065525792E-16, -8.062499998634404363, 5.148502694627439702 ) ) ;
#45287=CARTESIAN_POINT ( 'NONE',  ( -2.229367062499996610, 22.60416666803225993, 3.861377020970582219 ) ) ;
#45288=CARTESIAN_POINT ( 'NONE',  ( -2.229367062500000163, -48.72916666530106511, -3.861377020970580443 ) ) ;
#45290=CARTESIAN_POINT ( 'NONE',  ( 1.339745962155615144, -15.70534180126148271, 4.999999999999999112 ) ) ;
#45293=VERTEX_POINT ( 'NONE', #49134 ) ;
#45296=CARTESIAN_POINT ( 'NONE',  ( -4.458734124999998549, -77.22916666530106511, 2.574251347313722516 ) ) ;
#45297=CARTESIAN_POINT ( 'NONE',  ( 2.500000000000002220, -108.5416666639354730, 4.330127018922192761 ) ) ;
#45299=CARTESIAN_POINT ( 'NONE',  ( -2.500000000000000444, -65.16666666666667140, -4.330127018922193649 ) ) ;
#45302=CARTESIAN_POINT ( 'NONE',  ( 5.000000000000000888, -57.58333333333334281, 2.886751345948126879 ) ) ;
#45303=CARTESIAN_POINT ( 'NONE',  ( 5.000000000000000000, -36.29166666393547303, -2.886751345948130876 ) ) ;
#45305=VERTEX_POINT ( 'NONE', #5077 ) ;
#45307=CARTESIAN_POINT ( 'NONE',  ( 2.499999999999998668, -52.20833333060213732, -4.330127018922193649 ) ) ;
#45308=LINE ( 'NONE', #21187, #29726 ) ;
#45311=VECTOR ( 'NONE', #62918, 1000.000000000000000 ) ;
#45317=CARTESIAN_POINT ( 'NONE',  ( 1.975475456537005874E-15, -35.62499999726880162, 5.000000000000000000 ) ) ;
#45321=( BOUNDED_CURVE ( )  B_SPLINE_CURVE ( 2, ( #44090, #4864, #33509, #42837, #38629, #62479, #43147, #32879, #18706 ),
 .UNSPECIFIED., .F., .F. ) 
 B_SPLINE_CURVE_WITH_KNOTS ( ( 3, 2, 2, 2, 3 ),
 ( 0.3339285714285714080, 0.3345238095238095011, 0.3357142857142856873, 0.3369047619047619291, 0.3375000000000000222 ),
 .UNSPECIFIED. ) 
 CURVE ( )  GEOMETRIC_REPRESENTATION_ITEM ( )  RATIONAL_B_SPLINE_CURVE ( ( 0.9330127018922194093, 0.9330127018922194093, 1.000000000000000000, 0.8660254037844387076, 1.000000000000000000, 0.8660254037844387076, 1.000000000000000000, 0.9330127018922194093, 0.9330127018922194093 ) ) 
 REPRESENTATION_ITEM ( '' )  );
#45325=CARTESIAN_POINT ( 'NONE',  ( -4.458734124999999437, -47.64583333196775072, -2.574251347313719407 ) ) ;
#45326=CARTESIAN_POINT ( 'NONE',  ( 5.000000000000000000, -68.37499999726881583, -6.123233995736766282E-16 ) ) ;
#45328=CARTESIAN_POINT ( 'NONE',  ( -2.499999999999996447, -56.70833333060214443, 4.330127018922195425 ) ) ;
#45334=CARTESIAN_POINT ( 'NONE',  ( 9.457646018065525792E-16, -96.31249999863439371, 5.148502694627439702 ) ) ;
#45342=EDGE_CURVE ( 'NONE', #45000, #6575, #10094, .T. ) ;
#45345=CARTESIAN_POINT ( 'NONE',  ( -4.458734124999999437, -4.312499998634401699, 0.000000000000000000 ) ) ;
#45346=ADVANCED_FACE ( 'NONE', ( #39794 ), #29826, .T. ) ;
#45347=CARTESIAN_POINT ( 'NONE',  ( 5.000000000000000000, -50.29166666393548013, -2.886751345948130876 ) ) ;
#45348=CARTESIAN_POINT ( 'NONE',  ( 4.458734124999998549, -16.97916666530107221, -2.574251347313721627 ) ) ;
#45349=DIRECTION ( 'NONE',  ( 0.000000000000000000, 0.000000000000000000, 1.000000000000000000 ) ) ;
#45353=CARTESIAN_POINT ( 'NONE',  ( -3.152548672688508926E-16, 17.18750000136559564, -5.148502694627439702 ) ) ;
#45356=CARTESIAN_POINT ( 'NONE',  ( -5.000000000000000000, -13.08333333333333570, -2.886751345948128211 ) ) ;
#45357=CARTESIAN_POINT ( 'NONE',  ( -2.229367062500000163, -20.47916666530107221, -3.861377020970580443 ) ) ;
#45361=CARTESIAN_POINT ( 'NONE',  ( -2.500000000000000444, -45.04166666393547303, -4.330127018922193649 ) ) ;
#45362=CARTESIAN_POINT ( 'NONE',  ( -1.336351044127974539E-14, 21.37500000273118417, 5.000000000000000000 ) ) ;
#45363=CARTESIAN_POINT ( 'NONE',  ( -4.458734124999999437, 13.68750000136559386, 0.000000000000000000 ) ) ;
#45364=CARTESIAN_POINT ( 'NONE',  ( -5.000000000000000000, -8.958333330602144429, -2.886751345948128211 ) ) ;
#45367=CARTESIAN_POINT ( 'NONE',  ( -4.458734124999999437, -68.31249999863439371, 0.000000000000000000 ) ) ;
#45370=CARTESIAN_POINT ( 'NONE',  ( 2.500000000000002220, 2.333333333333333037, 4.330127018922192761 ) ) ;
#45373=CARTESIAN_POINT ( 'NONE',  ( -4.458734124999999437, -60.31249999863440081, 0.000000000000000000 ) ) ;
#45374=CARTESIAN_POINT ( 'NONE',  ( 5.000000000000000000, -93.37499999726881583, -6.123233995736766282E-16 ) ) ;
#45375=CARTESIAN_POINT ( 'NONE',  ( 4.458734125000000326, -35.89583333196773651, 2.574251347313718519 ) ) ;
#45376=CARTESIAN_POINT ( 'NONE',  ( -1.339745962155613812, -42.08034179853029144, -5.000000000000000000 ) ) ;
#45378=CARTESIAN_POINT ( 'NONE',  ( 1.975475456537005874E-15, -107.6249999972687874, 5.000000000000000000 ) ) ;
#45381=CARTESIAN_POINT ( 'NONE',  ( -2.500000000000000444, -42.16666666666667140, -4.330127018922193649 ) ) ;
#45383=ORIENTED_EDGE ( 'NONE', *, *, #24061, .F. ) ;
#45384=CARTESIAN_POINT ( 'NONE',  ( 9.457646018065525792E-16, -106.0624999986343795, 5.148502694627439702 ) ) ;
#45385=CARTESIAN_POINT ( 'NONE',  ( 2.229367062499998831, 0.1041666680322607397, -3.861377020970580887 ) ) ;
#45393=ORIENTED_EDGE ( 'NONE', *, *, #53074, .T. ) ;
#45394=CARTESIAN_POINT ( 'NONE',  ( 1.339745962155612702, -33.29465819873851729, -5.000000000000000000 ) ) ;
#45398=CARTESIAN_POINT ( 'NONE',  ( 5.000000000000000000, -101.2916666639354730, -2.886751345948130876 ) ) ;
#45400=CARTESIAN_POINT ( 'NONE',  ( -3.152548672688508926E-16, -32.81249999863440792, -5.148502694627439702 ) ) ;
#45401=LINE ( 'NONE', #50224, #55342 ) ;
#45408=CARTESIAN_POINT ( 'NONE',  ( -5.000000000000000000, 29.56250000136559208, 0.000000000000000000 ) ) ;
#45410=CARTESIAN_POINT ( 'NONE',  ( 2.229367062500001939, -77.22916666530106511, 3.861377020970579999 ) ) ;
#45411=CARTESIAN_POINT ( 'NONE',  ( -5.000000000000000000, 13.04166666939785379, -2.886751345948128211 ) ) ;
#45413=CARTESIAN_POINT ( 'NONE',  ( 5.000000000000000000, -16.41666666666667140, -2.886751345948130876 ) ) ;
#45415=CARTESIAN_POINT ( 'NONE',  ( -5.000000000000000000, 7.916666666666665186, -2.886751345948128211 ) ) ;
#45417=CARTESIAN_POINT ( 'NONE',  ( 2.229367062500001939, -4.229166665301070438, 3.861377020970579999 ) ) ;
#45424=DIRECTION ( 'NONE',  ( 0.000000000000000000, 0.000000000000000000, 1.000000000000000000 ) ) ;
#45426=CARTESIAN_POINT ( 'NONE',  ( 1.975475456537005874E-15, -75.62499999726880162, 5.000000000000000000 ) ) ;
#45428=CARTESIAN_POINT ( 'NONE',  ( -2.229367062500000163, -81.47916666530106511, -3.861377020970580443 ) ) ;
#45430=CARTESIAN_POINT ( 'NONE',  ( -4.458734124999998549, -3.229166665301069994, 2.574251347313722516 ) ) ;
#45434=CARTESIAN_POINT ( 'NONE',  ( -4.458734124999998549, -72.47916666530107932, 2.574251347313722516 ) ) ;
#45435=CARTESIAN_POINT ( 'NONE',  ( -2.499999999999996447, -29.70833333060215153, 4.330127018922195425 ) ) ;
#45437=CARTESIAN_POINT ( 'NONE',  ( -1.339745962155613812, -41.20534180126147561, -5.000000000000000000 ) ) ;
#45438=CARTESIAN_POINT ( 'NONE',  ( -1.339745962155618253, 23.20534180126147916, 4.999999999999996447 ) ) ;
#45440=CARTESIAN_POINT ( 'NONE',  ( 4.458734125000001214, -52.89583333196772941, 2.574251347313718519 ) ) ;
#45441=CARTESIAN_POINT ( 'NONE',  ( -3.152548672688508926E-16, -31.81249999863440436, -5.148502694627439702 ) ) ;
#45444=CARTESIAN_POINT ( 'NONE',  ( -5.000000000000000000, 20.91666666666666785, -2.886751345948128211 ) ) ;
#45447=CARTESIAN_POINT ( 'NONE',  ( 4.458734124999998549, -42.72916666530107221, -2.574251347313721627 ) ) ;
#45448=CARTESIAN_POINT ( 'NONE',  ( 2.500000000000002220, -78.54166666393547303, 4.330127018922192761 ) ) ;
#45452=CARTESIAN_POINT ( 'NONE',  ( -4.458734124999997661, -79.47916666530106511, 2.574251347313722516 ) ) ;
#45456=CARTESIAN_POINT ( 'NONE',  ( -2.499999999999996447, -27.83333333333333570, 4.330127018922195425 ) ) ;
#45458=ORIENTED_EDGE ( 'NONE', *, *, #61814, .T. ) ;
#45462=CARTESIAN_POINT ( 'NONE',  ( 5.000000000000000000, 20.70833333606451632, -2.886751345948129988 ) ) ;
#45468=CARTESIAN_POINT ( 'NONE',  ( -2.499999999999996447, -109.8333333333333428, 4.330127018922195425 ) ) ;
#45470=CARTESIAN_POINT ( 'NONE',  ( 5.000000000000000000, -11.29166666393547835, -2.886751345948130876 ) ) ;
#45474=CARTESIAN_POINT ( 'NONE',  ( -4.458734124999998549, -13.47916666530107221, 2.574251347313722516 ) ) ;
#45481=CARTESIAN_POINT ( 'NONE',  ( -2.499999999999996447, 25.29166666939785202, 4.330127018922195425 ) ) ;
#45483=ORIENTED_EDGE ( 'NONE', *, *, #59774, .F. ) ;
#45485=CARTESIAN_POINT ( 'NONE',  ( 1.339745962155612702, -58.29465819873852439, -5.000000000000000000 ) ) ;
#45489=CARTESIAN_POINT ( 'NONE',  ( -5.000000000000000000, -7.958333330602144429, -2.886751345948128211 ) ) ;
#45491=CARTESIAN_POINT ( 'NONE',  ( 0.000000000000000000, -120.0000000000000000, 5.000000000000000000 ) ) ;
#45493=ORIENTED_EDGE ( 'NONE', *, *, #8402, .F. ) ;
#45495=CARTESIAN_POINT ( 'NONE',  ( 2.229367062500001939, 15.02083333469892779, 3.861377020970579999 ) ) ;
#45501=CARTESIAN_POINT ( 'NONE',  ( -3.152548672688508926E-16, -64.56249999863440792, -5.148502694627439702 ) ) ;
#45503=CARTESIAN_POINT ( 'NONE',  ( 4.458734124999999437, 11.18750000136559386, -5.460374474430324690E-16 ) ) ;
#45505=CARTESIAN_POINT ( 'NONE',  ( -6.972266317189433020E-16, -99.24999999999998579, -5.000000000000000000 ) ) ;
#45506=CARTESIAN_POINT ( 'NONE',  ( -3.152548672688508926E-16, -53.81249999863439371, -5.148502694627439702 ) ) ;
#45507=CARTESIAN_POINT ( 'NONE',  ( -5.000000000000000000, -14.95833333060214265, -2.886751345948128211 ) ) ;
#45508=CARTESIAN_POINT ( 'NONE',  ( -1.339745962155613812, -109.2053418012614543, -5.000000000000000000 ) ) ;
#45513=CARTESIAN_POINT ( 'NONE',  ( -2.229367062500000163, -14.72916666530107221, -3.861377020970580443 ) ) ;
#45516=CARTESIAN_POINT ( 'NONE',  ( -3.152548672688508926E-16, -101.5624999986344221, -5.148502694627439702 ) ) ;
#45518=VERTEX_POINT ( 'NONE', #15686 ) ;
#45519=CARTESIAN_POINT ( 'NONE',  ( -2.229367062499996610, -102.3958333319677365, 3.861377020970582219 ) ) ;
#45521=CARTESIAN_POINT ( 'NONE',  ( -2.229367062500000163, -25.47916666530106866, -3.861377020970580443 ) ) ;
#45522=CARTESIAN_POINT ( 'NONE',  ( -3.535250795749689387E-16, -57.12499999726880873, -5.773502691896257311 ) ) ;
#45525=CARTESIAN_POINT ( 'NONE',  ( -4.458734124999997661, -22.22916666530107221, 2.574251347313722516 ) ) ;
#45526=CARTESIAN_POINT ( 'NONE',  ( 4.458734124999999437, -65.06249999863440792, -5.460374474430324690E-16 ) ) ;
#45527=CARTESIAN_POINT ( 'NONE',  ( 2.500000000000002220, 8.333333333333332149, 4.330127018922192761 ) ) ;
#45531=CARTESIAN_POINT ( 'NONE',  ( -2.499999999999996447, -8.833333333333332149, 4.330127018922195425 ) ) ;
#45533=ORIENTED_EDGE ( 'NONE', *, *, #32238, .F. ) ;
#45541=EDGE_CURVE ( 'NONE', #17564, #14134, #6676, .T. ) ;
#45543=CARTESIAN_POINT ( 'NONE',  ( -5.000000000000000000, 26.00000000000000000, 0.000000000000000000 ) ) ;
#45545=CARTESIAN_POINT ( 'NONE',  ( -2.500000000000000444, -78.16666666666665719, -4.330127018922193649 ) ) ;
#45550=CARTESIAN_POINT ( 'NONE',  ( -5.000000000000000000, -51.08333333333332860, -2.886751345948128211 ) ) ;
#45553=EDGE_CURVE ( 'NONE', #3800, #11847, #53409, .T. ) ;
#45555=ORIENTED_EDGE ( 'NONE', *, *, #23271, .T. ) ;
#45566=ORIENTED_EDGE ( 'NONE', *, *, #22028, .F. ) ;
#45568=ADVANCED_FACE ( 'NONE', ( #10220 ), #54282, .F. ) ;
#45569=CARTESIAN_POINT ( 'NONE',  ( -4.458734124999998549, -77.22916666530106511, 2.574251347313722516 ) ) ;
#45570=CARTESIAN_POINT ( 'NONE',  ( 2.229367062500001939, -109.2291666653010651, 3.861377020970579999 ) ) ;
#45577=CARTESIAN_POINT ( 'NONE',  ( 4.458734124999998549, -42.72916666530107932, -2.574251347313721627 ) ) ;
#45580=CARTESIAN_POINT ( 'NONE',  ( 4.458734125000000326, -49.89583333196772941, 2.574251347313718519 ) ) ;
#45582=CARTESIAN_POINT ( 'NONE',  ( -4.458734124999999437, 27.60416666803226349, -2.574251347313719407 ) ) ;
#45583=CARTESIAN_POINT ( 'NONE',  ( 4.458734124999999437, -17.81249999863440792, -5.460374474430324690E-16 ) ) ;
#45584=CARTESIAN_POINT ( 'NONE',  ( 1.060575238724906964E-15, -99.75000000000001421, 5.773502691896257311 ) ) ;
#45586=CARTESIAN_POINT ( 'NONE',  ( -3.152548672688508926E-16, -39.81249999863440081, -5.148502694627439702 ) ) ;
#45587=CARTESIAN_POINT ( 'NONE',  ( -5.000000000000000000, 6.125000002731185056, 0.000000000000000000 ) ) ;
#45588=CARTESIAN_POINT ( 'NONE',  ( -6.972266317189433020E-16, -7.124999997268814056, -5.000000000000000000 ) ) ;
#45593=CARTESIAN_POINT ( 'NONE',  ( -2.229367062500000163, -2.729166665301069550, -3.861377020970580443 ) ) ;
#45594=ORIENTED_EDGE ( 'NONE', *, *, #49892, .F. ) ;
#45595=CARTESIAN_POINT ( 'NONE',  ( -1.336351044127974539E-14, 24.37500000273118417, 5.000000000000000000 ) ) ;
#45597=CARTESIAN_POINT ( 'NONE',  ( 2.229367062500001939, -85.97916666530107932, 3.861377020970579999 ) ) ;
#45598=CARTESIAN_POINT ( 'NONE',  ( -4.458734124999999437, -35.39583333196773651, -2.574251347313719407 ) ) ;
#45600=CARTESIAN_POINT ( 'NONE',  ( -4.458734124999998549, -82.47916666530106511, 2.574251347313722516 ) ) ;
#45608=CARTESIAN_POINT ( 'NONE',  ( -2.229367062499996610, -10.14583333196773829, 3.861377020970582219 ) ) ;
#45609=CARTESIAN_POINT ( 'NONE',  ( -4.458734124999999437, 24.35416666803225993, -2.574251347313719407 ) ) ;
#45610=CARTESIAN_POINT ( 'NONE',  ( -4.458734124999999437, -47.64583333196775072, -2.574251347313719407 ) ) ;
#45614=DIRECTION ( 'NONE',  ( 0.000000000000000000, 0.000000000000000000, 1.000000000000000000 ) ) ;
#45615=ORIENTED_EDGE ( 'NONE', *, *, #3249, .F. ) ;
#45618=CARTESIAN_POINT ( 'NONE',  ( 4.458734125000001214, -76.89583333196775072, 2.574251347313718519 ) ) ;
#45619=CARTESIAN_POINT ( 'NONE',  ( 2.499999999999998668, -108.2083333306021444, -4.330127018922193649 ) ) ;
#45620=( BOUNDED_CURVE ( )  B_SPLINE_CURVE ( 2, ( #11391, #16545, #11076, #44847, #49993, #810, #31011, #5946, #20417 ),
 .UNSPECIFIED., .F., .F. ) 
 B_SPLINE_CURVE_WITH_KNOTS ( ( 3, 2, 2, 2, 3 ),
 ( 0.1017857142857142849, 0.1023809523809523780, 0.1035714285714285782, 0.1047619047619047644, 0.1053571428571428575 ),
 .UNSPECIFIED. ) 
 CURVE ( )  GEOMETRIC_REPRESENTATION_ITEM ( )  RATIONAL_B_SPLINE_CURVE ( ( 0.9330127018922194093, 0.9330127018922194093, 1.000000000000000000, 0.8660254037844387076, 1.000000000000000000, 0.8660254037844387076, 1.000000000000000000, 0.9330127018922194093, 0.9330127018922194093 ) ) 
 REPRESENTATION_ITEM ( '' )  );
#45622=CARTESIAN_POINT ( 'NONE',  ( -5.000000000000000000, -57.87499999726880873, 0.000000000000000000 ) ) ;
#45626=CARTESIAN_POINT ( 'NONE',  ( 5.000000000000000000, -59.50000000000000000, -6.123233995736766282E-16 ) ) ;
#45627=CARTESIAN_POINT ( 'NONE',  ( 2.500000000000002220, -90.54166666393547303, 4.330127018922192761 ) ) ;
#45629=VERTEX_POINT ( 'NONE', #26609 ) ;
#45630=CARTESIAN_POINT ( 'NONE',  ( -4.999999999999998224, -56.91666666666667140, 2.886751345948131764 ) ) ;
#45642=VERTEX_POINT ( 'NONE', #56526 ) ;
#45645=CARTESIAN_POINT ( 'NONE',  ( -2.229367062499996610, -44.39583333196774362, 3.861377020970582219 ) ) ;
#45646=CARTESIAN_POINT ( 'NONE',  ( 2.500000000000002220, -68.54166666393547303, 4.330127018922192761 ) ) ;
#45652=AXIS2_PLACEMENT_3D ( 'NONE', #8688, #28301, #3871 ) ;
#45653=CARTESIAN_POINT ( 'NONE',  ( -2.499999999999996447, 1.166666666666666519, 4.330127018922195425 ) ) ;
#45655=CARTESIAN_POINT ( 'NONE',  ( 4.458734124999999437, -95.06249999863440792, -5.460374474430324690E-16 ) ) ;
#45662=VERTEX_POINT ( 'NONE', #51694 ) ;
#45663=CARTESIAN_POINT ( 'NONE',  ( 9.457646018065525792E-16, -4.062499998634408804, 5.148502694627439702 ) ) ;
#45664=CARTESIAN_POINT ( 'NONE',  ( 2.229367062499998831, -22.89583333196773651, -3.861377020970580887 ) ) ;
#45671=CARTESIAN_POINT ( 'NONE',  ( 4.458734124999999437, 17.93750000136559208, -5.460374474430324690E-16 ) ) ;
#45672=EDGE_LOOP ( 'NONE', ( #44429, #23516, #32734, #31934 ) ) ;
#45673=CARTESIAN_POINT ( 'NONE',  ( -6.972266317189433020E-16, -37.25000000000000000, -5.000000000000000000 ) ) ;
#45674=CARTESIAN_POINT ( 'NONE',  ( 1.339745962155612702, -71.16965819600731891, -5.000000000000000000 ) ) ;
#45675=CARTESIAN_POINT ( 'NONE',  ( 4.458734124999998549, -20.72916666530106866, -2.574251347313721627 ) ) ;
#45680=EDGE_CURVE ( 'NONE', #32980, #62343, #7947, .T. ) ;
#45681=CARTESIAN_POINT ( 'NONE',  ( -3.535250795749689387E-16, -47.12499999726880873, -5.773502691896257311 ) ) ;
#45683=CARTESIAN_POINT ( 'NONE',  ( 2.229367062500001939, 8.020833334698926009, 3.861377020970579999 ) ) ;
#45685=CYLINDRICAL_SURFACE ( 'NONE', #41781, 5.000000000000000000 ) ;
#45688=CARTESIAN_POINT ( 'NONE',  ( -4.458734124999999437, -66.31249999863440792, 0.000000000000000000 ) ) ;
#45690=CARTESIAN_POINT ( 'NONE',  ( 5.000000000000000000, -0.5000000000000004441, -6.123233995736766282E-16 ) ) ;
#45692=CARTESIAN_POINT ( 'NONE',  ( -1.339745962155613812, 21.79465819873852084, -5.000000000000000000 ) ) ;
#45693=CARTESIAN_POINT ( 'NONE',  ( -4.458734124999998549, -61.22916666530106511, 2.574251347313722516 ) ) ;
#45694=CARTESIAN_POINT ( 'NONE',  ( 5.000000000000000888, -96.45833333060213022, 2.886751345948126879 ) ) ;
#45700=CARTESIAN_POINT ( 'NONE',  ( -4.330127018922101279, 45.00000000000000000, 7.500000000000002665 ) ) ;
#45702=CARTESIAN_POINT ( 'NONE',  ( 5.000000000000000000, -45.41666666666666430, -2.886751345948129988 ) ) ;
#45703=CARTESIAN_POINT ( 'NONE',  ( 5.000000000000000888, -13.58333333333333570, 2.886751345948126879 ) ) ;
#45705=CARTESIAN_POINT ( 'NONE',  ( 1.975475456537005874E-15, -86.62499999726880162, 5.000000000000000000 ) ) ;
#45707=CARTESIAN_POINT ( 'NONE',  ( 4.458734124999998549, -107.7291666653010509, -2.574251347313721627 ) ) ;
#45708=CARTESIAN_POINT ( 'NONE',  ( 2.229367062500001939, -2.229166665301068662, 3.861377020970579999 ) ) ;
#45709=CARTESIAN_POINT ( 'NONE',  ( 3.044556291839386294E-14, 17.87500000273118417, -5.000000000000000000 ) ) ;
#45713=DIRECTION ( 'NONE',  ( -0.000000000000000000, 1.000000000000000000, -0.000000000000000000 ) ) ;
#45718=CARTESIAN_POINT ( 'NONE',  ( -5.000000000000000000, -16.87499999726881583, 0.000000000000000000 ) ) ;
#45720=EDGE_LOOP ( 'NONE', ( #48811, #55071, #42953, #20331 ) ) ;
#45721=CARTESIAN_POINT ( 'NONE',  ( 0.000000000000000000, -120.0000000000000000, 5.000000000000000000 ) ) ;
#45723=CARTESIAN_POINT ( 'NONE',  ( 2.229367062499998831, -28.89583333196774007, -3.861377020970580887 ) ) ;
#45732=CARTESIAN_POINT ( 'NONE',  ( -2.499999999999996447, -93.70833333060214443, 4.330127018922195425 ) ) ;
#45733=ORIENTED_EDGE ( 'NONE', *, *, #38126, .F. ) ;
#45734=CARTESIAN_POINT ( 'NONE',  ( -4.458734124999998549, -80.47916666530106511, 2.574251347313722516 ) ) ;
#45740=CARTESIAN_POINT ( 'NONE',  ( -3.152548672688508926E-16, -3.812499998634408360, -5.148502694627439702 ) ) ;
#45741=VERTEX_POINT ( 'NONE', #38158 ) ;
#45743=CARTESIAN_POINT ( 'NONE',  ( -1.339745962155640457, 3.330341803992664218, 4.999999999999984901 ) ) ;
#45745=CARTESIAN_POINT ( 'NONE',  ( -6.972266317189433020E-16, -53.12499999726880162, -5.000000000000000000 ) ) ;
#45747=CARTESIAN_POINT ( 'NONE',  ( 1.975475456537005874E-15, -11.62499999726881406, 5.000000000000000000 ) ) ;
#45750=ORIENTED_EDGE ( 'NONE', *, *, #47442, .T. ) ;
#45751=CARTESIAN_POINT ( 'NONE',  ( 9.457646018065525792E-16, -89.06249999863439371, 5.148502694627439702 ) ) ;
#45752=DIRECTION ( 'NONE',  ( -0.000000000000000000, 1.000000000000000000, -0.000000000000000000 ) ) ;
#45753=CARTESIAN_POINT ( 'NONE',  ( 9.457646018065525792E-16, -2.062499998634407028, 5.148502694627439702 ) ) ;
#45756=CARTESIAN_POINT ( 'NONE',  ( 5.000000000000000000, -30.29166666393548013, -2.886751345948129988 ) ) ;
#45758=CARTESIAN_POINT ( 'NONE',  ( 4.458734124999998549, 22.27083333469892779, -2.574251347313721627 ) ) ;
#45759=CARTESIAN_POINT ( 'NONE',  ( -5.000000000000000000, -37.95833333060213022, -2.886751345948128211 ) ) ;
#45760=CARTESIAN_POINT ( 'NONE',  ( 2.229367062500001939, -48.97916666530107221, 3.861377020970579999 ) ) ;
#45761=CARTESIAN_POINT ( 'NONE',  ( -2.229367062500000163, -36.72916666530107221, -3.861377020970580443 ) ) ;
#45763=CARTESIAN_POINT ( 'NONE',  ( -1.339745962155610925, 9.330341803992663330, 5.000000000000000000 ) ) ;
#45764=CARTESIAN_POINT ( 'NONE',  ( -3.535250795749689387E-16, 20.74999999999999645, -5.773502691896257311 ) ) ;
#45767=CARTESIAN_POINT ( 'NONE',  ( -4.458734124999999437, -42.39583333196773651, -2.574251347313719407 ) ) ;
#45768=CARTESIAN_POINT ( 'NONE',  ( -5.000000000000000000, -79.95833333060213022, -2.886751345948128211 ) ) ;
#45771=CARTESIAN_POINT ( 'NONE',  ( 1.975475456537005874E-15, -31.75000000000000000, 5.000000000000000000 ) ) ;
#45772=CARTESIAN_POINT ( 'NONE',  ( 4.458734124999998549, -81.97916666530106511, -2.574251347313721627 ) ) ;
#45775=CARTESIAN_POINT ( 'NONE',  ( 5.000000000000000000, -28.49999999999999645, -6.123233995736766282E-16 ) ) ;
#45780=CARTESIAN_POINT ( 'NONE',  ( 4.458734125000001214, -88.89583333196773651, 2.574251347313718519 ) ) ;
#45781=CARTESIAN_POINT ( 'NONE',  ( 2.229367062500001939, 12.77083333469892779, 3.861377020970579999 ) ) ;
#45782=CARTESIAN_POINT ( 'NONE',  ( -2.499999999999996447, 16.29166666939785202, 4.330127018922195425 ) ) ;
#45790=CARTESIAN_POINT ( 'NONE',  ( 2.500000000000002220, -99.54166666393545881, 4.330127018922192761 ) ) ;
#45794=DIRECTION ( 'NONE',  ( -0.000000000000000000, 1.000000000000000000, -0.000000000000000000 ) ) ;
#45795=CARTESIAN_POINT ( 'NONE',  ( 4.458734125000001214, -16.14583333196773651, 2.574251347313718519 ) ) ;
#45801=( BOUNDED_CURVE ( )  B_SPLINE_CURVE ( 2, ( #51810, #17715, #46667, #36702, #52759, #56961, #2612, #32499, #22230 ),
 .UNSPECIFIED., .F., .F. ) 
 B_SPLINE_CURVE_WITH_KNOTS ( ( 3, 2, 2, 2, 3 ),
 ( 0.9232142857142857650, 0.9238095238095238582, 0.9250000000000000444, 0.9261904761904762307, 0.9267857142857143238 ),
 .UNSPECIFIED. ) 
 CURVE ( )  GEOMETRIC_REPRESENTATION_ITEM ( )  RATIONAL_B_SPLINE_CURVE ( ( 0.9330127018922194093, 0.9330127018922194093, 1.000000000000000000, 0.8660254037844387076, 1.000000000000000000, 0.8660254037844387076, 1.000000000000000000, 0.9330127018922194093, 0.9330127018922194093 ) ) 
 REPRESENTATION_ITEM ( '' )  );
#45807=CARTESIAN_POINT ( 'NONE',  ( -1.339745962155610925, -85.79465819873851729, 5.000000000000000000 ) ) ;
#45809=ORIENTED_EDGE ( 'NONE', *, *, #8391, .F. ) ;
#45810=CARTESIAN_POINT ( 'NONE',  ( -2.499999999999996447, -9.833333333333332149, 4.330127018922195425 ) ) ;
#45812=FACE_OUTER_BOUND ( 'NONE', #23451, .T. ) ;
#45814=ORIENTED_EDGE ( 'NONE', *, *, #18833, .T. ) ;
#45816=CARTESIAN_POINT ( 'NONE',  ( 1.975475456537005874E-15, -25.62499999726881228, 5.000000000000000000 ) ) ;
#45817=CARTESIAN_POINT ( 'NONE',  ( -2.229367062500000163, 11.52083333469892601, -3.861377020970580443 ) ) ;
#45820=LINE ( 'NONE', #11084, #37751 ) ;
#45822=CARTESIAN_POINT ( 'NONE',  ( 9.457646018065525792E-16, -67.06249999863440792, 5.148502694627439702 ) ) ;
#45823=LINE ( 'NONE', #26527, #17135 ) ;
#45824=CARTESIAN_POINT ( 'NONE',  ( -4.458734124999998549, 13.77083333469892779, 2.574251347313722516 ) ) ;
#45826=VECTOR ( 'NONE', #62770, 1000.000000000000000 ) ;
#45827=CARTESIAN_POINT ( 'NONE',  ( 1.339745962155641346, 7.830341803992665994, -4.999999999999983125 ) ) ;
#45829=CARTESIAN_POINT ( 'NONE',  ( 4.458734124999999437, -55.06249999863440081, -5.460374474430324690E-16 ) ) ;
#45830=CARTESIAN_POINT ( 'NONE',  ( -3.535250795749689387E-16, -13.12499999726881050, -5.773502691896257311 ) ) ;
#45831=CARTESIAN_POINT ( 'NONE',  ( 0.000000000000000000, -120.0000000000000000, 5.000000000000000000 ) ) ;
#45833=CARTESIAN_POINT ( 'NONE',  ( 2.500000000000002220, -64.54166666393547303, 4.330127018922192761 ) ) ;
#45834=CARTESIAN_POINT ( 'NONE',  ( 4.458734124999999437, -17.06249999863440792, -5.460374474430324690E-16 ) ) ;
#45837=CARTESIAN_POINT ( 'NONE',  ( 2.229367062500001939, -105.9791666653010651, 3.861377020970579999 ) ) ;
#45839=ORIENTED_EDGE ( 'NONE', *, *, #24466, .F. ) ;
#45840=CARTESIAN_POINT ( 'NONE',  ( -2.229367062499996610, -104.3958333319677365, 3.861377020970582219 ) ) ;
#45841=CARTESIAN_POINT ( 'NONE',  ( 9.457646018065525792E-16, -29.06249999863440081, 5.148502694627439702 ) ) ;
#45842=CARTESIAN_POINT ( 'NONE',  ( -4.999999999999999112, -63.79166666393547303, 2.886751345948131764 ) ) ;
#45845=CARTESIAN_POINT ( 'NONE',  ( 2.229367062499998831, -24.64583333196773651, -3.861377020970580887 ) ) ;
#45846=CARTESIAN_POINT ( 'NONE',  ( -4.458734124999999437, -65.56249999863440792, 0.000000000000000000 ) ) ;
#45849=DIRECTION ( 'NONE',  ( 0.000000000000000000, 0.000000000000000000, 1.000000000000000000 ) ) ;
#45851=CARTESIAN_POINT ( 'NONE',  ( -3.535250795749689387E-16, -9.250000000000001776, -5.773502691896257311 ) ) ;
#45860=CARTESIAN_POINT ( 'NONE',  ( 2.500000000000002220, 20.45833333606451987, 4.330127018922192761 ) ) ;
#45864=LINE ( 'NONE', #55213, #9950 ) ;
#45866=( BOUNDED_CURVE ( )  B_SPLINE_CURVE ( 2, ( #18762, #58015, #33567, #38692, #43516, #19072, #14255, #33878, #9427 ),
 .UNSPECIFIED., .F., .F. ) 
 B_SPLINE_CURVE_WITH_KNOTS ( ( 3, 2, 2, 2, 3 ),
 ( 0.6339285714285713969, 0.6345238095238094900, 0.6357142857142856762, 0.6369047619047618625, 0.6374999999999999556 ),
 .UNSPECIFIED. ) 
 CURVE ( )  GEOMETRIC_REPRESENTATION_ITEM ( )  RATIONAL_B_SPLINE_CURVE ( ( 0.9330127018922194093, 0.9330127018922194093, 1.000000000000000000, 0.8660254037844387076, 1.000000000000000000, 0.8660254037844387076, 1.000000000000000000, 0.9330127018922194093, 0.9330127018922194093 ) ) 
 REPRESENTATION_ITEM ( '' )  );
#45871=VECTOR ( 'NONE', #56446, 1000.000000000000000 ) ;
#45873=ORIENTED_EDGE ( 'NONE', *, *, #50629, .F. ) ;
#45884=CYLINDRICAL_SURFACE ( 'NONE', #52884, 5.000000000000000000 ) ;
#45886=CARTESIAN_POINT ( 'NONE',  ( 4.458734124999998549, -79.72916666530107932, -2.574251347313721627 ) ) ;
#45887=CARTESIAN_POINT ( 'NONE',  ( -4.458734124999999437, 28.68750000136559208, 0.000000000000000000 ) ) ;
#45889=VERTEX_POINT ( 'NONE', #57783 ) ;
#45894=CARTESIAN_POINT ( 'NONE',  ( 4.458734124999999437, -45.81249999863440081, -5.460374474430324690E-16 ) ) ;
#45896=( BOUNDED_CURVE ( )  B_SPLINE_CURVE ( 2, ( #37750, #3975, #23595, #51914, #3663, #38066, #43192, #8482, #18749 ),
 .UNSPECIFIED., .F., .F. ) 
 B_SPLINE_CURVE_WITH_KNOTS ( ( 3, 2, 2, 2, 3 ),
 ( 0.6053571428571428159, 0.6059523809523809090, 0.6071428571428570953, 0.6083333333333332815, 0.6089285714285714857 ),
 .UNSPECIFIED. ) 
 CURVE ( )  GEOMETRIC_REPRESENTATION_ITEM ( )  RATIONAL_B_SPLINE_CURVE ( ( 0.9330127018922194093, 0.9330127018922194093, 1.000000000000000000, 0.8660254037844387076, 1.000000000000000000, 0.8660254037844387076, 1.000000000000000000, 0.9330127018922130810, 0.9330127018922194093 ) ) 
 REPRESENTATION_ITEM ( '' )  );
#45898=CARTESIAN_POINT ( 'NONE',  ( 4.458734124999999437, -47.81249999863440792, -5.460374474430324690E-16 ) ) ;
#45900=CARTESIAN_POINT ( 'NONE',  ( 2.229367062500001939, 28.02083333469892779, 3.861377020970579999 ) ) ;
#45901=CARTESIAN_POINT ( 'NONE',  ( -4.999999999999999112, -98.91666666666665719, 2.886751345948131764 ) ) ;
#45904=CARTESIAN_POINT ( 'NONE',  ( 4.458734125000001214, -41.14583333196774362, 2.574251347313718519 ) ) ;
#45905=CARTESIAN_POINT ( 'NONE',  ( 5.000000000000000888, -0.4583333306021480369, 2.886751345948126879 ) ) ;
#45909=CARTESIAN_POINT ( 'NONE',  ( -3.152548672688508926E-16, -98.56249999863439371, -5.148502694627439702 ) ) ;
#45911=CARTESIAN_POINT ( 'NONE',  ( -4.458734124999999437, -0.5624999986344053626, 0.000000000000000000 ) ) ;
#45912=VERTEX_POINT ( 'NONE', #53259 ) ;
#45915=CARTESIAN_POINT ( 'NONE',  ( -2.499999999999996447, -75.83333333333334281, 4.330127018922195425 ) ) ;
#45916=CARTESIAN_POINT ( 'NONE',  ( -4.458734124999999437, -87.39583333196773651, -2.574251347313719407 ) ) ;
#45918=CARTESIAN_POINT ( 'NONE',  ( -4.458734124999999437, -85.64583333196773651, -2.574251347313719407 ) ) ;
#45923=CARTESIAN_POINT ( 'NONE',  ( -4.458734124999999437, -7.395833331967734736, -2.574251347313719407 ) ) ;
#45924=CARTESIAN_POINT ( 'NONE',  ( 2.229367062499998831, 17.10416666803225993, -3.861377020970580887 ) ) ;
#45925=CARTESIAN_POINT ( 'NONE',  ( 4.458734124999999437, -47.06249999863440792, -5.460374474430324690E-16 ) ) ;
#45932=CARTESIAN_POINT ( 'NONE',  ( 4.458734124999999437, -73.81249999863440792, -5.460374474430324690E-16 ) ) ;
#45933=CARTESIAN_POINT ( 'NONE',  ( 1.060575238724906964E-15, -108.6249999972688016, 5.773502691896257311 ) ) ;
#45936=DIRECTION ( 'NONE',  ( 0.000000000000000000, 0.000000000000000000, 1.000000000000000000 ) ) ;
#45938=CARTESIAN_POINT ( 'NONE',  ( 5.000000000000000000, -62.41666666666666430, -2.886751345948129988 ) ) ;
#45939=CARTESIAN_POINT ( 'NONE',  ( -6.972266317189433020E-16, -36.12499999726880162, -5.000000000000000000 ) ) ;
#45941=ORIENTED_EDGE ( 'NONE', *, *, #17400, .F. ) ;
#45942=CARTESIAN_POINT ( 'NONE',  ( 0.000000000000000000, -120.0000000000000000, 0.000000000000000000 ) ) ;
#45952=CARTESIAN_POINT ( 'NONE',  ( 1.339745962155614700, 27.83034180399266688, -4.999999999999999112 ) ) ;
#45954=ORIENTED_EDGE ( 'NONE', *, *, #10696, .F. ) ;
#45957=CARTESIAN_POINT ( 'NONE',  ( 9.457646018065525792E-16, -44.31249999863440081, 5.148502694627439702 ) ) ;
#45958=CARTESIAN_POINT ( 'NONE',  ( 1.339745962155612702, -34.29465819873851729, -5.000000000000000000 ) ) ;
#45969=DIRECTION ( 'NONE',  ( 0.000000000000000000, 0.000000000000000000, 1.000000000000000000 ) ) ;
#45971=CARTESIAN_POINT ( 'NONE',  ( 9.457646018065525792E-16, -94.31249999863440792, 5.148502694627439702 ) ) ;
#45978=CARTESIAN_POINT ( 'NONE',  ( 1.339745962155612702, -60.29465819873851729, -5.000000000000000000 ) ) ;
#45979=CARTESIAN_POINT ( 'NONE',  ( 9.457646018065525792E-16, -3.062499998634407472, 5.148502694627439702 ) ) ;
#45981=CARTESIAN_POINT ( 'NONE',  ( -2.229367062500000163, -21.72916666530107221, -3.861377020970580443 ) ) ;
#45984=CARTESIAN_POINT ( 'NONE',  ( 2.499999999999998668, -70.33333333333332860, -4.330127018922193649 ) ) ;
#45987=CARTESIAN_POINT ( 'NONE',  ( -4.458734124999999437, 15.35416666803225993, -2.574251347313719407 ) ) ;
#45988=ORIENTED_EDGE ( 'NONE', *, *, #59043, .F. ) ;
#45989=CYLINDRICAL_SURFACE ( 'NONE', #7962, 5.000000000000000000 ) ;
#45991=CARTESIAN_POINT ( 'NONE',  ( 2.499999999999998668, -87.33333333333332860, -4.330127018922193649 ) ) ;
#45992=CARTESIAN_POINT ( 'NONE',  ( 2.229367062499998831, -18.64583333196774007, -3.861377020970580887 ) ) ;
#45994=DIRECTION ( 'NONE',  ( -0.000000000000000000, 1.000000000000000000, -0.000000000000000000 ) ) ;
#45997=CARTESIAN_POINT ( 'NONE',  ( 5.000000000000000888, -47.45833333060214443, 2.886751345948126879 ) ) ;
#45998=DIRECTION ( 'NONE',  ( 0.000000000000000000, 0.000000000000000000, 1.000000000000000000 ) ) ;
#45999=CARTESIAN_POINT ( 'NONE',  ( 9.457646018065525792E-16, 9.937500001365593860, 5.148502694627439702 ) ) ;
#46003=CARTESIAN_POINT ( 'NONE',  ( -3.152548672688508926E-16, -69.56249999863439371, -5.148502694627439702 ) ) ;
#46005=AXIS2_PLACEMENT_3D ( 'NONE', #57709, #58014, #53186 ) ;
#46006=CARTESIAN_POINT ( 'NONE',  ( -5.000000000000000000, -3.000000000000002665, 0.000000000000000000 ) ) ;
#46009=CARTESIAN_POINT ( 'NONE',  ( -2.229367062499996610, -59.14583333196773651, 3.861377020970582219 ) ) ;
#46010=CARTESIAN_POINT ( 'NONE',  ( -5.000000000000000000, -95.95833333060214443, -2.886751345948128211 ) ) ;
#46011=EDGE_CURVE ( 'NONE', #54753, #9578, #51371, .T. ) ;
#46012=VECTOR ( 'NONE', #58587, 1000.000000000000000 ) ;
#46017=CARTESIAN_POINT ( 'NONE',  ( 2.500000000000002220, -48.66666666666666430, 4.330127018922192761 ) ) ;
#46018=CARTESIAN_POINT ( 'NONE',  ( 1.339745962155615144, -13.70534180126148094, 4.999999999999999112 ) ) ;
#46021=CARTESIAN_POINT ( 'NONE',  ( -2.229367062500000163, -106.4791666653010651, -3.861377020970580443 ) ) ;
#46022=CARTESIAN_POINT ( 'NONE',  ( -3.152548672688508926E-16, -3.812499998634408360, -5.148502694627439702 ) ) ;
#46030=LINE ( 'NONE', #61159, #33337 ) ;
#46032=ORIENTED_EDGE ( 'NONE', *, *, #23995, .F. ) ;
#46033=CARTESIAN_POINT ( 'NONE',  ( 1.339745962155615144, -101.5803417985302985, 4.999999999999999112 ) ) ;
#46035=CARTESIAN_POINT ( 'NONE',  ( 4.458734124999999437, -28.06249999863440081, -5.460374474430324690E-16 ) ) ;
#46036=CARTESIAN_POINT ( 'NONE',  ( -1.339745962155610925, -10.66965819600733312, 5.000000000000000000 ) ) ;
#46042=EDGE_CURVE ( 'NONE', #62035, #20917, #53301, .T. ) ;
#46044=ORIENTED_EDGE ( 'NONE', *, *, #6331, .F. ) ;
#46045=CARTESIAN_POINT ( 'NONE',  ( 4.458734124999998549, -80.97916666530106511, -2.574251347313721627 ) ) ;
#46046=CARTESIAN_POINT ( 'NONE',  ( -2.500000000000000444, 12.95833333606451809, -4.330127018922193649 ) ) ;
#46048=EDGE_CURVE ( 'NONE', #24763, #54724, #42220, .T. ) ;
#46049=ORIENTED_EDGE ( 'NONE', *, *, #5248, .T. ) ;
#46050=CARTESIAN_POINT ( 'NONE',  ( -6.972266317189433020E-16, -16.25000000000000000, -5.000000000000000000 ) ) ;
#46051=( BOUNDED_CURVE ( )  B_SPLINE_CURVE ( 2, ( #23714, #62946, #58108, #33664, #53283, #9219, #48759, #43615, #33978 ),
 .UNSPECIFIED., .F., .F. ) 
 B_SPLINE_CURVE_WITH_KNOTS ( ( 3, 2, 2, 2, 3 ),
 ( 0.3910714285714285698, 0.3916666666666666630, 0.3928571428571428492, 0.3940476190476190355, 0.3946428571428571286 ),
 .UNSPECIFIED. ) 
 CURVE ( )  GEOMETRIC_REPRESENTATION_ITEM ( )  RATIONAL_B_SPLINE_CURVE ( ( 0.9330127018922194093, 0.9330127018922194093, 1.000000000000000000, 0.8660254037844387076, 1.000000000000000000, 0.8660254037844387076, 1.000000000000000000, 0.9330127018922194093, 0.9330127018922194093 ) ) 
 REPRESENTATION_ITEM ( '' )  );
#46052=CARTESIAN_POINT ( 'NONE',  ( 0.000000000000000000, -120.0000000000000000, 0.000000000000000000 ) ) ;
#46054=CARTESIAN_POINT ( 'NONE',  ( -4.458734124999998549, -11.47916666530107044, 2.574251347313722516 ) ) ;
#46057=CARTESIAN_POINT ( 'NONE',  ( -1.339745962155613812, -10.08034179853029144, -5.000000000000000000 ) ) ;
#46060=CARTESIAN_POINT ( 'NONE',  ( -3.152548672688508926E-16, -7.812499998634405252, -5.148502694627439702 ) ) ;
#46061=EDGE_CURVE ( 'NONE', #2195, #59356, #2409, .T. ) ;
#46063=CARTESIAN_POINT ( 'NONE',  ( 1.339745962155615144, -64.70534180126146850, 4.999999999999999112 ) ) ;
#46065=CARTESIAN_POINT ( 'NONE',  ( 1.339745962155615144, -75.58034179853029855, 4.999999999999999112 ) ) ;
#46066=VERTEX_POINT ( 'NONE', #4998 ) ;
#46067=CARTESIAN_POINT ( 'NONE',  ( 9.457646018065525792E-16, -88.06249999863439371, 5.148502694627439702 ) ) ;
#46070=CARTESIAN_POINT ( 'NONE',  ( 2.229367062499998831, -5.645833331967740953, -3.861377020970580887 ) ) ;
#46072=VECTOR ( 'NONE', #23986, 1000.000000000000000 ) ;
#46073=CARTESIAN_POINT ( 'NONE',  ( -5.000000000000000000, -30.87499999726881228, 0.000000000000000000 ) ) ;
#46075=CARTESIAN_POINT ( 'NONE',  ( -4.458734124999999437, 23.60416666803225993, -2.574251347313719407 ) ) ;
#46076=CARTESIAN_POINT ( 'NONE',  ( 1.339745962155612702, -110.1696581960073189, -5.000000000000000000 ) ) ;
#46078=CARTESIAN_POINT ( 'NONE',  ( -4.458734124999998549, -52.22916666530106511, 2.574251347313722516 ) ) ;
#46079=CARTESIAN_POINT ( 'NONE',  ( 4.458734124999999437, -37.06249999863440792, -5.460374474430324690E-16 ) ) ;
#46082=CARTESIAN_POINT ( 'NONE',  ( 1.060575238724906964E-15, 15.25000000000000000, 5.773502691896257311 ) ) ;
#46084=CARTESIAN_POINT ( 'NONE',  ( 2.229367062500001939, -44.97916666530106511, 3.861377020970579999 ) ) ;
#46085=CARTESIAN_POINT ( 'NONE',  ( 2.499999999999998668, -76.20833333060214443, -4.330127018922193649 ) ) ;
#46088=CARTESIAN_POINT ( 'NONE',  ( -4.999999999999998224, -63.79166666393547303, 2.886751345948131764 ) ) ;
#46089=CARTESIAN_POINT ( 'NONE',  ( -3.152548672688508926E-16, -84.81249999863439371, -5.148502694627439702 ) ) ;
#46092=CARTESIAN_POINT ( 'NONE',  ( -2.500000000000000444, -31.16666666666666785, -4.330127018922193649 ) ) ;
#46094=ORIENTED_EDGE ( 'NONE', *, *, #45680, .F. ) ;
#46097=CARTESIAN_POINT ( 'NONE',  ( 4.458734125000001214, -89.89583333196775072, 2.574251347313718519 ) ) ;
#46098=CARTESIAN_POINT ( 'NONE',  ( 4.458734124999999437, 11.93750000136559564, -5.460374474430324690E-16 ) ) ;
#46099=CARTESIAN_POINT ( 'NONE',  ( -3.535250795749689387E-16, 14.87500000273118594, -5.773502691896257311 ) ) ;
#46103=VECTOR ( 'NONE', #56969, 1000.000000000000000 ) ;
#46109=CARTESIAN_POINT ( 'NONE',  ( -2.500000000000000444, -75.04166666393547303, -4.330127018922193649 ) ) ;
#46113=CARTESIAN_POINT ( 'NONE',  ( -2.229367062500000163, -16.72916666530107577, -3.861377020970580443 ) ) ;
#46114=CARTESIAN_POINT ( 'NONE',  ( -2.916731409357579869E-14, 17.37500000273118417, 5.000000000000000888 ) ) ;
#46122=ORIENTED_EDGE ( 'NONE', *, *, #24835, .F. ) ;
#46124=VERTEX_POINT ( 'NONE', #40678 ) ;
#46125=CARTESIAN_POINT ( 'NONE',  ( 4.458734124999998549, -59.97916666530107221, -2.574251347313721627 ) ) ;
#46126=DIRECTION ( 'NONE',  ( 0.000000000000000000, 0.000000000000000000, 1.000000000000000000 ) ) ;
#46127=CARTESIAN_POINT ( 'NONE',  ( 1.339745962155612702, -103.2946581987385173, -5.000000000000000000 ) ) ;
#46129=ORIENTED_EDGE ( 'NONE', *, *, #45541, .F. ) ;
#46131=CARTESIAN_POINT ( 'NONE',  ( 1.975475456537005874E-15, -77.62499999726881583, 5.000000000000000000 ) ) ;
#46133=ORIENTED_EDGE ( 'NONE', *, *, #55046, .T. ) ;
#46134=CARTESIAN_POINT ( 'NONE',  ( -2.499999999999996447, -109.7083333306021444, 4.330127018922195425 ) ) ;
#46135=CARTESIAN_POINT ( 'NONE',  ( -2.229367062500000163, 10.52083333469892779, -3.861377020970580443 ) ) ;
#46140=CARTESIAN_POINT ( 'NONE',  ( -1.339745962155610925, -23.66965819600732956, 5.000000000000000000 ) ) ;
#46144=EDGE_CURVE ( 'NONE', #50284, #35341, #35658, .T. ) ;
#46145=CARTESIAN_POINT ( 'NONE',  ( -3.152548672688508926E-16, -72.56249999863439371, -5.148502694627439702 ) ) ;
#46146=DIRECTION ( 'NONE',  ( -0.000000000000000000, 1.000000000000000000, -0.000000000000000000 ) ) ;
#46147=CARTESIAN_POINT ( 'NONE',  ( 4.458734124999998549, 10.27083333469892779, -2.574251347313721627 ) ) ;
#46149=CARTESIAN_POINT ( 'NONE',  ( -6.972266317189433020E-16, -63.25000000000000000, -5.000000000000000000 ) ) ;
#46152=CARTESIAN_POINT ( 'NONE',  ( -3.152548672688508926E-16, -52.81249999863440792, -5.148502694627439702 ) ) ;
#46153=CARTESIAN_POINT ( 'NONE',  ( 2.499999999999998668, -13.20833333060214976, -4.330127018922193649 ) ) ;
#46154=FACE_OUTER_BOUND ( 'NONE', #43926, .T. ) ;
#46155=CARTESIAN_POINT ( 'NONE',  ( 0.000000000000000000, -120.0000000000000000, 5.000000000000000000 ) ) ;
#46156=CARTESIAN_POINT ( 'NONE',  ( -6.972266317189433020E-16, -80.12499999726881583, -5.000000000000000000 ) ) ;
#46157=CARTESIAN_POINT ( 'NONE',  ( 2.229367062500001939, -20.22916666530107221, 3.861377020970579999 ) ) ;
#46158=ORIENTED_EDGE ( 'NONE', *, *, #35105, .T. ) ;
#46160=CARTESIAN_POINT ( 'NONE',  ( 9.457646018065525792E-16, -109.0624999986344221, 5.148502694627439702 ) ) ;
#46162=ORIENTED_EDGE ( 'NONE', *, *, #32793, .F. ) ;
#46163=CARTESIAN_POINT ( 'NONE',  ( 4.458734125000001214, -105.1458333319677365, 2.574251347313718519 ) ) ;
#46164=CARTESIAN_POINT ( 'NONE',  ( -4.458734124999999437, -28.39583333196774007, -2.574251347313719407 ) ) ;
#46165=CARTESIAN_POINT ( 'NONE',  ( -5.000000000000000000, -64.95833333060214443, -2.886751345948128211 ) ) ;
#46168=CARTESIAN_POINT ( 'NONE',  ( -2.229367062500000163, -23.47916666530107221, -3.861377020970580443 ) ) ;
#46169=CARTESIAN_POINT ( 'NONE',  ( 9.457646018065525792E-16, -67.31249999863440792, 5.148502694627439702 ) ) ;
#46170=CARTESIAN_POINT ( 'NONE',  ( -5.000000000000000000, -39.87499999726880162, 0.000000000000000000 ) ) ;
#46172=CARTESIAN_POINT ( 'NONE',  ( -6.972266317189433020E-16, -32.24999999999999289, -5.000000000000000000 ) ) ;
#46174=CARTESIAN_POINT ( 'NONE',  ( 2.500000000000002220, -12.66666666666666607, 4.330127018922192761 ) ) ;
#46176=ORIENTED_EDGE ( 'NONE', *, *, #62993, .T. ) ;
#46178=CARTESIAN_POINT ( 'NONE',  ( 6.158835246850667461E-14, -3.124999997268814944, -4.999999999999999112 ) ) ;
#46179=CARTESIAN_POINT ( 'NONE',  ( 1.339745962155615144, -38.58034179853029144, 4.999999999999999112 ) ) ;
#46182=CARTESIAN_POINT ( 'NONE',  ( 5.000000000000000000, 25.50000000000000000, -6.123233995736766282E-16 ) ) ;
#46191=ORIENTED_EDGE ( 'NONE', *, *, #22058, .T. ) ;
#46192=CARTESIAN_POINT ( 'NONE',  ( 2.500000000000002220, 26.33333333333333215, 4.330127018922192761 ) ) ;
#46195=ADVANCED_FACE ( 'NONE', ( #18382 ), #37370, .T. ) ;
#46207=EDGE_LOOP ( 'NONE', ( #50716, #8169, #28638, #20498 ) ) ;
#46208=CARTESIAN_POINT ( 'NONE',  ( 2.229367062499998831, -77.64583333196773651, -3.861377020970580887 ) ) ;
#46209=CARTESIAN_POINT ( 'NONE',  ( 9.457646018065525792E-16, -110.3124999986343937, 5.148502694627439702 ) ) ;
#46210=CARTESIAN_POINT ( 'NONE',  ( 2.499999999999998668, -18.33333333333333215, -4.330127018922193649 ) ) ;
#46212=CARTESIAN_POINT ( 'NONE',  ( 0.000000000000000000, -120.0000000000000000, 0.000000000000000000 ) ) ;
#46216=DIRECTION ( 'NONE',  ( 0.000000000000000000, 0.000000000000000000, 1.000000000000000000 ) ) ;
#46219=CARTESIAN_POINT ( 'NONE',  ( 4.458734124999998549, -56.72916666530107932, -2.574251347313721627 ) ) ;
#46221=CARTESIAN_POINT ( 'NONE',  ( -4.458734124999999437, 28.68750000136559208, 0.000000000000000000 ) ) ;
#46222=CARTESIAN_POINT ( 'NONE',  ( -5.000000000000000000, -104.0000000000000142, 0.000000000000000000 ) ) ;
#46224=CARTESIAN_POINT ( 'NONE',  ( -2.229367062499996610, -36.39583333196773651, 3.861377020970582219 ) ) ;
#46225=CARTESIAN_POINT ( 'NONE',  ( -5.000000000000000000, 3.125000002731185944, 0.000000000000000000 ) ) ;
#46230=CARTESIAN_POINT ( 'NONE',  ( 2.229367062499998831, -96.64583333196773651, -3.861377020970580887 ) ) ;
#46231=CARTESIAN_POINT ( 'NONE',  ( -4.458734124999999437, -7.645833331967734736, -2.574251347313719407 ) ) ;
#46235=CARTESIAN_POINT ( 'NONE',  ( -3.152548672688508926E-16, -89.56249999863439371, -5.148502694627439702 ) ) ;
#46237=CARTESIAN_POINT ( 'NONE',  ( 4.458734124999998549, -87.97916666530107932, -2.574251347313721627 ) ) ;
#46240=CARTESIAN_POINT ( 'NONE',  ( 0.000000000000000000, -120.0000000000000000, 5.000000000000000000 ) ) ;
#46242=AXIS2_PLACEMENT_3D ( 'NONE', #32865, #24154, #29273 ) ;
#46243=CARTESIAN_POINT ( 'NONE',  ( 4.458734124999998549, -8.729166665301073991, -2.574251347313721627 ) ) ;
#46244=CARTESIAN_POINT ( 'NONE',  ( 4.458734124999999437, 16.93750000136559564, -5.460374474430324690E-16 ) ) ;
#46245=CARTESIAN_POINT ( 'NONE',  ( -2.229367062500000163, -50.72916666530107221, -3.861377020970580443 ) ) ;
#46246=CYLINDRICAL_SURFACE ( 'NONE', #42839, 5.000000000000000000 ) ;
#46252=( BOUNDED_CURVE ( )  B_SPLINE_CURVE ( 2, ( #44149, #9120, #28728, #49307, #54125, #13941, #430, #10063, #53497 ),
 .UNSPECIFIED., .F., .F. ) 
 B_SPLINE_CURVE_WITH_KNOTS ( ( 3, 2, 2, 2, 3 ),
 ( 0.5660714285714285587, 0.5666666666666666519, 0.5678571428571428381, 0.5690476190476190244, 0.5696428571428571175 ),
 .UNSPECIFIED. ) 
 CURVE ( )  GEOMETRIC_REPRESENTATION_ITEM ( )  RATIONAL_B_SPLINE_CURVE ( ( 0.9330127018922194093, 0.9330127018922194093, 1.000000000000000000, 0.8660254037844387076, 1.000000000000000000, 0.8660254037844387076, 1.000000000000000000, 0.9330127018922194093, 0.9330127018922194093 ) ) 
 REPRESENTATION_ITEM ( '' )  );
#46254=CARTESIAN_POINT ( 'NONE',  ( -4.458734124999999437, -78.39583333196772230, -2.574251347313719407 ) ) ;
#46255=CARTESIAN_POINT ( 'NONE',  ( 4.458734125000001214, 27.85416666803225993, 2.574251347313718519 ) ) ;
#46258=CARTESIAN_POINT ( 'NONE',  ( -2.500000000000000444, -94.16666666666665719, -4.330127018922193649 ) ) ;
#46261=CARTESIAN_POINT ( 'NONE',  ( -4.999999999999999112, -63.91666666666666430, 2.886751345948131764 ) ) ;
#46267=CARTESIAN_POINT ( 'NONE',  ( -5.000000000000000000, 8.916666666666666075, -2.886751345948128211 ) ) ;
#46282=CARTESIAN_POINT ( 'NONE',  ( 4.458734124999999437, -53.06249999863440792, -5.460374474430324690E-16 ) ) ;
#46285=CARTESIAN_POINT ( 'NONE',  ( 1.975475456537005874E-15, -35.75000000000000711, 5.000000000000000000 ) ) ;
#46290=CARTESIAN_POINT ( 'NONE',  ( -6.972266317189433020E-16, 0.7499999999999996669, -5.000000000000000000 ) ) ;
#46293=CARTESIAN_POINT ( 'NONE',  ( 2.229367062500001939, -96.22916666530105090, 3.861377020970579999 ) ) ;
#46299=DIRECTION ( 'NONE',  ( 0.000000000000000000, 0.000000000000000000, 1.000000000000000000 ) ) ;
#46300=CARTESIAN_POINT ( 'NONE',  ( 4.458734125000001214, -2.895833331967738289, 2.574251347313718519 ) ) ;
#46301=CARTESIAN_POINT ( 'NONE',  ( -4.458734124999999437, -97.56249999863440792, 0.000000000000000000 ) ) ;
#46304=CARTESIAN_POINT ( 'NONE',  ( 9.457646018065525792E-16, -22.31249999863440792, 5.148502694627439702 ) ) ;
#46308=CARTESIAN_POINT ( 'NONE',  ( 2.499999999999998668, 23.79166666939785202, -4.330127018922193649 ) ) ;
#46310=CARTESIAN_POINT ( 'NONE',  ( 9.457646018065525792E-16, 15.68750000136559564, 5.148502694627439702 ) ) ;
#46314=CARTESIAN_POINT ( 'NONE',  ( -2.500000000000000444, -85.16666666666667140, -4.330127018922193649 ) ) ;
#46315=CARTESIAN_POINT ( 'NONE',  ( -3.152548672688508926E-16, -20.56249999863440081, -5.148502694627439702 ) ) ;
#46319=CARTESIAN_POINT ( 'NONE',  ( 5.000000000000000000, -48.29166666393547303, -2.886751345948129988 ) ) ;
#46320=CARTESIAN_POINT ( 'NONE',  ( 2.229367062500001939, 10.02083333469892779, 3.861377020970579999 ) ) ;
#46321=DIRECTION ( 'NONE',  ( -0.000000000000000000, 1.000000000000000000, -0.000000000000000000 ) ) ;
#46324=CARTESIAN_POINT ( 'NONE',  ( 2.229367062500001939, -67.97916666530106511, 3.861377020970579999 ) ) ;
#46326=CARTESIAN_POINT ( 'NONE',  ( -5.000000000000000000, -2.083333333333333037, -2.886751345948128211 ) ) ;
#46330=CARTESIAN_POINT ( 'NONE',  ( 2.229367062500001939, -57.97916666530107932, 3.861377020970579999 ) ) ;
#46331=CARTESIAN_POINT ( 'NONE',  ( 1.060575238724906964E-15, -93.62499999726880162, 5.773502691896257311 ) ) ;
#46332=EDGE_CURVE ( 'NONE', #29366, #60851, #57944, .T. ) ;
#46336=CARTESIAN_POINT ( 'NONE',  ( 4.330127018922258486, 45.00000000000000000, 7.499999999999910294 ) ) ;
#46337=CARTESIAN_POINT ( 'NONE',  ( -5.000000000000000000, -50.00000000000000000, 0.000000000000000000 ) ) ;
#46341=CARTESIAN_POINT ( 'NONE',  ( -4.458734124999999437, -109.3958333319677507, -2.574251347313719407 ) ) ;
#46342=CARTESIAN_POINT ( 'NONE',  ( 4.458734124999999437, -1.062499998634405696, -5.460374474430324690E-16 ) ) ;
#46343=CARTESIAN_POINT ( 'NONE',  ( -5.000000000000000000, -99.87499999726881583, 0.000000000000000000 ) ) ;
#46346=CARTESIAN_POINT ( 'NONE',  ( -1.339745962155613812, -26.20534180126147916, -5.000000000000000000 ) ) ;
#46347=EDGE_CURVE ( 'NONE', #22715, #1445, #8424, .T. ) ;
#46352=ADVANCED_FACE ( 'NONE', ( #32862 ), #47648, .T. ) ;
#46354=VERTEX_POINT ( 'NONE', #28027 ) ;
#46355=DIRECTION ( 'NONE',  ( -0.000000000000000000, 1.000000000000000000, -0.000000000000000000 ) ) ;
#46358=CARTESIAN_POINT ( 'NONE',  ( 4.458734125000001214, -32.14583333196773651, 2.574251347313718519 ) ) ;
#46365=ADVANCED_FACE ( 'NONE', ( #37066 ), #13862, .T. ) ;
#46369=CARTESIAN_POINT ( 'NONE',  ( -2.229367062499996610, -77.39583333196773651, 3.861377020970582219 ) ) ;
#46371=ORIENTED_EDGE ( 'NONE', *, *, #16560, .T. ) ;
#46376=CARTESIAN_POINT ( 'NONE',  ( -2.229367062499996610, -8.395833331967736513, 3.861377020970582219 ) ) ;
#46380=CARTESIAN_POINT ( 'NONE',  ( -2.500000000000000444, 2.958333336064520314, -4.330127018922193649 ) ) ;
#46381=EDGE_CURVE ( 'NONE', #51908, #18523, #47342, .T. ) ;
#46382=CARTESIAN_POINT ( 'NONE',  ( -2.229367062499996610, -8.395833331967736513, 3.861377020970582219 ) ) ;
#46383=DIRECTION ( 'NONE',  ( -0.000000000000000000, 1.000000000000000000, -0.000000000000000000 ) ) ;
#46389=CARTESIAN_POINT ( 'NONE',  ( 4.458734124999998549, -86.72916666530107932, -2.574251347313721627 ) ) ;
#46391=CARTESIAN_POINT ( 'NONE',  ( 9.457646018065525792E-16, -1.062499998634405696, 5.148502694627439702 ) ) ;
#46392=DIRECTION ( 'NONE',  ( -0.000000000000000000, 1.000000000000000000, -0.000000000000000000 ) ) ;
#46393=CARTESIAN_POINT ( 'NONE',  ( 5.000000000000000000, -31.37499999726880873, -6.123233995736766282E-16 ) ) ;
#46395=CARTESIAN_POINT ( 'NONE',  ( 9.457646018065525792E-16, 22.93750000136559919, 5.148502694627439702 ) ) ;
#46397=CARTESIAN_POINT ( 'NONE',  ( 9.457646018065525792E-16, -51.06249999863440792, 5.148502694627439702 ) ) ;
#46398=CARTESIAN_POINT ( 'NONE',  ( -2.229367062499996610, -39.39583333196773651, 3.861377020970582219 ) ) ;
#46401=CARTESIAN_POINT ( 'NONE',  ( -4.999999999999999112, 15.08333333333333215, 2.886751345948131764 ) ) ;
#46404=CARTESIAN_POINT ( 'NONE',  ( -4.458734124999999437, -45.39583333196773651, -2.574251347313719407 ) ) ;
#46405=CARTESIAN_POINT ( 'NONE',  ( 1.060575238724906964E-15, -80.62499999726881583, 5.773502691896257311 ) ) ;
#46408=CARTESIAN_POINT ( 'NONE',  ( 5.000000000000000000, -65.37499999726881583, -6.123233995736766282E-16 ) ) ;
#46411=CARTESIAN_POINT ( 'NONE',  ( 9.457646018065525792E-16, -83.31249999863440792, 5.148502694627439702 ) ) ;
#46413=CARTESIAN_POINT ( 'NONE',  ( 1.339745962155615144, 13.41965820146970501, 4.999999999999999112 ) ) ;
#46414=CARTESIAN_POINT ( 'NONE',  ( 5.000000000000000000, -33.41666666666666430, -2.886751345948129988 ) ) ;
#46419=CARTESIAN_POINT ( 'NONE',  ( 4.458734124999998549, -90.72916666530106511, -2.574251347313721627 ) ) ;
#46420=CARTESIAN_POINT ( 'NONE',  ( -2.229367062500000163, 11.27083333469892601, -3.861377020970580443 ) ) ;
#46421=CARTESIAN_POINT ( 'NONE',  ( -2.499999999999996447, 14.29166666939785202, 4.330127018922195425 ) ) ;
#46422=CARTESIAN_POINT ( 'NONE',  ( -5.000000000000000000, -43.95833333060214443, -2.886751345948128211 ) ) ;
#46428=CARTESIAN_POINT ( 'NONE',  ( 0.000000000000000000, -120.0000000000000000, 0.000000000000000000 ) ) ;
#46429=CARTESIAN_POINT ( 'NONE',  ( 2.500000000000002220, -33.54166666393547303, 4.330127018922192761 ) ) ;
#46431=LINE ( 'NONE', #17787, #14484 ) ;
#46436=CARTESIAN_POINT ( 'NONE',  ( -4.458734124999999437, -14.64583333196773474, -2.574251347313719407 ) ) ;
#46447=CARTESIAN_POINT ( 'NONE',  ( -2.229367062500000163, -63.72916666530106511, -3.861377020970580443 ) ) ;
#46449=CARTESIAN_POINT ( 'NONE',  ( 5.000000000000000888, 11.54166666939785202, 2.886751345948126879 ) ) ;
#46456=VERTEX_POINT ( 'NONE', #44389 ) ;
#46457=CARTESIAN_POINT ( 'NONE',  ( 5.000000000000000888, 11.41666666666666607, 2.886751345948126879 ) ) ;
#46458=CARTESIAN_POINT ( 'NONE',  ( 2.229367062500001939, 6.020833334698927786, 3.861377020970579999 ) ) ;
#46461=CARTESIAN_POINT ( 'NONE',  ( -2.499999999999996447, -23.70833333060214443, 4.330127018922195425 ) ) ;
#46464=CARTESIAN_POINT ( 'NONE',  ( -4.458734124999997661, -70.22916666530107932, 2.574251347313722516 ) ) ;
#46465=CARTESIAN_POINT ( 'NONE',  ( 4.458734125000001214, 14.10416666803225993, 2.574251347313718519 ) ) ;
#46466=CARTESIAN_POINT ( 'NONE',  ( 2.500000000000002220, -60.54166666393547303, 4.330127018922192761 ) ) ;
#46467=CARTESIAN_POINT ( 'NONE',  ( -5.000000000000000000, -89.00000000000000000, 0.000000000000000000 ) ) ;
#46468=CARTESIAN_POINT ( 'NONE',  ( 2.229367062499998831, -55.89583333196773651, -3.861377020970580887 ) ) ;
#46469=CARTESIAN_POINT ( 'NONE',  ( -2.500000000000000444, -14.04166666393548013, -4.330127018922193649 ) ) ;
#46470=DIRECTION ( 'NONE',  ( -0.000000000000000000, 1.000000000000000000, -0.000000000000000000 ) ) ;
#46472=CARTESIAN_POINT ( 'NONE',  ( 5.000000000000000000, -65.41666666666667140, -2.886751345948130876 ) ) ;
#46473=CARTESIAN_POINT ( 'NONE',  ( -4.458734124999999437, -20.56249999863440081, 0.000000000000000000 ) ) ;
#46474=ORIENTED_EDGE ( 'NONE', *, *, #10250, .F. ) ;
#46476=CARTESIAN_POINT ( 'NONE',  ( -2.499999999999996447, -60.83333333333333570, 4.330127018922195425 ) ) ;
#46477=CARTESIAN_POINT ( 'NONE',  ( 2.500000000000002220, 29.33333333333333215, 4.330127018922192761 ) ) ;
#46480=CARTESIAN_POINT ( 'NONE',  ( 4.458734125000001214, -101.1458333319677365, 2.574251347313718519 ) ) ;
#46481=CARTESIAN_POINT ( 'NONE',  ( 2.229367062500001939, -24.97916666530106866, 3.861377020970579999 ) ) ;
#46482=CARTESIAN_POINT ( 'NONE',  ( -3.535250795749689387E-16, -62.12499999726880873, -5.773502691896257311 ) ) ;
#46486=CARTESIAN_POINT ( 'NONE',  ( 2.229367062500001939, -23.97916666530107577, 3.861377020970579999 ) ) ;
#46487=CARTESIAN_POINT ( 'NONE',  ( -2.229367062499996610, -67.39583333196773651, 3.861377020970582219 ) ) ;
#46488=DIRECTION ( 'NONE',  ( 3.305092117221761110E-15, -0.000000000000000000, 1.000000000000000000 ) ) ;
#46490=CARTESIAN_POINT ( 'NONE',  ( -6.972266317189433020E-16, -49.12499999726880162, -5.000000000000000000 ) ) ;
#46492=CARTESIAN_POINT ( 'NONE',  ( 5.000000000000000000, -15.50000000000000000, -6.123233995736766282E-16 ) ) ;
#46495=DIRECTION ( 'NONE',  ( -0.000000000000000000, 1.000000000000000000, -0.000000000000000000 ) ) ;
#46497=EDGE_CURVE ( 'NONE', #63218, #43948, #39561, .T. ) ;
#46498=CARTESIAN_POINT ( 'NONE',  ( -1.339745962155613812, -87.08034179853028434, -5.000000000000000000 ) ) ;
#46499=CARTESIAN_POINT ( 'NONE',  ( -4.999999999999998224, -110.7916666639354730, 2.886751345948131764 ) ) ;
#46501=ADVANCED_FACE ( 'NONE', ( #58565 ), #10304, .T. ) ;
#46502=EDGE_CURVE ( 'NONE', #46066, #60305, #38213, .T. ) ;
#46510=ADVANCED_FACE ( 'NONE', ( #14486 ), #38611, .T. ) ;
#46531=CARTESIAN_POINT ( 'NONE',  ( -4.458734124999999437, -78.31249999863440792, 0.000000000000000000 ) ) ;
#46532=CARTESIAN_POINT ( 'NONE',  ( 4.458734124999999437, 26.18750000136559564, -5.460374474430324690E-16 ) ) ;
#46534=ORIENTED_EDGE ( 'NONE', *, *, #5983, .T. ) ;
#46535=FACE_OUTER_BOUND ( 'NONE', #6723, .T. ) ;
#46540=CARTESIAN_POINT ( 'NONE',  ( -2.499999999999996447, -82.83333333333332860, 4.330127018922195425 ) ) ;
#46542=CARTESIAN_POINT ( 'NONE',  ( 2.229367062499998831, -52.64583333196773651, -3.861377020970580887 ) ) ;
#46544=CARTESIAN_POINT ( 'NONE',  ( 2.229367062500001939, 26.02083333469892779, 3.861377020970579999 ) ) ;
#46545=CARTESIAN_POINT ( 'NONE',  ( 2.500000000000002220, -107.6666666666666572, 4.330127018922192761 ) ) ;
#46547=CARTESIAN_POINT ( 'NONE',  ( -4.458734124999999437, -36.64583333196773651, -2.574251347313719407 ) ) ;
#46548=CARTESIAN_POINT ( 'NONE',  ( 5.000000000000000000, -0.3749999972688135008, -6.123233995736766282E-16 ) ) ;
#46552=CARTESIAN_POINT ( 'NONE',  ( -6.972266317189433020E-16, 5.749999999999999112, -5.000000000000000000 ) ) ;
#46553=CARTESIAN_POINT ( 'NONE',  ( -2.229367062499996610, -101.1458333319677365, 3.861377020970582219 ) ) ;
#46554=CARTESIAN_POINT ( 'NONE',  ( 2.229367062499998831, -7.895833331967735624, -3.861377020970580887 ) ) ;
#46555=ORIENTED_EDGE ( 'NONE', *, *, #26597, .F. ) ;
#46557=CARTESIAN_POINT ( 'NONE',  ( -5.000000000000000000, -35.87499999726881583, 0.000000000000000000 ) ) ;
#46558=CARTESIAN_POINT ( 'NONE',  ( -4.458734124999999437, -95.31249999863440792, 0.000000000000000000 ) ) ;
#46560=CARTESIAN_POINT ( 'NONE',  ( -2.229367062499996610, -89.39583333196773651, 3.861377020970582219 ) ) ;
#46562=CARTESIAN_POINT ( 'NONE',  ( 1.975475456537005874E-15, -2.624999997268813168, 5.000000000000000000 ) ) ;
#46565=CARTESIAN_POINT ( 'NONE',  ( -4.458734124999997661, -6.229166665301072214, 2.574251347313722516 ) ) ;
#46566=CARTESIAN_POINT ( 'NONE',  ( 2.229367062499998831, 14.10416666803226171, -3.861377020970580887 ) ) ;
#46567=CARTESIAN_POINT ( 'NONE',  ( 2.229367062499998831, -52.89583333196773651, -3.861377020970580887 ) ) ;
#46572=ORIENTED_EDGE ( 'NONE', *, *, #22458, .T. ) ;
#46575=CARTESIAN_POINT ( 'NONE',  ( -4.458734124999999437, -82.31249999863440792, 0.000000000000000000 ) ) ;
#46576=CARTESIAN_POINT ( 'NONE',  ( 9.457646018065525792E-16, 24.68750000136559208, 5.148502694627439702 ) ) ;
#46581=DIRECTION ( 'NONE',  ( -0.000000000000000000, 1.000000000000000000, -0.000000000000000000 ) ) ;
#46583=CARTESIAN_POINT ( 'NONE',  ( -2.500000000000000444, -66.16666666666667140, -4.330127018922193649 ) ) ;
#46587=CARTESIAN_POINT ( 'NONE',  ( -5.000000000000000000, 27.91666666666666430, -2.886751345948128211 ) ) ;
#46600=CARTESIAN_POINT ( 'NONE',  ( 4.458734124999998549, -51.97916666530107221, -2.574251347313721627 ) ) ;
#46609=CARTESIAN_POINT ( 'NONE',  ( 4.458734124999998549, -100.9791666653010509, -2.574251347313721627 ) ) ;
#46610=CARTESIAN_POINT ( 'NONE',  ( 1.464175926609780648E-14, 23.87500000273118417, -5.000000000000000000 ) ) ;
#46611=ORIENTED_EDGE ( 'NONE', *, *, #31176, .F. ) ;
#46612=CARTESIAN_POINT ( 'NONE',  ( 6.123233995736766282E-16, -120.0000000000000000, -5.000000000000000000 ) ) ;
#46615=CARTESIAN_POINT ( 'NONE',  ( -4.458734124999998549, -0.2291666653010705768, 2.574251347313722516 ) ) ;
#46616=CARTESIAN_POINT ( 'NONE',  ( -2.229367062499996610, -94.39583333196773651, 3.861377020970582219 ) ) ;
#46619=CARTESIAN_POINT ( 'NONE',  ( 9.457646018065525792E-16, -20.31249999863440081, 5.148502694627439702 ) ) ;
#46625=CARTESIAN_POINT ( 'NONE',  ( -4.458734124999999437, 12.43750000136559564, 0.000000000000000000 ) ) ;
#46626=( BOUNDED_CURVE ( )  B_SPLINE_CURVE ( 2, ( #44974, #939, #35325, #20858, #40461, #41090, #31766, #16978, #21811 ),
 .UNSPECIFIED., .F., .F. ) 
 B_SPLINE_CURVE_WITH_KNOTS ( ( 3, 2, 2, 2, 3 ),
 ( 0.2946428571428571508, 0.2952380952380952439, 0.2964285714285714302, 0.2976190476190476164, 0.2982142857142857095 ),
 .UNSPECIFIED. ) 
 CURVE ( )  GEOMETRIC_REPRESENTATION_ITEM ( )  RATIONAL_B_SPLINE_CURVE ( ( 0.9330127018922194093, 0.9330127018922194093, 1.000000000000000000, 0.8660254037844387076, 1.000000000000000000, 0.8660254037844387076, 1.000000000000000000, 0.9330127018922194093, 0.9330127018922194093 ) ) 
 REPRESENTATION_ITEM ( '' )  );
#46627=ORIENTED_EDGE ( 'NONE', *, *, #56157, .F. ) ;
#46628=CARTESIAN_POINT ( 'NONE',  ( -5.000000000000000000, -52.87499999726881583, 0.000000000000000000 ) ) ;
#46630=CARTESIAN_POINT ( 'NONE',  ( 1.060575238724906964E-15, -89.74999999999998579, 5.773502691896257311 ) ) ;
#46631=CARTESIAN_POINT ( 'NONE',  ( -4.458734124999999437, -26.31249999863440792, 0.000000000000000000 ) ) ;
#46632=CARTESIAN_POINT ( 'NONE',  ( -2.229367062499996610, -68.39583333196773651, 3.861377020970582219 ) ) ;
#46636=CARTESIAN_POINT ( 'NONE',  ( -2.499999999999996447, -50.70833333060213732, 4.330127018922195425 ) ) ;
#46637=CARTESIAN_POINT ( 'NONE',  ( -6.972266317189433020E-16, -24.24999999999999645, -5.000000000000000000 ) ) ;
#46638=CARTESIAN_POINT ( 'NONE',  ( 2.229367062500001939, 7.020833334698928674, 3.861377020970579999 ) ) ;
#46639=CARTESIAN_POINT ( 'NONE',  ( 1.975475456537005874E-15, -40.62499999726879452, 5.000000000000000000 ) ) ;
#46642=CARTESIAN_POINT ( 'NONE',  ( 4.458734124999998549, -73.72916666530106511, -2.574251347313721627 ) ) ;
#46644=CARTESIAN_POINT ( 'NONE',  ( -2.499999999999996447, -1.833333333333332593, 4.330127018922195425 ) ) ;
#46647=CARTESIAN_POINT ( 'NONE',  ( 2.229367062500001939, -64.97916666530106511, 3.861377020970579999 ) ) ;
#46648=CARTESIAN_POINT ( 'NONE',  ( -3.535250795749689387E-16, -93.12499999726881583, -5.773502691896257311 ) ) ;
#46653=CARTESIAN_POINT ( 'NONE',  ( 5.000000000000000000, -48.41666666666665719, -2.886751345948129988 ) ) ;
#46654=CARTESIAN_POINT ( 'NONE',  ( -1.339745962155613812, 15.79465819873852261, -5.000000000000000000 ) ) ;
#46657=CARTESIAN_POINT ( 'NONE',  ( 4.458734125000001214, -3.145833331967738733, 2.574251347313718519 ) ) ;
#46658=( BOUNDED_CURVE ( )  B_SPLINE_CURVE ( 2, ( #21301, #39944, #54761, #54108, #10048, #29661, #10687, #416, #59592 ),
 .UNSPECIFIED., .F., .F. ) 
 B_SPLINE_CURVE_WITH_KNOTS ( ( 3, 2, 2, 2, 3 ),
 ( 0.5339285714285714191, 0.5345238095238095122, 0.5357142857142856984, 0.5369047619047618847, 0.5374999999999999778 ),
 .UNSPECIFIED. ) 
 CURVE ( )  GEOMETRIC_REPRESENTATION_ITEM ( )  RATIONAL_B_SPLINE_CURVE ( ( 0.9330127018922194093, 0.9330127018922194093, 1.000000000000000000, 0.8660254037844387076, 1.000000000000000000, 0.8660254037844387076, 1.000000000000000000, 0.9330127018922194093, 0.9330127018922194093 ) ) 
 REPRESENTATION_ITEM ( '' )  );
#46663=CARTESIAN_POINT ( 'NONE',  ( -2.500000000000000444, -5.041666663935480130, -4.330127018922193649 ) ) ;
#46667=CARTESIAN_POINT ( 'NONE',  ( 2.499999999999998668, -100.2083333306021444, -4.330127018922193649 ) ) ;
#46673=CARTESIAN_POINT ( 'NONE',  ( 4.458734125000001214, -35.14583333196772941, 2.574251347313718519 ) ) ;
#46674=CARTESIAN_POINT ( 'NONE',  ( 1.975475456537005874E-15, -10.62499999726881228, 5.000000000000000000 ) ) ;
#46681=CARTESIAN_POINT ( 'NONE',  ( 2.229367062500001939, -83.22916666530106511, 3.861377020970579999 ) ) ;
#46683=ORIENTED_EDGE ( 'NONE', *, *, #33680, .T. ) ;
#46685=LINE ( 'NONE', #51830, #55851 ) ;
#46687=EDGE_CURVE ( 'NONE', #54753, #8786, #35391, .T. ) ;
#46688=CARTESIAN_POINT ( 'NONE',  ( 4.458734125000001214, -8.145833331967736513, 2.574251347313718519 ) ) ;
#46692=CARTESIAN_POINT ( 'NONE',  ( 4.458734125000001214, -9.145833331967736513, 2.574251347313718519 ) ) ;
#46696=CARTESIAN_POINT ( 'NONE',  ( 4.458734125000000326, 27.85416666803225993, 2.574251347313718519 ) ) ;
#46698=CARTESIAN_POINT ( 'NONE',  ( 2.229367062499998831, -88.64583333196773651, -3.861377020970580887 ) ) ;
#46699=CARTESIAN_POINT ( 'NONE',  ( 1.975475456537005874E-15, -67.74999999999998579, 5.000000000000000000 ) ) ;
#46700=CARTESIAN_POINT ( 'NONE',  ( -2.229367062499996610, -10.14583333196773829, 3.861377020970582219 ) ) ;
#46701=CARTESIAN_POINT ( 'NONE',  ( 5.000000000000000000, -51.41666666666666430, -2.886751345948130876 ) ) ;
#46703=EDGE_CURVE ( 'NONE', #15515, #26615, #50873, .T. ) ;
#46705=CARTESIAN_POINT ( 'NONE',  ( -2.500000000000000444, -33.04166666393547303, -4.330127018922193649 ) ) ;
#46708=CARTESIAN_POINT ( 'NONE',  ( -3.152548672688508926E-16, 25.43750000136559208, -5.148502694627439702 ) ) ;
#46709=CARTESIAN_POINT ( 'NONE',  ( -2.480964764533239819E-13, -94.75000000000000000, 5.000000000000000000 ) ) ;
#46711=CARTESIAN_POINT ( 'NONE',  ( 4.458734124999999437, -51.81249999863440792, -5.460374474430324690E-16 ) ) ;
#46714=CARTESIAN_POINT ( 'NONE',  ( 1.060575238724906964E-15, 14.25000000000000178, 5.773502691896257311 ) ) ;
#46716=CYLINDRICAL_SURFACE ( 'NONE', #42827, 5.000000000000000000 ) ;
#46717=CARTESIAN_POINT ( 'NONE',  ( -3.152548672688508926E-16, -48.56249999863440792, -5.148502694627439702 ) ) ;
#46718=CARTESIAN_POINT ( 'NONE',  ( -5.000000000000000000, -80.95833333060214443, -2.886751345948128211 ) ) ;
#46722=CARTESIAN_POINT ( 'NONE',  ( 2.229367062499998831, -85.89583333196773651, -3.861377020970580887 ) ) ;
#46724=CARTESIAN_POINT ( 'NONE',  ( -4.999999999999999112, -32.91666666666666430, 2.886751345948131764 ) ) ;
#46725=CARTESIAN_POINT ( 'NONE',  ( -5.000000000000000000, 24.00000000000000000, 0.000000000000000000 ) ) ;
#46728=ORIENTED_EDGE ( 'NONE', *, *, #49600, .T. ) ;
#46729=CARTESIAN_POINT ( 'NONE',  ( -2.229367062499996610, -88.14583333196773651, 3.861377020970582219 ) ) ;
#46730=CARTESIAN_POINT ( 'NONE',  ( 4.458734125000001214, 15.85416666803226171, 2.574251347313718519 ) ) ;
#46731=CARTESIAN_POINT ( 'NONE',  ( 1.060575238724906964E-15, 16.37500000273118417, 5.773502691896257311 ) ) ;
#46732=CARTESIAN_POINT ( 'NONE',  ( -5.000000000000000000, -60.08333333333333570, -2.886751345948128211 ) ) ;
#46736=CARTESIAN_POINT ( 'NONE',  ( -2.500000000000000444, 14.95833333606451809, -4.330127018922193649 ) ) ;
#46737=CARTESIAN_POINT ( 'NONE',  ( -5.000000000000000000, -79.08333333333331439, -2.886751345948128211 ) ) ;
#46739=CARTESIAN_POINT ( 'NONE',  ( -4.999999999999998224, 20.08333333333333925, 2.886751345948131764 ) ) ;
#46740=CYLINDRICAL_SURFACE ( 'NONE', #32736, 5.000000000000000000 ) ;
#46741=CARTESIAN_POINT ( 'NONE',  ( 5.000000000000000000, -63.41666666666666430, -2.886751345948130876 ) ) ;
#46746=CARTESIAN_POINT ( 'NONE',  ( -3.152548672688508926E-16, -18.81249999863440792, -5.148502694627439702 ) ) ;
#46753=( BOUNDED_CURVE ( )  B_SPLINE_CURVE ( 2, ( #32228, #45763, #36429, #50590, #51859, #41553, #41878, #6850, #17128 ),
 .UNSPECIFIED., .F., .F. ) 
 B_SPLINE_CURVE_WITH_KNOTS ( ( 3, 2, 2, 2, 3 ),
 ( 0.1410714285714285698, 0.1416666666666666630, 0.1428571428571428492, 0.1440476190476190355, 0.1446428571428571563 ),
 .UNSPECIFIED. ) 
 CURVE ( )  GEOMETRIC_REPRESENTATION_ITEM ( )  RATIONAL_B_SPLINE_CURVE ( ( 0.9330127018922194093, 0.9330127018922194093, 1.000000000000000000, 0.8660254037844387076, 1.000000000000000000, 0.8660254037844387076, 1.000000000000000000, 0.9330127018922178550, 0.9330127018922194093 ) ) 
 REPRESENTATION_ITEM ( '' )  );
#46755=EDGE_LOOP ( 'NONE', ( #25726, #7854, #43594, #32856 ) ) ;
#46758=CARTESIAN_POINT ( 'NONE',  ( -4.458734124999998549, -60.47916666530105800, 2.574251347313722516 ) ) ;
#46759=CARTESIAN_POINT ( 'NONE',  ( -6.972266317189433020E-16, -25.24999999999999645, -5.000000000000000000 ) ) ;
#46760=FILL_AREA_STYLE_COLOUR ( '', #23560 ) ;
#46768=ORIENTED_EDGE ( 'NONE', *, *, #50698, .F. ) ;
#46770=CARTESIAN_POINT ( 'NONE',  ( -4.458734124999999437, 6.604166668032259047, -2.574251347313719407 ) ) ;
#46775=ORIENTED_EDGE ( 'NONE', *, *, #5800, .F. ) ;
#46776=CARTESIAN_POINT ( 'NONE',  ( -4.458734124999999437, -68.39583333196773651, -2.574251347313719407 ) ) ;
#46777=CARTESIAN_POINT ( 'NONE',  ( 1.339745962155612702, -10.16965819600733312, -5.000000000000000000 ) ) ;
#46778=CARTESIAN_POINT ( 'NONE',  ( -4.458734124999999437, 11.60416666803225993, -2.574251347313719407 ) ) ;
#46779=CARTESIAN_POINT ( 'NONE',  ( -1.339745962155610925, -41.79465819873852439, 5.000000000000000000 ) ) ;
#46780=CARTESIAN_POINT ( 'NONE',  ( 4.458734125000001214, -60.14583333196774362, 2.574251347313718519 ) ) ;
#46781=CARTESIAN_POINT ( 'NONE',  ( 1.060575238724906964E-15, -16.62499999726881583, 5.773502691896257311 ) ) ;
#46783=CARTESIAN_POINT ( 'NONE',  ( 0.000000000000000000, -120.0000000000000000, 5.000000000000000000 ) ) ;
#46784=CARTESIAN_POINT ( 'NONE',  ( 0.000000000000000000, -120.0000000000000000, 0.000000000000000000 ) ) ;
#46785=DIRECTION ( 'NONE',  ( -0.000000000000000000, 1.000000000000000000, -0.000000000000000000 ) ) ;
#46786=CARTESIAN_POINT ( 'NONE',  ( 4.458734124999999437, -33.81249999863440792, -5.460374474430324690E-16 ) ) ;
#46788=CARTESIAN_POINT ( 'NONE',  ( -2.229367062500000163, -23.72916666530107577, -3.861377020970580443 ) ) ;
#46789=ORIENTED_EDGE ( 'NONE', *, *, #58568, .T. ) ;
#46790=CARTESIAN_POINT ( 'NONE',  ( -6.972266317189433020E-16, -102.2499999999999858, -5.000000000000000000 ) ) ;
#46791=CARTESIAN_POINT ( 'NONE',  ( -4.458734124999999437, -109.3958333319677507, -2.574251347313719407 ) ) ;
#46794=CARTESIAN_POINT ( 'NONE',  ( -4.458734124999999437, -103.6458333319677223, -2.574251347313719407 ) ) ;
#46795=CARTESIAN_POINT ( 'NONE',  ( 4.458734125000001214, -24.89583333196773651, 2.574251347313718519 ) ) ;
#46796=CARTESIAN_POINT ( 'NONE',  ( -2.500000000000000444, -64.04166666393547303, -4.330127018922193649 ) ) ;
#46799=CARTESIAN_POINT ( 'NONE',  ( 9.457646018065525792E-16, -31.06249999863440436, 5.148502694627439702 ) ) ;
#46800=CARTESIAN_POINT ( 'NONE',  ( 4.458734124999999437, -72.06249999863439371, -5.460374474430324690E-16 ) ) ;
#46801=CARTESIAN_POINT ( 'NONE',  ( 1.975475456537005874E-15, -39.62499999726880162, 5.000000000000000000 ) ) ;
#46805=CARTESIAN_POINT ( 'NONE',  ( -5.000000000000000000, -16.00000000000000000, 0.000000000000000000 ) ) ;
#46807=ORIENTED_EDGE ( 'NONE', *, *, #52658, .F. ) ;
#46808=DIRECTION ( 'NONE',  ( 0.000000000000000000, 0.000000000000000000, 1.000000000000000000 ) ) ;
#46811=CARTESIAN_POINT ( 'NONE',  ( -4.999999999999998224, -2.791666663935478354, 2.886751345948131764 ) ) ;
#46814=EDGE_CURVE ( 'NONE', #56685, #59581, #23460, .T. ) ;
#46818=CARTESIAN_POINT ( 'NONE',  ( -5.000000000000000000, -80.87499999726881583, 0.000000000000000000 ) ) ;
#46819=LINE ( 'NONE', #2763, #46839 ) ;
#46823=CARTESIAN_POINT ( 'NONE',  ( -5.000000000000000000, -29.87499999726881228, 0.000000000000000000 ) ) ;
#46824=ORIENTED_EDGE ( 'NONE', *, *, #11313, .T. ) ;
#46831=ORIENTED_EDGE ( 'NONE', *, *, #20941, .T. ) ;
#46834=CARTESIAN_POINT ( 'NONE',  ( -2.499999999999996447, -50.70833333060213732, 4.330127018922195425 ) ) ;
#46837=CARTESIAN_POINT ( 'NONE',  ( -4.999999999999998224, 21.08333333333333215, 2.886751345948131764 ) ) ;
#46839=VECTOR ( 'NONE', #26452, 1000.000000000000000 ) ;
#46842=CARTESIAN_POINT ( 'NONE',  ( -2.229367062499996610, -79.14583333196773651, 3.861377020970582219 ) ) ;
#46843=CARTESIAN_POINT ( 'NONE',  ( 2.229367062500001939, 22.02083333469892779, 3.861377020970579999 ) ) ;
#46846=CARTESIAN_POINT ( 'NONE',  ( 5.000000000000000000, 14.49999999999999822, -6.123233995736766282E-16 ) ) ;
#46850=CARTESIAN_POINT ( 'NONE',  ( 5.000000000000000000, -74.29166666393547303, -2.886751345948130876 ) ) ;
#46854=CARTESIAN_POINT ( 'NONE',  ( -2.229367062500000163, -52.47916666530107221, -3.861377020970580443 ) ) ;
#46856=FACE_OUTER_BOUND ( 'NONE', #42637, .T. ) ;
#46857=EDGE_CURVE ( 'NONE', #14691, #2195, #22519, .T. ) ;
#46859=CARTESIAN_POINT ( 'NONE',  ( -2.500000000000000444, -109.1666666666666572, -4.330127018922193649 ) ) ;
#46860=LINE ( 'NONE', #2805, #45311 ) ;
#46861=CARTESIAN_POINT ( 'NONE',  ( -2.229367062499996610, -38.39583333196773651, 3.861377020970582219 ) ) ;
#46862=CARTESIAN_POINT ( 'NONE',  ( -5.000000000000000000, 2.125000002731185056, 0.000000000000000000 ) ) ;
#46868=CARTESIAN_POINT ( 'NONE',  ( 9.457646018065525792E-16, -102.0624999986344079, 5.148502694627439702 ) ) ;
#46869=CARTESIAN_POINT ( 'NONE',  ( 4.458734124999999437, -4.062499998634408804, -5.460374474430324690E-16 ) ) ;
#46870=ORIENTED_EDGE ( 'NONE', *, *, #24061, .T. ) ;
#46872=LINE ( 'NONE', #41080, #30849 ) ;
#46873=CARTESIAN_POINT ( 'NONE',  ( -2.229367062500000163, -93.47916666530106511, -3.861377020970580443 ) ) ;
#46874=EDGE_CURVE ( 'NONE', #55713, #39107, #55386, .T. ) ;
#46876=CARTESIAN_POINT ( 'NONE',  ( 2.229367062499998831, -86.89583333196773651, -3.861377020970580887 ) ) ;
#46880=CARTESIAN_POINT ( 'NONE',  ( 2.229367062499998831, -11.64583333196774007, -3.861377020970580887 ) ) ;
#46881=CARTESIAN_POINT ( 'NONE',  ( 2.229367062500001939, 18.77083333469892779, 3.861377020970579999 ) ) ;
#46882=CARTESIAN_POINT ( 'NONE',  ( 9.457646018065525792E-16, -52.31249999863440792, 5.148502694627439702 ) ) ;
#46886=CARTESIAN_POINT ( 'NONE',  ( 2.499999999999998668, -106.2083333306021444, -4.330127018922193649 ) ) ;
#46887=VERTEX_POINT ( 'NONE', #27015 ) ;
#46891=CARTESIAN_POINT ( 'NONE',  ( 1.339745962155616255, 26.83034180399266333, -4.999999999999997335 ) ) ;
#46892=CARTESIAN_POINT ( 'NONE',  ( 4.458734124999999437, -79.81249999863440792, -5.460374474430324690E-16 ) ) ;
#46893=CARTESIAN_POINT ( 'NONE',  ( -4.458734124999999437, 22.35416666803225638, -2.574251347313719407 ) ) ;
#46894=CIRCLE ( 'NONE', #38644, 5.000000000000000000 ) ;
#46899=LINE ( 'NONE', #7981, #57405 ) ;
#46901=CARTESIAN_POINT ( 'NONE',  ( 5.000000000000000888, -64.58333333333332860, 2.886751345948126879 ) ) ;
#46902=CARTESIAN_POINT ( 'NONE',  ( -6.972266317189433020E-16, -63.12499999726880162, -5.000000000000000000 ) ) ;
#46906=CARTESIAN_POINT ( 'NONE',  ( -4.999999999999998224, 28.08333333333332860, 2.886751345948131764 ) ) ;
#46907=CYLINDRICAL_SURFACE ( 'NONE', #34751, 5.000000000000000000 ) ;
#46919=CARTESIAN_POINT ( 'NONE',  ( 9.457646018065525792E-16, -53.31249999863441502, 5.148502694627439702 ) ) ;
#46928=CARTESIAN_POINT ( 'NONE',  ( 4.458734125000001214, -99.14583333196773651, 2.574251347313718519 ) ) ;
#46929=CARTESIAN_POINT ( 'NONE',  ( 1.975475456537005874E-15, -2.750000000000000888, 5.000000000000000000 ) ) ;
#46934=VECTOR ( 'NONE', #469, 1000.000000000000000 ) ;
#46935=CARTESIAN_POINT ( 'NONE',  ( 4.458734124999999437, -8.812499998634406140, -5.460374474430324690E-16 ) ) ;
#46937=( BOUNDED_CURVE ( )  B_SPLINE_CURVE ( 2, ( #2264, #11566, #16402, #22184, #36654, #55652, #56283, #31186, #32455 ),
 .UNSPECIFIED., .F., .F. ) 
 B_SPLINE_CURVE_WITH_KNOTS ( ( 3, 2, 2, 2, 3 ),
 ( 0.7303571428571428159, 0.7309523809523809090, 0.7321428571428570953, 0.7333333333333332815, 0.7339285714285714857 ),
 .UNSPECIFIED. ) 
 CURVE ( )  GEOMETRIC_REPRESENTATION_ITEM ( )  RATIONAL_B_SPLINE_CURVE ( ( 0.9330127018922194093, 0.9330127018922194093, 1.000000000000000000, 0.8660254037844387076, 1.000000000000000000, 0.8660254037844387076, 1.000000000000000000, 0.9330127018922130810, 0.9330127018922194093 ) ) 
 REPRESENTATION_ITEM ( '' )  );
#46938=CARTESIAN_POINT ( 'NONE',  ( -3.152548672688508926E-16, -93.81249999863440792, -5.148502694627439702 ) ) ;
#46940=CARTESIAN_POINT ( 'NONE',  ( 2.229367062500001939, -20.22916666530107221, 3.861377020970579999 ) ) ;
#46941=AXIS2_PLACEMENT_3D ( 'NONE', #35015, #39817, #287 ) ;
#46942=CARTESIAN_POINT ( 'NONE',  ( 1.975475456537005874E-15, -6.624999997268813168, 5.000000000000000000 ) ) ;
#46946=CARTESIAN_POINT ( 'NONE',  ( 2.500000000000002220, -70.66666666666667140, 4.330127018922192761 ) ) ;
#46947=CARTESIAN_POINT ( 'NONE',  ( -2.499999999999996447, -33.83333333333332860, 4.330127018922195425 ) ) ;
#46949=CARTESIAN_POINT ( 'NONE',  ( 4.458734124999999437, 12.93750000136559208, -5.460374474430324690E-16 ) ) ;
#46951=CARTESIAN_POINT ( 'NONE',  ( -1.339745962155613812, -5.205341801261476498, -5.000000000000000000 ) ) ;
#46953=CARTESIAN_POINT ( 'NONE',  ( 2.499999999999998668, -89.33333333333332860, -4.330127018922193649 ) ) ;
#46954=CARTESIAN_POINT ( 'NONE',  ( 2.229367062499998831, -24.64583333196773651, -3.861377020970580887 ) ) ;
#46956=CARTESIAN_POINT ( 'NONE',  ( -2.229367062499996610, -72.39583333196773651, 3.861377020970582219 ) ) ;
#46958=CARTESIAN_POINT ( 'NONE',  ( 6.123233995736766282E-16, -120.0000000000000000, -5.000000000000000000 ) ) ;
#46962=CARTESIAN_POINT ( 'NONE',  ( 4.458734124999999437, 6.187500001365593860, -5.460374474430324690E-16 ) ) ;
#46963=DIRECTION ( 'NONE',  ( -0.000000000000000000, 1.000000000000000000, -0.000000000000000000 ) ) ;
#46966=CARTESIAN_POINT ( 'NONE',  ( 9.457646018065525792E-16, -72.06249999863439371, 5.148502694627439702 ) ) ;
#46968=CARTESIAN_POINT ( 'NONE',  ( -5.000000000000000000, -2.000000000000001776, 0.000000000000000000 ) ) ;
#46970=CARTESIAN_POINT ( 'NONE',  ( -3.152548672688508926E-16, -64.56249999863440792, -5.148502694627439702 ) ) ;
#46971=CARTESIAN_POINT ( 'NONE',  ( 2.500000000000002220, -102.5416666639354588, 4.330127018922192761 ) ) ;
#46972=FACE_OUTER_BOUND ( 'NONE', #29715, .T. ) ;
#46974=DIRECTION ( 'NONE',  ( -0.000000000000000000, -1.000000000000000000, -0.000000000000000000 ) ) ;
#46976=CARTESIAN_POINT ( 'NONE',  ( -2.500000000000000444, -46.16666666666666430, -4.330127018922193649 ) ) ;
#46977=CARTESIAN_POINT ( 'NONE',  ( -2.500000000000000444, 26.83333333333333570, -4.330127018922193649 ) ) ;
#46978=CARTESIAN_POINT ( 'NONE',  ( 1.975475456537005874E-15, 16.24999999999999645, 5.000000000000000000 ) ) ;
#46980=CARTESIAN_POINT ( 'NONE',  ( 1.339745962155499015, -94.70534180126146850, 5.000000000000065725 ) ) ;
#46981=AXIS2_PLACEMENT_3D ( 'NONE', #27706, #47333, #37671 ) ;
#46987=EDGE_LOOP ( 'NONE', ( #6655, #55971, #39777, #15877 ) ) ;
#46990=ORIENTED_EDGE ( 'NONE', *, *, #30719, .F. ) ;
#46995=CARTESIAN_POINT ( 'NONE',  ( -2.229367062500000163, -34.72916666530107221, -3.861377020970580443 ) ) ;
#47004=CARTESIAN_POINT ( 'NONE',  ( -4.458734124999999437, -83.64583333196773651, -2.574251347313719407 ) ) ;
#47006=VERTEX_POINT ( 'NONE', #5412 ) ;
#47008=FACE_OUTER_BOUND ( 'NONE', #59590, .T. ) ;
#47010=CARTESIAN_POINT ( 'NONE',  ( -4.458734124999997661, -38.22916666530107932, 2.574251347313722516 ) ) ;
#47011=CARTESIAN_POINT ( 'NONE',  ( -2.229367062500000163, -9.729166665301068662, -3.861377020970580443 ) ) ;
#47012=ORIENTED_EDGE ( 'NONE', *, *, #3527, .F. ) ;
#47014=LINE ( 'NONE', #27702, #26536 ) ;
#47015=CARTESIAN_POINT ( 'NONE',  ( 4.458734124999999437, -9.062499998634406140, -5.460374474430324690E-16 ) ) ;
#47021=CARTESIAN_POINT ( 'NONE',  ( -4.458734124999999437, 27.35416666803225993, -2.574251347313719407 ) ) ;
#47023=CARTESIAN_POINT ( 'NONE',  ( 4.458734125000000326, -86.89583333196773651, 2.574251347313718519 ) ) ;
#47025=CARTESIAN_POINT ( 'NONE',  ( 4.458734125000001214, -10.89583333196773651, 2.574251347313718519 ) ) ;
#47027=CARTESIAN_POINT ( 'NONE',  ( 0.000000000000000000, -120.0000000000000000, 0.000000000000000000 ) ) ;
#47028=CARTESIAN_POINT ( 'NONE',  ( -3.535250795749689387E-16, -34.12499999726881583, -5.773502691896257311 ) ) ;
#47030=CARTESIAN_POINT ( 'NONE',  ( -2.229367062499996610, 24.85416666803225993, 3.861377020970582219 ) ) ;
#47031=CARTESIAN_POINT ( 'NONE',  ( -4.999999999999998224, -97.79166666393545881, 2.886751345948131764 ) ) ;
#47033=CARTESIAN_POINT ( 'NONE',  ( -4.458734124999999437, -58.39583333196774362, -2.574251347313719407 ) ) ;
#47036=CARTESIAN_POINT ( 'NONE',  ( -1.339745962155613812, -18.20534180126147916, -5.000000000000000000 ) ) ;
#47037=CARTESIAN_POINT ( 'NONE',  ( -2.500000000000000444, 17.83333333333333215, -4.330127018922193649 ) ) ;
#47039=CARTESIAN_POINT ( 'NONE',  ( 5.000000000000000000, -69.49999999999998579, -6.123233995736766282E-16 ) ) ;
#47040=CARTESIAN_POINT ( 'NONE',  ( 4.458734125000001214, -48.89583333196772941, 2.574251347313718519 ) ) ;
#47041=CARTESIAN_POINT ( 'NONE',  ( 5.000000000000000888, -84.45833333060214443, 2.886751345948126879 ) ) ;
#47043=CARTESIAN_POINT ( 'NONE',  ( 5.000000000000000000, -37.29166666393548724, -2.886751345948130876 ) ) ;
#47044=CARTESIAN_POINT ( 'NONE',  ( 5.000000000000000000, -36.41666666666666430, -2.886751345948130876 ) ) ;
#47045=CARTESIAN_POINT ( 'NONE',  ( -3.152548672688508926E-16, -85.81249999863440792, -5.148502694627439702 ) ) ;
#47047=CARTESIAN_POINT ( 'NONE',  ( 2.499999999999998668, -31.33333333333333215, -4.330127018922193649 ) ) ;
#47052=CARTESIAN_POINT ( 'NONE',  ( -3.152548672688508926E-16, -93.56249999863439371, -5.148502694627439702 ) ) ;
#47053=CARTESIAN_POINT ( 'NONE',  ( -4.458734124999998549, 13.52083333469892779, 2.574251347313722516 ) ) ;
#47054=CARTESIAN_POINT ( 'NONE',  ( -2.500000000000000444, 18.95833333606451632, -4.330127018922193649 ) ) ;
#47055=CARTESIAN_POINT ( 'NONE',  ( -4.999999999999998224, -59.91666666666665719, 2.886751345948131764 ) ) ;
#47059=CARTESIAN_POINT ( 'NONE',  ( -5.000000000000000000, 15.04166666939785202, -2.886751345948128211 ) ) ;
#47060=CARTESIAN_POINT ( 'NONE',  ( -2.499999999999996447, -79.83333333333332860, 4.330127018922195425 ) ) ;
#47063=CARTESIAN_POINT ( 'NONE',  ( -4.999999999999998224, -12.79166666393547835, 2.886751345948131764 ) ) ;
#47064=CARTESIAN_POINT ( 'NONE',  ( 3.044556291839386294E-14, 17.87500000273118417, -5.000000000000000000 ) ) ;
#47067=CARTESIAN_POINT ( 'NONE',  ( -2.500000000000000444, 13.83333333333333215, -4.330127018922193649 ) ) ;
#47068=CARTESIAN_POINT ( 'NONE',  ( 2.229367062500001939, -21.22916666530107221, 3.861377020970579999 ) ) ;
#47069=AXIS2_PLACEMENT_3D ( 'NONE', #3351, #22968, #18124 ) ;
#47070=CARTESIAN_POINT ( 'NONE',  ( 5.000000000000000888, -107.4583333306021586, 2.886751345948126879 ) ) ;
#47079=CARTESIAN_POINT ( 'NONE',  ( 5.000000000000000000, -85.37499999726880162, -6.123233995736766282E-16 ) ) ;
#47081=CARTESIAN_POINT ( 'NONE',  ( 4.458734124999999437, -68.06249999863440792, -5.460374474430324690E-16 ) ) ;
#47085=CARTESIAN_POINT ( 'NONE',  ( -1.339745962155613146, 27.33034180399266333, 5.000000000000000000 ) ) ;
#47091=CARTESIAN_POINT ( 'NONE',  ( -4.458734124999998549, 8.770833334698927786, 2.574251347313722516 ) ) ;
#47094=CARTESIAN_POINT ( 'NONE',  ( 1.339745962155612702, -108.1696581960073189, -5.000000000000000000 ) ) ;
#47095=CARTESIAN_POINT ( 'NONE',  ( 0.000000000000000000, -120.0000000000000000, 0.000000000000000000 ) ) ;
#47097=CARTESIAN_POINT ( 'NONE',  ( -3.152548672688508926E-16, -68.56249999863439371, -5.148502694627439702 ) ) ;
#47098=CARTESIAN_POINT ( 'NONE',  ( 4.458734124999998549, 5.270833334698926897, -2.574251347313721627 ) ) ;
#47099=CARTESIAN_POINT ( 'NONE',  ( -5.000000000000000000, -89.08333333333332860, -2.886751345948128211 ) ) ;
#47100=CARTESIAN_POINT ( 'NONE',  ( 4.458734124999998549, -58.97916666530105800, -2.574251347313721627 ) ) ;
#47101=CARTESIAN_POINT ( 'NONE',  ( 5.000000000000000888, -19.45833333060214798, 2.886751345948126879 ) ) ;
#47102=CARTESIAN_POINT ( 'NONE',  ( -4.999999999999998224, -32.79166666393547303, 2.886751345948131764 ) ) ;
#47103=CARTESIAN_POINT ( 'NONE',  ( -5.000000000000000000, -44.95833333060214443, -2.886751345948128211 ) ) ;
#47104=CARTESIAN_POINT ( 'NONE',  ( 0.000000000000000000, -114.9999999999999858, 5.000000000000000000 ) ) ;
#47106=CARTESIAN_POINT ( 'NONE',  ( -4.458734124999999437, -39.31249999863440081, 0.000000000000000000 ) ) ;
#47107=CARTESIAN_POINT ( 'NONE',  ( -2.229367062499996610, -22.39583333196773651, 3.861377020970582219 ) ) ;
#47108=EDGE_LOOP ( 'NONE', ( #59746, #6569, #2054, #28707 ) ) ;
#47109=AXIS2_PLACEMENT_3D ( 'NONE', #61190, #17112, #20991 ) ;
#47111=CARTESIAN_POINT ( 'NONE',  ( 5.000000000000000000, 28.58333333333333215, -2.886751345948129988 ) ) ;
#47113=ORIENTED_EDGE ( 'NONE', *, *, #18185, .F. ) ;
#47114=CARTESIAN_POINT ( 'NONE',  ( -3.152548672688508926E-16, -108.8124999986343937, -5.148502694627439702 ) ) ;
#47115=CARTESIAN_POINT ( 'NONE',  ( -2.229367062499996610, -34.14583333196772941, 3.861377020970582219 ) ) ;
#47116=CARTESIAN_POINT ( 'NONE',  ( 1.060575238724906964E-15, -63.62499999726881583, 5.773502691896257311 ) ) ;
#47120=CARTESIAN_POINT ( 'NONE',  ( -2.229367062500000163, -30.47916666530107221, -3.861377020970580443 ) ) ;
#47121=CARTESIAN_POINT ( 'NONE',  ( 4.458734125000000326, -71.14583333196773651, 2.574251347313718519 ) ) ;
#47126=CARTESIAN_POINT ( 'NONE',  ( -2.500000000000000444, -18.16666666666666430, -4.330127018922193649 ) ) ;
#47128=ORIENTED_EDGE ( 'NONE', *, *, #29898, .T. ) ;
#47131=CARTESIAN_POINT ( 'NONE',  ( -1.339745962155610925, -86.66965819600733312, 5.000000000000000000 ) ) ;
#47134=EDGE_CURVE ( 'NONE', #1494, #25237, #5095, .T. ) ;
#47135=AXIS2_PLACEMENT_3D ( 'NONE', #28442, #48057, #450 ) ;
#47138=( BOUNDED_CURVE ( )  B_SPLINE_CURVE ( 2, ( #59846, #16726, #55007, #40522, #5480, #26059, #30227, #36342, #16410 ),
 .UNSPECIFIED., .F., .F. ) 
 B_SPLINE_CURVE_WITH_KNOTS ( ( 3, 2, 2, 2, 3 ),
 ( 0.3624999999999999889, 0.3630952380952380820, 0.3642857142857142683, 0.3654761904761904545, 0.3660714285714285476 ),
 .UNSPECIFIED. ) 
 CURVE ( )  GEOMETRIC_REPRESENTATION_ITEM ( )  RATIONAL_B_SPLINE_CURVE ( ( 0.9330127018922194093, 0.9330127018922194093, 1.000000000000000000, 0.8660254037844387076, 1.000000000000000000, 0.8660254037844387076, 1.000000000000000000, 0.9330127018922194093, 0.9330127018922194093 ) ) 
 REPRESENTATION_ITEM ( '' )  );
#47139=DIRECTION ( 'NONE',  ( -0.000000000000000000, 1.000000000000000000, -0.000000000000000000 ) ) ;
#47145=DIRECTION ( 'NONE',  ( 0.000000000000000000, 0.000000000000000000, 1.000000000000000000 ) ) ;
#47148=ADVANCED_FACE ( 'NONE', ( #38541 ), #24713, .T. ) ;
#47150=ORIENTED_EDGE ( 'NONE', *, *, #18533, .F. ) ;
#47152=EDGE_CURVE ( 'NONE', #22810, #35769, #31137, .T. ) ;
#47154=CARTESIAN_POINT ( 'NONE',  ( -2.499999999999996447, -11.83333333333333393, 4.330127018922195425 ) ) ;
#47164=CARTESIAN_POINT ( 'NONE',  ( 4.458734125000001214, -84.89583333196773651, 2.574251347313718519 ) ) ;
#47165=CARTESIAN_POINT ( 'NONE',  ( 2.229367062500001939, 24.02083333469892779, 3.861377020970579999 ) ) ;
#47167=ORIENTED_EDGE ( 'NONE', *, *, #58893, .T. ) ;
#47168=CARTESIAN_POINT ( 'NONE',  ( 1.975475456537005874E-15, -69.62499999726880162, 5.000000000000000000 ) ) ;
#47174=CARTESIAN_POINT ( 'NONE',  ( 2.229367062500001939, -55.97916666530107221, 3.861377020970579999 ) ) ;
#47175=CARTESIAN_POINT ( 'NONE',  ( 2.499999999999998668, 21.66666666666666785, -4.330127018922193649 ) ) ;
#47176=CARTESIAN_POINT ( 'NONE',  ( 4.458734124999998549, 24.27083333469892779, -2.574251347313721627 ) ) ;
#47177=CARTESIAN_POINT ( 'NONE',  ( -3.535250795749689387E-16, -106.2499999999999858, -5.773502691896257311 ) ) ;
#47179=CARTESIAN_POINT ( 'NONE',  ( 4.458734124999998549, -45.97916666530106511, -2.574251347313721627 ) ) ;
#47180=EDGE_CURVE ( 'NONE', #48706, #28142, #63644, .T. ) ;
#47181=CARTESIAN_POINT ( 'NONE',  ( -2.500000000000000444, 0.9583333360645186483, -4.330127018922193649 ) ) ;
#47185=CARTESIAN_POINT ( 'NONE',  ( 4.458734124999998549, -102.7291666653010651, -2.574251347313721627 ) ) ;
#47186=CARTESIAN_POINT ( 'NONE',  ( 2.229367062499998831, -3.895833331967739177, -3.861377020970580887 ) ) ;
#47187=( BOUNDED_CURVE ( )  B_SPLINE_CURVE ( 2, ( #61269, #46779, #17191, #22666, #57705, #2412, #17522, #37141, #26855 ),
 .UNSPECIFIED., .F., .F. ) 
 B_SPLINE_CURVE_WITH_KNOTS ( ( 3, 2, 2, 2, 3 ),
 ( 0.5124999999999999556, 0.5130952380952380487, 0.5142857142857142350, 0.5154761904761904212, 0.5160714285714286254 ),
 .UNSPECIFIED. ) 
 CURVE ( )  GEOMETRIC_REPRESENTATION_ITEM ( )  RATIONAL_B_SPLINE_CURVE ( ( 0.9330127018922194093, 0.9330127018922194093, 1.000000000000000000, 0.8660254037844387076, 1.000000000000000000, 0.8660254037844387076, 1.000000000000000000, 0.9330127018922130810, 0.9330127018922194093 ) ) 
 REPRESENTATION_ITEM ( '' )  );
#47188=ORIENTED_EDGE ( 'NONE', *, *, #16664, .F. ) ;
#47189=CARTESIAN_POINT ( 'NONE',  ( -6.972266317189433020E-16, -86.12499999726880162, -5.000000000000000000 ) ) ;
#47190=CARTESIAN_POINT ( 'NONE',  ( 2.229367062499998831, -94.64583333196773651, -3.861377020970580887 ) ) ;
#47192=CARTESIAN_POINT ( 'NONE',  ( -2.229367062500000163, -85.72916666530107932, -3.861377020970580443 ) ) ;
#47194=LINE ( 'NONE', #7013, #14040 ) ;
#47196=CARTESIAN_POINT ( 'NONE',  ( 4.458734125000000326, -12.89583333196774362, 2.574251347313718519 ) ) ;
#47197=CARTESIAN_POINT ( 'NONE',  ( -2.229367062499996610, 14.60416666803226171, 3.861377020970582219 ) ) ;
#47198=CARTESIAN_POINT ( 'NONE',  ( -2.229367062499996610, -52.39583333196773651, 3.861377020970582219 ) ) ;
#47199=CARTESIAN_POINT ( 'NONE',  ( -2.499999999999996447, 17.29166666939785557, 4.330127018922195425 ) ) ;
#47202=CARTESIAN_POINT ( 'NONE',  ( -1.339745962155613812, -39.20534180126147561, -5.000000000000000000 ) ) ;
#47203=ORIENTED_EDGE ( 'NONE', *, *, #18045, .T. ) ;
#47207=CARTESIAN_POINT ( 'NONE',  ( 5.000000000000000000, -68.49999999999998579, -6.123233995736766282E-16 ) ) ;
#47208=CARTESIAN_POINT ( 'NONE',  ( 9.457646018065525792E-16, -78.06249999863440792, 5.148502694627439702 ) ) ;
#47209=CARTESIAN_POINT ( 'NONE',  ( -4.458734124999998549, 25.52083333469893134, 2.574251347313722516 ) ) ;
#47216=CARTESIAN_POINT ( 'NONE',  ( 2.499999999999998668, -68.33333333333332860, -4.330127018922193649 ) ) ;
#47219=VERTEX_POINT ( 'NONE', #25675 ) ;
#47220=CARTESIAN_POINT ( 'NONE',  ( -1.339745962155613812, -62.08034179853028434, -5.000000000000000000 ) ) ;
#47221=CARTESIAN_POINT ( 'NONE',  ( 6.158835246850667461E-14, 8.749999999999998224, -4.999999999999999112 ) ) ;
#47222=CARTESIAN_POINT ( 'NONE',  ( 1.339745962155612702, -40.29465819873851729, -5.000000000000000000 ) ) ;
#47225=CARTESIAN_POINT ( 'NONE',  ( 5.000000000000000888, -62.58333333333333570, 2.886751345948126879 ) ) ;
#47229=ORIENTED_EDGE ( 'NONE', *, *, #17017, .F. ) ;
#47233=ORIENTED_EDGE ( 'NONE', *, *, #10339, .T. ) ;
#47236=CARTESIAN_POINT ( 'NONE',  ( 2.229367062499998831, -50.89583333196772941, -3.861377020970580887 ) ) ;
#47246=CARTESIAN_POINT ( 'NONE',  ( 4.458734124999998549, -97.97916666530105090, -2.574251347313721627 ) ) ;
#47248=ORIENTED_EDGE ( 'NONE', *, *, #49885, .F. ) ;
#47253=CARTESIAN_POINT ( 'NONE',  ( -4.458734124999998549, -9.229166665301068662, 2.574251347313722516 ) ) ;
#47254=CARTESIAN_POINT ( 'NONE',  ( -4.458734124999999437, -96.56249999863440792, 0.000000000000000000 ) ) ;
#47256=CARTESIAN_POINT ( 'NONE',  ( 9.457646018065525792E-16, -26.31249999863440792, 5.148502694627439702 ) ) ;
#47257=CARTESIAN_POINT ( 'NONE',  ( 1.975475456537005874E-15, -92.62499999726881583, 5.000000000000000000 ) ) ;
#47263=CARTESIAN_POINT ( 'NONE',  ( -4.458734124999999437, 8.437500001365595637, 0.000000000000000000 ) ) ;
#47264=VERTEX_POINT ( 'NONE', #6381 ) ;
#47265=CARTESIAN_POINT ( 'NONE',  ( -2.499999999999996447, -52.70833333060213732, 4.330127018922195425 ) ) ;
#47266=CARTESIAN_POINT ( 'NONE',  ( 1.975475456537005874E-15, -66.62499999726881583, 5.000000000000000000 ) ) ;
#47267=CARTESIAN_POINT ( 'NONE',  ( 2.500000000000002220, -88.66666666666665719, 4.330127018922192761 ) ) ;
#47268=CARTESIAN_POINT ( 'NONE',  ( 4.458734124999998549, -26.72916666530106866, -2.574251347313721627 ) ) ;
#47269=CARTESIAN_POINT ( 'NONE',  ( -2.229367062500000163, -69.72916666530107932, -3.861377020970580443 ) ) ;
#47273=CARTESIAN_POINT ( 'NONE',  ( 4.458734125000000326, 1.104166668032261711, 2.574251347313718519 ) ) ;
#47277=CARTESIAN_POINT ( 'NONE',  ( -4.458734124999998549, -70.22916666530107932, 2.574251347313722516 ) ) ;
#47279=CARTESIAN_POINT ( 'NONE',  ( -5.000000000000000000, -5.083333333333334814, -2.886751345948128211 ) ) ;
#47282=CARTESIAN_POINT ( 'NONE',  ( 4.458734125000001214, -63.89583333196772941, 2.574251347313718519 ) ) ;
#47283=CARTESIAN_POINT ( 'NONE',  ( -5.000000000000000000, -99.87499999726881583, 0.000000000000000000 ) ) ;
#47286=ADVANCED_FACE ( 'NONE', ( #50746 ), #25029, .T. ) ;
#47287=CARTESIAN_POINT ( 'NONE',  ( -4.458734124999999437, -103.5624999986344079, 0.000000000000000000 ) ) ;
#47289=CARTESIAN_POINT ( 'NONE',  ( 2.499999999999998668, -46.33333333333333570, -4.330127018922193649 ) ) ;
#47292=ORIENTED_EDGE ( 'NONE', *, *, #6777, .T. ) ;
#47306=ADVANCED_FACE ( 'NONE', ( #26296 ), #25348, .T. ) ;
#47308=CARTESIAN_POINT ( 'NONE',  ( -4.458734124999999437, -33.56249999863440792, 0.000000000000000000 ) ) ;
#47313=CYLINDRICAL_SURFACE ( 'NONE', #53895, 5.000000000000000000 ) ;
#47317=( BOUNDED_CURVE ( )  B_SPLINE_CURVE ( 2, ( #58540, #24439, #34084, #59174, #39536, #40190, #15108, #6107, #10591 ),
 .UNSPECIFIED., .F., .F. ) 
 B_SPLINE_CURVE_WITH_KNOTS ( ( 3, 2, 2, 2, 3 ),
 ( 0.8517857142857142572, 0.8523809523809523503, 0.8535714285714285365, 0.8547619047619047228, 0.8553571428571428159 ),
 .UNSPECIFIED. ) 
 CURVE ( )  GEOMETRIC_REPRESENTATION_ITEM ( )  RATIONAL_B_SPLINE_CURVE ( ( 0.9330127018922194093, 0.9330127018922194093, 1.000000000000000000, 0.8660254037844387076, 1.000000000000000000, 0.8660254037844387076, 1.000000000000000000, 0.9330127018922194093, 0.9330127018922194093 ) ) 
 REPRESENTATION_ITEM ( '' )  );
#47319=CARTESIAN_POINT ( 'NONE',  ( 2.500000000000002220, -54.66666666666667140, 4.330127018922192761 ) ) ;
#47320=CARTESIAN_POINT ( 'NONE',  ( 4.458734124999999437, -83.06249999863440792, -5.460374474430324690E-16 ) ) ;
#47324=CYLINDRICAL_SURFACE ( 'NONE', #382, 5.000000000000000000 ) ;
#47326=CARTESIAN_POINT ( 'NONE',  ( -4.458734124999999437, -6.562499998634403475, 0.000000000000000000 ) ) ;
#47327=ORIENTED_EDGE ( 'NONE', *, *, #815, .F. ) ;
#47328=DIRECTION ( 'NONE',  ( -0.000000000000000000, 1.000000000000000000, -0.000000000000000000 ) ) ;
#47329=CARTESIAN_POINT ( 'NONE',  ( -6.972266317189433020E-16, -64.24999999999998579, -5.000000000000000000 ) ) ;
#47330=CARTESIAN_POINT ( 'NONE',  ( -3.152548672688508926E-16, -6.812499998634404363, -5.148502694627439702 ) ) ;
#47331=DIRECTION ( 'NONE',  ( -0.000000000000000000, 1.000000000000000000, -0.000000000000000000 ) ) ;
#47333=DIRECTION ( 'NONE',  ( -0.000000000000000000, 1.000000000000000000, -0.000000000000000000 ) ) ;
#47335=CARTESIAN_POINT ( 'NONE',  ( -4.458734124999999437, 25.43750000136559208, 0.000000000000000000 ) ) ;
#47337=CARTESIAN_POINT ( 'NONE',  ( -2.229367062500000163, -89.47916666530106511, -3.861377020970580443 ) ) ;
#47338=CARTESIAN_POINT ( 'NONE',  ( -2.499999999999996447, -77.83333333333334281, 4.330127018922195425 ) ) ;
#47339=CARTESIAN_POINT ( 'NONE',  ( -4.458734124999998549, -9.229166665301068662, 2.574251347313722516 ) ) ;
#47341=DIRECTION ( 'NONE',  ( -0.000000000000000000, 1.000000000000000000, -0.000000000000000000 ) ) ;
#47342=LINE ( 'NONE', #43130, #10925 ) ;
#47343=CARTESIAN_POINT ( 'NONE',  ( -1.339745962155610925, 15.20534180126147916, 5.000000000000000000 ) ) ;
#47344=CARTESIAN_POINT ( 'NONE',  ( 1.060575238724906964E-15, -38.62499999726881583, 5.773502691896257311 ) ) ;
#47345=CARTESIAN_POINT ( 'NONE',  ( 2.229367062499998831, 19.35416666803225993, -3.861377020970580887 ) ) ;
#47346=CARTESIAN_POINT ( 'NONE',  ( 1.975475456537005874E-15, -97.62499999726880162, 5.000000000000000000 ) ) ;
#47348=CARTESIAN_POINT ( 'NONE',  ( -4.458734124999999437, -54.31249999863440081, 0.000000000000000000 ) ) ;
#47350=CYLINDRICAL_SURFACE ( 'NONE', #21679, 5.000000000000000000 ) ;
#47351=CARTESIAN_POINT ( 'NONE',  ( 2.499999999999998668, 12.66666666666666607, -4.330127018922193649 ) ) ;
#47354=CARTESIAN_POINT ( 'NONE',  ( -4.458734124999999437, -50.39583333196773651, -2.574251347313719407 ) ) ;
#47355=CARTESIAN_POINT ( 'NONE',  ( 5.000000000000000000, -85.37499999726880162, -6.123233995736766282E-16 ) ) ;
#47358=EDGE_CURVE ( 'NONE', #62035, #45003, #31432, .T. ) ;
#47360=CARTESIAN_POINT ( 'NONE',  ( 2.229367062499998831, -86.89583333196773651, -3.861377020970580887 ) ) ;
#47363=CARTESIAN_POINT ( 'NONE',  ( -4.999999999999999112, -34.91666666666666430, 2.886751345948131764 ) ) ;
#47367=EDGE_LOOP ( 'NONE', ( #20842, #1875, #47776, #5648 ) ) ;
#47368=CARTESIAN_POINT ( 'NONE',  ( -4.458734124999999437, -98.39583333196773651, -2.574251347313719407 ) ) ;
#47369=CARTESIAN_POINT ( 'NONE',  ( -2.229367062499996610, 10.60416666803225993, 3.861377020970582219 ) ) ;
#47370=CARTESIAN_POINT ( 'NONE',  ( 2.500000000000002220, 12.45833333606451809, 4.330127018922192761 ) ) ;
#47371=CARTESIAN_POINT ( 'NONE',  ( -2.499999999999996447, -43.70833333060214443, 4.330127018922195425 ) ) ;
#47375=CARTESIAN_POINT ( 'NONE',  ( -5.000000000000000000, -79.00000000000000000, 0.000000000000000000 ) ) ;
#47377=CARTESIAN_POINT ( 'NONE',  ( -6.972266317189433020E-16, -13.12499999726881050, -5.000000000000000000 ) ) ;
#47382=CARTESIAN_POINT ( 'NONE',  ( 9.457646018065525792E-16, -21.31249999863440081, 5.148502694627439702 ) ) ;
#47390=ORIENTED_EDGE ( 'NONE', *, *, #14895, .F. ) ;
#47393=CARTESIAN_POINT ( 'NONE',  ( 9.457646018065525792E-16, -68.31249999863442213, 5.148502694627439702 ) ) ;
#47400=DIRECTION ( 'NONE',  ( 0.000000000000000000, 0.000000000000000000, 1.000000000000000000 ) ) ;
#47401=CARTESIAN_POINT ( 'NONE',  ( -2.229367062500000163, 7.520833334698929562, -3.861377020970580443 ) ) ;
#47404=CARTESIAN_POINT ( 'NONE',  ( -4.999999999999998224, 6.208333336064520758, 2.886751345948131764 ) ) ;
#47406=( BOUNDED_CURVE ( )  B_SPLINE_CURVE ( 2, ( #38093, #57719, #58338, #54133, #10395, #58651, #24878, #24555, #129 ),
 .UNSPECIFIED., .F., .F. ) 
 B_SPLINE_CURVE_WITH_KNOTS ( ( 3, 2, 2, 2, 3 ),
 ( 0.5696428571428571175, 0.5702380952380952106, 0.5714285714285713969, 0.5726190476190475831, 0.5732142857142856762 ),
 .UNSPECIFIED. ) 
 CURVE ( )  GEOMETRIC_REPRESENTATION_ITEM ( )  RATIONAL_B_SPLINE_CURVE ( ( 0.9330127018922194093, 0.9330127018922194093, 1.000000000000000000, 0.8660254037844387076, 1.000000000000000000, 0.8660254037844387076, 1.000000000000000000, 0.9330127018922194093, 0.9330127018922194093 ) ) 
 REPRESENTATION_ITEM ( '' )  );
#47408=CARTESIAN_POINT ( 'NONE',  ( -4.458734124999999437, -72.31249999863439371, 0.000000000000000000 ) ) ;
#47410=CARTESIAN_POINT ( 'NONE',  ( 4.458734125000001214, 5.104166668032261711, 2.574251347313718519 ) ) ;
#47412=CARTESIAN_POINT ( 'NONE',  ( -4.458734124999999437, -59.56249999863440081, 0.000000000000000000 ) ) ;
#47413=CARTESIAN_POINT ( 'NONE',  ( 5.000000000000000000, -22.29166666393548368, -2.886751345948129988 ) ) ;
#47414=CARTESIAN_POINT ( 'NONE',  ( -5.000000000000000000, -32.95833333060215153, -2.886751345948128211 ) ) ;
#47415=CARTESIAN_POINT ( 'NONE',  ( -5.000000000000000000, -44.87499999726880873, 0.000000000000000000 ) ) ;
#47417=CARTESIAN_POINT ( 'NONE',  ( 1.339745962155612702, -65.29465819873851729, -5.000000000000000000 ) ) ;
#47418=CARTESIAN_POINT ( 'NONE',  ( -4.458734124999998549, -41.22916666530107221, 2.574251347313722516 ) ) ;
#47419=CARTESIAN_POINT ( 'NONE',  ( 2.229367062499998831, -22.89583333196773651, -3.861377020970580887 ) ) ;
#47420=ORIENTED_EDGE ( 'NONE', *, *, #33908, .F. ) ;
#47422=CARTESIAN_POINT ( 'NONE',  ( -4.458734124999999437, -108.3958333319677365, -2.574251347313719407 ) ) ;
#47425=CARTESIAN_POINT ( 'NONE',  ( -2.229367062500000163, -109.7291666653010651, -3.861377020970580443 ) ) ;
#47426=VECTOR ( 'NONE', #33646, 1000.000000000000000 ) ;
#47427=CARTESIAN_POINT ( 'NONE',  ( -2.229367062500000163, -31.47916666530107577, -3.861377020970580443 ) ) ;
#47428=CARTESIAN_POINT ( 'NONE',  ( -2.500000000000000444, -69.04166666393547303, -4.330127018922193649 ) ) ;
#47431=CARTESIAN_POINT ( 'NONE',  ( 4.458734124999998549, -28.72916666530107221, -2.574251347313721627 ) ) ;
#47432=CARTESIAN_POINT ( 'NONE',  ( 2.229367062500001939, -69.22916666530107932, 3.861377020970579999 ) ) ;
#47437=CARTESIAN_POINT ( 'NONE',  ( 1.060575238724906964E-15, -17.75000000000000355, 5.773502691896257311 ) ) ;
#47442=EDGE_CURVE ( 'NONE', #11069, #14391, #52925, .T. ) ;
#47443=CARTESIAN_POINT ( 'NONE',  ( 5.000000000000000888, 26.54166666939785202, 2.886751345948126879 ) ) ;
#47444=FACE_OUTER_BOUND ( 'NONE', #37641, .T. ) ;
#47451=CARTESIAN_POINT ( 'NONE',  ( -1.339745962155610925, -29.66965819600733312, 5.000000000000000000 ) ) ;
#47452=VERTEX_POINT ( 'NONE', #60731 ) ;
#47457=ORIENTED_EDGE ( 'NONE', *, *, #42050, .T. ) ;
#47459=ORIENTED_EDGE ( 'NONE', *, *, #29535, .T. ) ;
#47460=CARTESIAN_POINT ( 'NONE',  ( 1.339745962155615144, -53.70534180126147561, 4.999999999999999112 ) ) ;
#47462=CARTESIAN_POINT ( 'NONE',  ( -2.499999999999996447, -38.70833333060213732, 4.330127018922195425 ) ) ;
#47466=CARTESIAN_POINT ( 'NONE',  ( 4.458734124999999437, -83.81249999863439371, -5.460374474430324690E-16 ) ) ;
#47467=CARTESIAN_POINT ( 'NONE',  ( -3.152548672688508926E-16, 23.43750000136559564, -5.148502694627439702 ) ) ;
#47474=LINE ( 'NONE', #17589, #3818 ) ;
#47477=CARTESIAN_POINT ( 'NONE',  ( 9.457646018065525792E-16, -52.06249999863440792, 5.148502694627439702 ) ) ;
#47478=CARTESIAN_POINT ( 'NONE',  ( 4.458734124999998549, 23.27083333469892423, -2.574251347313721627 ) ) ;
#47480=( BOUNDED_CURVE ( )  B_SPLINE_CURVE ( 2, ( #27393, #7790, #37680, #46701, #42818, #7163, #26773, #32861, #3600 ),
 .UNSPECIFIED., .F., .F. ) 
 B_SPLINE_CURVE_WITH_KNOTS ( ( 3, 2, 2, 2, 3 ),
 ( 0.5803571428571429047, 0.5809523809523809978, 0.5821428571428571841, 0.5833333333333333703, 0.5839285714285714635 ),
 .UNSPECIFIED. ) 
 CURVE ( )  GEOMETRIC_REPRESENTATION_ITEM ( )  RATIONAL_B_SPLINE_CURVE ( ( 0.9330127018922194093, 0.9330127018922194093, 1.000000000000000000, 0.8660254037844387076, 1.000000000000000000, 0.8660254037844387076, 1.000000000000000000, 0.9330127018922194093, 0.9330127018922194093 ) ) 
 REPRESENTATION_ITEM ( '' )  );
#47483=CARTESIAN_POINT ( 'NONE',  ( 4.458734125000001214, -42.14583333196773651, 2.574251347313718519 ) ) ;
#47484=CARTESIAN_POINT ( 'NONE',  ( -3.535250795749689387E-16, -6.124999997268812280, -5.773502691896257311 ) ) ;
#47486=CARTESIAN_POINT ( 'NONE',  ( 0.000000000000000000, -120.0000000000000000, 0.000000000000000000 ) ) ;
#47488=CARTESIAN_POINT ( 'NONE',  ( 4.458734125000000326, -103.8958333319677365, 2.574251347313718519 ) ) ;
#47489=CARTESIAN_POINT ( 'NONE',  ( -2.229367062500000163, -4.729166665301071326, -3.861377020970580443 ) ) ;
#47492=CARTESIAN_POINT ( 'NONE',  ( 4.458734125000001214, -90.89583333196772230, 2.574251347313718519 ) ) ;
#47494=CARTESIAN_POINT ( 'NONE',  ( 4.458734124999998549, -93.97916666530106511, -2.574251347313721627 ) ) ;
#47496=DIRECTION ( 'NONE',  ( -0.000000000000000000, 1.000000000000000000, -0.000000000000000000 ) ) ;
#47499=ADVANCED_FACE ( 'NONE', ( #932 ), #54941, .T. ) ;
#47500=CARTESIAN_POINT ( 'NONE',  ( -3.152548672688508926E-16, -11.56249999863440792, -5.148502694627439702 ) ) ;
#47501=CARTESIAN_POINT ( 'NONE',  ( 4.458734125000001214, 12.85416666803226171, 2.574251347313718519 ) ) ;
#47502=EDGE_CURVE ( 'NONE', #35740, #43806, #839, .T. ) ;
#47503=CARTESIAN_POINT ( 'NONE',  ( -2.229367062499996610, -51.39583333196773651, 3.861377020970582219 ) ) ;
#47504=FACE_OUTER_BOUND ( 'NONE', #16334, .T. ) ;
#47505=CARTESIAN_POINT ( 'NONE',  ( -5.000000000000000000, -37.00000000000000711, 0.000000000000000000 ) ) ;
#47511=CARTESIAN_POINT ( 'NONE',  ( 5.000000000000000000, -68.41666666666667140, -2.886751345948130876 ) ) ;
#47513=CARTESIAN_POINT ( 'NONE',  ( -4.458734124999999437, -81.31249999863440792, 0.000000000000000000 ) ) ;
#47514=CARTESIAN_POINT ( 'NONE',  ( 2.229367062500001939, 24.77083333469892779, 3.861377020970579999 ) ) ;
#47515=EDGE_CURVE ( 'NONE', #62207, #45023, #61678, .T. ) ;
#47517=DIRECTION ( 'NONE',  ( 0.000000000000000000, 0.000000000000000000, 1.000000000000000000 ) ) ;
#47518=CARTESIAN_POINT ( 'NONE',  ( 0.000000000000000000, -120.0000000000000000, 0.000000000000000000 ) ) ;
#47520=CARTESIAN_POINT ( 'NONE',  ( 5.000000000000000888, -68.58333333333334281, 2.886751345948126879 ) ) ;
#47523=DIRECTION ( 'NONE',  ( -0.000000000000000000, 1.000000000000000000, -0.000000000000000000 ) ) ;
#47524=CYLINDRICAL_SURFACE ( 'NONE', #28862, 5.000000000000000000 ) ;
#47528=CARTESIAN_POINT ( 'NONE',  ( 1.339745962155615144, -62.70534180126146850, 4.999999999999999112 ) ) ;
#47530=EDGE_CURVE ( 'NONE', #50712, #28828, #62307, .T. ) ;
#47532=EDGE_LOOP ( 'NONE', ( #46122, #47545, #36477, #16085 ) ) ;
#47538=CARTESIAN_POINT ( 'NONE',  ( -4.458734124999999437, -49.56249999863440792, 0.000000000000000000 ) ) ;
#47540=CARTESIAN_POINT ( 'NONE',  ( -5.000000000000000000, -54.87499999726880162, 0.000000000000000000 ) ) ;
#47545=ORIENTED_EDGE ( 'NONE', *, *, #60184, .T. ) ;
#47548=CARTESIAN_POINT ( 'NONE',  ( -2.229367062500000163, -97.72916666530105090, -3.861377020970580443 ) ) ;
#47554=CARTESIAN_POINT ( 'NONE',  ( 1.339745962155615144, -83.70534180126149693, 4.999999999999999112 ) ) ;
#47555=ADVANCED_FACE ( 'NONE', ( #37533 ), #27561, .T. ) ;
#47556=CARTESIAN_POINT ( 'NONE',  ( 4.458734124999998549, -5.729166665301072214, -2.574251347313721627 ) ) ;
#47557=CARTESIAN_POINT ( 'NONE',  ( -4.458734124999999437, -93.64583333196772230, -2.574251347313719407 ) ) ;
#47560=CARTESIAN_POINT ( 'NONE',  ( 4.458734125000001214, -30.14583333196773296, 2.574251347313718519 ) ) ;
#47561=DIRECTION ( 'NONE',  ( -0.000000000000000000, 1.000000000000000000, -0.000000000000000000 ) ) ;
#47564=CARTESIAN_POINT ( 'NONE',  ( 5.000000000000000000, -17.41666666666666430, -2.886751345948130876 ) ) ;
#47566=CARTESIAN_POINT ( 'NONE',  ( -2.229367062499996610, 12.60416666803226171, 3.861377020970582219 ) ) ;
#47567=ORIENTED_EDGE ( 'NONE', *, *, #6078, .T. ) ;
#47569=DIRECTION ( 'NONE',  ( -0.000000000000000000, 1.000000000000000000, -0.000000000000000000 ) ) ;
#47570=CARTESIAN_POINT ( 'NONE',  ( 2.500000000000002220, -89.66666666666665719, 4.330127018922192761 ) ) ;
#47571=CARTESIAN_POINT ( 'NONE',  ( -2.229367062500000163, -22.47916666530107221, -3.861377020970580443 ) ) ;
#47573=CARTESIAN_POINT ( 'NONE',  ( -4.458734124999999437, -78.64583333196773651, -2.574251347313719407 ) ) ;
#47577=CARTESIAN_POINT ( 'NONE',  ( -2.229367062499996610, 0.8541666680322613781, 3.861377020970582219 ) ) ;
#47578=CARTESIAN_POINT ( 'NONE',  ( -3.152548672688508926E-16, 28.18750000136559564, -5.148502694627439702 ) ) ;
#47579=EDGE_CURVE ( 'NONE', #53022, #13464, #7335, .T. ) ;
#47580=CARTESIAN_POINT ( 'NONE',  ( -2.229367062500000163, -37.72916666530107221, -3.861377020970580443 ) ) ;
#47583=CARTESIAN_POINT ( 'NONE',  ( -2.229367062499996610, -70.14583333196773651, 3.861377020970582219 ) ) ;
#47585=CARTESIAN_POINT ( 'NONE',  ( 5.000000000000000888, -6.583333333333329485, 2.886751345948126879 ) ) ;
#47588=CARTESIAN_POINT ( 'NONE',  ( 4.458734124999999437, -64.81249999863440792, -5.460374474430324690E-16 ) ) ;
#47589=CARTESIAN_POINT ( 'NONE',  ( -2.500000000000000444, -100.0416666639354588, -4.330127018922193649 ) ) ;
#47593=CARTESIAN_POINT ( 'NONE',  ( -2.229367062500000163, -108.7291666653010651, -3.861377020970580443 ) ) ;
#47595=CARTESIAN_POINT ( 'NONE',  ( 5.000000000000000888, -55.58333333333333570, 2.886751345948126879 ) ) ;
#47597=EDGE_LOOP ( 'NONE', ( #49880, #26893, #57521, #22679 ) ) ;
#47603=CARTESIAN_POINT ( 'NONE',  ( -5.000000000000000000, -5.999999999999998224, 0.000000000000000000 ) ) ;
#47609=ORIENTED_EDGE ( 'NONE', *, *, #53448, .F. ) ;
#47614=CARTESIAN_POINT ( 'NONE',  ( 4.458734124999999437, -34.06249999863440792, -5.460374474430324690E-16 ) ) ;
#47621=CARTESIAN_POINT ( 'NONE',  ( 5.000000000000000000, -54.41666666666667140, -2.886751345948130876 ) ) ;
#47622=CARTESIAN_POINT ( 'NONE',  ( 4.458734124999999437, -84.06249999863439371, -5.460374474430324690E-16 ) ) ;
#47626=CARTESIAN_POINT ( 'NONE',  ( -5.000000000000000000, -105.0000000000000142, 0.000000000000000000 ) ) ;
#47633=CARTESIAN_POINT ( 'NONE',  ( -2.229367062500000163, -14.72916666530107221, -3.861377020970580443 ) ) ;
#47635=CARTESIAN_POINT ( 'NONE',  ( -5.000000000000000000, -35.08333333333332860, -2.886751345948128211 ) ) ;
#47637=CARTESIAN_POINT ( 'NONE',  ( -6.972266317189433020E-16, -96.12499999726880162, -5.000000000000000000 ) ) ;
#47639=CARTESIAN_POINT ( 'NONE',  ( 2.229367062499998831, 25.10416666803225993, -3.861377020970580887 ) ) ;
#47640=VERTEX_POINT ( 'NONE', #17285 ) ;
#47641=CARTESIAN_POINT ( 'NONE',  ( 4.458734124999999437, -90.81249999863440792, -5.460374474430324690E-16 ) ) ;
#47642=CARTESIAN_POINT ( 'NONE',  ( -2.499999999999996447, -30.83333333333333215, 4.330127018922195425 ) ) ;
#47643=CARTESIAN_POINT ( 'NONE',  ( 1.339745962155615144, 7.419658201469705894, 4.999999999999999112 ) ) ;
#47644=CARTESIAN_POINT ( 'NONE',  ( -4.458734124999998549, -8.229166665301073991, 2.574251347313722516 ) ) ;
#47645=EDGE_CURVE ( 'NONE', #43789, #4593, #47194, .T. ) ;
#47648=CYLINDRICAL_SURFACE ( 'NONE', #54031, 5.000000000000000000 ) ;
#47649=CARTESIAN_POINT ( 'NONE',  ( 5.000000000000000000, -36.37499999726881583, -6.123233995736766282E-16 ) ) ;
#47650=CARTESIAN_POINT ( 'NONE',  ( 4.458734125000000326, 20.10416666803225638, 2.574251347313718519 ) ) ;
#47651=CARTESIAN_POINT ( 'NONE',  ( -5.000000000000000000, -4.083333333333334814, -2.886751345948128211 ) ) ;
#47654=CARTESIAN_POINT ( 'NONE',  ( -4.458734124999998549, -54.22916666530107221, 2.574251347313722516 ) ) ;
#47657=CARTESIAN_POINT ( 'NONE',  ( 5.000000000000000000, 7.583333333333333925, -2.886751345948129988 ) ) ;
#47661=EDGE_CURVE ( 'NONE', #29252, #60646, #22520, .T. ) ;
#47662=CARTESIAN_POINT ( 'NONE',  ( 4.458734125000001214, -45.89583333196774362, 2.574251347313718519 ) ) ;
#47663=CARTESIAN_POINT ( 'NONE',  ( -2.500000000000000444, -86.04166666393547303, -4.330127018922193649 ) ) ;
#47666=CARTESIAN_POINT ( 'NONE',  ( -2.499999999999996447, -104.7083333306021444, 4.330127018922195425 ) ) ;
#47667=CARTESIAN_POINT ( 'NONE',  ( 9.457646018065525792E-16, -92.31249999863440792, 5.148502694627439702 ) ) ;
#47669=CARTESIAN_POINT ( 'NONE',  ( 5.000000000000000000, -37.41666666666666430, -2.886751345948129988 ) ) ;
#47670=CARTESIAN_POINT ( 'NONE',  ( 1.339745962155641346, 8.830341803992666883, -4.999999999999983125 ) ) ;
#47671=EDGE_LOOP ( 'NONE', ( #59096, #12942, #39158, #32887 ) ) ;
#47673=ORIENTED_EDGE ( 'NONE', *, *, #30204, .F. ) ;
#47674=CARTESIAN_POINT ( 'NONE',  ( 9.457646018065525792E-16, -96.06249999863440792, 5.148502694627439702 ) ) ;
#47675=CARTESIAN_POINT ( 'NONE',  ( -2.229367062499996610, 6.604166668032259935, 3.861377020970582219 ) ) ;
#47676=CARTESIAN_POINT ( 'NONE',  ( 2.499999999999998668, 9.791666669397850242, -4.330127018922193649 ) ) ;
#47680=( BOUNDED_CURVE ( )  B_SPLINE_CURVE ( 2, ( #45362, #29920, #30557, #54048, #1327, #20926, #25101, #44393, #6134 ),
 .UNSPECIFIED., .F., .F. ) 
 B_SPLINE_CURVE_WITH_KNOTS ( ( 3, 2, 2, 2, 3 ),
 ( 0.05535714285714286170, 0.05595238095238095483, 0.05714285714285714107, 0.05833333333333333426, 0.05892857142857142738 ),
 .UNSPECIFIED. ) 
 CURVE ( )  GEOMETRIC_REPRESENTATION_ITEM ( )  RATIONAL_B_SPLINE_CURVE ( ( 0.9330127018922194093, 0.9330127018922197424, 1.000000000000000000, 0.8660254037844387076, 1.000000000000000000, 0.8660254037844387076, 1.000000000000000000, 0.9330127018922194093, 0.9330127018922194093 ) ) 
 REPRESENTATION_ITEM ( '' )  );
#47681=CARTESIAN_POINT ( 'NONE',  ( -4.769696007084728073, -120.0000000000000000, 1.499999999999999556 ) ) ;
#47685=CARTESIAN_POINT ( 'NONE',  ( 1.975475456537005874E-15, -5.624999997268812280, 5.000000000000000000 ) ) ;
#47689=CARTESIAN_POINT ( 'NONE',  ( -4.458734124999999437, -19.64583333196774362, -2.574251347313719407 ) ) ;
#47690=CARTESIAN_POINT ( 'NONE',  ( -1.339745962155613812, -58.20534180126147561, -5.000000000000000000 ) ) ;
#47697=ORIENTED_EDGE ( 'NONE', *, *, #18939, .F. ) ;
#47699=EDGE_LOOP ( 'NONE', ( #11728, #13682, #6974, #23898 ) ) ;
#47700=CARTESIAN_POINT ( 'NONE',  ( 4.458734125000001214, -69.14583333196773651, 2.574251347313718519 ) ) ;
#47706=CARTESIAN_POINT ( 'NONE',  ( -4.458734124999999437, 3.354166668032260823, -2.574251347313719407 ) ) ;
#47708=VECTOR ( 'NONE', #52202, 1000.000000000000000 ) ;
#47709=CARTESIAN_POINT ( 'NONE',  ( 0.000000000000000000, -120.0000000000000000, 0.000000000000000000 ) ) ;
#47710=CARTESIAN_POINT ( 'NONE',  ( 4.458734124999999437, 2.187500001365593416, -5.460374474430324690E-16 ) ) ;
#47716=CARTESIAN_POINT ( 'NONE',  ( 4.458734124999998549, -77.72916666530106511, -2.574251347313721627 ) ) ;
#47717=CARTESIAN_POINT ( 'NONE',  ( 5.000000000000000888, -10.45833333060214443, 2.886751345948126879 ) ) ;
#47718=CARTESIAN_POINT ( 'NONE',  ( 4.458734124999999437, 5.187500001365596525, -5.460374474430324690E-16 ) ) ;
#47719=CARTESIAN_POINT ( 'NONE',  ( -4.458734124999999437, -57.56249999863440081, 0.000000000000000000 ) ) ;
#47720=CARTESIAN_POINT ( 'NONE',  ( -2.500000000000000444, -22.04166666393548013, -4.330127018922193649 ) ) ;
#47722=CARTESIAN_POINT ( 'NONE',  ( 2.499999999999998668, -42.20833333060214443, -4.330127018922193649 ) ) ;
#47724=( BOUNDED_CURVE ( )  B_SPLINE_CURVE ( 2, ( #42799, #4823, #38590, #33162, #29572, #24442, #49203, #43421, #28631 ),
 .UNSPECIFIED., .F., .F. ) 
 B_SPLINE_CURVE_WITH_KNOTS ( ( 3, 2, 2, 2, 3 ),
 ( 0.9875000000000000444, 0.9880952380952381375, 0.9892857142857143238, 0.9904761904761905100, 0.9910714285714286031 ),
 .UNSPECIFIED. ) 
 CURVE ( )  GEOMETRIC_REPRESENTATION_ITEM ( )  RATIONAL_B_SPLINE_CURVE ( ( 0.9330127018922194093, 0.9330127018922194093, 1.000000000000000000, 0.8660254037844387076, 1.000000000000000000, 0.8660254037844387076, 1.000000000000000000, 0.9330127018922194093, 0.9330127018922194093 ) ) 
 REPRESENTATION_ITEM ( '' )  );
#47727=CARTESIAN_POINT ( 'NONE',  ( 4.458734124999999437, -41.81249999863440081, -5.460374474430324690E-16 ) ) ;
#47728=CARTESIAN_POINT ( 'NONE',  ( 9.457646018065525792E-16, -28.31249999863440081, 5.148502694627439702 ) ) ;
#47729=( BOUNDED_CURVE ( )  B_SPLINE_CURVE ( 2, ( #34435, #6149, #25116, #38948, #5188, #34125, #54064, #58586, #53747 ),
 .UNSPECIFIED., .F., .F. ) 
 B_SPLINE_CURVE_WITH_KNOTS ( ( 3, 2, 2, 2, 3 ),
 ( 0.02321428571428571508, 0.02380952380952380820, 0.02500000000000000139, 0.02619047619047619110, 0.02678571428571428770 ),
 .UNSPECIFIED. ) 
 CURVE ( )  GEOMETRIC_REPRESENTATION_ITEM ( )  RATIONAL_B_SPLINE_CURVE ( ( 0.9330127018922194093, 0.9330127018922195203, 1.000000000000000000, 0.8660254037844387076, 1.000000000000000000, 0.8660254037844387076, 1.000000000000000000, 0.9330127018922191873, 0.9330127018922194093 ) ) 
 REPRESENTATION_ITEM ( '' )  );
#47730=CARTESIAN_POINT ( 'NONE',  ( 6.123233995736766282E-16, -120.0000000000000000, -5.000000000000000000 ) ) ;
#47731=CARTESIAN_POINT ( 'NONE',  ( 2.500000000000002220, 28.33333333333333215, 4.330127018922192761 ) ) ;
#47733=ORIENTED_EDGE ( 'NONE', *, *, #40512, .F. ) ;
#47734=CARTESIAN_POINT ( 'NONE',  ( -4.458734124999998549, -110.4791666653010793, 2.574251347313722516 ) ) ;
#47735=CARTESIAN_POINT ( 'NONE',  ( 4.458734124999999437, -32.81249999863440792, -5.460374474430324690E-16 ) ) ;
#47736=CARTESIAN_POINT ( 'NONE',  ( 2.500000000000002220, -70.54166666393547303, 4.330127018922192761 ) ) ;
#47739=ADVANCED_FACE ( 'NONE', ( #14342 ), #39407, .T. ) ;
#47740=CARTESIAN_POINT ( 'NONE',  ( -4.458734124999999437, -27.31249999863440081, 0.000000000000000000 ) ) ;
#47741=CARTESIAN_POINT ( 'NONE',  ( 4.458734124999999437, -77.06249999863440792, -5.460374474430324690E-16 ) ) ;
#47746=CARTESIAN_POINT ( 'NONE',  ( -2.499999999999996447, -17.83333333333333215, 4.330127018922195425 ) ) ;
#47749=CARTESIAN_POINT ( 'NONE',  ( -6.972266317189433020E-16, -28.25000000000000000, -5.000000000000000000 ) ) ;
#47751=CARTESIAN_POINT ( 'NONE',  ( -3.535250795749689387E-16, 26.87500000273118772, -5.773502691896257311 ) ) ;
#47759=( BOUNDED_CURVE ( )  B_SPLINE_CURVE ( 2, ( #8220, #13035, #56800, #4024, #37804, #28454, #27824, #23327, #7903 ),
 .UNSPECIFIED., .F., .F. ) 
 B_SPLINE_CURVE_WITH_KNOTS ( ( 3, 2, 2, 2, 3 ),
 ( 0.5767857142857142350, 0.5773809523809523281, 0.5785714285714286254, 0.5797619047619048116, 0.5803571428571429047 ),
 .UNSPECIFIED. ) 
 CURVE ( )  GEOMETRIC_REPRESENTATION_ITEM ( )  RATIONAL_B_SPLINE_CURVE ( ( 0.9330127018922194093, 0.9330127018922194093, 1.000000000000000000, 0.8660254037844387076, 1.000000000000000000, 0.8660254037844387076, 1.000000000000000000, 0.9330127018922194093, 0.9330127018922194093 ) ) 
 REPRESENTATION_ITEM ( '' )  );
#47760=CARTESIAN_POINT ( 'NONE',  ( 1.975475456537005874E-15, -87.62499999726880162, 5.000000000000000000 ) ) ;
#47766=ORIENTED_EDGE ( 'NONE', *, *, #54232, .T. ) ;
#47768=VERTEX_POINT ( 'NONE', #39095 ) ;
#47769=CARTESIAN_POINT ( 'NONE',  ( -4.999999999999998224, -95.91666666666665719, 2.886751345948131764 ) ) ;
#47770=CARTESIAN_POINT ( 'NONE',  ( 5.000000000000000000, -53.49999999999999289, -6.123233995736766282E-16 ) ) ;
#47776=ORIENTED_EDGE ( 'NONE', *, *, #25634, .T. ) ;
#47777=CARTESIAN_POINT ( 'NONE',  ( 2.229367062499998831, -82.64583333196773651, -3.861377020970580887 ) ) ;
#47778=CARTESIAN_POINT ( 'NONE',  ( -2.229367062500000163, 17.52083333469892779, -3.861377020970580443 ) ) ;
#47780=VERTEX_POINT ( 'NONE', #53584 ) ;
#47786=CARTESIAN_POINT ( 'NONE',  ( 4.458734125000000326, -57.89583333196773651, 2.574251347313718519 ) ) ;
#47788=CARTESIAN_POINT ( 'NONE',  ( -3.152548672688508926E-16, 22.43750000136559208, -5.148502694627439702 ) ) ;
#47789=CARTESIAN_POINT ( 'NONE',  ( -6.972266317189433020E-16, -97.24999999999998579, -5.000000000000000000 ) ) ;
#47792=CARTESIAN_POINT ( 'NONE',  ( -3.152548672688508926E-16, -42.81249999863440081, -5.148502694627439702 ) ) ;
#47793=CARTESIAN_POINT ( 'NONE',  ( 2.499999999999998668, -2.208333330602146205, -4.330127018922193649 ) ) ;
#47794=CARTESIAN_POINT ( 'NONE',  ( 2.500000000000002220, -31.66666666666666075, 4.330127018922192761 ) ) ;
#47797=CARTESIAN_POINT ( 'NONE',  ( 4.458734124999998549, -104.7291666653010509, -2.574251347313721627 ) ) ;
#47798=CARTESIAN_POINT ( 'NONE',  ( 9.457646018065525792E-16, -10.31249999863440969, 5.148502694627439702 ) ) ;
#47799=VERTEX_POINT ( 'NONE', #28189 ) ;
#47800=CARTESIAN_POINT ( 'NONE',  ( 2.499999999999998668, -52.33333333333332860, -4.330127018922193649 ) ) ;
#47801=CARTESIAN_POINT ( 'NONE',  ( 2.229367062499998831, -95.64583333196773651, -3.861377020970580887 ) ) ;
#47803=CARTESIAN_POINT ( 'NONE',  ( -4.458734124999999437, -90.56249999863440792, 0.000000000000000000 ) ) ;
#47804=CARTESIAN_POINT ( 'NONE',  ( -3.535250795749689387E-16, -53.12499999726881583, -5.773502691896257311 ) ) ;
#47805=CARTESIAN_POINT ( 'NONE',  ( -6.972266317189433020E-16, -42.12499999726880873, -5.000000000000000000 ) ) ;
#47807=CARTESIAN_POINT ( 'NONE',  ( 2.229367062500001939, -12.97916666530107221, 3.861377020970579999 ) ) ;
#47808=CARTESIAN_POINT ( 'NONE',  ( -2.229367062500000163, 9.270833334698927786, -3.861377020970580443 ) ) ;
#47809=CARTESIAN_POINT ( 'NONE',  ( 2.229367062499998831, -55.89583333196773651, -3.861377020970580887 ) ) ;
#47811=CARTESIAN_POINT ( 'NONE',  ( -5.000000000000000000, -106.0833333333333286, -2.886751345948128211 ) ) ;
#47813=CARTESIAN_POINT ( 'NONE',  ( 1.339745962155615144, -8.580341798530293218, 4.999999999999999112 ) ) ;
#47817=DIRECTION ( 'NONE',  ( 1.000000000000000000, 0.000000000000000000, -1.061635649774262664E-14 ) ) ;
#47818=CARTESIAN_POINT ( 'NONE',  ( 0.000000000000000000, -120.0000000000000000, 0.000000000000000000 ) ) ;
#47819=CARTESIAN_POINT ( 'NONE',  ( -4.458734124999998549, -84.22916666530107932, 2.574251347313722516 ) ) ;
#47820=CARTESIAN_POINT ( 'NONE',  ( -4.458734124999999437, 23.43750000136559564, 0.000000000000000000 ) ) ;
#47822=LINE ( 'NONE', #3781, #23651 ) ;
#47825=CARTESIAN_POINT ( 'NONE',  ( -2.500000000000000444, -70.16666666666667140, -4.330127018922193649 ) ) ;
#47827=ORIENTED_EDGE ( 'NONE', *, *, #52922, .T. ) ;
#47830=CARTESIAN_POINT ( 'NONE',  ( 1.339745962155615144, -40.70534180126147561, 4.999999999999999112 ) ) ;
#47833=EDGE_CURVE ( 'NONE', #62764, #19054, #17984, .T. ) ;
#47834=CARTESIAN_POINT ( 'NONE',  ( -5.000000000000000000, 5.000000000000000888, 0.000000000000000000 ) ) ;
#47844=CARTESIAN_POINT ( 'NONE',  ( 2.229367062500001939, -56.22916666530107221, 3.861377020970579999 ) ) ;
#47851=ORIENTED_EDGE ( 'NONE', *, *, #50698, .T. ) ;
#47855=CARTESIAN_POINT ( 'NONE',  ( -2.229367062499996610, -100.3958333319677365, 3.861377020970582219 ) ) ;
#47856=CARTESIAN_POINT ( 'NONE',  ( -6.972266317189433020E-16, -27.12499999726881228, -5.000000000000000000 ) ) ;
#47861=CARTESIAN_POINT ( 'NONE',  ( 4.458734125000001214, -9.895833331967736513, 2.574251347313718519 ) ) ;
#47862=CARTESIAN_POINT ( 'NONE',  ( 4.458734125000000326, -103.1458333319677507, 2.574251347313718519 ) ) ;
#47863=( BOUNDED_CURVE ( )  B_SPLINE_CURVE ( 2, ( #30910, #21264, #36060, #60513, #55689, #32170, #56003, #36693, #26404 ),
 .UNSPECIFIED., .F., .F. ) 
 B_SPLINE_CURVE_WITH_KNOTS ( ( 3, 2, 2, 2, 3 ),
 ( 0.7303571428571428159, 0.7309523809523809090, 0.7321428571428570953, 0.7333333333333332815, 0.7339285714285714857 ),
 .UNSPECIFIED. ) 
 CURVE ( )  GEOMETRIC_REPRESENTATION_ITEM ( )  RATIONAL_B_SPLINE_CURVE ( ( 0.9330127018922194093, 0.9330127018922194093, 1.000000000000000000, 0.8660254037844387076, 1.000000000000000000, 0.8660254037844387076, 1.000000000000000000, 0.9330127018922130810, 0.9330127018922194093 ) ) 
 REPRESENTATION_ITEM ( '' )  );
#47865=CARTESIAN_POINT ( 'NONE',  ( -3.152548672688508926E-16, -28.81249999863440436, -5.148502694627439702 ) ) ;
#47869=CARTESIAN_POINT ( 'NONE',  ( -5.000000000000000000, 16.91666666666666785, -2.886751345948128211 ) ) ;
#47871=CARTESIAN_POINT ( 'NONE',  ( -4.458734124999997661, 9.520833334698927786, 2.574251347313722516 ) ) ;
#47872=ORIENTED_EDGE ( 'NONE', *, *, #2726, .F. ) ;
#47875=CARTESIAN_POINT ( 'NONE',  ( -4.999999999999998224, 16.20833333606451987, 2.886751345948131764 ) ) ;
#47876=CARTESIAN_POINT ( 'NONE',  ( 5.000000000000000000, -88.50000000000000000, -6.123233995736766282E-16 ) ) ;
#47877=CARTESIAN_POINT ( 'NONE',  ( 4.458734125000001214, -26.89583333196774007, 2.574251347313718519 ) ) ;
#47878=DIRECTION ( 'NONE',  ( -0.000000000000000000, 1.000000000000000000, -0.000000000000000000 ) ) ;
#47879=CARTESIAN_POINT ( 'NONE',  ( 4.458734124999998549, -74.97916666530106511, -2.574251347313721627 ) ) ;
#47882=DIRECTION ( 'NONE',  ( -0.000000000000000000, 1.000000000000000000, -0.000000000000000000 ) ) ;
#47883=VECTOR ( 'NONE', #47882, 1000.000000000000000 ) ;
#47885=CARTESIAN_POINT ( 'NONE',  ( 4.458734124999998549, 1.270833334698927342, -2.574251347313721627 ) ) ;
#47886=CARTESIAN_POINT ( 'NONE',  ( 4.458734124999999437, 27.93750000136559208, -5.460374474430324690E-16 ) ) ;
#47887=CARTESIAN_POINT ( 'NONE',  ( -3.152548672688508926E-16, -39.81249999863440081, -5.148502694627439702 ) ) ;
#47890=CARTESIAN_POINT ( 'NONE',  ( -3.152548672688508926E-16, -72.56249999863439371, -5.148502694627439702 ) ) ;
#47893=CARTESIAN_POINT ( 'NONE',  ( 9.457646018065525792E-16, -64.06249999863440792, 5.148502694627439702 ) ) ;
#47894=CARTESIAN_POINT ( 'NONE',  ( -2.499999999999996447, -97.70833333060213022, 4.330127018922195425 ) ) ;
#47898=CARTESIAN_POINT ( 'NONE',  ( 4.458734125000000326, -104.1458333319677365, 2.574251347313718519 ) ) ;
#47900=CARTESIAN_POINT ( 'NONE',  ( -5.000000000000000000, -52.00000000000000711, 0.000000000000000000 ) ) ;
#47901=CARTESIAN_POINT ( 'NONE',  ( 2.499999999999998668, -72.20833333060214443, -4.330127018922193649 ) ) ;
#47913=ORIENTED_EDGE ( 'NONE', *, *, #41458, .T. ) ;
#47920=CARTESIAN_POINT ( 'NONE',  ( -4.458734124999999437, -35.56249999863440792, 0.000000000000000000 ) ) ;
#47923=AXIS2_PLACEMENT_3D ( 'NONE', #22857, #37630, #17070 ) ;
#47931=CARTESIAN_POINT ( 'NONE',  ( -6.972266317189433020E-16, -54.24999999999999289, -5.000000000000000000 ) ) ;
#47934=EDGE_CURVE ( 'NONE', #40505, #42214, #59044, .T. ) ;
#47935=CARTESIAN_POINT ( 'NONE',  ( -4.458734124999998549, -83.47916666530107932, 2.574251347313722516 ) ) ;
#47937=VERTEX_POINT ( 'NONE', #47805 ) ;
#47938=LINE ( 'NONE', #22250, #56331 ) ;
#47939=CARTESIAN_POINT ( 'NONE',  ( 6.158835246850666199E-14, -2.124999997268816276, -4.999999999999999112 ) ) ;
#47942=ORIENTED_EDGE ( 'NONE', *, *, #17820, .T. ) ;
#47943=CARTESIAN_POINT ( 'NONE',  ( -2.499999999999996447, -13.83333333333333570, 4.330127018922195425 ) ) ;
#47944=CARTESIAN_POINT ( 'NONE',  ( 4.458734124999999437, -12.06249999863440081, -5.460374474430324690E-16 ) ) ;
#47950=CARTESIAN_POINT ( 'NONE',  ( 2.229367062499998831, 24.10416666803225993, -3.861377020970580887 ) ) ;
#47952=CARTESIAN_POINT ( 'NONE',  ( 2.229367062500001939, -91.97916666530106511, 3.861377020970579999 ) ) ;
#47955=CARTESIAN_POINT ( 'NONE',  ( -4.458734124999998549, -10.22916666530106866, 2.574251347313722516 ) ) ;
#47956=DIRECTION ( 'NONE',  ( 0.000000000000000000, 0.000000000000000000, 1.000000000000000000 ) ) ;
#47957=CARTESIAN_POINT ( 'NONE',  ( 0.000000000000000000, -120.0000000000000000, 5.000000000000000000 ) ) ;
#47959=CARTESIAN_POINT ( 'NONE',  ( 5.000000000000000888, -38.45833333060213732, 2.886751345948126879 ) ) ;
#47961=CARTESIAN_POINT ( 'NONE',  ( 2.229367062500001939, 19.02083333469892779, 3.861377020970579999 ) ) ;
#47964=CARTESIAN_POINT ( 'NONE',  ( 2.229367062499998831, -55.64583333196773651, -3.861377020970580887 ) ) ;
#47967=CARTESIAN_POINT ( 'NONE',  ( -3.535250795749689387E-16, 10.74999999999999822, -5.773502691896257311 ) ) ;
#47969=CARTESIAN_POINT ( 'NONE',  ( -2.499999999999996447, -45.83333333333333570, 4.330127018922195425 ) ) ;
#47970=CARTESIAN_POINT ( 'NONE',  ( -4.458734124999999437, -46.31249999863440792, 0.000000000000000000 ) ) ;
#47971=CARTESIAN_POINT ( 'NONE',  ( -4.999999999999999112, -81.79166666393547303, 2.886751345948131764 ) ) ;
#47973=VECTOR ( 'NONE', #57864, 1000.000000000000000 ) ;
#47975=CYLINDRICAL_SURFACE ( 'NONE', #48282, 5.000000000000000000 ) ;
#47976=CARTESIAN_POINT ( 'NONE',  ( 1.975475456537005874E-15, -91.74999999999998579, 5.000000000000000000 ) ) ;
#47977=AXIS2_PLACEMENT_3D ( 'NONE', #31203, #8043, #51160 ) ;
#47978=CARTESIAN_POINT ( 'NONE',  ( -3.152548672688508926E-16, -89.81249999863440792, -5.148502694627439702 ) ) ;
#47980=CARTESIAN_POINT ( 'NONE',  ( 2.500000000000002220, -36.66666666666666430, 4.330127018922192761 ) ) ;
#47982=EDGE_LOOP ( 'NONE', ( #6792, #55710, #59178, #22068 ) ) ;
#47985=CARTESIAN_POINT ( 'NONE',  ( -2.229367062500000163, -93.47916666530106511, -3.861377020970580443 ) ) ;
#47986=CARTESIAN_POINT ( 'NONE',  ( 4.458734124999998549, 8.020833334698926009, -2.574251347313721627 ) ) ;
#47987=CARTESIAN_POINT ( 'NONE',  ( 1.060575238724906964E-15, 11.37500000273118594, 5.773502691896257311 ) ) ;
#47991=LINE ( 'NONE', #47681, #36966 ) ;
#47992=EDGE_CURVE ( 'NONE', #16995, #31397, #39754, .T. ) ;
#47993=ADVANCED_FACE ( 'NONE', ( #30077 ), #39726, .T. ) ;
#48001=CARTESIAN_POINT ( 'NONE',  ( -2.229367062499996610, -19.39583333196774007, 3.861377020970582219 ) ) ;
#48002=CARTESIAN_POINT ( 'NONE',  ( 0.000000000000000000, -120.0000000000000000, 5.000000000000000000 ) ) ;
#48007=ADVANCED_FACE ( 'NONE', ( #847 ), #49708, .T. ) ;
#48011=EDGE_CURVE ( 'NONE', #42214, #44744, #29048, .T. ) ;
#48013=CARTESIAN_POINT ( 'NONE',  ( 2.229367062500001939, -70.22916666530107932, 3.861377020970579999 ) ) ;
#48017=ORIENTED_EDGE ( 'NONE', *, *, #58198, .T. ) ;
#48022=CARTESIAN_POINT ( 'NONE',  ( -2.229367062499996610, 0.6041666680322611560, 3.861377020970582219 ) ) ;
#48023=ORIENTED_EDGE ( 'NONE', *, *, #909, .T. ) ;
#48031=CARTESIAN_POINT ( 'NONE',  ( -4.458734124999999437, -78.39583333196772230, -2.574251347313719407 ) ) ;
#48033=CARTESIAN_POINT ( 'NONE',  ( -4.458734124999998549, 8.770833334698927786, 2.574251347313722516 ) ) ;
#48034=CARTESIAN_POINT ( 'NONE',  ( 1.975475456537005874E-15, -15.62499999726881406, 5.000000000000000000 ) ) ;
#48035=CARTESIAN_POINT ( 'NONE',  ( -4.458734124999998549, -59.47916666530106511, 2.574251347313722516 ) ) ;
#48036=CARTESIAN_POINT ( 'NONE',  ( 1.060575238724906964E-15, -20.62499999726880873, 5.773502691896257311 ) ) ;
#48039=CARTESIAN_POINT ( 'NONE',  ( -1.339745962155613812, -106.0803417985302843, -5.000000000000000000 ) ) ;
#48041=CARTESIAN_POINT ( 'NONE',  ( -2.229367062499996610, -42.14583333196773651, 3.861377020970582219 ) ) ;
#48042=CARTESIAN_POINT ( 'NONE',  ( -2.229367062500000163, -27.72916666530107221, -3.861377020970580443 ) ) ;
#48043=FACE_OUTER_BOUND ( 'NONE', #7081, .T. ) ;
#48044=CARTESIAN_POINT ( 'NONE',  ( 5.000000000000000888, 26.41666666666666430, 2.886751345948126879 ) ) ;
#48047=CARTESIAN_POINT ( 'NONE',  ( -3.152548672688508926E-16, -106.8124999986343795, -5.148502694627439702 ) ) ;
#48048=CARTESIAN_POINT ( 'NONE',  ( -4.458734124999999437, -33.31249999863440792, 0.000000000000000000 ) ) ;
#48049=CARTESIAN_POINT ( 'NONE',  ( 2.500000000000002220, -69.54166666393547303, 4.330127018922192761 ) ) ;
#48053=CARTESIAN_POINT ( 'NONE',  ( -3.152548672688508926E-16, -29.56249999863440436, -5.148502694627439702 ) ) ;
#48054=CARTESIAN_POINT ( 'NONE',  ( 4.458734125000000326, -73.14583333196772230, 2.574251347313718519 ) ) ;
#48057=DIRECTION ( 'NONE',  ( -0.000000000000000000, 1.000000000000000000, -0.000000000000000000 ) ) ;
#48059=CARTESIAN_POINT ( 'NONE',  ( 5.000000000000000888, -22.58333333333333215, 2.886751345948126879 ) ) ;
#48061=ORIENTED_EDGE ( 'NONE', *, *, #44085, .T. ) ;
#48062=CARTESIAN_POINT ( 'NONE',  ( 1.975475456537005874E-15, -78.62499999726881583, 5.000000000000000000 ) ) ;
#48064=CARTESIAN_POINT ( 'NONE',  ( 1.975475456537005874E-15, -90.62499999726880162, 5.000000000000000000 ) ) ;
#48074=ORIENTED_EDGE ( 'NONE', *, *, #51594, .F. ) ;
#48080=ORIENTED_EDGE ( 'NONE', *, *, #26824, .F. ) ;
#48083=CARTESIAN_POINT ( 'NONE',  ( 5.000000000000000000, -53.41666666666667140, -2.886751345948130876 ) ) ;
#48086=ORIENTED_EDGE ( 'NONE', *, *, #6693, .F. ) ;
#48087=EDGE_CURVE ( 'NONE', #58058, #12673, #42019, .T. ) ;
#48093=CARTESIAN_POINT ( 'NONE',  ( 4.458734124999998549, -83.72916666530107932, -2.574251347313721627 ) ) ;
#48094=CARTESIAN_POINT ( 'NONE',  ( 9.457646018065525792E-16, 19.93750000136559208, 5.148502694627439702 ) ) ;
#48095=CARTESIAN_POINT ( 'NONE',  ( -1.339745962155613812, -18.08034179853029499, -5.000000000000000000 ) ) ;
#48103=( BOUNDED_CURVE ( )  B_SPLINE_CURVE ( 2, ( #16289, #1832, #21433, #5682, #35909, #874, #46192, #55541, #6964 ),
 .UNSPECIFIED., .F., .F. ) 
 B_SPLINE_CURVE_WITH_KNOTS ( ( 3, 2, 2, 2, 3 ),
 ( 0.02321428571428571508, 0.02380952380952380820, 0.02500000000000000139, 0.02619047619047619110, 0.02678571428571428770 ),
 .UNSPECIFIED. ) 
 CURVE ( )  GEOMETRIC_REPRESENTATION_ITEM ( )  RATIONAL_B_SPLINE_CURVE ( ( 0.9330127018922194093, 0.9330127018922195203, 1.000000000000000000, 0.8660254037844387076, 1.000000000000000000, 0.8660254037844387076, 1.000000000000000000, 0.9330127018922191873, 0.9330127018922194093 ) ) 
 REPRESENTATION_ITEM ( '' )  );
#48105=CARTESIAN_POINT ( 'NONE',  ( -2.229367062500000163, -57.47916666530107932, -3.861377020970580443 ) ) ;
#48107=CARTESIAN_POINT ( 'NONE',  ( -2.229367062500000163, 25.52083333469892779, -3.861377020970580443 ) ) ;
#48108=VECTOR ( 'NONE', #58609, 1000.000000000000000 ) ;
#48109=CARTESIAN_POINT ( 'NONE',  ( 2.499999999999998668, -42.33333333333333570, -4.330127018922193649 ) ) ;
#48111=CARTESIAN_POINT ( 'NONE',  ( 4.458734125000001214, -44.14583333196773651, 2.574251347313718519 ) ) ;
#48112=CARTESIAN_POINT ( 'NONE',  ( 5.000000000000000000, -5.291666663935480130, -2.886751345948129988 ) ) ;
#48113=CARTESIAN_POINT ( 'NONE',  ( -1.339745962155613812, -93.20534180126148271, -5.000000000000000000 ) ) ;
#48116=CARTESIAN_POINT ( 'NONE',  ( -3.152548672688508926E-16, -106.5624999986343937, -5.148502694627439702 ) ) ;
#48117=CARTESIAN_POINT ( 'NONE',  ( 4.458734125000000326, -12.14583333196774007, 2.574251347313718519 ) ) ;
#48118=ORIENTED_EDGE ( 'NONE', *, *, #9960, .F. ) ;
#48120=CARTESIAN_POINT ( 'NONE',  ( -2.229367062500000163, -97.47916666530105090, -3.861377020970580443 ) ) ;
#48122=CARTESIAN_POINT ( 'NONE',  ( -3.152548672688508926E-16, -94.81249999863442213, -5.148502694627439702 ) ) ;
#48123=CARTESIAN_POINT ( 'NONE',  ( 5.000000000000000000, -53.29166666393547303, -2.886751345948129988 ) ) ;
#48128=CARTESIAN_POINT ( 'NONE',  ( 4.458734124999999437, -12.81249999863440259, -5.460374474430324690E-16 ) ) ;
#48129=CARTESIAN_POINT ( 'NONE',  ( -4.458734124999998549, 13.52083333469892779, 2.574251347313722516 ) ) ;
#48130=CARTESIAN_POINT ( 'NONE',  ( -4.458734124999997661, -57.47916666530108643, 2.574251347313722516 ) ) ;
#48131=DIRECTION ( 'NONE',  ( -0.000000000000000000, 1.000000000000000000, -0.000000000000000000 ) ) ;
#48132=CARTESIAN_POINT ( 'NONE',  ( -6.972266317189433020E-16, 6.875000002731185944, -5.000000000000000000 ) ) ;
#48134=CARTESIAN_POINT ( 'NONE',  ( 1.339745962155615144, -106.5803417985302843, 4.999999999999999112 ) ) ;
#48140=CARTESIAN_POINT ( 'NONE',  ( -4.458734124999999437, -87.31249999863439371, 0.000000000000000000 ) ) ;
#48141=CARTESIAN_POINT ( 'NONE',  ( -4.458734124999998549, 19.52083333469893134, 2.574251347313722516 ) ) ;
#48143=EDGE_CURVE ( 'NONE', #15979, #45293, #15552, .T. ) ;
#48144=CARTESIAN_POINT ( 'NONE',  ( -5.000000000000000000, -48.00000000000000000, 0.000000000000000000 ) ) ;
#48147=CARTESIAN_POINT ( 'NONE',  ( -4.999999999999999112, -68.91666666666667140, 2.886751345948131764 ) ) ;
#48150=CARTESIAN_POINT ( 'NONE',  ( 5.000000000000000000, -79.41666666666665719, -2.886751345948130876 ) ) ;
#48162=ORIENTED_EDGE ( 'NONE', *, *, #45342, .F. ) ;
#48165=CARTESIAN_POINT ( 'NONE',  ( 2.229367062499998831, -57.89583333196773651, -3.861377020970580887 ) ) ;
#48168=ORIENTED_EDGE ( 'NONE', *, *, #9514, .T. ) ;
#48171=AXIS2_PLACEMENT_3D ( 'NONE', #9755, #29362, #53517 ) ;
#48173=ORIENTED_EDGE ( 'NONE', *, *, #23271, .F. ) ;
#48176=CARTESIAN_POINT ( 'NONE',  ( 4.458734124999998549, -102.9791666653010651, -2.574251347313721627 ) ) ;
#48181=CARTESIAN_POINT ( 'NONE',  ( 2.229367062499998831, -37.64583333196773651, -3.861377020970580887 ) ) ;
#48183=CARTESIAN_POINT ( 'NONE',  ( 9.457646018065525792E-16, -8.062499998634404363, 5.148502694627439702 ) ) ;
#48184=CARTESIAN_POINT ( 'NONE',  ( -4.458734124999999437, -98.64583333196773651, -2.574251347313719407 ) ) ;
#48186=CARTESIAN_POINT ( 'NONE',  ( -2.229367062500000163, -27.72916666530107221, -3.861377020970580443 ) ) ;
#48190=CARTESIAN_POINT ( 'NONE',  ( -1.339745962155613812, -16.20534180126148271, -5.000000000000000000 ) ) ;
#48193=CARTESIAN_POINT ( 'NONE',  ( 9.457646018065525792E-16, 6.687500001365594748, 5.148502694627439702 ) ) ;
#48195=CARTESIAN_POINT ( 'NONE',  ( -5.000000000000000000, 1.999999999999998224, 0.000000000000000000 ) ) ;
#48197=CARTESIAN_POINT ( 'NONE',  ( -5.000000000000000000, -94.00000000000000000, 0.000000000000000000 ) ) ;
#48198=CARTESIAN_POINT ( 'NONE',  ( -2.229367062499996610, -30.14583333196773651, 3.861377020970582219 ) ) ;
#48200=CARTESIAN_POINT ( 'NONE',  ( 2.229367062500001939, -75.22916666530106511, 3.861377020970579999 ) ) ;
#48201=EDGE_CURVE ( 'NONE', #20975, #14229, #334, .T. ) ;
#48205=CARTESIAN_POINT ( 'NONE',  ( 2.229367062500001939, 3.020833334698928674, 3.861377020970579999 ) ) ;
#48206=CARTESIAN_POINT ( 'NONE',  ( 2.229367062499998831, 27.10416666803225993, -3.861377020970580887 ) ) ;
#48207=CARTESIAN_POINT ( 'NONE',  ( -4.458734124999999437, -43.64583333196773651, -2.574251347313719407 ) ) ;
#48212=CARTESIAN_POINT ( 'NONE',  ( -2.229367062499996610, -71.14583333196773651, 3.861377020970582219 ) ) ;
#48213=CARTESIAN_POINT ( 'NONE',  ( 5.000000000000000000, -102.2916666639354588, -2.886751345948129988 ) ) ;
#48214=CARTESIAN_POINT ( 'NONE',  ( 1.975475456537005874E-15, -41.74999999999999289, 5.000000000000000000 ) ) ;
#48216=CARTESIAN_POINT ( 'NONE',  ( 4.458734124999998549, -106.9791666653010509, -2.574251347313721627 ) ) ;
#48218=CARTESIAN_POINT ( 'NONE',  ( 1.060575238724906964E-15, -52.75000000000000000, 5.773502691896257311 ) ) ;
#48221=ORIENTED_EDGE ( 'NONE', *, *, #815, .T. ) ;
#48230=CARTESIAN_POINT ( 'NONE',  ( 5.000000000000000888, -45.45833333060214443, 2.886751345948126879 ) ) ;
#48232=ORIENTED_EDGE ( 'NONE', *, *, #18815, .F. ) ;
#48236=CARTESIAN_POINT ( 'NONE',  ( 2.229367062500001939, -40.22916666530107221, 3.861377020970579999 ) ) ;
#48238=CARTESIAN_POINT ( 'NONE',  ( 6.123233995736766282E-16, -120.0000000000000000, -5.000000000000000000 ) ) ;
#48241=AXIS2_PLACEMENT_3D ( 'NONE', #14043, #53287, #37876 ) ;
#48245=( BOUNDED_CURVE ( )  B_SPLINE_CURVE ( 2, ( #50367, #35576, #30418, #41025, #31059, #16905, #26560, #6314, #40704 ),
 .UNSPECIFIED., .F., .F. ) 
 B_SPLINE_CURVE_WITH_KNOTS ( ( 3, 2, 2, 2, 3 ),
 ( 0.8589285714285714857, 0.8595238095238095788, 0.8607142857142857650, 0.8619047619047619513, 0.8625000000000000444 ),
 .UNSPECIFIED. ) 
 CURVE ( )  GEOMETRIC_REPRESENTATION_ITEM ( )  RATIONAL_B_SPLINE_CURVE ( ( 0.9330127018922194093, 0.9330127018922256266, 1.000000000000000000, 0.8660254037844387076, 1.000000000000000000, 0.8660254037844387076, 1.000000000000000000, 0.9330127018922194093, 0.9330127018922194093 ) ) 
 REPRESENTATION_ITEM ( '' )  );
#48247=CARTESIAN_POINT ( 'NONE',  ( -4.458734124999999437, -89.56249999863440792, 0.000000000000000000 ) ) ;
#48252=CARTESIAN_POINT ( 'NONE',  ( 5.000000000000000888, -43.58333333333333570, 2.886751345948126879 ) ) ;
#48256=CARTESIAN_POINT ( 'NONE',  ( -2.229367062500000163, -9.729166665301068662, -3.861377020970580443 ) ) ;
#48261=CARTESIAN_POINT ( 'NONE',  ( 4.458734124999999437, 18.93750000136559564, -5.460374474430324690E-16 ) ) ;
#48263=CARTESIAN_POINT ( 'NONE',  ( 2.229367062500001939, -90.97916666530106511, 3.861377020970579999 ) ) ;
#48264=CARTESIAN_POINT ( 'NONE',  ( -5.000000000000000000, -33.87499999726880873, 0.000000000000000000 ) ) ;
#48266=CARTESIAN_POINT ( 'NONE',  ( -2.229367062500000163, -13.47916666530107221, -3.861377020970580443 ) ) ;
#48268=CARTESIAN_POINT ( 'NONE',  ( 0.000000000000000000, -120.0000000000000000, 0.000000000000000000 ) ) ;
#48271=CARTESIAN_POINT ( 'NONE',  ( -2.499999999999996447, -35.70833333060213732, 4.330127018922195425 ) ) ;
#48272=FACE_OUTER_BOUND ( 'NONE', #30210, .T. ) ;
#48273=CARTESIAN_POINT ( 'NONE',  ( -2.229367062500000163, 17.52083333469892779, -3.861377020970580443 ) ) ;
#48274=CARTESIAN_POINT ( 'NONE',  ( 5.000000000000000000, -46.29166666393545881, -2.886751345948130876 ) ) ;
#48276=CARTESIAN_POINT ( 'NONE',  ( -3.152548672688508926E-16, -57.56249999863439371, -5.148502694627439702 ) ) ;
#48279=CARTESIAN_POINT ( 'NONE',  ( -5.000000000000000000, 9.000000000000001776, 0.000000000000000000 ) ) ;
#48281=CARTESIAN_POINT ( 'NONE',  ( 5.000000000000000888, -69.58333333333332860, 2.886751345948126879 ) ) ;
#48282=AXIS2_PLACEMENT_3D ( 'NONE', #53746, #63418, #8750 ) ;
#48283=CARTESIAN_POINT ( 'NONE',  ( 2.229367062500001939, -53.97916666530107221, 3.861377020970579999 ) ) ;
#48284=CARTESIAN_POINT ( 'NONE',  ( -2.499999999999996447, -83.70833333060214443, 4.330127018922195425 ) ) ;
#48286=CARTESIAN_POINT ( 'NONE',  ( 2.500000000000002220, -14.54166666393548191, 4.330127018922192761 ) ) ;
#48287=EDGE_CURVE ( 'NONE', #54583, #43806, #18828, .T. ) ;
#48291=CARTESIAN_POINT ( 'NONE',  ( 2.229367062500001939, -92.22916666530106511, 3.861377020970579999 ) ) ;
#48293=CARTESIAN_POINT ( 'NONE',  ( -5.000000000000000000, -38.99999999999999289, 0.000000000000000000 ) ) ;
#48295=VERTEX_POINT ( 'NONE', #23979 ) ;
#48296=CARTESIAN_POINT ( 'NONE',  ( 2.229367062500001939, -97.97916666530105090, 3.861377020970579999 ) ) ;
#48297=CARTESIAN_POINT ( 'NONE',  ( 2.229367062499998831, 10.10416666803225993, -3.861377020970580887 ) ) ;
#48298=CARTESIAN_POINT ( 'NONE',  ( -2.499999999999996447, 9.291666669397853795, 4.330127018922195425 ) ) ;
#48299=( BOUNDED_CURVE ( )  B_SPLINE_CURVE ( 2, ( #50331, #25564, #6912, #6277, #59670, #45180, #16241, #50648, #1783 ),
 .UNSPECIFIED., .F., .F. ) 
 B_SPLINE_CURVE_WITH_KNOTS ( ( 3, 2, 2, 2, 3 ),
 ( 0.3946428571428571286, 0.3952380952380952217, 0.3964285714285714080, 0.3976190476190475942, 0.3982142857142857428 ),
 .UNSPECIFIED. ) 
 CURVE ( )  GEOMETRIC_REPRESENTATION_ITEM ( )  RATIONAL_B_SPLINE_CURVE ( ( 0.9330127018922194093, 0.9330127018922194093, 1.000000000000000000, 0.8660254037844387076, 1.000000000000000000, 0.8660254037844387076, 1.000000000000000000, 0.9330127018922163007, 0.9330127018922194093 ) ) 
 REPRESENTATION_ITEM ( '' )  );
#48302=EDGE_CURVE ( 'NONE', #5147, #59356, #54842, .T. ) ;
#48307=CARTESIAN_POINT ( 'NONE',  ( -6.972266317189433020E-16, -11.25000000000000178, -5.000000000000000000 ) ) ;
#48308=CARTESIAN_POINT ( 'NONE',  ( -4.458734124999999437, 29.43750000136559208, 0.000000000000000000 ) ) ;
#48309=CARTESIAN_POINT ( 'NONE',  ( -1.336351044127974539E-14, 25.24999999999999645, 5.000000000000000000 ) ) ;
#48311=CARTESIAN_POINT ( 'NONE',  ( -2.500000000000000444, -90.04166666393547303, -4.330127018922193649 ) ) ;
#48312=CARTESIAN_POINT ( 'NONE',  ( -2.229367062499996610, -27.39583333196774007, 3.861377020970582219 ) ) ;
#48321=ORIENTED_EDGE ( 'NONE', *, *, #24179, .F. ) ;
#48324=ORIENTED_EDGE ( 'NONE', *, *, #30823, .T. ) ;
#48325=CARTESIAN_POINT ( 'NONE',  ( 4.458734124999998549, -67.97916666530107932, -2.574251347313721627 ) ) ;
#48327=FILL_AREA_STYLE ('',( #46760 ) ) ;
#48330=( BOUNDED_CURVE ( )  B_SPLINE_CURVE ( 2, ( #15853, #54775, #6209, #1082, #49935, #58955, #5890, #35160, #55418, #20363, #11336, #30959, #59278, #25498, #24545, #39961, #15209, #120, #35476, #5245, #19714, #55093, #11018, #34490, #54124, #10062, #29674, #49306, #54459, #10385, #49627, #22597, #37070, #6844, #27399, #56694, #61198, #61520, #12922, #12610, #7166, #57007, #32223, #51542, #2033, #11647, #27091, #17120, #17450, #36746, #51854, #46708, #31915, #21319, #12299, #41547, #7797, #51230, #47030, #2980, #26457, #21638, #31268, #32543, #2653, #22272, #42194, #16488, #6525, #56051, #60879, #40920, #7478, #46075, #61836, #26776, #41231, #17758, #37374, #26138, #2343, #46395, #11967, #41873, #16803, #21951, #56376, #36423, #31597, #45758, #1710, #60563, #36109, #55732, #50902, #37685, #9354, #14490, #52170, #13869, #13567, #63092, #18387, #9048, #28966, #38006, #28032, #48589, #28657, #43134, #52801, #42507, #42822, #43758, #14177, #47650, #8736, #63403, #8114, #3604, #33185, #27718, #18694, #57948, #47345, #23534, #53111, #38616, #47961, #19319, #57328, #3295, #18063, #23211, #38320, #22914, #28344, #19002, #38935, #58571, #62774, #62467, #43447, #58251, #57639, #33492, #48273, #3916, #4229, #23844, #62144, #33804, #53420, #13243, #4530, #24155, #32866, #52496, #8429, #19639, #34111, #59854, #58875, #15778, #29274, #35395, #39886, #34420, #5806, #9666, #20927, #48904, #6135, #30235, #55017, #49858, #59531, #20613, #40218, #10939, #39, #35082, #25423, #10309, #50183, #1009, #54049, #30558, #25749, #25102, #45042, #40531, #45363, #34757, #1328, #59206, #24788, #60173, #29921, #53733, #4849, #24469, #675, #44074, #10622, #15464, #39249, #54701, #5488, #14806, #15135, #9986, #29598, #49230, #20284, #5170, #49546, #44394, #353, #19955, #39566, #54383, #44712, #6770, #50517, #61129, #36036, #41801, #36351, #50830, #2584, #12537, #16095, #11894, #31841, #16418, #46320, #45999, #21565, #17053, #35718, #1964, #2278, #55348, #16734, #36669, #51473, #41162, #1640, #36994, #42117, #11262, #41478, #60807, #21882, #27020, #7410, #51157, #32148, #56621, #45683, #56298, #7091, #55981, #6457, #26381, #12226, #30886, #11582, #31514, #26705, #26066, #46638, #21240, #22202, #27331, #40847, #51784, #60490, #61445, #17373, #7726, #46962, #2907, #22522, #55668, #31201, #27646, #33109, #52725, #3843, #33730, #9283, #37612, #53036, #8974, #57253, #8657, #43066, #13169, #42746, #12852, #4158, #3221, #61759, #23138, #32471, #33417, #57568, #57873, #28584, #48519, #18929, #23775, #22839, #43377, #56931, #63022, #23463, #62072, #48205, #37935, #28899, #28270, #42430, #38545, #24087, #8355, #4460, #52100, #17687, #17986, #18310, #58175, #27957, #37302, #14105, #18630, #8041, #52423, #13797, #47885, #53348, #47273, #32794, #62389, #47577, #13493, #3529, #62704, #38252, #35012, #58497, #5735, #4771, #14421, #20539, #63647, #602, #34352, #15704, #49789, #24716, #40136, #936, #43999, #29844, #44971, #19883, #19566, #39178, #59455, #15387, #54625, #15068, #10241, #49477, #58803, #53982, #59780, #39496, #14735, #30160, #35322, #43682, #59132, #10550, #9911, #5415, #29519, #49153, #25353, #44320, #54943, #10870, #5097, #25032, #30487, #34680, #284, #54299, #50109, #53665, #6064, #44642, #20212, #34043, #39814, #63328, #19245, #38861, #9598, #29206, #48831, #24398, #21489, #41403, #25989, #55904, #55591, #31126, #16655, #35965, #11510, #11815, #1252, #26299, #7015, #61055, #50749, #11190, #46565, #51709, #25678, #51076, #6694, #31434, #36586, #16975, #60734, #41715, #1563, #22123, #2204, #36280, #45923, #16018, #16343, #17287, #51395, #21165, #1886, #36911, #45286, #40772, #41087, #40457, #31762, #30812, #20855, #26623, #46243, #12142, #21808, #56542, #50444, #60097, #55271, #60418, #56222, #35645, #7337, #26948, #12461, #32072, #2505, #61366, #6384, #45608, #52021, #52957, #17915, #58096, #61681, #27253, #7965, #27879, #28510, #37536, #7650, #18552, #28192, #42040, #61995, #3764, #47500, #46880, #62309, #23388, #27563, #2824, #32713, #57176, #8895, #3451, #62630, #22443, #33341, #32395, #17613, #48128, #47196, #47807, #13094, #43299, #42670, #23702, #4079, #37229, #18233, #37858, #8275, #56855, #52341, #62935, #18849, #3140, #23065, #38470, #12773, #22759, #57491, #42356, #13717, #13410, #33031, #52647, #8581, #42988, #38174, #57796, #14026, #33655, #19161, #29124, #39411, #24001, #29434, #519, #44889, #59696, #44240, #49067, #20454, #204, #33967, #34924, #15627, #63565, #40052, #43603, #15302, #38779, #34272, #54217, #49394, #5014, #5656, #20129, #53587, #10468, #39729, #19802, #44561, #53273, #59368, #53898, #54545, #14653, #43918, #30080, #58418, #10155, #59049, #49711, #14977, #25269, #29760, #34585, #4382, #5338, #24633, #850, #9823, #9208, #28821, #9517, #24956, #48442, #63247, #48747, #14345, #4689, #24311, #19485, #39098, #58727, #5987, #16581, #55188, #60974, #55514, #6303, #21732, #31687, #35244, #31047, #50997, #35564, #1807, #1486, #50671, #26225, #45525, #21089, #21411, #10794, #35885, #36201, #6937, #60338, #20772, #56142, #61288, #54863, #60658, #16266, #41014, #46168, #26548, #11109, #16895, #30733, #11429, #46486, #30406, #50355, #6612, #50030, #41327, #40377, #25592, #45845, #45206, #2130, #55823, #31356, #36511, #22043, #12062, #51322, #11738, #1172, #7260, #26873, #2433, #41636, #60018, #15942, #25907, #40693, #61607, #62558, #44088, #27491, #4862, #7571, #36837, #17541, #37467, #38100, #13336, #57100, #33270, #47740, #37161, #57724, #3696, #8203, #8512, #24482, #23310, #17844, #42911, #42285, #7887, #18478, #13017, #28122, #32003, #13650, #47431, #52889, #57415, #42601, #51637, #23000, #52266, #8825, #61925, #28439, #48053, #56784, #3383, #17210, #32636, #12703, #32317, #32956, #52581, #56467, #3068, #47120, #27183, #62238, #51947, #12389, #27806, #22685, #46799, #2746, #22365, #18157, #41965, #37784, #39897, #34769, #54395, #54715, #19651, #367, #59543, #39263, #29934, #10635, #5818, #10322, #10000, #35408, #20939, #53, #30247, #5500, #49871, #59867, #1021, #15478, #25763, #50195, #5186, #35094, #25436, #25114, #29612, #49559, #49242, #20297, #15791, #1340, #58888, #45054, #20626, #14819, #40232, #39579, #6147, #34433, #44725, #54061, #59217, #44407, #55029, #24802, #10953, #19969, #15149, #687, #45375, #30572, #53639, #33706, #56672, #48496, #9572, #13770, #51832, #44294, #43971, #38833, #53007, #61810, #7774, #19538, #17736, #27377, #34326, #33392, #14395, #48181, #29488, #53951, #24060, #8946, #24369, #4433, #47010, #28560, #37354, #19854, #34017, #29179, #48805, #4744, #28874, #43657, #63298, #4133, #23755, #9882, #53326, #63617, #56984, #39152, #43350, #2959, #62996, #38520, #18906, #58777, #58148, #9259, #12590, #14077, #19216, #58470, #22576, #14707, #42173, #49124, #5066, #24686, #256, #32203, #30457, #6356, #50408, #25960, #5708, #60066, #60390, #25323, #5389, #10841, #50082, #45260, #11480, #50721, #15357, #30785, #45577, #34982, #6039, #20825, #54597, #20508, #59750, #15032, #25644, #1226, #39468, #40426, #11163, #35294, #35615, #1533, #26272, #16316, #21138, #574, #34648, #40107, #15990, #55241, #901, #25004, #35937, #1856, #59105, #40743, #15675, #55565, #44943, #31100, #6665, #54914, #10519, #45894, #54272, #10212, #29815, #49447, #30133, #44614, #20183, #49762, #39781, #59428, #49765, #6042, #45262, #577, #30136, #25008, #50086, #39785, #60394, #20828, #21141, #16319, #11792, #45898, #50724, #5711, #6668, #20186, #26275, #30788, #25326, #35940, #59433, #31410, #15994, #44947, #1859, #51048, #35297, #44617, #15360, #34985, #905, #1229, #21465, #54918, #54600, #55568, #45580, #10522, #15678, #40746, #40429, #20513, #40110, #11484, #25648, #31103, #60069, #10844, #41064, #35618, #60711, #59753, #16632, #30460, #55245, #36253, #11165, #1536, #50413, #55881, #6359, #25963, #47477, #27857, #7313, #56835, #8256, #46854, #26925, #46542, #22736, #42335, #17894, #42018, #37209, #12752, #22097, #61342, #23046, #2800, #61974, #12116, #3431, #6993, #22420, #37515, #2484, #32374, #36889, #12439, #51997, #26603, #41694, #17264, #32051, #42650, #7939, #56518, #57156, #61659, #41380, #51687, #17592, #7628, #27232, #13070, #32689, #52321, #27543, #47174, #3117, #62291, #18213, #37836, #57468, #13387, #31741, #33008, #46219, #2182, #51373, #21786, #61026, #16951, #36564, #56195, #8559, #48105, #62914, #58073, #62607, #48726, #47786, #4666, #182, #23366, #29410, #33317, #43582, #19462, #63541, #39077, #24290, #23978, #4989, #49043, #18530, #63224, #19139, #58394, #24611, #19782, #28488, #43892, #58705, #44217, #14632, #39390, #13696, #33632, #9187, #28171, #14322, #52626, #38756, #53564, #34246, #48415, #59021, #38150, #3744, #57775, #4058, #33943, #42964, #28800, #53875, #14952, #52936, #9489, #4359, #8873, #23676, #9802, #43274, #18827, #29100, #38446, #14005, #53251, #496, #15603, #35539, #30707, #10772, #50650, #1464, #34901, #55488, #21066, #25567, #25885, #50332, #54523, #29738, #21386, #40671, #15917, #30061, #39706, #55166, #45182, #45501, #1148, #60316, #11085, #59994, #49370, #40353, #10132, #6588, #6279, #60636, #44860, #40992, #24932, #54193, #10446, #54841, #11404, #823, #34563, #16243, #35863, #5315, #25245, #31023, #30382, #44540, #20748, #26203, #49688, #45822, #59672, #20429, #1786, #50005, #20100, #59346, #15278, #5634, #40029, #35221, #5956, #37138, #7237, #52239, #57076, #46776, #31665, #47097, #7548, #2722, #17821, #56445, #16871, #36489, #32295, #51922, #27468, #51615, #22344, #41942, #51302, #26851, #32612, #12366, #7862, #21710, #61902, #46464, #11718, #3045, #56116, #61584, #2407, #22021, #17519, #36180, #12040, #41614, #61265, #26526, #12681, #31335, #22663, #27783, #50972, #12990, #60952, #27160, #42261, #56759, #37445, #8180, #47408, #3358, #22975, #46145, #42576, #16556, #55801, #6914, #2109, #17188, #41302, #36814, #31981, #58321, #34175, #23285, #43198, #13312, #4594, #3672, #62215, #23601, #32934, #33870, #58006, #14247, #53488, #48966, #19388, #24217, #42887, #43824, #57390, #63469, #4289, #62532, #9417, #38380, #29336, #39006, #24537, #18132, #23907, #62840, #48343, #29027, #48652, #33557, #14556, #58637, #28098, #53179, #9112, #43508, #53798, #9732, #38074, #4918, #57702, #18452, #37758, #28720, #52557, #18755, #8490, #47716, #13628, #33246, #13932, #52866, #8799, #63154, #28412, #48031, #3982, #19064, #38682, #30306, #14873, #20353, #55086, #35787, #50576, #35152, #39951, #11326, #54767, #24860, #25815, #54449, #49926, #30630, #50252, #6200, #10054, #25167, #45109, #44140, #11008, #1074, #34482, #34826, #40286, #59599, #111, #10697, #59924, #421, #39315, #30950, #45428, #25487, #39631, #49298, #20680, #5880, #35466, #58943, #20993, #20025, #15847, #10377, #16160, #40598, #1393, #59270, #60242, #55409, #54116, #15201, #5238, #6519, #19706, #29667, #44462, #29986, #49618, #5555, #44781, #743, #15532, #42186, #21942, #61512, #31262, #7787, #36415, #21309, #50896, #7159, #31589, #22265, #41224, #41540, #17114, #56045, #11961, #1705, #26769, #7473, #41865, #51223, #11641, #36738, #17441, #56369, #51844, #2646, #51536, #40913, #31907, #61192, #32215, #46389, #2972, #47023, #26447, #21632, #6839, #52163, #37059, #56686, #61826, #36101, #32534, #2336, #16797, #60558, #27083, #46067, #27390, #12292, #60871, #12602, #22589, #26131, #46698, #17750, #37367, #56998, #12912, #45751, #16480, #55726, #2027, #57939, #47337, #8724, #53102, #23835, #33176, #57317, #28957, #34101, #8106, #33481, #52791, #18992, #37997, #28648, #48580, #57629, #47641, #4521, #48263, #62765, #28337, #62135, #62456, #63393, #33795, #3596, #13234, #24146, #43125, #63082, #47952, #3287, #38311, #13857, #27710, #18685, #9037, #58240, #3905, #19311, #32857, #22903, #37675, #23201, #4221, #42498, #23524, #38607, #38926, #14480, #43438, #58560, #18054, #13558, #14168, #53412, #18376, #9343, #43749, #52486, #8419, #28022, #42814, #54691, #50736, #29910, #7004, #21477, #54039, #11805, #41075, #53726, #44701, #6680, #9977, #48895, #41392, #60721, #35073, #49220, #58866, #10613, #39876, #24459, #49537, #1872, #46230, #61041, #666, #5478, #21797, #59198, #25093, #20275, #344, #59521, #16644, #36267, #55892, #19630, #34747, #31114, #26287, #15456, #26613, #31421, #29589, #51060, #2193, #45909, #16964, #9657, #5160, #4839, #29266, #44064, #30, #24780, #14798, #39240, #34410, #44384, #19944, #39556, #15126, #54374, #10301, #42346, #7952, #42661, #17603, #3441, #27553, #7326, #32062, #61353, #62618, #13081, #52331, #8570, #46553, #42976, #22432, #27243, #26936, #17903, #56530, #62300, #56845, #7639, #23056, #46868, #31751, #41705, #37219, #42029, #32702, #51698, #52010, #47185, #2811, #61670, #22748, #12129, #12762, #37525, #8266, #32385, #22112, #57481, #36575, #3127, #18222, #47488, #37848, #61984, #57166, #13397, #27868, #12451, #33020, #52636, #28181, #47797, #2496, #3754, #23376, #56205, #51384, #17276, #36900, #43287, #63235, #38766, #57786, #48734, #24299, #18542, #53575, #19471, #5001, #14333, #29748, #4068, #38161, #48116, #58084, #39398, #48428, #14015, #14964, #9502, #43903, #54203, #49379, #33642, #9811, #29421, #10141, #14641, #5324, #62923, #19149, #58405, #13706, #4677, #63551, #33328, #29111, #39085, #24620, #34258, #53886, #24943, #59033, #44226, #18838, #192, #52947, #19791, #58715, #38456, #49052, #8883, #44549, #28497, #23988, #33954, #34572, #28809, #23687 ),
 .UNSPECIFIED., .F., .F. ) 
 B_SPLINE_CURVE_WITH_KNOTS ( ( 3, 2, 2, 2, 2, 2, 2, 2, 2, 2, 2, 2, 2, 2, 2, 2, 2, 2, 2, 2, 2, 2, 2, 2, 2, 2, 2, 2, 2, 2, 2, 2, 2, 2, 2, 2, 2, 2, 2, 2, 2, 2, 2, 2, 2, 2, 2, 2, 2, 2, 2, 2, 2, 2, 2, 2, 2, 2, 2, 2, 2, 2, 2, 2, 2, 2, 2, 2, 2, 2, 2, 2, 2, 2, 2, 2, 2, 2, 2, 2, 2, 2, 2, 2, 2, 2, 2, 2, 2, 2, 2, 2, 2, 2, 2, 2, 2, 2, 2, 2, 2, 2, 2, 2, 2, 2, 2, 2, 2, 2, 2, 2, 2, 2, 2, 2, 2, 2, 2, 2, 2, 2, 2, 2, 2, 2, 2, 2, 2, 2, 2, 2, 2, 2, 2, 2, 2, 2, 2, 2, 2, 2, 2, 2, 2, 2, 2, 2, 2, 2, 2, 2, 2, 2, 2, 2, 2, 2, 2, 2, 2, 2, 2, 2, 2, 2, 2, 2, 2, 2, 2, 2, 2, 2, 2, 2, 2, 2, 2, 2, 2, 2, 2, 2, 2, 2, 2, 2, 2, 2, 2, 2, 2, 2, 2, 2, 2, 2, 2, 2, 2, 2, 2, 2, 2, 2, 2, 2, 2, 2, 2, 2, 2, 2, 2, 2, 2, 2, 2, 2, 2, 2, 2, 2, 2, 2, 2, 2, 2, 2, 2, 2, 2, 2, 2, 2, 2, 2, 2, 2, 2, 2, 2, 2, 2, 2, 2, 2, 2, 2, 2, 2, 2, 2, 2, 2, 2, 2, 2, 2, 2, 2, 2, 2, 2, 2, 2, 2, 2, 2, 2, 2, 2, 2, 2, 2, 2, 2, 2, 2, 2, 2, 2, 2, 2, 2, 2, 2, 2, 2, 2, 2, 2, 2, 2, 2, 2, 2, 2, 2, 2, 2, 2, 2, 2, 2, 2, 2, 2, 2, 2, 2, 2, 2, 2, 2, 2, 2, 2, 2, 2, 2, 2, 2, 2, 2, 2, 2, 2, 2, 2, 2, 2, 2, 2, 2, 2, 2, 2, 2, 2, 2, 2, 2, 2, 2, 2, 2, 2, 2, 2, 2, 2, 2, 2, 2, 2, 2, 2, 2, 2, 2, 2, 2, 2, 2, 2, 2, 2, 2, 2, 2, 2, 2, 2, 2, 2, 2, 2, 2, 2, 2, 2, 2, 2, 2, 2, 2, 2, 2, 2, 2, 2, 2, 2, 2, 2, 2, 2, 2, 2, 2, 2, 2, 2, 2, 2, 2, 2, 2, 2, 2, 2, 2, 2, 2, 2, 2, 2, 2, 2, 2, 2, 2, 2, 2, 2, 2, 2, 2, 2, 2, 2, 2, 2, 2, 2, 2, 2, 2, 2, 2, 2, 2, 2, 2, 2, 2, 2, 2, 2, 2, 2, 2, 2, 2, 2, 2, 2, 2, 2, 2, 2, 2, 2, 2, 2, 2, 2, 2, 2, 2, 2, 2, 2, 2, 2, 2, 2, 2, 2, 2, 2, 2, 2, 2, 2, 2, 2, 2, 2, 2, 2, 2, 2, 2, 2, 2, 2, 2, 2, 2, 2, 2, 2, 2, 2, 2, 2, 2, 2, 2, 2, 2, 2, 2, 2, 2, 2, 2, 2, 2, 2, 2, 2, 2, 2, 2, 2, 2, 2, 2, 2, 2, 2, 2, 2, 2, 2, 2, 2, 2, 2, 2, 2, 2, 2, 2, 2, 2, 2, 2, 2, 2, 2, 2, 2, 2, 2, 2, 2, 2, 2, 2, 2, 2, 2, 2, 2, 2, 2, 2, 2, 2, 2, 2, 2, 2, 2, 2, 2, 2, 2, 2, 2, 2, 2, 2, 2, 2, 2, 2, 2, 2, 2, 2, 2, 2, 2, 2, 2, 2, 2, 2, 2, 2, 2, 2, 2, 2, 2, 2, 2, 2, 2, 2, 2, 2, 2, 2, 2, 2, 2, 2, 2, 2, 2, 2, 2, 2, 2, 2, 2, 2, 2, 2, 2, 2, 2, 2, 2, 2, 2, 2, 2, 2, 2, 2, 2, 2, 2, 2, 2, 2, 2, 2, 2, 2, 2, 2, 2, 2, 2, 2, 2, 2, 2, 2, 2, 2, 2, 2, 2, 2, 2, 2, 2, 2, 2, 2, 2, 2, 2, 2, 2, 2, 2, 2, 2, 2, 2, 2, 2, 2, 2, 2, 2, 2, 2, 2, 2, 2, 2, 2, 2, 2, 2, 2, 2, 2, 2, 2, 2, 2, 2, 2, 2, 2, 2, 2, 2, 2, 2, 2, 2, 2, 2, 2, 2, 2, 2, 2, 2, 2, 2, 2, 2, 2, 2, 2, 2, 2, 2, 2, 2, 2, 2, 2, 2, 2, 2, 2, 2, 2, 2, 2, 2, 2, 2, 2, 2, 2, 2, 2, 2, 2, 2, 2, 2, 2, 2, 2, 2, 2, 2, 2, 2, 2, 2, 2, 2, 2, 2, 2, 2, 2, 2, 2, 2, 2, 2, 2, 2, 2, 2, 2, 2, 2, 2, 2, 2, 2, 2, 2, 2, 2, 2, 2, 2, 2, 2, 2, 2, 2, 2, 2, 2, 2, 2, 2, 2, 2, 2, 2, 2, 2, 2, 2, 2, 2, 2, 2, 2, 2, 2, 2, 2, 2, 2, 2, 3 ),
 ( 0.000000000000000000, 0.001190476190476190584, 0.002380952380952381167, 0.003571428571428571317, 0.004761904761904762334, 0.005952380952380952051, 0.007142857142857142634, 0.008333333333333333218, 0.009523809523809524669, 0.01071428571428571438, 0.01190476190476190410, 0.01309523809523809555, 0.01428571428571428527, 0.01547619047619047672, 0.01666666666666666644, 0.01785714285714285615, 0.01904761904761904934, 0.02023809523809523905, 0.02142857142857142877, 0.02261904761904761849, 0.02380952380952380820, 0.02500000000000000139, 0.02619047619047619110, 0.02738095238095238082, 0.02857142857142857054, 0.02976190476190476025, 0.03095238095238095344, 0.03214285714285713969, 0.03333333333333333287, 0.03452380952380952606, 0.03571428571428571230, 0.03690476190476190549, 0.03809523809523809867, 0.03928571428571428492, 0.04047619047619047811, 0.04166666666666666435, 0.04285714285714285754, 0.04404761904761905073, 0.04523809523809523697, 0.04642857142857143016, 0.04761904761904761640, 0.04880952380952380959, 0.05000000000000000278, 0.05119047619047618902, 0.05238095238095238221, 0.05357142857142856845, 0.05476190476190476164, 0.05595238095238095483, 0.05714285714285714107, 0.05833333333333333426, 0.05952380952380952051, 0.06071428571428571369, 0.06190476190476190688, 0.06309523809523809312, 0.06428571428571427937, 0.06547619047619047949, 0.06666666666666666574, 0.06785714285714285199, 0.06904761904761905211, 0.07023809523809523836, 0.07142857142857142461, 0.07261904761904762473, 0.07380952380952381098, 0.07499999999999999722, 0.07619047619047619735, 0.07738095238095238360, 0.07857142857142856984, 0.07976190476190475609, 0.08095238095238095621, 0.08214285714285714246, 0.08333333333333332871, 0.08452380952380952883, 0.08571428571428571508, 0.08690476190476190133, 0.08809523809523810145, 0.08928571428571428770, 0.09047619047619047394, 0.09166666666666666019, 0.09285714285714286031, 0.09404761904761904656, 0.09523809523809523281, 0.09642857142857143293, 0.09761904761904761918, 0.09880952380952380543, 0.1000000000000000056, 0.1011904761904761918, 0.1023809523809523780, 0.1035714285714285782, 0.1047619047619047644, 0.1059523809523809507, 0.1071428571428571369, 0.1083333333333333370, 0.1095238095238095233, 0.1107142857142857095, 0.1119047619047619097, 0.1130952380952380959, 0.1142857142857142821, 0.1154761904761904823, 0.1166666666666666685, 0.1178571428571428548, 0.1190476190476190410, 0.1202380952380952411, 0.1214285714285714274, 0.1226190476190476136, 0.1238095238095238138, 0.1250000000000000000, 0.1261904761904761862, 0.1273809523809523725, 0.1285714285714285587, 0.1297619047619047727, 0.1309523809523809590, 0.1321428571428571452, 0.1333333333333333315, 0.1345238095238095177, 0.1357142857142857040, 0.1369047619047619180, 0.1380952380952381042, 0.1392857142857142905, 0.1404761904761904767, 0.1416666666666666630, 0.1428571428571428492, 0.1440476190476190355, 0.1452380952380952495, 0.1464285714285714357, 0.1476190476190476220, 0.1488095238095238082, 0.1499999999999999944, 0.1511904761904761807, 0.1523809523809523947, 0.1535714285714285809, 0.1547619047619047672, 0.1559523809523809534, 0.1571428571428571397, 0.1583333333333333259, 0.1595238095238095122, 0.1607142857142857262, 0.1619047619047619124, 0.1630952380952380987, 0.1642857142857142849, 0.1654761904761904712, 0.1666666666666666574, 0.1678571428571428437, 0.1690476190476190577, 0.1702380952380952439, 0.1714285714285714302, 0.1726190476190476164, 0.1738095238095238027, 0.1749999999999999889, 0.1761904761904762029, 0.1773809523809523891, 0.1785714285714285754, 0.1797619047619047616, 0.1809523809523809479, 0.1821428571428571341, 0.1833333333333333204, 0.1845238095238095344, 0.1857142857142857206, 0.1869047619047619069, 0.1880952380952380931, 0.1892857142857142794, 0.1904761904761904656, 0.1916666666666666796, 0.1928571428571428659, 0.1940476190476190521, 0.1952380952380952384, 0.1964285714285714246, 0.1976190476190476109, 0.1988095238095237971, 0.2000000000000000111, 0.2011904761904761973, 0.2023809523809523836, 0.2035714285714285698, 0.2047619047619047561, 0.2059523809523809423, 0.2071428571428571563, 0.2083333333333333426, 0.2095238095238095288, 0.2107142857142857151, 0.2119047619047619013, 0.2130952380952380876, 0.2142857142857142738, 0.2154761904761904878, 0.2166666666666666741, 0.2178571428571428603, 0.2190476190476190466, 0.2202380952380952328, 0.2214285714285714191, 0.2226190476190476053, 0.2238095238095238193, 0.2250000000000000056, 0.2261904761904761918, 0.2273809523809523780, 0.2285714285714285643, 0.2297619047619047505, 0.2309523809523809645, 0.2321428571428571508, 0.2333333333333333370, 0.2345238095238095233, 0.2357142857142857095, 0.2369047619047618958, 0.2380952380952380820, 0.2392857142857142960, 0.2404761904761904823, 0.2416666666666666685, 0.2428571428571428548, 0.2440476190476190410, 0.2452380952380952273, 0.2464285714285714413, 0.2476190476190476275, 0.2488095238095238138, 0.2500000000000000000, 0.2511904761904761862, 0.2523809523809523725, 0.2535714285714285587, 0.2547619047619047450, 0.2559523809523809312, 0.2571428571428571175, 0.2583333333333333592, 0.2595238095238095455, 0.2607142857142857317, 0.2619047619047619180, 0.2630952380952381042, 0.2642857142857142905, 0.2654761904761904767, 0.2666666666666666630, 0.2678571428571428492, 0.2690476190476190355, 0.2702380952380952217, 0.2714285714285714080, 0.2726190476190475942, 0.2738095238095238360, 0.2750000000000000222, 0.2761904761904762085, 0.2773809523809523947, 0.2785714285714285809, 0.2797619047619047672, 0.2809523809523809534, 0.2821428571428571397, 0.2833333333333333259, 0.2845238095238095122, 0.2857142857142856984, 0.2869047619047618847, 0.2880952380952380709, 0.2892857142857143127, 0.2904761904761904989, 0.2916666666666666852, 0.2928571428571428714, 0.2940476190476190577, 0.2952380952380952439, 0.2964285714285714302, 0.2976190476190476164, 0.2988095238095238027, 0.2999999999999999889, 0.3011904761904761751, 0.3023809523809523614, 0.3035714285714285476, 0.3047619047619047894, 0.3059523809523809756, 0.3071428571428571619, 0.3083333333333333481, 0.3095238095238095344, 0.3107142857142857206, 0.3119047619047619069, 0.3130952380952380931, 0.3142857142857142794, 0.3154761904761904656, 0.3166666666666666519, 0.3178571428571428381, 0.3190476190476190244, 0.3202380952380952106, 0.3214285714285714524, 0.3226190476190476386, 0.3238095238095238249, 0.3250000000000000111, 0.3261904761904761973, 0.3273809523809523836, 0.3285714285714285698, 0.3297619047619047561, 0.3309523809523809423, 0.3321428571428571286, 0.3333333333333333148, 0.3345238095238095011, 0.3357142857142856873, 0.3369047619047619291, 0.3380952380952381153, 0.3392857142857143016, 0.3404761904761904878, 0.3416666666666666741, 0.3428571428571428603, 0.3440476190476190466, 0.3452380952380952328, 0.3464285714285714191, 0.3476190476190476053, 0.3488095238095237915, 0.3499999999999999778, 0.3511904761904761640, 0.3523809523809524058, 0.3535714285714285920, 0.3547619047619047783, 0.3559523809523809645, 0.3571428571428571508, 0.3583333333333333370, 0.3595238095238095233, 0.3607142857142857095, 0.3619047619047618958, 0.3630952380952380820, 0.3642857142857142683, 0.3654761904761904545, 0.3666666666666666408, 0.3678571428571428825, 0.3690476190476190688, 0.3702380952380952550, 0.3714285714285714413, 0.3726190476190476275, 0.3738095238095238138, 0.3750000000000000000, 0.3761904761904761862, 0.3773809523809523725, 0.3785714285714285587, 0.3797619047619047450, 0.3809523809523809312, 0.3821428571428571175, 0.3833333333333333592, 0.3845238095238095455, 0.3857142857142857317, 0.3869047619047619180, 0.3880952380952381042, 0.3892857142857142905, 0.3904761904761904767, 0.3916666666666666630, 0.3928571428571428492, 0.3940476190476190355, 0.3952380952380952217, 0.3964285714285714080, 0.3976190476190475942, 0.3988095238095238360, 0.4000000000000000222, 0.4011904761904762085, 0.4023809523809523947, 0.4035714285714285809, 0.4047619047619047672, 0.4059523809523809534, 0.4071428571428571397, 0.4083333333333333259, 0.4095238095238095122, 0.4107142857142856984, 0.4119047619047618847, 0.4130952380952380709, 0.4142857142857143127, 0.4154761904761904989, 0.4166666666666666852, 0.4178571428571428714, 0.4190476190476190577, 0.4202380952380952439, 0.4214285714285714302, 0.4226190476190476164, 0.4238095238095238027, 0.4249999999999999889, 0.4261904761904761751, 0.4273809523809523614, 0.4285714285714285476, 0.4297619047619047894, 0.4309523809523809756, 0.4321428571428571619, 0.4333333333333333481, 0.4345238095238095344, 0.4357142857142857206, 0.4369047619047619069, 0.4380952380952380931, 0.4392857142857142794, 0.4404761904761904656, 0.4416666666666666519, 0.4428571428571428381, 0.4440476190476190244, 0.4452380952380952106, 0.4464285714285714524, 0.4476190476190476386, 0.4488095238095238249, 0.4500000000000000111, 0.4511904761904761973, 0.4523809523809523836, 0.4535714285714285698, 0.4547619047619047561, 0.4559523809523809423, 0.4571428571428571286, 0.4583333333333333148, 0.4595238095238095011, 0.4607142857142856873, 0.4619047619047619291, 0.4630952380952381153, 0.4642857142857143016, 0.4654761904761904878, 0.4666666666666666741, 0.4678571428571428603, 0.4690476190476190466, 0.4702380952380952328, 0.4714285714285714191, 0.4726190476190476053, 0.4738095238095237915, 0.4749999999999999778, 0.4761904761904761640, 0.4773809523809524058, 0.4785714285714285920, 0.4797619047619047783, 0.4809523809523809645, 0.4821428571428571508, 0.4833333333333333370, 0.4845238095238095233, 0.4857142857142857095, 0.4869047619047618958, 0.4880952380952380820, 0.4892857142857142683, 0.4904761904761904545, 0.4916666666666666408, 0.4928571428571428825, 0.4940476190476190688, 0.4952380952380952550, 0.4964285714285714413, 0.4976190476190476275, 0.4988095238095238138, 0.5000000000000000000, 0.5011904761904761862, 0.5023809523809523725, 0.5035714285714285587, 0.5047619047619047450, 0.5059523809523809312, 0.5071428571428571175, 0.5083333333333333037, 0.5095238095238094900, 0.5107142857142856762, 0.5119047619047618625, 0.5130952380952380487, 0.5142857142857142350, 0.5154761904761904212, 0.5166666666666667185, 0.5178571428571429047, 0.5190476190476190910, 0.5202380952380952772, 0.5214285714285714635, 0.5226190476190476497, 0.5238095238095238360, 0.5250000000000000222, 0.5261904761904762085, 0.5273809523809523947, 0.5285714285714285809, 0.5297619047619047672, 0.5309523809523809534, 0.5321428571428571397, 0.5333333333333333259, 0.5345238095238095122, 0.5357142857142856984, 0.5369047619047618847, 0.5380952380952380709, 0.5392857142857142572, 0.5404761904761904434, 0.5416666666666666297, 0.5428571428571428159, 0.5440476190476190022, 0.5452380952380951884, 0.5464285714285713746, 0.5476190476190476719, 0.5488095238095238582, 0.5500000000000000444, 0.5511904761904762307, 0.5523809523809524169, 0.5535714285714286031, 0.5547619047619047894, 0.5559523809523809756, 0.5571428571428571619, 0.5583333333333333481, 0.5595238095238095344, 0.5607142857142857206, 0.5619047619047619069, 0.5630952380952380931, 0.5642857142857142794, 0.5654761904761904656, 0.5666666666666666519, 0.5678571428571428381, 0.5690476190476190244, 0.5702380952380952106, 0.5714285714285713969, 0.5726190476190475831, 0.5738095238095237693, 0.5749999999999999556, 0.5761904761904761418, 0.5773809523809523281, 0.5785714285714286254, 0.5797619047619048116, 0.5809523809523809978, 0.5821428571428571841, 0.5833333333333333703, 0.5845238095238095566, 0.5857142857142857428, 0.5869047619047619291, 0.5880952380952381153, 0.5892857142857143016, 0.5904761904761904878, 0.5916666666666666741, 0.5928571428571428603, 0.5940476190476190466, 0.5952380952380952328, 0.5964285714285714191, 0.5976190476190476053, 0.5988095238095237915, 0.5999999999999999778, 0.6011904761904761640, 0.6023809523809523503, 0.6035714285714285365, 0.6047619047619047228, 0.6059523809523809090, 0.6071428571428570953, 0.6083333333333332815, 0.6095238095238095788, 0.6107142857142857650, 0.6119047619047619513, 0.6130952380952381375, 0.6142857142857143238, 0.6154761904761905100, 0.6166666666666666963, 0.6178571428571428825, 0.6190476190476190688, 0.6202380952380952550, 0.6214285714285714413, 0.6226190476190476275, 0.6238095238095238138, 0.6250000000000000000, 0.6261904761904761862, 0.6273809523809523725, 0.6285714285714285587, 0.6297619047619047450, 0.6309523809523809312, 0.6321428571428571175, 0.6333333333333333037, 0.6345238095238094900, 0.6357142857142856762, 0.6369047619047618625, 0.6380952380952380487, 0.6392857142857142350, 0.6404761904761904212, 0.6416666666666667185, 0.6428571428571429047, 0.6440476190476190910, 0.6452380952380952772, 0.6464285714285714635, 0.6476190476190476497, 0.6488095238095238360, 0.6500000000000000222, 0.6511904761904762085, 0.6523809523809523947, 0.6535714285714285809, 0.6547619047619047672, 0.6559523809523809534, 0.6571428571428571397, 0.6583333333333333259, 0.6595238095238095122, 0.6607142857142856984, 0.6619047619047618847, 0.6630952380952380709, 0.6642857142857142572, 0.6654761904761904434, 0.6666666666666666297, 0.6678571428571428159, 0.6690476190476190022, 0.6702380952380951884, 0.6714285714285713746, 0.6726190476190476719, 0.6738095238095238582, 0.6750000000000000444, 0.6761904761904762307, 0.6773809523809524169, 0.6785714285714286031, 0.6797619047619047894, 0.6809523809523809756, 0.6821428571428571619, 0.6833333333333333481, 0.6845238095238095344, 0.6857142857142857206, 0.6869047619047619069, 0.6880952380952380931, 0.6892857142857142794, 0.6904761904761904656, 0.6916666666666666519, 0.6928571428571428381, 0.6940476190476190244, 0.6952380952380952106, 0.6964285714285713969, 0.6976190476190475831, 0.6988095238095237693, 0.6999999999999999556, 0.7011904761904761418, 0.7023809523809523281, 0.7035714285714286254, 0.7047619047619048116, 0.7059523809523809978, 0.7071428571428571841, 0.7083333333333333703, 0.7095238095238095566, 0.7107142857142857428, 0.7119047619047619291, 0.7130952380952381153, 0.7142857142857143016, 0.7154761904761904878, 0.7166666666666666741, 0.7178571428571428603, 0.7190476190476190466, 0.7202380952380952328, 0.7214285714285714191, 0.7226190476190476053, 0.7238095238095237915, 0.7249999999999999778, 0.7261904761904761640, 0.7273809523809523503, 0.7285714285714285365, 0.7297619047619047228, 0.7309523809523809090, 0.7321428571428570953, 0.7333333333333332815, 0.7345238095238095788, 0.7357142857142857650, 0.7369047619047619513, 0.7380952380952381375, 0.7392857142857143238, 0.7404761904761905100, 0.7416666666666666963, 0.7428571428571428825, 0.7440476190476190688, 0.7452380952380952550, 0.7464285714285714413, 0.7476190476190476275, 0.7488095238095238138, 0.7500000000000000000, 0.7511904761904761862, 0.7523809523809523725, 0.7535714285714285587, 0.7547619047619047450, 0.7559523809523809312, 0.7571428571428571175, 0.7583333333333333037, 0.7595238095238094900, 0.7607142857142856762, 0.7619047619047618625, 0.7630952380952380487, 0.7642857142857142350, 0.7654761904761904212, 0.7666666666666667185, 0.7678571428571429047, 0.7690476190476190910, 0.7702380952380952772, 0.7714285714285714635, 0.7726190476190476497, 0.7738095238095238360, 0.7750000000000000222, 0.7761904761904762085, 0.7773809523809523947, 0.7785714285714285809, 0.7797619047619047672, 0.7809523809523809534, 0.7821428571428571397, 0.7833333333333333259, 0.7845238095238095122, 0.7857142857142856984, 0.7869047619047618847, 0.7880952380952380709, 0.7892857142857142572, 0.7904761904761904434, 0.7916666666666666297, 0.7928571428571428159, 0.7940476190476190022, 0.7952380952380951884, 0.7964285714285713746, 0.7976190476190476719, 0.7988095238095238582, 0.8000000000000000444, 0.8011904761904762307, 0.8023809523809524169, 0.8035714285714286031, 0.8047619047619047894, 0.8059523809523809756, 0.8071428571428571619, 0.8083333333333333481, 0.8095238095238095344, 0.8107142857142857206, 0.8119047619047619069, 0.8130952380952380931, 0.8142857142857142794, 0.8154761904761904656, 0.8166666666666666519, 0.8178571428571428381, 0.8190476190476190244, 0.8202380952380952106, 0.8214285714285713969, 0.8226190476190475831, 0.8238095238095237693, 0.8249999999999999556, 0.8261904761904761418, 0.8273809523809523281, 0.8285714285714286254, 0.8297619047619048116, 0.8309523809523809978, 0.8321428571428571841, 0.8333333333333333703, 0.8345238095238095566, 0.8357142857142857428, 0.8369047619047619291, 0.8380952380952381153, 0.8392857142857143016, 0.8404761904761904878, 0.8416666666666666741, 0.8428571428571428603, 0.8440476190476190466, 0.8452380952380952328, 0.8464285714285714191, 0.8476190476190476053, 0.8488095238095237915, 0.8499999999999999778, 0.8511904761904761640, 0.8523809523809523503, 0.8535714285714285365, 0.8547619047619047228, 0.8559523809523809090, 0.8571428571428570953, 0.8583333333333332815, 0.8595238095238095788, 0.8607142857142857650, 0.8619047619047619513, 0.8630952380952381375, 0.8642857142857143238, 0.8654761904761905100, 0.8666666666666666963, 0.8678571428571428825, 0.8690476190476190688, 0.8702380952380952550, 0.8714285714285714413, 0.8726190476190476275, 0.8738095238095238138, 0.8750000000000000000, 0.8761904761904761862, 0.8773809523809523725, 0.8785714285714285587, 0.8797619047619047450, 0.8809523809523809312, 0.8821428571428571175, 0.8833333333333333037, 0.8845238095238094900, 0.8857142857142856762, 0.8869047619047618625, 0.8880952380952380487, 0.8892857142857142350, 0.8904761904761904212, 0.8916666666666667185, 0.8928571428571429047, 0.8940476190476190910, 0.8952380952380952772, 0.8964285714285714635, 0.8976190476190476497, 0.8988095238095238360, 0.9000000000000000222, 0.9011904761904762085, 0.9023809523809523947, 0.9035714285714285809, 0.9047619047619047672, 0.9059523809523809534, 0.9071428571428571397, 0.9083333333333333259, 0.9095238095238095122, 0.9107142857142856984, 0.9119047619047618847, 0.9130952380952380709, 0.9142857142857142572, 0.9154761904761904434, 0.9166666666666666297, 0.9178571428571428159, 0.9190476190476190022, 0.9202380952380951884, 0.9214285714285713746, 0.9226190476190476719, 0.9238095238095238582, 0.9250000000000000444, 0.9261904761904762307, 0.9273809523809524169, 0.9285714285714286031, 0.9297619047619047894, 0.9309523809523809756, 0.9321428571428571619, 0.9333333333333333481, 0.9345238095238095344, 0.9357142857142857206, 0.9369047619047619069, 0.9380952380952380931, 0.9392857142857142794, 0.9404761904761904656, 0.9416666666666666519, 0.9428571428571428381, 0.9440476190476190244, 0.9452380952380952106, 0.9464285714285713969, 0.9476190476190475831, 0.9488095238095237693, 0.9499999999999999556, 0.9511904761904761418, 0.9523809523809523281, 0.9535714285714286254, 0.9547619047619048116, 0.9559523809523809978, 0.9571428571428571841, 0.9583333333333333703, 0.9595238095238095566, 0.9607142857142857428, 0.9619047619047619291, 0.9630952380952381153, 0.9642857142857143016, 0.9654761904761904878, 0.9666666666666666741, 0.9678571428571428603, 0.9690476190476190466, 0.9702380952380952328, 0.9714285714285714191, 0.9726190476190476053, 0.9738095238095237915, 0.9749999999999999778, 0.9761904761904761640, 0.9773809523809523503, 0.9785714285714285365, 0.9797619047619047228, 0.9809523809523809090, 0.9821428571428570953, 0.9833333333333332815, 0.9845238095238095788, 0.9857142857142857650, 0.9869047619047619513, 0.9880952380952381375, 0.9892857142857143238, 0.9904761904761905100, 0.9916666666666666963, 0.9928571428571428825, 0.9940476190476190688, 0.9952380952380952550, 0.9964285714285714413, 0.9976190476190476275, 0.9988095238095238138, 1.000000000000000000 ),
 .UNSPECIFIED. ) 
 CURVE ( )  GEOMETRIC_REPRESENTATION_ITEM ( )  RATIONAL_B_SPLINE_CURVE ( ( 1.000000000000000000, 0.8660254037844387076, 1.000000000000000000, 0.8660254037844387076, 1.000000000000000000, 0.8660254037844387076, 1.000000000000000000, 0.8660254037844387076, 1.000000000000000000, 0.8660254037844387076, 1.000000000000000000, 0.8660254037844387076, 1.000000000000000000, 0.8660254037844387076, 1.000000000000000000, 0.8660254037844387076, 1.000000000000000000, 0.8660254037844387076, 1.000000000000000000, 0.8660254037844387076, 1.000000000000000000, 0.8660254037844387076, 1.000000000000000000, 0.8660254037844387076, 1.000000000000000000, 0.8660254037844387076, 1.000000000000000000, 0.8660254037844387076, 1.000000000000000000, 0.8660254037844387076, 1.000000000000000000, 0.8660254037844387076, 1.000000000000000000, 0.8660254037844387076, 1.000000000000000000, 0.8660254037844387076, 1.000000000000000000, 0.8660254037844387076, 1.000000000000000000, 0.8660254037844387076, 1.000000000000000000, 0.8660254037844387076, 1.000000000000000000, 0.8660254037844387076, 1.000000000000000000, 0.8660254037844387076, 1.000000000000000000, 0.8660254037844387076, 1.000000000000000000, 0.8660254037844387076, 1.000000000000000000, 0.8660254037844387076, 1.000000000000000000, 0.8660254037844387076, 1.000000000000000000, 0.8660254037844387076, 1.000000000000000000, 0.8660254037844387076, 1.000000000000000000, 0.8660254037844387076, 1.000000000000000000, 0.8660254037844387076, 1.000000000000000000, 0.8660254037844387076, 1.000000000000000000, 0.8660254037844387076, 1.000000000000000000, 0.8660254037844387076, 1.000000000000000000, 0.8660254037844387076, 1.000000000000000000, 0.8660254037844387076, 1.000000000000000000, 0.8660254037844387076, 1.000000000000000000, 0.8660254037844387076, 1.000000000000000000, 0.8660254037844387076, 1.000000000000000000, 0.8660254037844387076, 1.000000000000000000, 0.8660254037844387076, 1.000000000000000000, 0.8660254037844387076, 1.000000000000000000, 0.8660254037844387076, 1.000000000000000000, 0.8660254037844387076, 1.000000000000000000, 0.8660254037844387076, 1.000000000000000000, 0.8660254037844387076, 1.000000000000000000, 0.8660254037844387076, 1.000000000000000000, 0.8660254037844387076, 1.000000000000000000, 0.8660254037844387076, 1.000000000000000000, 0.8660254037844387076, 1.000000000000000000, 0.8660254037844387076, 1.000000000000000000, 0.8660254037844387076, 1.000000000000000000, 0.8660254037844387076, 1.000000000000000000, 0.8660254037844387076, 1.000000000000000000, 0.8660254037844387076, 1.000000000000000000, 0.8660254037844387076, 1.000000000000000000, 0.8660254037844387076, 1.000000000000000000, 0.8660254037844387076, 1.000000000000000000, 0.8660254037844387076, 1.000000000000000000, 0.8660254037844387076, 1.000000000000000000, 0.8660254037844387076, 1.000000000000000000, 0.8660254037844387076, 1.000000000000000000, 0.8660254037844387076, 1.000000000000000000, 0.8660254037844387076, 1.000000000000000000, 0.8660254037844387076, 1.000000000000000000, 0.8660254037844387076, 1.000000000000000000, 0.8660254037844387076, 1.000000000000000000, 0.8660254037844387076, 1.000000000000000000, 0.8660254037844387076, 1.000000000000000000, 0.8660254037844387076, 1.000000000000000000, 0.8660254037844387076, 1.000000000000000000, 0.8660254037844387076, 1.000000000000000000, 0.8660254037844387076, 1.000000000000000000, 0.8660254037844387076, 1.000000000000000000, 0.8660254037844387076, 1.000000000000000000, 0.8660254037844387076, 1.000000000000000000, 0.8660254037844387076, 1.000000000000000000, 0.8660254037844387076, 1.000000000000000000, 0.8660254037844387076, 1.000000000000000000, 0.8660254037844387076, 1.000000000000000000, 0.8660254037844387076, 1.000000000000000000, 0.8660254037844387076, 1.000000000000000000, 0.8660254037844387076, 1.000000000000000000, 0.8660254037844387076, 1.000000000000000000, 0.8660254037844387076, 1.000000000000000000, 0.8660254037844387076, 1.000000000000000000, 0.8660254037844387076, 1.000000000000000000, 0.8660254037844387076, 1.000000000000000000, 0.8660254037844387076, 1.000000000000000000, 0.8660254037844387076, 1.000000000000000000, 0.8660254037844387076, 1.000000000000000000, 0.8660254037844387076, 1.000000000000000000, 0.8660254037844387076, 1.000000000000000000, 0.8660254037844387076, 1.000000000000000000, 0.8660254037844387076, 1.000000000000000000, 0.8660254037844387076, 1.000000000000000000, 0.8660254037844387076, 1.000000000000000000, 0.8660254037844387076, 1.000000000000000000, 0.8660254037844387076, 1.000000000000000000, 0.8660254037844387076, 1.000000000000000000, 0.8660254037844387076, 1.000000000000000000, 0.8660254037844387076, 1.000000000000000000, 0.8660254037844387076, 1.000000000000000000, 0.8660254037844387076, 1.000000000000000000, 0.8660254037844387076, 1.000000000000000000, 0.8660254037844387076, 1.000000000000000000, 0.8660254037844387076, 1.000000000000000000, 0.8660254037844387076, 1.000000000000000000, 0.8660254037844387076, 1.000000000000000000, 0.8660254037844387076, 1.000000000000000000, 0.8660254037844387076, 1.000000000000000000, 0.8660254037844387076, 1.000000000000000000, 0.8660254037844387076, 1.000000000000000000, 0.8660254037844387076, 1.000000000000000000, 0.8660254037844387076, 1.000000000000000000, 0.8660254037844387076, 1.000000000000000000, 0.8660254037844387076, 1.000000000000000000, 0.8660254037844387076, 1.000000000000000000, 0.8660254037844387076, 1.000000000000000000, 0.8660254037844387076, 1.000000000000000000, 0.8660254037844387076, 1.000000000000000000, 0.8660254037844387076, 1.000000000000000000, 0.8660254037844387076, 1.000000000000000000, 0.8660254037844387076, 1.000000000000000000, 0.8660254037844387076, 1.000000000000000000, 0.8660254037844387076, 1.000000000000000000, 0.8660254037844387076, 1.000000000000000000, 0.8660254037844387076, 1.000000000000000000, 0.8660254037844387076, 1.000000000000000000, 0.8660254037844387076, 1.000000000000000000, 0.8660254037844387076, 1.000000000000000000, 0.8660254037844387076, 1.000000000000000000, 0.8660254037844387076, 1.000000000000000000, 0.8660254037844387076, 1.000000000000000000, 0.8660254037844387076, 1.000000000000000000, 0.8660254037844387076, 1.000000000000000000, 0.8660254037844387076, 1.000000000000000000, 0.8660254037844387076, 1.000000000000000000, 0.8660254037844387076, 1.000000000000000000, 0.8660254037844387076, 1.000000000000000000, 0.8660254037844387076, 1.000000000000000000, 0.8660254037844387076, 1.000000000000000000, 0.8660254037844387076, 1.000000000000000000, 0.8660254037844387076, 1.000000000000000000, 0.8660254037844387076, 1.000000000000000000, 0.8660254037844387076, 1.000000000000000000, 0.8660254037844387076, 1.000000000000000000, 0.8660254037844387076, 1.000000000000000000, 0.8660254037844387076, 1.000000000000000000, 0.8660254037844387076, 1.000000000000000000, 0.8660254037844387076, 1.000000000000000000, 0.8660254037844387076, 1.000000000000000000, 0.8660254037844387076, 1.000000000000000000, 0.8660254037844387076, 1.000000000000000000, 0.8660254037844387076, 1.000000000000000000, 0.8660254037844387076, 1.000000000000000000, 0.8660254037844387076, 1.000000000000000000, 0.8660254037844387076, 1.000000000000000000, 0.8660254037844387076, 1.000000000000000000, 0.8660254037844387076, 1.000000000000000000, 0.8660254037844387076, 1.000000000000000000, 0.8660254037844387076, 1.000000000000000000, 0.8660254037844387076, 1.000000000000000000, 0.8660254037844387076, 1.000000000000000000, 0.8660254037844387076, 1.000000000000000000, 0.8660254037844387076, 1.000000000000000000, 0.8660254037844387076, 1.000000000000000000, 0.8660254037844387076, 1.000000000000000000, 0.8660254037844387076, 1.000000000000000000, 0.8660254037844387076, 1.000000000000000000, 0.8660254037844387076, 1.000000000000000000, 0.8660254037844387076, 1.000000000000000000, 0.8660254037844387076, 1.000000000000000000, 0.8660254037844387076, 1.000000000000000000, 0.8660254037844387076, 1.000000000000000000, 0.8660254037844387076, 1.000000000000000000, 0.8660254037844387076, 1.000000000000000000, 0.8660254037844387076, 1.000000000000000000, 0.8660254037844387076, 1.000000000000000000, 0.8660254037844387076, 1.000000000000000000, 0.8660254037844387076, 1.000000000000000000, 0.8660254037844387076, 1.000000000000000000, 0.8660254037844387076, 1.000000000000000000, 0.8660254037844387076, 1.000000000000000000, 0.8660254037844387076, 1.000000000000000000, 0.8660254037844387076, 1.000000000000000000, 0.8660254037844387076, 1.000000000000000000, 0.8660254037844387076, 1.000000000000000000, 0.8660254037844387076, 1.000000000000000000, 0.8660254037844387076, 1.000000000000000000, 0.8660254037844387076, 1.000000000000000000, 0.8660254037844387076, 1.000000000000000000, 0.8660254037844387076, 1.000000000000000000, 0.8660254037844387076, 1.000000000000000000, 0.8660254037844387076, 1.000000000000000000, 0.8660254037844387076, 1.000000000000000000, 0.8660254037844387076, 1.000000000000000000, 0.8660254037844387076, 1.000000000000000000, 0.8660254037844387076, 1.000000000000000000, 0.8660254037844387076, 1.000000000000000000, 0.8660254037844387076, 1.000000000000000000, 0.8660254037844387076, 1.000000000000000000, 0.8660254037844387076, 1.000000000000000000, 0.8660254037844387076, 1.000000000000000000, 0.8660254037844387076, 1.000000000000000000, 0.8660254037844387076, 1.000000000000000000, 0.8660254037844387076, 1.000000000000000000, 0.8660254037844387076, 1.000000000000000000, 0.8660254037844387076, 1.000000000000000000, 0.8660254037844387076, 1.000000000000000000, 0.8660254037844387076, 1.000000000000000000, 0.8660254037844387076, 1.000000000000000000, 0.8660254037844387076, 1.000000000000000000, 0.8660254037844387076, 1.000000000000000000, 0.8660254037844387076, 1.000000000000000000, 0.8660254037844387076, 1.000000000000000000, 0.8660254037844387076, 1.000000000000000000, 0.8660254037844387076, 1.000000000000000000, 0.8660254037844387076, 1.000000000000000000, 0.8660254037844387076, 1.000000000000000000, 0.8660254037844387076, 1.000000000000000000, 0.8660254037844387076, 1.000000000000000000, 0.8660254037844387076, 1.000000000000000000, 0.8660254037844387076, 1.000000000000000000, 0.8660254037844387076, 1.000000000000000000, 0.8660254037844387076, 1.000000000000000000, 0.8660254037844387076, 1.000000000000000000, 0.8660254037844387076, 1.000000000000000000, 0.8660254037844387076, 1.000000000000000000, 0.8660254037844387076, 1.000000000000000000, 0.8660254037844387076, 1.000000000000000000, 0.8660254037844387076, 1.000000000000000000, 0.8660254037844387076, 1.000000000000000000, 0.8660254037844387076, 1.000000000000000000, 0.8660254037844387076, 1.000000000000000000, 0.8660254037844387076, 1.000000000000000000, 0.8660254037844387076, 1.000000000000000000, 0.8660254037844387076, 1.000000000000000000, 0.8660254037844387076, 1.000000000000000000, 0.8660254037844387076, 1.000000000000000000, 0.8660254037844387076, 1.000000000000000000, 0.8660254037844387076, 1.000000000000000000, 0.8660254037844387076, 1.000000000000000000, 0.8660254037844387076, 1.000000000000000000, 0.8660254037844387076, 1.000000000000000000, 0.8660254037844387076, 1.000000000000000000, 0.8660254037844387076, 1.000000000000000000, 0.8660254037844387076, 1.000000000000000000, 0.8660254037844387076, 1.000000000000000000, 0.8660254037844387076, 1.000000000000000000, 0.8660254037844387076, 1.000000000000000000, 0.8660254037844387076, 1.000000000000000000, 0.8660254037844387076, 1.000000000000000000, 0.8660254037844387076, 1.000000000000000000, 0.8660254037844387076, 1.000000000000000000, 0.8660254037844387076, 1.000000000000000000, 0.8660254037844387076, 1.000000000000000000, 0.8660254037844387076, 1.000000000000000000, 0.8660254037844387076, 1.000000000000000000, 0.8660254037844387076, 1.000000000000000000, 0.8660254037844387076, 1.000000000000000000, 0.8660254037844387076, 1.000000000000000000, 0.8660254037844387076, 1.000000000000000000, 0.8660254037844387076, 1.000000000000000000, 0.8660254037844387076, 1.000000000000000000, 0.8660254037844387076, 1.000000000000000000, 0.8660254037844387076, 1.000000000000000000, 0.8660254037844387076, 1.000000000000000000, 0.8660254037844387076, 1.000000000000000000, 0.8660254037844387076, 1.000000000000000000, 0.8660254037844387076, 1.000000000000000000, 0.8660254037844387076, 1.000000000000000000, 0.8660254037844387076, 1.000000000000000000, 0.8660254037844387076, 1.000000000000000000, 0.8660254037844387076, 1.000000000000000000, 0.8660254037844387076, 1.000000000000000000, 0.8660254037844387076, 1.000000000000000000, 0.8660254037844387076, 1.000000000000000000, 0.8660254037844387076, 1.000000000000000000, 0.8660254037844387076, 1.000000000000000000, 0.8660254037844387076, 1.000000000000000000, 0.8660254037844387076, 1.000000000000000000, 0.8660254037844387076, 1.000000000000000000, 0.8660254037844387076, 1.000000000000000000, 0.8660254037844387076, 1.000000000000000000, 0.8660254037844387076, 1.000000000000000000, 0.8660254037844387076, 1.000000000000000000, 0.8660254037844387076, 1.000000000000000000, 0.8660254037844387076, 1.000000000000000000, 0.8660254037844387076, 1.000000000000000000, 0.8660254037844387076, 1.000000000000000000, 0.8660254037844387076, 1.000000000000000000, 0.8660254037844387076, 1.000000000000000000, 0.8660254037844387076, 1.000000000000000000, 0.8660254037844387076, 1.000000000000000000, 0.8660254037844387076, 1.000000000000000000, 0.8660254037844387076, 1.000000000000000000, 0.8660254037844387076, 1.000000000000000000, 0.8660254037844387076, 1.000000000000000000, 0.8660254037844387076, 1.000000000000000000, 0.8660254037844387076, 1.000000000000000000, 0.8660254037844387076, 1.000000000000000000, 0.8660254037844387076, 1.000000000000000000, 0.8660254037844387076, 1.000000000000000000, 0.8660254037844387076, 1.000000000000000000, 0.8660254037844387076, 1.000000000000000000, 0.8660254037844387076, 1.000000000000000000, 0.8660254037844387076, 1.000000000000000000, 0.8660254037844387076, 1.000000000000000000, 0.8660254037844387076, 1.000000000000000000, 0.8660254037844387076, 1.000000000000000000, 0.8660254037844387076, 1.000000000000000000, 0.8660254037844387076, 1.000000000000000000, 0.8660254037844387076, 1.000000000000000000, 0.8660254037844387076, 1.000000000000000000, 0.8660254037844387076, 1.000000000000000000, 0.8660254037844387076, 1.000000000000000000, 0.8660254037844387076, 1.000000000000000000, 0.8660254037844387076, 1.000000000000000000, 0.8660254037844387076, 1.000000000000000000, 0.8660254037844387076, 1.000000000000000000, 0.8660254037844387076, 1.000000000000000000, 0.8660254037844387076, 1.000000000000000000, 0.8660254037844387076, 1.000000000000000000, 0.8660254037844387076, 1.000000000000000000, 0.8660254037844387076, 1.000000000000000000, 0.8660254037844387076, 1.000000000000000000, 0.8660254037844387076, 1.000000000000000000, 0.8660254037844387076, 1.000000000000000000, 0.8660254037844387076, 1.000000000000000000, 0.8660254037844387076, 1.000000000000000000, 0.8660254037844387076, 1.000000000000000000, 0.8660254037844387076, 1.000000000000000000, 0.8660254037844387076, 1.000000000000000000, 0.8660254037844387076, 1.000000000000000000, 0.8660254037844387076, 1.000000000000000000, 0.8660254037844387076, 1.000000000000000000, 0.8660254037844387076, 1.000000000000000000, 0.8660254037844387076, 1.000000000000000000, 0.8660254037844387076, 1.000000000000000000, 0.8660254037844387076, 1.000000000000000000, 0.8660254037844387076, 1.000000000000000000, 0.8660254037844387076, 1.000000000000000000, 0.8660254037844387076, 1.000000000000000000, 0.8660254037844387076, 1.000000000000000000, 0.8660254037844387076, 1.000000000000000000, 0.8660254037844387076, 1.000000000000000000, 0.8660254037844387076, 1.000000000000000000, 0.8660254037844387076, 1.000000000000000000, 0.8660254037844387076, 1.000000000000000000, 0.8660254037844387076, 1.000000000000000000, 0.8660254037844387076, 1.000000000000000000, 0.8660254037844387076, 1.000000000000000000, 0.8660254037844387076, 1.000000000000000000, 0.8660254037844387076, 1.000000000000000000, 0.8660254037844387076, 1.000000000000000000, 0.8660254037844387076, 1.000000000000000000, 0.8660254037844387076, 1.000000000000000000, 0.8660254037844387076, 1.000000000000000000, 0.8660254037844387076, 1.000000000000000000, 0.8660254037844387076, 1.000000000000000000, 0.8660254037844387076, 1.000000000000000000, 0.8660254037844387076, 1.000000000000000000, 0.8660254037844387076, 1.000000000000000000, 0.8660254037844387076, 1.000000000000000000, 0.8660254037844387076, 1.000000000000000000, 0.8660254037844387076, 1.000000000000000000, 0.8660254037844387076, 1.000000000000000000, 0.8660254037844387076, 1.000000000000000000, 0.8660254037844387076, 1.000000000000000000, 0.8660254037844387076, 1.000000000000000000, 0.8660254037844387076, 1.000000000000000000, 0.8660254037844387076, 1.000000000000000000, 0.8660254037844387076, 1.000000000000000000, 0.8660254037844387076, 1.000000000000000000, 0.8660254037844387076, 1.000000000000000000, 0.8660254037844387076, 1.000000000000000000, 0.8660254037844387076, 1.000000000000000000, 0.8660254037844387076, 1.000000000000000000, 0.8660254037844387076, 1.000000000000000000, 0.8660254037844387076, 1.000000000000000000, 0.8660254037844387076, 1.000000000000000000, 0.8660254037844387076, 1.000000000000000000, 0.8660254037844387076, 1.000000000000000000, 0.8660254037844387076, 1.000000000000000000, 0.8660254037844387076, 1.000000000000000000, 0.8660254037844387076, 1.000000000000000000, 0.8660254037844387076, 1.000000000000000000, 0.8660254037844387076, 1.000000000000000000, 0.8660254037844387076, 1.000000000000000000, 0.8660254037844387076, 1.000000000000000000, 0.8660254037844387076, 1.000000000000000000, 0.8660254037844387076, 1.000000000000000000, 0.8660254037844387076, 1.000000000000000000, 0.8660254037844387076, 1.000000000000000000, 0.8660254037844387076, 1.000000000000000000, 0.8660254037844387076, 1.000000000000000000, 0.8660254037844387076, 1.000000000000000000, 0.8660254037844387076, 1.000000000000000000, 0.8660254037844387076, 1.000000000000000000, 0.8660254037844387076, 1.000000000000000000, 0.8660254037844387076, 1.000000000000000000, 0.8660254037844387076, 1.000000000000000000, 0.8660254037844387076, 1.000000000000000000, 0.8660254037844387076, 1.000000000000000000, 0.8660254037844387076, 1.000000000000000000, 0.8660254037844387076, 1.000000000000000000, 0.8660254037844387076, 1.000000000000000000, 0.8660254037844387076, 1.000000000000000000, 0.8660254037844387076, 1.000000000000000000, 0.8660254037844387076, 1.000000000000000000, 0.8660254037844387076, 1.000000000000000000, 0.8660254037844387076, 1.000000000000000000, 0.8660254037844387076, 1.000000000000000000, 0.8660254037844387076, 1.000000000000000000, 0.8660254037844387076, 1.000000000000000000, 0.8660254037844387076, 1.000000000000000000, 0.8660254037844387076, 1.000000000000000000, 0.8660254037844387076, 1.000000000000000000, 0.8660254037844387076, 1.000000000000000000, 0.8660254037844387076, 1.000000000000000000, 0.8660254037844387076, 1.000000000000000000, 0.8660254037844387076, 1.000000000000000000, 0.8660254037844387076, 1.000000000000000000, 0.8660254037844387076, 1.000000000000000000, 0.8660254037844387076, 1.000000000000000000, 0.8660254037844387076, 1.000000000000000000, 0.8660254037844387076, 1.000000000000000000, 0.8660254037844387076, 1.000000000000000000, 0.8660254037844387076, 1.000000000000000000, 0.8660254037844387076, 1.000000000000000000, 0.8660254037844387076, 1.000000000000000000, 0.8660254037844387076, 1.000000000000000000, 0.8660254037844387076, 1.000000000000000000, 0.8660254037844387076, 1.000000000000000000, 0.8660254037844387076, 1.000000000000000000, 0.8660254037844387076, 1.000000000000000000, 0.8660254037844387076, 1.000000000000000000, 0.8660254037844387076, 1.000000000000000000, 0.8660254037844387076, 1.000000000000000000, 0.8660254037844387076, 1.000000000000000000, 0.8660254037844387076, 1.000000000000000000, 0.8660254037844387076, 1.000000000000000000, 0.8660254037844387076, 1.000000000000000000, 0.8660254037844387076, 1.000000000000000000, 0.8660254037844387076, 1.000000000000000000, 0.8660254037844387076, 1.000000000000000000, 0.8660254037844387076, 1.000000000000000000, 0.8660254037844387076, 1.000000000000000000, 0.8660254037844387076, 1.000000000000000000, 0.8660254037844387076, 1.000000000000000000, 0.8660254037844387076, 1.000000000000000000, 0.8660254037844387076, 1.000000000000000000, 0.8660254037844387076, 1.000000000000000000, 0.8660254037844387076, 1.000000000000000000, 0.8660254037844387076, 1.000000000000000000, 0.8660254037844387076, 1.000000000000000000, 0.8660254037844387076, 1.000000000000000000, 0.8660254037844387076, 1.000000000000000000, 0.8660254037844387076, 1.000000000000000000, 0.8660254037844387076, 1.000000000000000000, 0.8660254037844387076, 1.000000000000000000, 0.8660254037844387076, 1.000000000000000000, 0.8660254037844387076, 1.000000000000000000, 0.8660254037844387076, 1.000000000000000000, 0.8660254037844387076, 1.000000000000000000, 0.8660254037844387076, 1.000000000000000000, 0.8660254037844387076, 1.000000000000000000, 0.8660254037844387076, 1.000000000000000000, 0.8660254037844387076, 1.000000000000000000, 0.8660254037844387076, 1.000000000000000000, 0.8660254037844387076, 1.000000000000000000, 0.8660254037844387076, 1.000000000000000000, 0.8660254037844387076, 1.000000000000000000, 0.8660254037844387076, 1.000000000000000000, 0.8660254037844387076, 1.000000000000000000, 0.8660254037844387076, 1.000000000000000000, 0.8660254037844387076, 1.000000000000000000, 0.8660254037844387076, 1.000000000000000000, 0.8660254037844387076, 1.000000000000000000, 0.8660254037844387076, 1.000000000000000000, 0.8660254037844387076, 1.000000000000000000, 0.8660254037844387076, 1.000000000000000000, 0.8660254037844387076, 1.000000000000000000, 0.8660254037844387076, 1.000000000000000000, 0.8660254037844387076, 1.000000000000000000, 0.8660254037844387076, 1.000000000000000000, 0.8660254037844387076, 1.000000000000000000, 0.8660254037844387076, 1.000000000000000000, 0.8660254037844387076, 1.000000000000000000, 0.8660254037844387076, 1.000000000000000000, 0.8660254037844387076, 1.000000000000000000, 0.8660254037844387076, 1.000000000000000000, 0.8660254037844387076, 1.000000000000000000, 0.8660254037844387076, 1.000000000000000000, 0.8660254037844387076, 1.000000000000000000, 0.8660254037844387076, 1.000000000000000000, 0.8660254037844387076, 1.000000000000000000, 0.8660254037844387076, 1.000000000000000000, 0.8660254037844387076, 1.000000000000000000, 0.8660254037844387076, 1.000000000000000000, 0.8660254037844387076, 1.000000000000000000, 0.8660254037844387076, 1.000000000000000000, 0.8660254037844387076, 1.000000000000000000, 0.8660254037844387076, 1.000000000000000000, 0.8660254037844387076, 1.000000000000000000, 0.8660254037844387076, 1.000000000000000000, 0.8660254037844387076, 1.000000000000000000, 0.8660254037844387076, 1.000000000000000000, 0.8660254037844387076, 1.000000000000000000, 0.8660254037844387076, 1.000000000000000000, 0.8660254037844387076, 1.000000000000000000, 0.8660254037844387076, 1.000000000000000000, 0.8660254037844387076, 1.000000000000000000, 0.8660254037844387076, 1.000000000000000000, 0.8660254037844387076, 1.000000000000000000, 0.8660254037844387076, 1.000000000000000000, 0.8660254037844387076, 1.000000000000000000, 0.8660254037844387076, 1.000000000000000000, 0.8660254037844387076, 1.000000000000000000, 0.8660254037844387076, 1.000000000000000000, 0.8660254037844387076, 1.000000000000000000, 0.8660254037844387076, 1.000000000000000000, 0.8660254037844387076, 1.000000000000000000, 0.8660254037844387076, 1.000000000000000000, 0.8660254037844387076, 1.000000000000000000, 0.8660254037844387076, 1.000000000000000000, 0.8660254037844387076, 1.000000000000000000, 0.8660254037844387076, 1.000000000000000000, 0.8660254037844387076, 1.000000000000000000, 0.8660254037844387076, 1.000000000000000000, 0.8660254037844387076, 1.000000000000000000, 0.8660254037844387076, 1.000000000000000000, 0.8660254037844387076, 1.000000000000000000, 0.8660254037844387076, 1.000000000000000000, 0.8660254037844387076, 1.000000000000000000, 0.8660254037844387076, 1.000000000000000000, 0.8660254037844387076, 1.000000000000000000, 0.8660254037844387076, 1.000000000000000000, 0.8660254037844387076, 1.000000000000000000, 0.8660254037844387076, 1.000000000000000000, 0.8660254037844387076, 1.000000000000000000, 0.8660254037844387076, 1.000000000000000000, 0.8660254037844387076, 1.000000000000000000, 0.8660254037844387076, 1.000000000000000000, 0.8660254037844387076, 1.000000000000000000, 0.8660254037844387076, 1.000000000000000000, 0.8660254037844387076, 1.000000000000000000, 0.8660254037844387076, 1.000000000000000000, 0.8660254037844387076, 1.000000000000000000, 0.8660254037844387076, 1.000000000000000000, 0.8660254037844387076, 1.000000000000000000, 0.8660254037844387076, 1.000000000000000000, 0.8660254037844387076, 1.000000000000000000, 0.8660254037844387076, 1.000000000000000000, 0.8660254037844387076, 1.000000000000000000, 0.8660254037844387076, 1.000000000000000000, 0.8660254037844387076, 1.000000000000000000, 0.8660254037844387076, 1.000000000000000000, 0.8660254037844387076, 1.000000000000000000, 0.8660254037844387076, 1.000000000000000000, 0.8660254037844387076, 1.000000000000000000, 0.8660254037844387076, 1.000000000000000000, 0.8660254037844387076, 1.000000000000000000, 0.8660254037844387076, 1.000000000000000000, 0.8660254037844387076, 1.000000000000000000, 0.8660254037844387076, 1.000000000000000000, 0.8660254037844387076, 1.000000000000000000, 0.8660254037844387076, 1.000000000000000000, 0.8660254037844387076, 1.000000000000000000, 0.8660254037844387076, 1.000000000000000000, 0.8660254037844387076, 1.000000000000000000, 0.8660254037844387076, 1.000000000000000000, 0.8660254037844387076, 1.000000000000000000, 0.8660254037844387076, 1.000000000000000000, 0.8660254037844387076, 1.000000000000000000, 0.8660254037844387076, 1.000000000000000000, 0.8660254037844387076, 1.000000000000000000, 0.8660254037844387076, 1.000000000000000000, 0.8660254037844387076, 1.000000000000000000, 0.8660254037844387076, 1.000000000000000000, 0.8660254037844387076, 1.000000000000000000, 0.8660254037844387076, 1.000000000000000000, 0.8660254037844387076, 1.000000000000000000, 0.8660254037844387076, 1.000000000000000000, 0.8660254037844387076, 1.000000000000000000, 0.8660254037844387076, 1.000000000000000000, 0.8660254037844387076, 1.000000000000000000, 0.8660254037844387076, 1.000000000000000000, 0.8660254037844387076, 1.000000000000000000, 0.8660254037844387076, 1.000000000000000000, 0.8660254037844387076, 1.000000000000000000, 0.8660254037844387076, 1.000000000000000000, 0.8660254037844387076, 1.000000000000000000, 0.8660254037844387076, 1.000000000000000000, 0.8660254037844387076, 1.000000000000000000, 0.8660254037844387076, 1.000000000000000000, 0.8660254037844387076, 1.000000000000000000, 0.8660254037844387076, 1.000000000000000000, 0.8660254037844387076, 1.000000000000000000, 0.8660254037844387076, 1.000000000000000000, 0.8660254037844387076, 1.000000000000000000, 0.8660254037844387076, 1.000000000000000000, 0.8660254037844387076, 1.000000000000000000, 0.8660254037844387076, 1.000000000000000000, 0.8660254037844387076, 1.000000000000000000, 0.8660254037844387076, 1.000000000000000000, 0.8660254037844387076, 1.000000000000000000, 0.8660254037844387076, 1.000000000000000000, 0.8660254037844387076, 1.000000000000000000, 0.8660254037844387076, 1.000000000000000000, 0.8660254037844387076, 1.000000000000000000, 0.8660254037844387076, 1.000000000000000000, 0.8660254037844387076, 1.000000000000000000, 0.8660254037844387076, 1.000000000000000000, 0.8660254037844387076, 1.000000000000000000, 0.8660254037844387076, 1.000000000000000000, 0.8660254037844387076, 1.000000000000000000, 0.8660254037844387076, 1.000000000000000000, 0.8660254037844387076, 1.000000000000000000, 0.8660254037844387076, 1.000000000000000000, 0.8660254037844387076, 1.000000000000000000, 0.8660254037844387076, 1.000000000000000000, 0.8660254037844387076, 1.000000000000000000, 0.8660254037844387076, 1.000000000000000000, 0.8660254037844387076, 1.000000000000000000, 0.8660254037844387076, 1.000000000000000000, 0.8660254037844387076, 1.000000000000000000, 0.8660254037844387076, 1.000000000000000000, 0.8660254037844387076, 1.000000000000000000, 0.8660254037844387076, 1.000000000000000000, 0.8660254037844387076, 1.000000000000000000, 0.8660254037844387076, 1.000000000000000000, 0.8660254037844387076, 1.000000000000000000, 0.8660254037844387076, 1.000000000000000000, 0.8660254037844387076, 1.000000000000000000, 0.8660254037844387076, 1.000000000000000000, 0.8660254037844387076, 1.000000000000000000, 0.8660254037844387076, 1.000000000000000000, 0.8660254037844387076, 1.000000000000000000, 0.8660254037844387076, 1.000000000000000000, 0.8660254037844387076, 1.000000000000000000, 0.8660254037844387076, 1.000000000000000000, 0.8660254037844387076, 1.000000000000000000, 0.8660254037844387076, 1.000000000000000000, 0.8660254037844387076, 1.000000000000000000, 0.8660254037844387076, 1.000000000000000000, 0.8660254037844387076, 1.000000000000000000, 0.8660254037844387076, 1.000000000000000000, 0.8660254037844387076, 1.000000000000000000, 0.8660254037844387076, 1.000000000000000000, 0.8660254037844387076, 1.000000000000000000, 0.8660254037844387076, 1.000000000000000000, 0.8660254037844387076, 1.000000000000000000, 0.8660254037844387076, 1.000000000000000000, 0.8660254037844387076, 1.000000000000000000, 0.8660254037844387076, 1.000000000000000000, 0.8660254037844387076, 1.000000000000000000, 0.8660254037844387076, 1.000000000000000000, 0.8660254037844387076, 1.000000000000000000, 0.8660254037844387076, 1.000000000000000000, 0.8660254037844387076, 1.000000000000000000, 0.8660254037844387076, 1.000000000000000000, 0.8660254037844387076, 1.000000000000000000, 0.8660254037844387076, 1.000000000000000000, 0.8660254037844387076, 1.000000000000000000, 0.8660254037844387076, 1.000000000000000000, 0.8660254037844387076, 1.000000000000000000, 0.8660254037844387076, 1.000000000000000000, 0.8660254037844387076, 1.000000000000000000, 0.8660254037844387076, 1.000000000000000000, 0.8660254037844387076, 1.000000000000000000, 0.8660254037844387076, 1.000000000000000000, 0.8660254037844387076, 1.000000000000000000, 0.8660254037844387076, 1.000000000000000000, 0.8660254037844387076, 1.000000000000000000, 0.8660254037844387076, 1.000000000000000000, 0.8660254037844387076, 1.000000000000000000, 0.8660254037844387076, 1.000000000000000000, 0.8660254037844387076, 1.000000000000000000, 0.8660254037844387076, 1.000000000000000000, 0.8660254037844387076, 1.000000000000000000, 0.8660254037844387076, 1.000000000000000000, 0.8660254037844387076, 1.000000000000000000, 0.8660254037844387076, 1.000000000000000000, 0.8660254037844387076, 1.000000000000000000, 0.8660254037844387076, 1.000000000000000000, 0.8660254037844387076, 1.000000000000000000, 0.8660254037844387076, 1.000000000000000000, 0.8660254037844387076, 1.000000000000000000, 0.8660254037844387076, 1.000000000000000000, 0.8660254037844387076, 1.000000000000000000, 0.8660254037844387076, 1.000000000000000000, 0.8660254037844387076, 1.000000000000000000, 0.8660254037844387076, 1.000000000000000000, 0.8660254037844387076, 1.000000000000000000, 0.8660254037844387076, 1.000000000000000000, 0.8660254037844387076, 1.000000000000000000, 0.8660254037844387076, 1.000000000000000000, 0.8660254037844387076, 1.000000000000000000, 0.8660254037844387076, 1.000000000000000000, 0.8660254037844387076, 1.000000000000000000, 0.8660254037844387076, 1.000000000000000000, 0.8660254037844387076, 1.000000000000000000, 0.8660254037844387076, 1.000000000000000000, 0.8660254037844387076, 1.000000000000000000, 0.8660254037844387076, 1.000000000000000000, 0.8660254037844387076, 1.000000000000000000, 0.8660254037844387076, 1.000000000000000000, 0.8660254037844387076, 1.000000000000000000, 0.8660254037844387076, 1.000000000000000000, 0.8660254037844387076, 1.000000000000000000, 0.8660254037844387076, 1.000000000000000000, 0.8660254037844387076, 1.000000000000000000, 0.8660254037844387076, 1.000000000000000000, 0.8660254037844387076, 1.000000000000000000, 0.8660254037844387076, 1.000000000000000000, 0.8660254037844387076, 1.000000000000000000, 0.8660254037844387076, 1.000000000000000000, 0.8660254037844387076, 1.000000000000000000, 0.8660254037844387076, 1.000000000000000000, 0.8660254037844387076, 1.000000000000000000, 0.8660254037844387076, 1.000000000000000000, 0.8660254037844387076, 1.000000000000000000, 0.8660254037844387076, 1.000000000000000000, 0.8660254037844387076, 1.000000000000000000, 0.8660254037844387076, 1.000000000000000000, 0.8660254037844387076, 1.000000000000000000, 0.8660254037844387076, 1.000000000000000000, 0.8660254037844387076, 1.000000000000000000, 0.8660254037844387076, 1.000000000000000000, 0.8660254037844387076, 1.000000000000000000, 0.8660254037844387076, 1.000000000000000000, 0.8660254037844387076, 1.000000000000000000, 0.8660254037844387076, 1.000000000000000000, 0.8660254037844387076, 1.000000000000000000, 0.8660254037844387076, 1.000000000000000000, 0.8660254037844387076, 1.000000000000000000, 0.8660254037844387076, 1.000000000000000000, 0.8660254037844387076, 1.000000000000000000, 0.8660254037844387076, 1.000000000000000000, 0.8660254037844387076, 1.000000000000000000, 0.8660254037844387076, 1.000000000000000000, 0.8660254037844387076, 1.000000000000000000, 0.8660254037844387076, 1.000000000000000000, 0.8660254037844387076, 1.000000000000000000, 0.8660254037844387076, 1.000000000000000000, 0.8660254037844387076, 1.000000000000000000, 0.8660254037844387076, 1.000000000000000000, 0.8660254037844387076, 1.000000000000000000, 0.8660254037844387076, 1.000000000000000000, 0.8660254037844387076, 1.000000000000000000, 0.8660254037844387076, 1.000000000000000000, 0.8660254037844387076, 1.000000000000000000, 0.8660254037844387076, 1.000000000000000000, 0.8660254037844387076, 1.000000000000000000, 0.8660254037844387076, 1.000000000000000000, 0.8660254037844387076, 1.000000000000000000, 0.8660254037844387076, 1.000000000000000000, 0.8660254037844387076, 1.000000000000000000, 0.8660254037844387076, 1.000000000000000000, 0.8660254037844387076, 1.000000000000000000, 0.8660254037844387076, 1.000000000000000000, 0.8660254037844387076, 1.000000000000000000, 0.8660254037844387076, 1.000000000000000000, 0.8660254037844387076, 1.000000000000000000, 0.8660254037844387076, 1.000000000000000000, 0.8660254037844387076, 1.000000000000000000, 0.8660254037844387076, 1.000000000000000000, 0.8660254037844387076, 1.000000000000000000, 0.8660254037844387076, 1.000000000000000000, 0.8660254037844387076, 1.000000000000000000, 0.8660254037844387076, 1.000000000000000000, 0.8660254037844387076, 1.000000000000000000, 0.8660254037844387076, 1.000000000000000000, 0.8660254037844387076, 1.000000000000000000, 0.8660254037844387076, 1.000000000000000000, 0.8660254037844387076, 1.000000000000000000, 0.8660254037844387076, 1.000000000000000000, 0.8660254037844387076, 1.000000000000000000, 0.8660254037844387076, 1.000000000000000000, 0.8660254037844387076, 1.000000000000000000, 0.8660254037844387076, 1.000000000000000000, 0.8660254037844387076, 1.000000000000000000, 0.8660254037844387076, 1.000000000000000000, 0.8660254037844387076, 1.000000000000000000, 0.8660254037844387076, 1.000000000000000000, 0.8660254037844387076, 1.000000000000000000, 0.8660254037844387076, 1.000000000000000000, 0.8660254037844387076, 1.000000000000000000, 0.8660254037844387076, 1.000000000000000000, 0.8660254037844387076, 1.000000000000000000, 0.8660254037844387076, 1.000000000000000000, 0.8660254037844387076, 1.000000000000000000, 0.8660254037844387076, 1.000000000000000000, 0.8660254037844387076, 1.000000000000000000, 0.8660254037844387076, 1.000000000000000000, 0.8660254037844387076, 1.000000000000000000, 0.8660254037844387076, 1.000000000000000000, 0.8660254037844387076, 1.000000000000000000, 0.8660254037844387076, 1.000000000000000000, 0.8660254037844387076, 1.000000000000000000, 0.8660254037844387076, 1.000000000000000000, 0.8660254037844387076, 1.000000000000000000, 0.8660254037844387076, 1.000000000000000000, 0.8660254037844387076, 1.000000000000000000, 0.8660254037844387076, 1.000000000000000000, 0.8660254037844387076, 1.000000000000000000, 0.8660254037844387076, 1.000000000000000000, 0.8660254037844387076, 1.000000000000000000, 0.8660254037844387076, 1.000000000000000000, 0.8660254037844387076, 1.000000000000000000, 0.8660254037844387076, 1.000000000000000000, 0.8660254037844387076, 1.000000000000000000, 0.8660254037844387076, 1.000000000000000000, 0.8660254037844387076, 1.000000000000000000, 0.8660254037844387076, 1.000000000000000000, 0.8660254037844387076, 1.000000000000000000, 0.8660254037844387076, 1.000000000000000000, 0.8660254037844387076, 1.000000000000000000, 0.8660254037844387076, 1.000000000000000000, 0.8660254037844387076, 1.000000000000000000, 0.8660254037844387076, 1.000000000000000000, 0.8660254037844387076, 1.000000000000000000, 0.8660254037844387076, 1.000000000000000000, 0.8660254037844387076, 1.000000000000000000, 0.8660254037844387076, 1.000000000000000000, 0.8660254037844387076, 1.000000000000000000, 0.8660254037844387076, 1.000000000000000000, 0.8660254037844387076, 1.000000000000000000, 0.8660254037844387076, 1.000000000000000000, 0.8660254037844387076, 1.000000000000000000, 0.8660254037844387076, 1.000000000000000000, 0.8660254037844387076, 1.000000000000000000, 0.8660254037844387076, 1.000000000000000000, 0.8660254037844387076, 1.000000000000000000, 0.8660254037844387076, 1.000000000000000000, 0.8660254037844387076, 1.000000000000000000, 0.8660254037844387076, 1.000000000000000000, 0.8660254037844387076, 1.000000000000000000 ) ) 
 REPRESENTATION_ITEM ( '' )  );
#48332=VECTOR ( 'NONE', #7821, 1000.000000000000000 ) ;
#48334=CARTESIAN_POINT ( 'NONE',  ( 4.458734125000001214, 2.854166668032259491, 2.574251347313718519 ) ) ;
#48336=DIRECTION ( 'NONE',  ( 0.000000000000000000, 0.000000000000000000, 1.000000000000000000 ) ) ;
#48339=CARTESIAN_POINT ( 'NONE',  ( 2.499999999999998668, 16.66666666666666785, -4.330127018922193649 ) ) ;
#48342=ORIENTED_EDGE ( 'NONE', *, *, #41668, .F. ) ;
#48343=CARTESIAN_POINT ( 'NONE',  ( 2.229367062500001939, -75.97916666530106511, 3.861377020970579999 ) ) ;
#48345=CARTESIAN_POINT ( 'NONE',  ( -2.229367062499996610, 8.854166668032261711, 3.861377020970582219 ) ) ;
#48350=CARTESIAN_POINT ( 'NONE',  ( -3.152548672688508926E-16, -66.81249999863442213, -5.148502694627439702 ) ) ;
#48351=CARTESIAN_POINT ( 'NONE',  ( -5.000000000000000000, -17.95833333060214798, -2.886751345948128211 ) ) ;
#48353=CARTESIAN_POINT ( 'NONE',  ( 5.000000000000000888, -44.45833333060214443, 2.886751345948126879 ) ) ;
#48354=CARTESIAN_POINT ( 'NONE',  ( -4.458734124999999437, -110.4374999986343937, 0.000000000000000000 ) ) ;
#48357=CARTESIAN_POINT ( 'NONE',  ( 2.229367062499998831, -40.64583333196773651, -3.861377020970580887 ) ) ;
#48358=CARTESIAN_POINT ( 'NONE',  ( -2.229367062500000163, -28.72916666530107221, -3.861377020970580443 ) ) ;
#48360=CARTESIAN_POINT ( 'NONE',  ( 2.500000000000002220, 25.33333333333333215, 4.330127018922192761 ) ) ;
#48362=CARTESIAN_POINT ( 'NONE',  ( -4.458734124999998549, -107.4791666653010651, 2.574251347313722516 ) ) ;
#48363=CARTESIAN_POINT ( 'NONE',  ( -4.458734124999998549, -32.22916666530106511, 2.574251347313722516 ) ) ;
#48364=CARTESIAN_POINT ( 'NONE',  ( 2.500000000000002220, -66.54166666393547303, 4.330127018922192761 ) ) ;
#48365=ADVANCED_FACE ( 'NONE', ( #15604 ), #15279, .T. ) ;
#48369=CARTESIAN_POINT ( 'NONE',  ( 2.229367062500001939, -74.22916666530106511, 3.861377020970579999 ) ) ;
#48372=CARTESIAN_POINT ( 'NONE',  ( -1.339745962155610925, -27.66965819600733667, 5.000000000000000000 ) ) ;
#48373=CYLINDRICAL_SURFACE ( 'NONE', #61588, 5.000000000000000000 ) ;
#48374=CARTESIAN_POINT ( 'NONE',  ( -4.999999999999999112, -20.91666666666666785, 2.886751345948131764 ) ) ;
#48376=ORIENTED_EDGE ( 'NONE', *, *, #13729, .T. ) ;
#48378=CARTESIAN_POINT ( 'NONE',  ( 2.499999999999998668, 1.666666666666666963, -4.330127018922193649 ) ) ;
#48380=CARTESIAN_POINT ( 'NONE',  ( 2.500000000000002220, 24.45833333606451987, 4.330127018922192761 ) ) ;
#48383=AXIS2_PLACEMENT_3D ( 'NONE', #42925, #7898, #36849 ) ;
#48384=CARTESIAN_POINT ( 'NONE',  ( 0.000000000000000000, -120.0000000000000000, 5.000000000000000000 ) ) ;
#48386=CARTESIAN_POINT ( 'NONE',  ( -2.916731409357579869E-14, 13.25000000000000178, 5.000000000000000888 ) ) ;
#48389=CARTESIAN_POINT ( 'NONE',  ( 1.339745962155729053, -56.16965819600732601, -4.999999999999933387 ) ) ;
#48390=CARTESIAN_POINT ( 'NONE',  ( 1.339745962155612702, 0.7053418012614794952, -5.000000000000000000 ) ) ;
#48394=ORIENTED_EDGE ( 'NONE', *, *, #46857, .T. ) ;
#48396=VERTEX_POINT ( 'NONE', #6589 ) ;
#48397=FACE_OUTER_BOUND ( 'NONE', #5176, .T. ) ;
#48407=CARTESIAN_POINT ( 'NONE',  ( -2.229367062500000163, 16.52083333469892779, -3.861377020970580443 ) ) ;
#48408=CARTESIAN_POINT ( 'NONE',  ( 1.339745962155612702, -12.16965819600733667, -5.000000000000000000 ) ) ;
#48409=ORIENTED_EDGE ( 'NONE', *, *, #24727, .T. ) ;
#48415=CARTESIAN_POINT ( 'NONE',  ( 4.458734124999999437, -60.81249999863440081, -5.460374474430324690E-16 ) ) ;
#48418=CARTESIAN_POINT ( 'NONE',  ( -2.229367062500000163, 22.52083333469892423, -3.861377020970580443 ) ) ;
#48419=CARTESIAN_POINT ( 'NONE',  ( 5.000000000000000000, -42.49999999999999289, -6.123233995736766282E-16 ) ) ;
#48423=CARTESIAN_POINT ( 'NONE',  ( -2.229367062499996610, -46.39583333196774362, 3.861377020970582219 ) ) ;
#48424=CARTESIAN_POINT ( 'NONE',  ( -4.999999999999999112, -3.791666663935478798, 2.886751345948131764 ) ) ;
#48428=CARTESIAN_POINT ( 'NONE',  ( 4.458734124999999437, -106.8124999986343937, -5.460374474430324690E-16 ) ) ;
#48429=CARTESIAN_POINT ( 'NONE',  ( 4.458734124999999437, -12.06249999863440081, -5.460374474430324690E-16 ) ) ;
#48430=EDGE_CURVE ( 'NONE', #36504, #44414, #25568, .T. ) ;
#48431=ORIENTED_EDGE ( 'NONE', *, *, #15284, .F. ) ;
#48432=CARTESIAN_POINT ( 'NONE',  ( 5.000000000000000888, -52.58333333333332860, 2.886751345948126879 ) ) ;
#48433=CARTESIAN_POINT ( 'NONE',  ( 4.458734124999999437, -99.81249999863440792, -5.460374474430324690E-16 ) ) ;
#48435=CARTESIAN_POINT ( 'NONE',  ( -3.152548672688508926E-16, -91.81249999863442213, -5.148502694627439702 ) ) ;
#48436=CARTESIAN_POINT ( 'NONE',  ( -2.500000000000000444, -52.04166666393547303, -4.330127018922193649 ) ) ;
#48437=EDGE_CURVE ( 'NONE', #50402, #11950, #6915, .T. ) ;
#48439=EDGE_CURVE ( 'NONE', #33230, #55713, #7238, .T. ) ;
#48442=CARTESIAN_POINT ( 'NONE',  ( -2.229367062499996610, -20.14583333196774007, 3.861377020970582219 ) ) ;
#48443=CARTESIAN_POINT ( 'NONE',  ( -4.458734124999998549, 12.52083333469892779, 2.574251347313722516 ) ) ;
#48444=CARTESIAN_POINT ( 'NONE',  ( -4.458734124999999437, -61.64583333196774362, -2.574251347313719407 ) ) ;
#48447=CARTESIAN_POINT ( 'NONE',  ( 1.975475456537005874E-15, -34.62499999726880873, 5.000000000000000000 ) ) ;
#48449=EDGE_CURVE ( 'NONE', #46456, #23583, #36490, .T. ) ;
#48450=ORIENTED_EDGE ( 'NONE', *, *, #58125, .F. ) ;
#48452=DIRECTION ( 'NONE',  ( -0.000000000000000000, 1.000000000000000000, -0.000000000000000000 ) ) ;
#48453=EDGE_CURVE ( 'NONE', #57839, #34229, #26637, .T. ) ;
#48454=CARTESIAN_POINT ( 'NONE',  ( 1.975475456537005874E-15, -64.62499999726880162, 5.000000000000000000 ) ) ;
#48456=CARTESIAN_POINT ( 'NONE',  ( 9.457646018065525792E-16, -86.06249999863439371, 5.148502694627439702 ) ) ;
#48457=CARTESIAN_POINT ( 'NONE',  ( -3.152548672688508926E-16, 20.18750000136559208, -5.148502694627439702 ) ) ;
#48459=EDGE_CURVE ( 'NONE', #721, #14946, #45823, .T. ) ;
#48463=CARTESIAN_POINT ( 'NONE',  ( 2.499999999999998668, -71.33333333333332860, -4.330127018922193649 ) ) ;
#48465=ORIENTED_EDGE ( 'NONE', *, *, #55161, .F. ) ;
#48467=ORIENTED_EDGE ( 'NONE', *, *, #22818, .T. ) ;
#48479=CARTESIAN_POINT ( 'NONE',  ( 0.000000000000000000, -120.0000000000000000, 0.000000000000000000 ) ) ;
#48480=CARTESIAN_POINT ( 'NONE',  ( 9.457646018065525792E-16, -59.31249999863440081, 5.148502694627439702 ) ) ;
#48481=( BOUNDED_CURVE ( )  B_SPLINE_CURVE ( 2, ( #20377, #40623, #4083, #54473, #10400, #28514, #23706, #30012, #45131 ),
 .UNSPECIFIED., .F., .F. ) 
 B_SPLINE_CURVE_WITH_KNOTS ( ( 3, 2, 2, 2, 3 ),
 ( 0.3160714285714285587, 0.3166666666666666519, 0.3178571428571428381, 0.3190476190476190244, 0.3196428571428571175 ),
 .UNSPECIFIED. ) 
 CURVE ( )  GEOMETRIC_REPRESENTATION_ITEM ( )  RATIONAL_B_SPLINE_CURVE ( ( 0.9330127018922194093, 0.9330127018922194093, 1.000000000000000000, 0.8660254037844387076, 1.000000000000000000, 0.8660254037844387076, 1.000000000000000000, 0.9330127018922194093, 0.9330127018922194093 ) ) 
 REPRESENTATION_ITEM ( '' )  );
#48483=CARTESIAN_POINT ( 'NONE',  ( -5.000000000000000000, 10.12500000273118594, 0.000000000000000000 ) ) ;
#48488=ORIENTED_EDGE ( 'NONE', *, *, #16562, .F. ) ;
#48491=CARTESIAN_POINT ( 'NONE',  ( 4.458734124999999437, -103.0624999986344079, -5.460374474430324690E-16 ) ) ;
#48496=CARTESIAN_POINT ( 'NONE',  ( -4.458734124999999437, -36.31249999863440792, 0.000000000000000000 ) ) ;
#48498=CARTESIAN_POINT ( 'NONE',  ( 4.458734125000001214, -11.89583333196774007, 2.574251347313718519 ) ) ;
#48499=CARTESIAN_POINT ( 'NONE',  ( -2.229367062500000163, -100.7291666653010651, -3.861377020970580443 ) ) ;
#48501=CARTESIAN_POINT ( 'NONE',  ( -4.458734124999999437, -28.56249999863440081, 0.000000000000000000 ) ) ;
#48508=CARTESIAN_POINT ( 'NONE',  ( 4.458734124999998549, 3.020833334698928674, -2.574251347313721627 ) ) ;
#48509=ORIENTED_EDGE ( 'NONE', *, *, #27265, .F. ) ;
#48512=CARTESIAN_POINT ( 'NONE',  ( -2.499999999999996447, -97.83333333333332860, 4.330127018922195425 ) ) ;
#48513=CARTESIAN_POINT ( 'NONE',  ( -2.229367062500000163, -27.47916666530107221, -3.861377020970580443 ) ) ;
#48514=CARTESIAN_POINT ( 'NONE',  ( 5.000000000000000000, -73.41666666666665719, -2.886751345948130876 ) ) ;
#48515=CARTESIAN_POINT ( 'NONE',  ( -4.458734124999999437, -74.64583333196773651, -2.574251347313719407 ) ) ;
#48519=CARTESIAN_POINT ( 'NONE',  ( -4.458734124999997661, 3.770833334698929562, 2.574251347313722516 ) ) ;
#48520=CARTESIAN_POINT ( 'NONE',  ( -4.458734124999999437, 25.35416666803225993, -2.574251347313719407 ) ) ;
#48521=CARTESIAN_POINT ( 'NONE',  ( 4.458734124999999437, -45.06249999863440081, -5.460374474430324690E-16 ) ) ;
#48524=ORIENTED_EDGE ( 'NONE', *, *, #35811, .F. ) ;
#48526=( BOUNDED_CURVE ( )  B_SPLINE_CURVE ( 2, ( #21681, #31306, #22310, #62183, #3017, #22632, #2381, #7833, #42231 ),
 .UNSPECIFIED., .F., .F. ) 
 B_SPLINE_CURVE_WITH_KNOTS ( ( 3, 2, 2, 2, 3 ),
 ( 0.5196428571428571841, 0.5202380952380952772, 0.5214285714285714635, 0.5226190476190476497, 0.5232142857142857428 ),
 .UNSPECIFIED. ) 
 CURVE ( )  GEOMETRIC_REPRESENTATION_ITEM ( )  RATIONAL_B_SPLINE_CURVE ( ( 0.9330127018922194093, 0.9330127018922194093, 1.000000000000000000, 0.8660254037844387076, 1.000000000000000000, 0.8660254037844387076, 1.000000000000000000, 0.9330127018922194093, 0.9330127018922194093 ) ) 
 REPRESENTATION_ITEM ( '' )  );
#48528=CARTESIAN_POINT ( 'NONE',  ( -4.458734124999999437, -71.31249999863439371, 0.000000000000000000 ) ) ;
#48529=CARTESIAN_POINT ( 'NONE',  ( -2.499999999999996447, -107.7083333306021444, 4.330127018922195425 ) ) ;
#48531=EDGE_CURVE ( 'NONE', #31783, #47937, #5957, .T. ) ;
#48533=CARTESIAN_POINT ( 'NONE',  ( -2.229367062500000163, -107.7291666653010651, -3.861377020970580443 ) ) ;
#48535=CARTESIAN_POINT ( 'NONE',  ( -3.535250795749689387E-16, -54.24999999999999289, -5.773502691896257311 ) ) ;
#48536=CARTESIAN_POINT ( 'NONE',  ( -2.500000000000000444, -66.16666666666667140, -4.330127018922193649 ) ) ;
#48548=CARTESIAN_POINT ( 'NONE',  ( 1.339745962155615144, -98.70534180126146850, 4.999999999999999112 ) ) ;
#48550=ORIENTED_EDGE ( 'NONE', *, *, #33124, .T. ) ;
#48554=CARTESIAN_POINT ( 'NONE',  ( 4.458734124999998549, -39.97916666530107221, -2.574251347313721627 ) ) ;
#48564=CARTESIAN_POINT ( 'NONE',  ( -3.152548672688508926E-16, -91.81249999863442213, -5.148502694627439702 ) ) ;
#48565=LINE ( 'NONE', #13541, #54363 ) ;
#48566=ORIENTED_EDGE ( 'NONE', *, *, #5618, .T. ) ;
#48567=CARTESIAN_POINT ( 'NONE',  ( -6.972266317189433020E-16, -47.24999999999999289, -5.000000000000000000 ) ) ;
#48570=DIRECTION ( 'NONE',  ( -0.000000000000000000, 1.000000000000000000, -0.000000000000000000 ) ) ;
#48572=CARTESIAN_POINT ( 'NONE',  ( 2.500000000000002220, -78.66666666666665719, 4.330127018922192761 ) ) ;
#48573=CARTESIAN_POINT ( 'NONE',  ( -2.229367062500000163, -11.72916666530107044, -3.861377020970580443 ) ) ;
#48578=CARTESIAN_POINT ( 'NONE',  ( 2.229367062500001939, 19.77083333469892779, 3.861377020970579999 ) ) ;
#48579=ORIENTED_EDGE ( 'NONE', *, *, #26460, .T. ) ;
#48580=CARTESIAN_POINT ( 'NONE',  ( 2.229367062499998831, -90.64583333196773651, -3.861377020970580887 ) ) ;
#48583=CARTESIAN_POINT ( 'NONE',  ( -2.229367062500000163, -14.47916666530107221, -3.861377020970580443 ) ) ;
#48584=CARTESIAN_POINT ( 'NONE',  ( 2.500000000000002220, -39.54166666393548013, 4.330127018922192761 ) ) ;
#48587=CARTESIAN_POINT ( 'NONE',  ( -5.000000000000000000, -38.95833333060214443, -2.886751345948128211 ) ) ;
#48589=CARTESIAN_POINT ( 'NONE',  ( -4.458734124999997661, 20.77083333469892779, 2.574251347313722516 ) ) ;
#48590=CARTESIAN_POINT ( 'NONE',  ( -6.972266317189433020E-16, -51.12499999726880873, -5.000000000000000000 ) ) ;
#48593=CARTESIAN_POINT ( 'NONE',  ( -3.152548672688508926E-16, -64.56249999863440792, -5.148502694627439702 ) ) ;
#48596=CARTESIAN_POINT ( 'NONE',  ( 5.000000000000000000, 9.583333333333333925, -2.886751345948129988 ) ) ;
#48599=CARTESIAN_POINT ( 'NONE',  ( 2.229367062499998831, -52.64583333196773651, -3.861377020970580887 ) ) ;
#48600=CARTESIAN_POINT ( 'NONE',  ( 2.499999999999998668, -89.20833333060214443, -4.330127018922193649 ) ) ;
#48602=( BOUNDED_CURVE ( )  B_SPLINE_CURVE ( 2, ( #50735, #60720, #40757, #50428, #2192, #31420, #60406, #51059, #11498 ),
 .UNSPECIFIED., .F., .F. ) 
 B_SPLINE_CURVE_WITH_KNOTS ( ( 3, 2, 2, 2, 3 ),
 ( 0.7232142857142856984, 0.7238095238095237915, 0.7249999999999999778, 0.7261904761904761640, 0.7267857142857142572 ),
 .UNSPECIFIED. ) 
 CURVE ( )  GEOMETRIC_REPRESENTATION_ITEM ( )  RATIONAL_B_SPLINE_CURVE ( ( 0.9330127018922194093, 0.9330127018922194093, 1.000000000000000000, 0.8660254037844387076, 1.000000000000000000, 0.8660254037844387076, 1.000000000000000000, 0.9330127018922194093, 0.9330127018922194093 ) ) 
 REPRESENTATION_ITEM ( '' )  );
#48605=CARTESIAN_POINT ( 'NONE',  ( 4.458734124999998549, -89.97916666530106511, -2.574251347313721627 ) ) ;
#48607=CARTESIAN_POINT ( 'NONE',  ( -2.499999999999996447, -35.83333333333332860, 4.330127018922195425 ) ) ;
#48608=CARTESIAN_POINT ( 'NONE',  ( 1.975475456537005874E-15, 19.25000000000000000, 5.000000000000000000 ) ) ;
#48609=CARTESIAN_POINT ( 'NONE',  ( 1.339745962155615144, -22.70534180126147916, 4.999999999999999112 ) ) ;
#48611=CARTESIAN_POINT ( 'NONE',  ( -2.229367062500000163, -102.4791666653010651, -3.861377020970580443 ) ) ;
#48612=CARTESIAN_POINT ( 'NONE',  ( 2.229367062499998831, 8.104166668032261711, -3.861377020970580887 ) ) ;
#48621=CARTESIAN_POINT ( 'NONE',  ( 2.500000000000002220, 19.33333333333333570, 4.330127018922192761 ) ) ;
#48625=CARTESIAN_POINT ( 'NONE',  ( -3.152548672688508926E-16, -25.81249999863440792, -5.148502694627439702 ) ) ;
#48626=CARTESIAN_POINT ( 'NONE',  ( -6.972266317189433020E-16, -58.24999999999999289, -5.000000000000000000 ) ) ;
#48637=CARTESIAN_POINT ( 'NONE',  ( -2.229367062499996610, -73.39583333196773651, 3.861377020970582219 ) ) ;
#48643=CARTESIAN_POINT ( 'NONE',  ( 9.457646018065525792E-16, 0.6875000013655957476, 5.148502694627439702 ) ) ;
#48652=CARTESIAN_POINT ( 'NONE',  ( -2.229367062499996610, -76.14583333196773651, 3.861377020970582219 ) ) ;
#48653=CARTESIAN_POINT ( 'NONE',  ( 1.339745962155615144, -0.5803417985302927740, 4.999999999999999112 ) ) ;
#48654=CARTESIAN_POINT ( 'NONE',  ( -4.458734124999998549, -0.2291666653010705768, 2.574251347313722516 ) ) ;
#48657=CARTESIAN_POINT ( 'NONE',  ( 4.458734124999998549, -63.97916666530107221, -2.574251347313721627 ) ) ;
#48658=CARTESIAN_POINT ( 'NONE',  ( -4.999999999999999112, -26.79166666393548013, 2.886751345948131764 ) ) ;
#48660=CYLINDRICAL_SURFACE ( 'NONE', #37797, 5.000000000000000000 ) ;
#48663=CARTESIAN_POINT ( 'NONE',  ( -4.458734124999999437, -45.39583333196773651, -2.574251347313719407 ) ) ;
#48664=CARTESIAN_POINT ( 'NONE',  ( -4.458734124999999437, -27.64583333196774007, -2.574251347313719407 ) ) ;
#48666=( BOUNDED_CURVE ( )  B_SPLINE_CURVE ( 2, ( #59458, #15390, #30163, #5738, #34683, #54303, #10244, #45290, #25356 ),
 .UNSPECIFIED., .F., .F. ) 
 B_SPLINE_CURVE_WITH_KNOTS ( ( 3, 2, 2, 2, 3 ),
 ( 0.3232142857142857317, 0.3238095238095238249, 0.3250000000000000111, 0.3261904761904761973, 0.3267857142857142905 ),
 .UNSPECIFIED. ) 
 CURVE ( )  GEOMETRIC_REPRESENTATION_ITEM ( )  RATIONAL_B_SPLINE_CURVE ( ( 0.9330127018922194093, 0.9330127018922194093, 1.000000000000000000, 0.8660254037844387076, 1.000000000000000000, 0.8660254037844387076, 1.000000000000000000, 0.9330127018922194093, 0.9330127018922194093 ) ) 
 REPRESENTATION_ITEM ( '' )  );
#48668=CARTESIAN_POINT ( 'NONE',  ( 5.000000000000000888, 28.41666666666666430, 2.886751345948126879 ) ) ;
#48671=CARTESIAN_POINT ( 'NONE',  ( 2.229367062500001939, -34.97916666530107221, 3.861377020970579999 ) ) ;
#48672=CARTESIAN_POINT ( 'NONE',  ( 5.000000000000000888, -67.45833333060213022, 2.886751345948126879 ) ) ;
#48675=CARTESIAN_POINT ( 'NONE',  ( -2.229367062499996610, -76.39583333196773651, 3.861377020970582219 ) ) ;
#48679=FACE_OUTER_BOUND ( 'NONE', #2124, .T. ) ;
#48680=CARTESIAN_POINT ( 'NONE',  ( 1.060575238724906964E-15, -22.75000000000000000, 5.773502691896257311 ) ) ;
#48686=CARTESIAN_POINT ( 'NONE',  ( 5.000000000000000000, 26.70833333606451632, -2.886751345948129988 ) ) ;
#48690=CARTESIAN_POINT ( 'NONE',  ( -2.499999999999996447, 8.291666669397852019, 4.330127018922195425 ) ) ;
#48694=CARTESIAN_POINT ( 'NONE',  ( 2.499999999999998668, -89.20833333060214443, -4.330127018922193649 ) ) ;
#48695=CARTESIAN_POINT ( 'NONE',  ( -6.972266317189433020E-16, -88.12499999726880162, -5.000000000000000000 ) ) ;
#48696=( BOUNDED_CURVE ( )  B_SPLINE_CURVE ( 2, ( #4591, #24214, #43820, #47404, #3355, #22972, #42572, #28095, #3668 ),
 .UNSPECIFIED., .F., .F. ) 
 B_SPLINE_CURVE_WITH_KNOTS ( ( 3, 2, 2, 2, 3 ),
 ( 0.1625000000000000056, 0.1630952380952380987, 0.1642857142857142849, 0.1654761904761904712, 0.1660714285714285643 ),
 .UNSPECIFIED. ) 
 CURVE ( )  GEOMETRIC_REPRESENTATION_ITEM ( )  RATIONAL_B_SPLINE_CURVE ( ( 0.9330127018922194093, 0.9330127018922194093, 1.000000000000000000, 0.8660254037844387076, 1.000000000000000000, 0.8660254037844387076, 1.000000000000000000, 0.9330127018922194093, 0.9330127018922194093 ) ) 
 REPRESENTATION_ITEM ( '' )  );
#48697=CARTESIAN_POINT ( 'NONE',  ( 2.229367062499998831, -22.64583333196773651, -3.861377020970580887 ) ) ;
#48698=CARTESIAN_POINT ( 'NONE',  ( -5.000000000000000000, -71.95833333060214443, -2.886751345948128211 ) ) ;
#48702=AXIS2_PLACEMENT_3D ( 'NONE', #1993, #20964, #41192 ) ;
#48704=ORIENTED_EDGE ( 'NONE', *, *, #28849, .T. ) ;
#48706=VERTEX_POINT ( 'NONE', #3359 ) ;
#48707=DIRECTION ( 'NONE',  ( 0.000000000000000000, 0.000000000000000000, 1.000000000000000000 ) ) ;
#48708=CARTESIAN_POINT ( 'NONE',  ( 1.339745962155615144, -9.580341798530296771, 4.999999999999999112 ) ) ;
#48712=EDGE_CURVE ( 'NONE', #26939, #58774, #59511, .T. ) ;
#48719=CARTESIAN_POINT ( 'NONE',  ( 4.458734125000001214, 20.10416666803225993, 2.574251347313718519 ) ) ;
#48721=EDGE_CURVE ( 'NONE', #13464, #25378, #5328, .T. ) ;
#48726=CARTESIAN_POINT ( 'NONE',  ( 4.458734124999999437, -57.81249999863440081, -5.460374474430324690E-16 ) ) ;
#48727=CARTESIAN_POINT ( 'NONE',  ( 4.458734124999998549, 17.27083333469892779, -2.574251347313721627 ) ) ;
#48729=CARTESIAN_POINT ( 'NONE',  ( 4.458734124999998549, -49.97916666530106511, -2.574251347313721627 ) ) ;
#48730=CARTESIAN_POINT ( 'NONE',  ( 5.000000000000000888, -8.458333330602146205, 2.886751345948126879 ) ) ;
#48734=CARTESIAN_POINT ( 'NONE',  ( 4.458734124999998549, -105.7291666653010651, -2.574251347313721627 ) ) ;
#48735=CARTESIAN_POINT ( 'NONE',  ( -4.458734124999999437, -13.56249999863440259, 0.000000000000000000 ) ) ;
#48737=CARTESIAN_POINT ( 'NONE',  ( -4.458734124999999437, -99.31249999863440792, 0.000000000000000000 ) ) ;
#48739=CARTESIAN_POINT ( 'NONE',  ( 4.458734125000001214, -95.14583333196772230, 2.574251347313718519 ) ) ;
#48741=CARTESIAN_POINT ( 'NONE',  ( -2.500000000000000444, -8.166666666666669627, -4.330127018922193649 ) ) ;
#48742=CARTESIAN_POINT ( 'NONE',  ( -4.999999999999999112, -50.79166666393547303, 2.886751345948131764 ) ) ;
#48743=CARTESIAN_POINT ( 'NONE',  ( 1.975475456537005874E-15, -36.62499999726880873, 5.000000000000000000 ) ) ;
#48747=CARTESIAN_POINT ( 'NONE',  ( -4.458734124999999437, -20.31249999863440081, 0.000000000000000000 ) ) ;
#48748=CARTESIAN_POINT ( 'NONE',  ( -4.458734124999999437, 13.35416666803225993, -2.574251347313719407 ) ) ;
#48749=CARTESIAN_POINT ( 'NONE',  ( -3.152548672688508926E-16, -59.81249999863440792, -5.148502694627439702 ) ) ;
#48754=CARTESIAN_POINT ( 'NONE',  ( 5.000000000000000000, -5.416666666666666963, -2.886751345948129988 ) ) ;
#48758=CARTESIAN_POINT ( 'NONE',  ( -1.339745962155613812, -92.08034179853028434, -5.000000000000000000 ) ) ;
#48759=CARTESIAN_POINT ( 'NONE',  ( -2.500000000000000444, -25.16666666666666430, -4.330127018922193649 ) ) ;
#48760=CARTESIAN_POINT ( 'NONE',  ( -4.458734124999999437, -83.31249999863439371, 0.000000000000000000 ) ) ;
#48761=CARTESIAN_POINT ( 'NONE',  ( -4.458734124999998549, 21.52083333469893134, 2.574251347313722516 ) ) ;
#48763=CARTESIAN_POINT ( 'NONE',  ( 2.500000000000002220, -0.6666666666666660745, 4.330127018922192761 ) ) ;
#48765=CARTESIAN_POINT ( 'NONE',  ( 1.339745962155612702, 20.83034180399265978, -5.000000000000000000 ) ) ;
#48767=CARTESIAN_POINT ( 'NONE',  ( 5.000000000000000888, -76.58333333333332860, 2.886751345948126879 ) ) ;
#48769=ORIENTED_EDGE ( 'NONE', *, *, #25215, .F. ) ;
#48770=DIRECTION ( 'NONE',  ( 0.000000000000000000, 0.000000000000000000, 1.000000000000000000 ) ) ;
#48771=EDGE_LOOP ( 'NONE', ( #57938, #16623, #12568, #1000 ) ) ;
#48776=EDGE_CURVE ( 'NONE', #27142, #29335, #42577, .T. ) ;
#48788=CARTESIAN_POINT ( 'NONE',  ( 2.229367062499998831, -56.89583333196773651, -3.861377020970580887 ) ) ;
#48791=EDGE_LOOP ( 'NONE', ( #33541, #19686, #3172, #57030 ) ) ;
#48794=ADVANCED_FACE ( 'NONE', ( #28099 ), #3673, .T. ) ;
#48796=( BOUNDED_CURVE ( )  B_SPLINE_CURVE ( 2, ( #16087, #11573, #25742, #35711, #50822, #45356, #55339, #11255, #30880 ),
 .UNSPECIFIED., .F., .F. ) 
 B_SPLINE_CURVE_WITH_KNOTS ( ( 3, 2, 2, 2, 3 ),
 ( 0.3053571428571428825, 0.3059523809523809756, 0.3071428571428571619, 0.3083333333333333481, 0.3089285714285714413 ),
 .UNSPECIFIED. ) 
 CURVE ( )  GEOMETRIC_REPRESENTATION_ITEM ( )  RATIONAL_B_SPLINE_CURVE ( ( 0.9330127018922194093, 0.9330127018922194093, 1.000000000000000000, 0.8660254037844387076, 1.000000000000000000, 0.8660254037844387076, 1.000000000000000000, 0.9330127018922194093, 0.9330127018922194093 ) ) 
 REPRESENTATION_ITEM ( '' )  );
#48799=CARTESIAN_POINT ( 'NONE',  ( 4.458734124999999437, -104.0624999986344079, -5.460374474430324690E-16 ) ) ;
#48805=CARTESIAN_POINT ( 'NONE',  ( 4.458734124999998549, -38.72916666530106511, -2.574251347313721627 ) ) ;
#48808=CARTESIAN_POINT ( 'NONE',  ( 6.158835246850667461E-14, -2.250000000000001776, -4.999999999999999112 ) ) ;
#48809=CARTESIAN_POINT ( 'NONE',  ( 9.457646018065525792E-16, -11.06249999863440969, 5.148502694627439702 ) ) ;
#48810=CARTESIAN_POINT ( 'NONE',  ( 4.458734124999998549, -100.9791666653010509, -2.574251347313721627 ) ) ;
#48811=ORIENTED_EDGE ( 'NONE', *, *, #48449, .F. ) ;
#48813=CARTESIAN_POINT ( 'NONE',  ( -3.152548672688508926E-16, -34.81249999863440792, -5.148502694627439702 ) ) ;
#48817=CARTESIAN_POINT ( 'NONE',  ( 1.339745962155615144, -17.70534180126147916, 4.999999999999999112 ) ) ;
#48820=CARTESIAN_POINT ( 'NONE',  ( -4.458734124999999437, 3.354166668032260823, -2.574251347313719407 ) ) ;
#48824=CARTESIAN_POINT ( 'NONE',  ( 2.500000000000002220, -96.66666666666665719, 4.330127018922192761 ) ) ;
#48825=CARTESIAN_POINT ( 'NONE',  ( 2.229367062500001939, -31.97916666530106866, 3.861377020970579999 ) ) ;
#48826=CARTESIAN_POINT ( 'NONE',  ( -5.000000000000000000, -22.87499999726881228, 0.000000000000000000 ) ) ;
#48827=CARTESIAN_POINT ( 'NONE',  ( 4.458734124999999437, -78.06249999863440792, -5.460374474430324690E-16 ) ) ;
#48831=CARTESIAN_POINT ( 'NONE',  ( 4.458734124999998549, -4.729166665301071326, -2.574251347313721627 ) ) ;
#48832=CARTESIAN_POINT ( 'NONE',  ( 4.458734124999999437, 24.93750000136559208, -5.460374474430324690E-16 ) ) ;
#48833=CARTESIAN_POINT ( 'NONE',  ( -2.229367062499996610, -42.39583333196773651, 3.861377020970582219 ) ) ;
#48838=CARTESIAN_POINT ( 'NONE',  ( -2.229367062500000163, -67.47916666530106511, -3.861377020970580443 ) ) ;
#48839=CARTESIAN_POINT ( 'NONE',  ( -2.500000000000000444, -107.0416666639354730, -4.330127018922193649 ) ) ;
#48840=AXIS2_PLACEMENT_3D ( 'NONE', #62069, #31836, #12533 ) ;
#48843=CARTESIAN_POINT ( 'NONE',  ( 1.975475456537005874E-15, -33.75000000000000000, 5.000000000000000000 ) ) ;
#48845=CARTESIAN_POINT ( 'NONE',  ( -2.499999999999996447, -54.83333333333332860, 4.330127018922195425 ) ) ;
#48848=ORIENTED_EDGE ( 'NONE', *, *, #13362, .F. ) ;
#48850=( BOUNDED_CURVE ( )  B_SPLINE_CURVE ( 2, ( #19896, #34694, #11527, #54641, #36297, #55920, #49805, #35982, #20228 ),
 .UNSPECIFIED., .F., .F. ) 
 B_SPLINE_CURVE_WITH_KNOTS ( ( 3, 2, 2, 2, 3 ),
 ( 0.4339285714285714413, 0.4345238095238095344, 0.4357142857142857206, 0.4369047619047619069, 0.4375000000000000000 ),
 .UNSPECIFIED. ) 
 CURVE ( )  GEOMETRIC_REPRESENTATION_ITEM ( )  RATIONAL_B_SPLINE_CURVE ( ( 0.9330127018922194093, 0.9330127018922194093, 1.000000000000000000, 0.8660254037844387076, 1.000000000000000000, 0.8660254037844387076, 1.000000000000000000, 0.9330127018922194093, 0.9330127018922194093 ) ) 
 REPRESENTATION_ITEM ( '' )  );
#48851=CARTESIAN_POINT ( 'NONE',  ( -1.339745962155625802, 13.20534180126147916, 4.999999999999991118 ) ) ;
#48865=CARTESIAN_POINT ( 'NONE',  ( -4.458734124999999437, -43.56249999863440081, 0.000000000000000000 ) ) ;
#48868=CARTESIAN_POINT ( 'NONE',  ( -1.339745962155610925, -56.66965819600733312, 5.000000000000000000 ) ) ;
#48874=CARTESIAN_POINT ( 'NONE',  ( -2.229367062500000163, -90.72916666530106511, -3.861377020970580443 ) ) ;
#48876=ORIENTED_EDGE ( 'NONE', *, *, #39672, .F. ) ;
#48877=EDGE_CURVE ( 'NONE', #50850, #54554, #40273, .T. ) ;
#48879=CARTESIAN_POINT ( 'NONE',  ( 1.975475456537005874E-15, 6.375000002731185944, 5.000000000000000000 ) ) ;
#48884=CARTESIAN_POINT ( 'NONE',  ( -2.229367062500000163, 3.520833334698929118, -3.861377020970580443 ) ) ;
#48887=CARTESIAN_POINT ( 'NONE',  ( 9.457646018065525792E-16, -14.31249999863440259, 5.148502694627439702 ) ) ;
#48888=CARTESIAN_POINT ( 'NONE',  ( -6.972266317189433020E-16, -105.1249999972687874, -5.000000000000000000 ) ) ;
#48890=DIRECTION ( 'NONE',  ( -0.000000000000000000, 1.000000000000000000, -0.000000000000000000 ) ) ;
#48893=CARTESIAN_POINT ( 'NONE',  ( 4.458734124999999437, 21.93750000136559208, -5.460374474430324690E-16 ) ) ;
#48895=CARTESIAN_POINT ( 'NONE',  ( 4.458734124999998549, -95.72916666530107932, -2.574251347313721627 ) ) ;
#48898=CARTESIAN_POINT ( 'NONE',  ( -2.229367062499996610, -16.14583333196773651, 3.861377020970582219 ) ) ;
#48901=CARTESIAN_POINT ( 'NONE',  ( -5.000000000000000000, -88.00000000000000000, 0.000000000000000000 ) ) ;
#48902=CARTESIAN_POINT ( 'NONE',  ( 2.500000000000002220, -41.54166666393548013, 4.330127018922192761 ) ) ;
#48903=CARTESIAN_POINT ( 'NONE',  ( 5.000000000000000000, -29.50000000000000000, -6.123233995736766282E-16 ) ) ;
#48904=CARTESIAN_POINT ( 'NONE',  ( -3.152548672688508926E-16, 15.43750000136559564, -5.148502694627439702 ) ) ;
#48908=CARTESIAN_POINT ( 'NONE',  ( 4.458734124999999437, -62.81249999863440792, -5.460374474430324690E-16 ) ) ;
#48911=CARTESIAN_POINT ( 'NONE',  ( 1.060575238724906964E-15, 11.25000000000000000, 5.773502691896257311 ) ) ;
#48914=CARTESIAN_POINT ( 'NONE',  ( 9.457646018065525792E-16, -56.06249999863440792, 5.148502694627439702 ) ) ;
#48915=CARTESIAN_POINT ( 'NONE',  ( 1.060575238724906964E-15, -90.62499999726880162, 5.773502691896257311 ) ) ;
#48920=CARTESIAN_POINT ( 'NONE',  ( -3.535250795749689387E-16, -36.25000000000000711, -5.773502691896257311 ) ) ;
#48921=CARTESIAN_POINT ( 'NONE',  ( -1.339745962155555858, -20.08034179853028789, -5.000000000000032863 ) ) ;
#48923=EDGE_LOOP ( 'NONE', ( #20352, #33238, #60618, #51743 ) ) ;
#48924=CARTESIAN_POINT ( 'NONE',  ( -3.152548672688508926E-16, -102.5624999986344079, -5.148502694627439702 ) ) ;
#48925=CARTESIAN_POINT ( 'NONE',  ( 2.229367062500001939, 1.770833334698927786, 3.861377020970579999 ) ) ;
#48926=CARTESIAN_POINT ( 'NONE',  ( 5.000000000000000000, -80.41666666666665719, -2.886751345948130876 ) ) ;
#48930=CARTESIAN_POINT ( 'NONE',  ( -5.000000000000000000, 2.999999999999999112, 0.000000000000000000 ) ) ;
#48938=CARTESIAN_POINT ( 'NONE',  ( -4.999999999999998224, 24.20833333606451987, 2.886751345948131764 ) ) ;
#48939=CARTESIAN_POINT ( 'NONE',  ( -4.458734124999999437, -22.56249999863440436, 0.000000000000000000 ) ) ;
#48940=DIRECTION ( 'NONE',  ( -0.000000000000000000, 1.000000000000000000, -0.000000000000000000 ) ) ;
#48950=CARTESIAN_POINT ( 'NONE',  ( -4.458734124999999437, -75.56249999863440792, 0.000000000000000000 ) ) ;
#48952=ORIENTED_EDGE ( 'NONE', *, *, #55511, .F. ) ;
#48953=CARTESIAN_POINT ( 'NONE',  ( 3.044556291839386294E-14, 12.75000000000000000, -5.000000000000000000 ) ) ;
#48956=CARTESIAN_POINT ( 'NONE',  ( 4.458734124999999437, -0.06249999863440491854, -5.460374474430324690E-16 ) ) ;
#48957=ORIENTED_EDGE ( 'NONE', *, *, #39366, .F. ) ;
#48958=CARTESIAN_POINT ( 'NONE',  ( -4.999999999999998224, -19.91666666666666430, 2.886751345948131764 ) ) ;
#48965=ORIENTED_EDGE ( 'NONE', *, *, #54173, .T. ) ;
#48966=CARTESIAN_POINT ( 'NONE',  ( -3.152548672688508926E-16, -74.56249999863442213, -5.148502694627439702 ) ) ;
#48968=CARTESIAN_POINT ( 'NONE',  ( -4.458734124999999437, 2.604166668032263043, -2.574251347313719407 ) ) ;
#48969=VECTOR ( 'NONE', #29119, 1000.000000000000000 ) ;
#48970=AXIS2_PLACEMENT_3D ( 'NONE', #18756, #14248, #44141 ) ;
#48971=( BOUNDED_CURVE ( )  B_SPLINE_CURVE ( 2, ( #17971, #8643, #3828, #58158, #9269, #34029, #42729, #22825, #32776 ),
 .UNSPECIFIED., .F., .F. ) 
 B_SPLINE_CURVE_WITH_KNOTS ( ( 3, 2, 2, 2, 3 ),
 ( 0.8625000000000000444, 0.8630952380952381375, 0.8642857142857143238, 0.8654761904761905100, 0.8660714285714286031 ),
 .UNSPECIFIED. ) 
 CURVE ( )  GEOMETRIC_REPRESENTATION_ITEM ( )  RATIONAL_B_SPLINE_CURVE ( ( 0.9330127018922194093, 0.9330127018922194093, 1.000000000000000000, 0.8660254037844387076, 1.000000000000000000, 0.8660254037844387076, 1.000000000000000000, 0.9330127018922194093, 0.9330127018922194093 ) ) 
 REPRESENTATION_ITEM ( '' )  );
#48973=CARTESIAN_POINT ( 'NONE',  ( 2.229367062500001939, -66.22916666530106511, 3.861377020970579999 ) ) ;
#48975=CARTESIAN_POINT ( 'NONE',  ( 5.000000000000000000, -23.37499999726881228, -6.123233995736766282E-16 ) ) ;
#48977=CARTESIAN_POINT ( 'NONE',  ( 2.500000000000002220, -28.54166666393548013, 4.330127018922192761 ) ) ;
#48979=DIRECTION ( 'NONE',  ( 0.000000000000000000, 0.000000000000000000, 1.000000000000000000 ) ) ;
#48980=CARTESIAN_POINT ( 'NONE',  ( 9.457646018065525792E-16, -46.06249999863440081, 5.148502694627439702 ) ) ;
#48981=CARTESIAN_POINT ( 'NONE',  ( 9.457646018065525792E-16, -27.31249999863440081, 5.148502694627439702 ) ) ;
#48983=LINE ( 'NONE', #55099, #41166 ) ;
#48984=CARTESIAN_POINT ( 'NONE',  ( -4.999999999999999112, 27.08333333333333215, 2.886751345948131764 ) ) ;
#48988=CARTESIAN_POINT ( 'NONE',  ( -3.152548672688508926E-16, -39.56249999863440081, -5.148502694627439702 ) ) ;
#48989=CARTESIAN_POINT ( 'NONE',  ( -2.500000000000000444, -71.04166666393547303, -4.330127018922193649 ) ) ;
#48992=CARTESIAN_POINT ( 'NONE',  ( -4.458734124999997661, -72.47916666530107932, 2.574251347313722516 ) ) ;
#48997=CARTESIAN_POINT ( 'NONE',  ( -2.500000000000000444, -24.16666666666666430, -4.330127018922193649 ) ) ;
#49001=ORIENTED_EDGE ( 'NONE', *, *, #21146, .F. ) ;
#49003=CARTESIAN_POINT ( 'NONE',  ( -4.999999999999999112, 23.20833333606451632, 2.886751345948131764 ) ) ;
#49004=CARTESIAN_POINT ( 'NONE',  ( 1.339745962155612702, 4.830341803992664218, -5.000000000000000000 ) ) ;
#49010=CARTESIAN_POINT ( 'NONE',  ( 1.975475456537005874E-15, -91.62499999726877320, 5.000000000000000000 ) ) ;
#49011=CARTESIAN_POINT ( 'NONE',  ( -5.000000000000000000, -87.87499999726880162, 0.000000000000000000 ) ) ;
#49013=CARTESIAN_POINT ( 'NONE',  ( 9.457646018065525792E-16, -21.06249999863440436, 5.148502694627439702 ) ) ;
#49014=AXIS2_PLACEMENT_3D ( 'NONE', #2179, #36885, #56192 ) ;
#49015=CARTESIAN_POINT ( 'NONE',  ( 1.339745962155615144, 10.41965820146970501, 4.999999999999999112 ) ) ;
#49026=CARTESIAN_POINT ( 'NONE',  ( 1.339745962155615144, -4.705341801261478274, 4.999999999999999112 ) ) ;
#49027=CARTESIAN_POINT ( 'NONE',  ( 2.499999999999998668, -9.208333330602146205, -4.330127018922193649 ) ) ;
#49029=VERTEX_POINT ( 'NONE', #54768 ) ;
#49030=CARTESIAN_POINT ( 'NONE',  ( 1.339745962155615144, -23.58034179853029144, 4.999999999999999112 ) ) ;
#49034=ORIENTED_EDGE ( 'NONE', *, *, #54997, .F. ) ;
#49035=CARTESIAN_POINT ( 'NONE',  ( 6.123233995736766282E-16, -120.0000000000000000, -5.000000000000000000 ) ) ;
#49036=CARTESIAN_POINT ( 'NONE',  ( -2.229367062500000163, 21.52083333469892779, -3.861377020970580443 ) ) ;
#49040=FACE_OUTER_BOUND ( 'NONE', #35862, .T. ) ;
#49041=CARTESIAN_POINT ( 'NONE',  ( 5.000000000000000888, -100.5833333333333286, 2.886751345948126879 ) ) ;
#49043=CARTESIAN_POINT ( 'NONE',  ( 2.229367062500001939, -58.97916666530106511, 3.861377020970579999 ) ) ;
#49045=CARTESIAN_POINT ( 'NONE',  ( -2.229367062500000163, 17.52083333469892779, -3.861377020970580443 ) ) ;
#49046=DIRECTION ( 'NONE',  ( -0.000000000000000000, 1.000000000000000000, -0.000000000000000000 ) ) ;
#49047=CARTESIAN_POINT ( 'NONE',  ( -4.458734124999999437, -48.56249999863440792, 0.000000000000000000 ) ) ;
#49048=CARTESIAN_POINT ( 'NONE',  ( -5.000000000000000000, -7.958333330602145317, -2.886751345948128211 ) ) ;
#49051=CARTESIAN_POINT ( 'NONE',  ( -5.000000000000000000, -74.00000000000000000, 0.000000000000000000 ) ) ;
#49052=CARTESIAN_POINT ( 'NONE',  ( 2.229367062499998831, -109.6458333319677365, -3.861377020970580887 ) ) ;
#49053=CARTESIAN_POINT ( 'NONE',  ( 4.458734124999999437, -11.06249999863440792, -5.460374474430324690E-16 ) ) ;
#49054=ORIENTED_EDGE ( 'NONE', *, *, #12644, .T. ) ;
#49056=CARTESIAN_POINT ( 'NONE',  ( -2.499999999999996447, -46.70833333060214443, 4.330127018922195425 ) ) ;
#49057=CARTESIAN_POINT ( 'NONE',  ( 2.229367062500001939, -97.97916666530105090, 3.861377020970579999 ) ) ;
#49059=CARTESIAN_POINT ( 'NONE',  ( 4.458734124999998549, -96.97916666530106511, -2.574251347313721627 ) ) ;
#49063=CARTESIAN_POINT ( 'NONE',  ( -2.500000000000000444, -57.04166666393548013, -4.330127018922193649 ) ) ;
#49067=CARTESIAN_POINT ( 'NONE',  ( -4.458734124999999437, -16.31249999863440436, 0.000000000000000000 ) ) ;
#49068=CARTESIAN_POINT ( 'NONE',  ( 2.229367062500001939, 4.770833334698926897, 3.861377020970579999 ) ) ;
#49069=CARTESIAN_POINT ( 'NONE',  ( -3.152548672688508926E-16, -58.81249999863440081, -5.148502694627439702 ) ) ;
#49073=CARTESIAN_POINT ( 'NONE',  ( 5.000000000000000888, -8.583333333333330373, 2.886751345948126879 ) ) ;
#49074=ORIENTED_EDGE ( 'NONE', *, *, #58870, .F. ) ;
#49076=( BOUNDED_CURVE ( )  B_SPLINE_CURVE ( 2, ( #51612, #31977, #41939, #61580, #17515, #32292, #7545, #50647, #3042 ),
 .UNSPECIFIED., .F., .F. ) 
 B_SPLINE_CURVE_WITH_KNOTS ( ( 3, 2, 2, 2, 3 ),
 ( 0.7660714285714286254, 0.7666666666666667185, 0.7678571428571429047, 0.7690476190476190910, 0.7696428571428571841 ),
 .UNSPECIFIED. ) 
 CURVE ( )  GEOMETRIC_REPRESENTATION_ITEM ( )  RATIONAL_B_SPLINE_CURVE ( ( 0.9330127018922194093, 0.9330127018922256266, 1.000000000000000000, 0.8660254037844387076, 1.000000000000000000, 0.8660254037844387076, 1.000000000000000000, 0.9330127018922194093, 0.9330127018922194093 ) ) 
 REPRESENTATION_ITEM ( '' )  );
#49080=CARTESIAN_POINT ( 'NONE',  ( 9.457646018065525792E-16, -87.06249999863440792, 5.148502694627439702 ) ) ;
#49081=CARTESIAN_POINT ( 'NONE',  ( 4.458734125000001214, 19.85416666803226349, 2.574251347313718519 ) ) ;
#49084=CARTESIAN_POINT ( 'NONE',  ( 1.339745962155615144, -0.7053418012614794952, 4.999999999999999112 ) ) ;
#49085=EDGE_CURVE ( 'NONE', #8062, #42248, #62078, .T. ) ;
#49086=CARTESIAN_POINT ( 'NONE',  ( -1.339745962155613812, -7.205341801261479162, -5.000000000000000000 ) ) ;
#49089=CARTESIAN_POINT ( 'NONE',  ( -4.999999999999999112, -77.91666666666665719, 2.886751345948131764 ) ) ;
#49092=FACE_OUTER_BOUND ( 'NONE', #15200, .T. ) ;
#49094=CARTESIAN_POINT ( 'NONE',  ( 0.000000000000000000, -120.0000000000000000, 0.000000000000000000 ) ) ;
#49097=EDGE_CURVE ( 'NONE', #37277, #61639, #8707, .T. ) ;
#49100=ORIENTED_EDGE ( 'NONE', *, *, #18613, .F. ) ;
#49107=CARTESIAN_POINT ( 'NONE',  ( -3.152548672688508926E-16, -59.81249999863440792, -5.148502694627439702 ) ) ;
#49111=ORIENTED_EDGE ( 'NONE', *, *, #47934, .T. ) ;
#49115=ORIENTED_EDGE ( 'NONE', *, *, #61459, .T. ) ;
#49118=ADVANCED_FACE ( 'NONE', ( #5881 ), #1075, .T. ) ;
#49119=CARTESIAN_POINT ( 'NONE',  ( 4.458734124999999437, -107.0624999986343937, -5.460374474430324690E-16 ) ) ;
#49124=CARTESIAN_POINT ( 'NONE',  ( 2.229367062500001939, -40.97916666530107221, 3.861377020970579999 ) ) ;
#49127=CARTESIAN_POINT ( 'NONE',  ( 2.500000000000002220, 29.33333333333333215, 4.330127018922192761 ) ) ;
#49128=CARTESIAN_POINT ( 'NONE',  ( 4.458734125000001214, -14.89583333196773474, 2.574251347313718519 ) ) ;
#49129=CARTESIAN_POINT ( 'NONE',  ( 9.457646018065525792E-16, -102.3124999986343937, 5.148502694627439702 ) ) ;
#49132=CARTESIAN_POINT ( 'NONE',  ( 4.458734124999998549, -33.97916666530107221, -2.574251347313721627 ) ) ;
#49133=CARTESIAN_POINT ( 'NONE',  ( 5.000000000000000000, 7.708333336064517205, -2.886751345948129988 ) ) ;
#49134=CARTESIAN_POINT ( 'NONE',  ( 1.975475456537005874E-15, 10.24999999999999822, 5.000000000000000000 ) ) ;
#49140=CARTESIAN_POINT ( 'NONE',  ( -2.229367062500000163, 4.270833334698926897, -3.861377020970580443 ) ) ;
#49141=VERTEX_POINT ( 'NONE', #40287 ) ;
#49143=CARTESIAN_POINT ( 'NONE',  ( 5.000000000000000000, -97.50000000000000000, -6.123233995736766282E-16 ) ) ;
#49144=CARTESIAN_POINT ( 'NONE',  ( 2.229367062499998831, -30.64583333196773651, -3.861377020970580887 ) ) ;
#49145=CARTESIAN_POINT ( 'NONE',  ( -1.339745962155610925, -35.79465819873851729, 5.000000000000000000 ) ) ;
#49146=CARTESIAN_POINT ( 'NONE',  ( -4.458734124999998549, -79.47916666530106511, 2.574251347313722516 ) ) ;
#49147=ADVANCED_FACE ( 'NONE', ( #56046 ), #1706, .T. ) ;
#49151=ADVANCED_FACE ( 'NONE', ( #21311 ), #59600, .T. ) ;
#49153=CARTESIAN_POINT ( 'NONE',  ( 4.458734124999999437, -2.812499998634407472, -5.460374474430324690E-16 ) ) ;
#49154=CARTESIAN_POINT ( 'NONE',  ( -4.458734124999998549, 22.52083333469892423, 2.574251347313722516 ) ) ;
#49155=CARTESIAN_POINT ( 'NONE',  ( -4.458734124999997661, -42.47916666530106511, 2.574251347313722516 ) ) ;
#49158=ORIENTED_EDGE ( 'NONE', *, *, #23584, .T. ) ;
#49160=VECTOR ( 'NONE', #9385, 1000.000000000000000 ) ;
#49161=CARTESIAN_POINT ( 'NONE',  ( 9.457646018065525792E-16, -71.06249999863440792, 5.148502694627439702 ) ) ;
#49162=CARTESIAN_POINT ( 'NONE',  ( -5.000000000000000000, -102.8749999972688158, 0.000000000000000000 ) ) ;
#49164=EDGE_CURVE ( 'NONE', #28144, #46456, #29164, .T. ) ;
#49165=( BOUNDED_CURVE ( )  B_SPLINE_CURVE ( 2, ( #26513, #6266, #51289, #50959, #11705, #45489, #6900, #26191, #60300 ),
 .UNSPECIFIED., .F., .F. ) 
 B_SPLINE_CURVE_WITH_KNOTS ( ( 3, 2, 2, 2, 3 ),
 ( 0.2625000000000000111, 0.2630952380952381042, 0.2642857142857142905, 0.2654761904761904767, 0.2660714285714285698 ),
 .UNSPECIFIED. ) 
 CURVE ( )  GEOMETRIC_REPRESENTATION_ITEM ( )  RATIONAL_B_SPLINE_CURVE ( ( 0.9330127018922194093, 0.9330127018922194093, 1.000000000000000000, 0.8660254037844387076, 1.000000000000000000, 0.8660254037844387076, 1.000000000000000000, 0.9330127018922194093, 0.9330127018922194093 ) ) 
 REPRESENTATION_ITEM ( '' )  );
#49168=EDGE_CURVE ( 'NONE', #20011, #14094, #26756, .T. ) ;
#49169=CARTESIAN_POINT ( 'NONE',  ( 4.458734124999998549, -108.9791666653010651, -2.574251347313721627 ) ) ;
#49171=CARTESIAN_POINT ( 'NONE',  ( -2.500000000000000444, -60.16666666666665719, -4.330127018922193649 ) ) ;
#49172=CYLINDRICAL_SURFACE ( 'NONE', #15148, 5.000000000000000000 ) ;
#49186=CARTESIAN_POINT ( 'NONE',  ( 2.499999999999998668, 5.666666666666666963, -4.330127018922193649 ) ) ;
#49193=CARTESIAN_POINT ( 'NONE',  ( -2.229367062499996610, -43.39583333196773651, 3.861377020970582219 ) ) ;
#49196=CARTESIAN_POINT ( 'NONE',  ( -1.339745962155613812, -57.08034179853028434, -5.000000000000000000 ) ) ;
#49202=CARTESIAN_POINT ( 'NONE',  ( -3.152548672688508926E-16, -86.81249999863439371, -5.148502694627439702 ) ) ;
#49203=CARTESIAN_POINT ( 'NONE',  ( 2.500000000000002220, -108.6666666666666572, 4.330127018922192761 ) ) ;
#49205=CARTESIAN_POINT ( 'NONE',  ( -2.499999999999996447, 14.29166666939785202, 4.330127018922195425 ) ) ;
#49208=( GEOMETRIC_REPRESENTATION_CONTEXT ( 3 ) GLOBAL_UNCERTAINTY_ASSIGNED_CONTEXT ( ( #57501 ) ) GLOBAL_UNIT_ASSIGNED_CONTEXT ( ( #53783, #43808, #24203 ) ) REPRESENTATION_CONTEXT ( 'NONE', 'WORKASPACE' ) );
#49209=CARTESIAN_POINT ( 'NONE',  ( 1.975475456537005874E-15, -82.62499999726878741, 5.000000000000000000 ) ) ;
#49210=VECTOR ( 'NONE', #29890, 1000.000000000000000 ) ;
#49212=CARTESIAN_POINT ( 'NONE',  ( -3.152548672688508926E-16, 1.437500001365596525, -5.148502694627439702 ) ) ;
#49213=CARTESIAN_POINT ( 'NONE',  ( 1.975475456537005874E-15, -13.75000000000000000, 5.000000000000000000 ) ) ;
#49214=CARTESIAN_POINT ( 'NONE',  ( 2.229367062500001939, -15.22916666530107399, 3.861377020970579999 ) ) ;
#49218=CARTESIAN_POINT ( 'NONE',  ( -4.458734124999999437, 23.43750000136559564, 0.000000000000000000 ) ) ;
#49220=CARTESIAN_POINT ( 'NONE',  ( 9.457646018065525792E-16, -96.06249999863439371, 5.148502694627439702 ) ) ;
#49221=CARTESIAN_POINT ( 'NONE',  ( -5.000000000000000000, -33.95833333060213732, -2.886751345948128211 ) ) ;
#49223=CARTESIAN_POINT ( 'NONE',  ( -4.458734124999998549, -12.22916666530106866, 2.574251347313722516 ) ) ;
#49224=CARTESIAN_POINT ( 'NONE',  ( 1.339745962155612702, -39.16965819600733312, -5.000000000000000000 ) ) ;
#49228=CARTESIAN_POINT ( 'NONE',  ( 5.000000000000000000, -40.37499999726880162, -6.123233995736766282E-16 ) ) ;
#49230=CARTESIAN_POINT ( 'NONE',  ( 9.457646018065525792E-16, 11.93750000136559564, 5.148502694627439702 ) ) ;
#49233=CARTESIAN_POINT ( 'NONE',  ( 2.229367062500001939, -63.97916666530106511, 3.861377020970579999 ) ) ;
#49236=( BOUNDED_CURVE ( )  B_SPLINE_CURVE ( 2, ( #20533, #40131, #59772, #29514, #34038, #49784, #25671, #50104, #15699 ),
 .UNSPECIFIED., .F., .F. ) 
 B_SPLINE_CURVE_WITH_KNOTS ( ( 3, 2, 2, 2, 3 ),
 ( 0.2803571428571428603, 0.2809523809523809534, 0.2821428571428571397, 0.2833333333333333259, 0.2839285714285714191 ),
 .UNSPECIFIED. ) 
 CURVE ( )  GEOMETRIC_REPRESENTATION_ITEM ( )  RATIONAL_B_SPLINE_CURVE ( ( 0.9330127018922194093, 0.9330127018922194093, 1.000000000000000000, 0.8660254037844387076, 1.000000000000000000, 0.8660254037844387076, 1.000000000000000000, 0.9330127018922194093, 0.9330127018922194093 ) ) 
 REPRESENTATION_ITEM ( '' )  );
#49237=CARTESIAN_POINT ( 'NONE',  ( 2.499999999999998668, 6.666666666666667851, -4.330127018922193649 ) ) ;
#49240=CARTESIAN_POINT ( 'NONE',  ( 4.458734124999998549, -51.72916666530107221, -2.574251347313721627 ) ) ;
#49241=CARTESIAN_POINT ( 'NONE',  ( -2.499999999999996447, -90.70833333060214443, 4.330127018922195425 ) ) ;
#49242=CARTESIAN_POINT ( 'NONE',  ( 9.457646018065525792E-16, -34.06249999863440792, 5.148502694627439702 ) ) ;
#49244=CARTESIAN_POINT ( 'NONE',  ( 1.975475456537005874E-15, 20.37500000273118417, 5.000000000000000000 ) ) ;
#49248=CARTESIAN_POINT ( 'NONE',  ( 1.060575238724906964E-15, -42.75000000000000000, 5.773502691896257311 ) ) ;
#49249=CARTESIAN_POINT ( 'NONE',  ( 0.000000000000000000, -120.0000000000000000, 0.000000000000000000 ) ) ;
#49250=EDGE_CURVE ( 'NONE', #28956, #54753, #18107, .T. ) ;
#49252=ORIENTED_EDGE ( 'NONE', *, *, #16412, .T. ) ;
#49253=CARTESIAN_POINT ( 'NONE',  ( 4.458734124999999437, -101.8124999986344079, -5.460374474430324690E-16 ) ) ;
#49254=CARTESIAN_POINT ( 'NONE',  ( 4.458734124999998549, 2.020833334698927786, -2.574251347313721627 ) ) ;
#49262=EDGE_CURVE ( 'NONE', #59301, #61600, #6648, .T. ) ;
#49267=DIRECTION ( 'NONE',  ( 0.000000000000000000, 0.000000000000000000, 1.000000000000000000 ) ) ;
#49269=CARTESIAN_POINT ( 'NONE',  ( 5.000000000000000888, -20.58333333333333215, 2.886751345948126879 ) ) ;
#49271=( BOUNDED_CURVE ( )  B_SPLINE_CURVE ( 2, ( #39282, #4559, #44427, #387, #13901, #53143, #39598, #28995, #48307 ),
 .UNSPECIFIED., .F., .F. ) 
 B_SPLINE_CURVE_WITH_KNOTS ( ( 3, 2, 2, 2, 3 ),
 ( 0.2910714285714285920, 0.2916666666666666852, 0.2928571428571428714, 0.2940476190476190577, 0.2946428571428571508 ),
 .UNSPECIFIED. ) 
 CURVE ( )  GEOMETRIC_REPRESENTATION_ITEM ( )  RATIONAL_B_SPLINE_CURVE ( ( 0.9330127018922194093, 0.9330127018922194093, 1.000000000000000000, 0.8660254037844387076, 1.000000000000000000, 0.8660254037844387076, 1.000000000000000000, 0.9330127018922194093, 0.9330127018922194093 ) ) 
 REPRESENTATION_ITEM ( '' )  );
#49272=DIRECTION ( 'NONE',  ( -0.000000000000000000, 1.000000000000000000, -0.000000000000000000 ) ) ;
#49273=CARTESIAN_POINT ( 'NONE',  ( -2.229367062500000163, -23.72916666530107577, -3.861377020970580443 ) ) ;
#49280=ORIENTED_EDGE ( 'NONE', *, *, #40160, .F. ) ;
#49281=ORIENTED_EDGE ( 'NONE', *, *, #49683, .F. ) ;
#49282=CARTESIAN_POINT ( 'NONE',  ( 9.457646018065525792E-16, -72.31249999863440792, 5.148502694627439702 ) ) ;
#49283=LINE ( 'NONE', #90, #10186 ) ;
#49285=DIRECTION ( 'NONE',  ( -1.000000000000000000, 0.000000000000000000, 3.614007241618347908E-17 ) ) ;
#49287=CARTESIAN_POINT ( 'NONE',  ( 2.500000000000002220, -31.54166666393548724, 4.330127018922192761 ) ) ;
#49289=CARTESIAN_POINT ( 'NONE',  ( -3.152548672688508926E-16, -2.812499998634407028, -5.148502694627439702 ) ) ;
#49291=CARTESIAN_POINT ( 'NONE',  ( -6.972266317189433020E-16, -20.24999999999999289, -5.000000000000000000 ) ) ;
#49298=CARTESIAN_POINT ( 'NONE',  ( 4.458734124999998549, -81.72916666530106511, -2.574251347313721627 ) ) ;
#49300=CARTESIAN_POINT ( 'NONE',  ( -2.229367062500000163, -0.4791666653010707710, -3.861377020970580443 ) ) ;
#49301=CARTESIAN_POINT ( 'NONE',  ( -5.000000000000000000, -86.00000000000000000, 0.000000000000000000 ) ) ;
#49303=CARTESIAN_POINT ( 'NONE',  ( 2.229367062499998831, -66.89583333196773651, -3.861377020970580887 ) ) ;
#49304=CARTESIAN_POINT ( 'NONE',  ( 1.060575238724906964E-15, -23.62499999726881228, 5.773502691896257311 ) ) ;
#49306=CARTESIAN_POINT ( 'NONE',  ( -3.152548672688508926E-16, 27.43750000136559564, -5.148502694627439702 ) ) ;
#49307=CARTESIAN_POINT ( 'NONE',  ( 5.000000000000000000, -49.41666666666666430, -2.886751345948130876 ) ) ;
#49308=CARTESIAN_POINT ( 'NONE',  ( -4.458734124999999437, -45.31249999863440081, 0.000000000000000000 ) ) ;
#49309=CARTESIAN_POINT ( 'NONE',  ( 2.229367062500001939, -33.22916666530106511, 3.861377020970579999 ) ) ;
#49311=DIRECTION ( 'NONE',  ( -0.000000000000000000, 1.000000000000000000, -0.000000000000000000 ) ) ;
#49312=CARTESIAN_POINT ( 'NONE',  ( 2.499999999999998668, 21.66666666666666785, -4.330127018922193649 ) ) ;
#49315=CARTESIAN_POINT ( 'NONE',  ( -2.229367062499996610, -37.14583333196773651, 3.861377020970582219 ) ) ;
#49316=CARTESIAN_POINT ( 'NONE',  ( -5.000000000000000000, -75.87499999726880162, 0.000000000000000000 ) ) ;
#49320=CARTESIAN_POINT ( 'NONE',  ( -2.229367062500000163, -80.72916666530106511, -3.861377020970580443 ) ) ;
#49323=CARTESIAN_POINT ( 'NONE',  ( 2.499999999999998668, 18.79166666939785202, -4.330127018922193649 ) ) ;
#49325=CARTESIAN_POINT ( 'NONE',  ( 2.499999999999998668, -23.33333333333333215, -4.330127018922193649 ) ) ;
#49329=ORIENTED_EDGE ( 'NONE', *, *, #22300, .T. ) ;
#49331=CARTESIAN_POINT ( 'NONE',  ( -2.500000000000000444, 19.95833333606451987, -4.330127018922193649 ) ) ;
#49338=CARTESIAN_POINT ( 'NONE',  ( -2.499999999999996447, 0.1666666666666656582, 4.330127018922195425 ) ) ;
#49340=CARTESIAN_POINT ( 'NONE',  ( 6.123233995736766282E-16, -120.0000000000000000, -5.000000000000000000 ) ) ;
#49341=CARTESIAN_POINT ( 'NONE',  ( 2.229367062499998831, -21.64583333196774007, -3.861377020970580887 ) ) ;
#49342=CARTESIAN_POINT ( 'NONE',  ( 1.975475456537005874E-15, -97.62499999726880162, 5.000000000000000000 ) ) ;
#49345=VECTOR ( 'NONE', #59707, 1000.000000000000000 ) ;
#49347=ORIENTED_EDGE ( 'NONE', *, *, #37350, .F. ) ;
#49350=ORIENTED_EDGE ( 'NONE', *, *, #7490, .T. ) ;
#49351=CARTESIAN_POINT ( 'NONE',  ( 0.000000000000000000, -120.0000000000000000, 0.000000000000000000 ) ) ;
#49354=VERTEX_POINT ( 'NONE', #32535 ) ;
#49355=CARTESIAN_POINT ( 'NONE',  ( -6.972266317189433020E-16, -23.12499999726880873, -5.000000000000000000 ) ) ;
#49359=VERTEX_POINT ( 'NONE', #17115 ) ;
#49360=( BOUNDED_CURVE ( )  B_SPLINE_CURVE ( 2, ( #55555, #1523, #30446, #50394, #20173, #11467, #6030, #25313, #15665 ),
 .UNSPECIFIED., .F., .F. ) 
 B_SPLINE_CURVE_WITH_KNOTS ( ( 3, 2, 2, 2, 3 ),
 ( 0.8125000000000000000, 0.8130952380952380931, 0.8142857142857142794, 0.8154761904761904656, 0.8160714285714285587 ),
 .UNSPECIFIED. ) 
 CURVE ( )  GEOMETRIC_REPRESENTATION_ITEM ( )  RATIONAL_B_SPLINE_CURVE ( ( 0.9330127018922194093, 0.9330127018922194093, 1.000000000000000000, 0.8660254037844387076, 1.000000000000000000, 0.8660254037844387076, 1.000000000000000000, 0.9330127018922194093, 0.9330127018922194093 ) ) 
 REPRESENTATION_ITEM ( '' )  );
#49362=CARTESIAN_POINT ( 'NONE',  ( 2.229367062500001939, 12.02083333469892601, 3.861377020970579999 ) ) ;
#49363=CARTESIAN_POINT ( 'NONE',  ( -5.000000000000000000, -9.874999997268815832, 0.000000000000000000 ) ) ;
#49364=ORIENTED_EDGE ( 'NONE', *, *, #3325, .F. ) ;
#49367=CARTESIAN_POINT ( 'NONE',  ( 1.339745962155612702, -44.29465819873851729, -5.000000000000000000 ) ) ;
#49368=LINE ( 'NONE', #9487, #29501 ) ;
#49370=CARTESIAN_POINT ( 'NONE',  ( 2.229367062500001939, -64.97916666530106511, 3.861377020970579999 ) ) ;
#49372=CARTESIAN_POINT ( 'NONE',  ( 9.457646018065525792E-16, 19.93750000136559208, 5.148502694627439702 ) ) ;
#49374=CARTESIAN_POINT ( 'NONE',  ( 9.457646018065525792E-16, -49.31249999863441502, 5.148502694627439702 ) ) ;
#49375=CARTESIAN_POINT ( 'NONE',  ( -4.999999999999999112, -6.791666663935481907, 2.886751345948131764 ) ) ;
#49377=DIRECTION ( 'NONE',  ( 0.000000000000000000, -1.000000000000000000, 0.000000000000000000 ) ) ;
#49379=CARTESIAN_POINT ( 'NONE',  ( -4.458734124999999437, -107.3124999986343937, 0.000000000000000000 ) ) ;
#49382=CARTESIAN_POINT ( 'NONE',  ( -4.458734124999997661, -14.47916666530107221, 2.574251347313722516 ) ) ;
#49385=CARTESIAN_POINT ( 'NONE',  ( 2.229367062499998831, -99.64583333196773651, -3.861377020970580887 ) ) ;
#49387=CARTESIAN_POINT ( 'NONE',  ( 4.458734124999998549, -94.97916666530106511, -2.574251347313721627 ) ) ;
#49390=CARTESIAN_POINT ( 'NONE',  ( -5.000000000000000000, -59.95833333060215153, -2.886751345948128211 ) ) ;
#49391=CARTESIAN_POINT ( 'NONE',  ( 0.000000000000000000, -120.0000000000000000, 0.000000000000000000 ) ) ;
#49394=CARTESIAN_POINT ( 'NONE',  ( -4.458734124999999437, -17.39583333196773651, -2.574251347313719407 ) ) ;
#49395=CARTESIAN_POINT ( 'NONE',  ( -4.458734124999998549, 6.520833334698930450, 2.574251347313722516 ) ) ;
#49396=CARTESIAN_POINT ( 'NONE',  ( -4.458734124999999437, -56.56249999863440081, 0.000000000000000000 ) ) ;
#49399=CYLINDRICAL_SURFACE ( 'NONE', #16865, 5.000000000000000000 ) ;
#49401=CARTESIAN_POINT ( 'NONE',  ( 5.000000000000000000, -4.416666666666666075, -2.886751345948129988 ) ) ;
#49405=CARTESIAN_POINT ( 'NONE',  ( -2.499999999999996447, -8.833333333333332149, 4.330127018922195425 ) ) ;
#49407=CARTESIAN_POINT ( 'NONE',  ( 2.229367062499998831, -91.64583333196773651, -3.861377020970580887 ) ) ;
#49408=CARTESIAN_POINT ( 'NONE',  ( 4.458734124999998549, 21.02083333469892779, -2.574251347313721627 ) ) ;
#49410=CARTESIAN_POINT ( 'NONE',  ( -1.339745962155610925, -6.794658198738519062, 5.000000000000000000 ) ) ;
#49413=CARTESIAN_POINT ( 'NONE',  ( -3.535250795749689387E-16, -76.24999999999998579, -5.773502691896257311 ) ) ;
#49414=( BOUNDED_CURVE ( )  B_SPLINE_CURVE ( 2, ( #16942, #2791, #46210, #61333, #6659, #2172, #21778, #36555, #26266 ),
 .UNSPECIFIED., .F., .F. ) 
 B_SPLINE_CURVE_WITH_KNOTS ( ( 3, 2, 2, 2, 3 ),
 ( 0.3446428571428571397, 0.3452380952380952328, 0.3464285714285714191, 0.3476190476190476053, 0.3482142857142856984 ),
 .UNSPECIFIED. ) 
 CURVE ( )  GEOMETRIC_REPRESENTATION_ITEM ( )  RATIONAL_B_SPLINE_CURVE ( ( 0.9330127018922194093, 0.9330127018922194093, 1.000000000000000000, 0.8660254037844387076, 1.000000000000000000, 0.8660254037844387076, 1.000000000000000000, 0.9330127018922194093, 0.9330127018922194093 ) ) 
 REPRESENTATION_ITEM ( '' )  );
#49417=FACE_OUTER_BOUND ( 'NONE', #25121, .T. ) ;
#49419=CARTESIAN_POINT ( 'NONE',  ( -1.339745962155613812, -104.2053418012614827, -5.000000000000000000 ) ) ;
#49429=CARTESIAN_POINT ( 'NONE',  ( 9.457646018065525792E-16, -64.31249999863440792, 5.148502694627439702 ) ) ;
#49431=FACE_OUTER_BOUND ( 'NONE', #57272, .T. ) ;
#49437=DIRECTION ( 'NONE',  ( 0.000000000000000000, 0.000000000000000000, 1.000000000000000000 ) ) ;
#49441=CARTESIAN_POINT ( 'NONE',  ( -2.229367062500000163, -106.7291666653010651, -3.861377020970580443 ) ) ;
#49447=CARTESIAN_POINT ( 'NONE',  ( -2.229367062499996610, -46.14583333196774362, 3.861377020970582219 ) ) ;
#49451=CARTESIAN_POINT ( 'NONE',  ( 4.458734124999999437, -14.81249999863440436, -5.460374474430324690E-16 ) ) ;
#49452=CARTESIAN_POINT ( 'NONE',  ( 1.060575238724906964E-15, -101.7500000000000000, 5.773502691896257311 ) ) ;
#49456=CARTESIAN_POINT ( 'NONE',  ( -4.458734124999998549, -32.47916666530107221, 2.574251347313722516 ) ) ;
#49458=CARTESIAN_POINT ( 'NONE',  ( -3.535250795749689387E-16, 4.875000002731184168, -5.773502691896257311 ) ) ;
#49464=( BOUNDED_CURVE ( )  B_SPLINE_CURVE ( 2, ( #59918, #15839, #6513, #1066, #34820, #11319, #16473, #736, #40907 ),
 .UNSPECIFIED., .F., .F. ) 
 B_SPLINE_CURVE_WITH_KNOTS ( ( 3, 2, 2, 2, 3 ),
 ( 0.8660714285714286031, 0.8666666666666666963, 0.8678571428571428825, 0.8690476190476190688, 0.8696428571428571619 ),
 .UNSPECIFIED. ) 
 CURVE ( )  GEOMETRIC_REPRESENTATION_ITEM ( )  RATIONAL_B_SPLINE_CURVE ( ( 0.9330127018922194093, 0.9330127018922194093, 1.000000000000000000, 0.8660254037844387076, 1.000000000000000000, 0.8660254037844387076, 1.000000000000000000, 0.9330127018922194093, 0.9330127018922194093 ) ) 
 REPRESENTATION_ITEM ( '' )  );
#49465=CARTESIAN_POINT ( 'NONE',  ( 4.458734124999999437, 1.937500001365593416, -5.460374474430324690E-16 ) ) ;
#49468=CARTESIAN_POINT ( 'NONE',  ( -4.999999999999998224, -75.91666666666665719, 2.886751345948131764 ) ) ;
#49469=CARTESIAN_POINT ( 'NONE',  ( 5.000000000000000888, -98.58333333333332860, 2.886751345948126879 ) ) ;
#49470=CARTESIAN_POINT ( 'NONE',  ( 2.229367062499998831, -31.64583333196773651, -3.861377020970580887 ) ) ;
#49471=CARTESIAN_POINT ( 'NONE',  ( 1.975475456537005874E-15, -95.75000000000000000, 5.000000000000000000 ) ) ;
#49472=CARTESIAN_POINT ( 'NONE',  ( -4.458734124999998549, -81.47916666530106511, 2.574251347313722516 ) ) ;
#49477=CARTESIAN_POINT ( 'NONE',  ( 2.229367062499998831, -1.645833331967737401, -3.861377020970580887 ) ) ;
#49478=CARTESIAN_POINT ( 'NONE',  ( 2.229367062499998831, 24.10416666803225993, -3.861377020970580887 ) ) ;
#49479=CARTESIAN_POINT ( 'NONE',  ( -3.152548672688508926E-16, -42.81249999863440081, -5.148502694627439702 ) ) ;
#49480=CARTESIAN_POINT ( 'NONE',  ( 2.499999999999998668, -105.3333333333333286, -4.330127018922193649 ) ) ;
#49482=VERTEX_POINT ( 'NONE', #34411 ) ;
#49484=CARTESIAN_POINT ( 'NONE',  ( 4.458734125000001214, -67.89583333196773651, 2.574251347313718519 ) ) ;
#49485=CARTESIAN_POINT ( 'NONE',  ( -3.535250795749689387E-16, -107.1249999972687874, -5.773502691896257311 ) ) ;
#49487=ADVANCED_FACE ( 'NONE', ( #23836 ), #44065, .T. ) ;
#49490=CARTESIAN_POINT ( 'NONE',  ( 2.499999999999998668, -60.33333333333333570, -4.330127018922193649 ) ) ;
#49491=CARTESIAN_POINT ( 'NONE',  ( -1.339745962155610925, -65.79465819873851729, 5.000000000000000000 ) ) ;
#49495=CARTESIAN_POINT ( 'NONE',  ( 2.500000000000002220, -67.66666666666667140, 4.330127018922192761 ) ) ;
#49501=EDGE_LOOP ( 'NONE', ( #11463, #60622, #6192, #29 ) ) ;
#49505=ORIENTED_EDGE ( 'NONE', *, *, #52370, .F. ) ;
#49509=CARTESIAN_POINT ( 'NONE',  ( -2.229367062499996610, -41.39583333196773651, 3.861377020970582219 ) ) ;
#49510=CARTESIAN_POINT ( 'NONE',  ( -6.972266317189433020E-16, -16.12499999726881228, -5.000000000000000000 ) ) ;
#49512=DIRECTION ( 'NONE',  ( -0.000000000000000000, 1.000000000000000000, -0.000000000000000000 ) ) ;
#49514=EDGE_CURVE ( 'NONE', #21194, #27082, #35772, .T. ) ;
#49519=CARTESIAN_POINT ( 'NONE',  ( -4.458734124999998549, -90.47916666530106511, 2.574251347313722516 ) ) ;
#49525=CARTESIAN_POINT ( 'NONE',  ( 1.975475456537005874E-15, -38.75000000000000000, 5.000000000000000000 ) ) ;
#49527=CARTESIAN_POINT ( 'NONE',  ( 2.229367062499998831, 2.354166668032262599, -3.861377020970580887 ) ) ;
#49528=DIRECTION ( 'NONE',  ( -0.000000000000000000, 1.000000000000000000, -0.000000000000000000 ) ) ;
#49529=CARTESIAN_POINT ( 'NONE',  ( -2.229367062500000163, -17.72916666530106866, -3.861377020970580443 ) ) ;
#49533=CARTESIAN_POINT ( 'NONE',  ( 2.499999999999998668, -55.20833333060214443, -4.330127018922193649 ) ) ;
#49535=CARTESIAN_POINT ( 'NONE',  ( -2.229367062500000163, 23.27083333469892779, -3.861377020970580443 ) ) ;
#49537=CARTESIAN_POINT ( 'NONE',  ( -2.229367062500000163, -96.47916666530105090, -3.861377020970580443 ) ) ;
#49539=CARTESIAN_POINT ( 'NONE',  ( 2.499999999999998668, -57.20833333060214443, -4.330127018922193649 ) ) ;
#49540=CARTESIAN_POINT ( 'NONE',  ( 2.229367062500001939, -14.97916666530107399, 3.861377020970579999 ) ) ;
#49541=CARTESIAN_POINT ( 'NONE',  ( 0.000000000000000000, -120.0000000000000000, 0.000000000000000000 ) ) ;
#49542=CARTESIAN_POINT ( 'NONE',  ( 0.000000000000000000, -120.0000000000000000, 0.000000000000000000 ) ) ;
#49543=( BOUNDED_CURVE ( )  B_SPLINE_CURVE ( 2, ( #54258, #25309, #24357, #58459, #9560, #63605, #20169, #58766, #24044 ),
 .UNSPECIFIED., .F., .F. ) 
 B_SPLINE_CURVE_WITH_KNOTS ( ( 3, 2, 2, 2, 3 ),
 ( 0.1803571428571428548, 0.1809523809523809479, 0.1821428571428571341, 0.1833333333333333204, 0.1839285714285714413 ),
 .UNSPECIFIED. ) 
 CURVE ( )  GEOMETRIC_REPRESENTATION_ITEM ( )  RATIONAL_B_SPLINE_CURVE ( ( 0.9330127018922194093, 0.9330127018922194093, 1.000000000000000000, 0.8660254037844387076, 1.000000000000000000, 0.8660254037844387076, 1.000000000000000000, 0.9330127018922178550, 0.9330127018922194093 ) ) 
 REPRESENTATION_ITEM ( '' )  );
#49545=CARTESIAN_POINT ( 'NONE',  ( 5.000000000000000000, -41.37499999726880162, -6.123233995736766282E-16 ) ) ;
#49546=CARTESIAN_POINT ( 'NONE',  ( -4.458734124999999437, 11.68750000136559564, 0.000000000000000000 ) ) ;
#49547=CARTESIAN_POINT ( 'NONE',  ( 3.044556291839386294E-14, 11.87500000273118417, -5.000000000000000000 ) ) ;
#49550=CARTESIAN_POINT ( 'NONE',  ( 4.458734125000001214, -59.89583333196774362, 2.574251347313718519 ) ) ;
#49551=ORIENTED_EDGE ( 'NONE', *, *, #62637, .F. ) ;
#49553=CARTESIAN_POINT ( 'NONE',  ( -2.499999999999996447, 6.166666666666667851, 4.330127018922195425 ) ) ;
#49555=CARTESIAN_POINT ( 'NONE',  ( -1.339745962155610925, -59.66965819600732601, 5.000000000000000000 ) ) ;
#49556=CARTESIAN_POINT ( 'NONE',  ( 9.457646018065525792E-16, -55.06249999863439371, 5.148502694627439702 ) ) ;
#49557=CARTESIAN_POINT ( 'NONE',  ( -2.500000000000000444, -87.04166666393547303, -4.330127018922193649 ) ) ;
#49558=EDGE_CURVE ( 'NONE', #33932, #4271, #9086, .T. ) ;
#49559=CARTESIAN_POINT ( 'NONE',  ( 2.229367062500001939, -33.97916666530107221, 3.861377020970579999 ) ) ;
#49560=CYLINDRICAL_SURFACE ( 'NONE', #12403, 5.000000000000000000 ) ;
#49561=( BOUNDED_CURVE ( )  B_SPLINE_CURVE ( 2, ( #38493, #5599, #17935, #4104, #24026, #23411, #13743, #30031, #33364 ),
 .UNSPECIFIED., .F., .F. ) 
 B_SPLINE_CURVE_WITH_KNOTS ( ( 3, 2, 2, 2, 3 ),
 ( 0.7767857142857143016, 0.7773809523809523947, 0.7785714285714285809, 0.7797619047619047672, 0.7803571428571428603 ),
 .UNSPECIFIED. ) 
 CURVE ( )  GEOMETRIC_REPRESENTATION_ITEM ( )  RATIONAL_B_SPLINE_CURVE ( ( 0.9330127018922194093, 0.9330127018922194093, 1.000000000000000000, 0.8660254037844387076, 1.000000000000000000, 0.8660254037844387076, 1.000000000000000000, 0.9330127018922194093, 0.9330127018922194093 ) ) 
 REPRESENTATION_ITEM ( '' )  );
#49565=CARTESIAN_POINT ( 'NONE',  ( -2.499999999999996447, -40.83333333333333570, 4.330127018922195425 ) ) ;
#49566=CARTESIAN_POINT ( 'NONE',  ( 2.500000000000002220, -86.54166666393547303, 4.330127018922192761 ) ) ;
#49567=ORIENTED_EDGE ( 'NONE', *, *, #22999, .F. ) ;
#49568=CARTESIAN_POINT ( 'NONE',  ( 2.229367062500001939, -100.9791666653010651, 3.861377020970579999 ) ) ;
#49569=CARTESIAN_POINT ( 'NONE',  ( 4.458734124999999437, 1.937500001365593416, -5.460374474430324690E-16 ) ) ;
#49570=CARTESIAN_POINT ( 'NONE',  ( 5.000000000000000000, -59.50000000000000000, -6.123233995736766282E-16 ) ) ;
#49578=FACE_OUTER_BOUND ( 'NONE', #14467, .T. ) ;
#49580=CARTESIAN_POINT ( 'NONE',  ( 1.464175926609780648E-14, 24.74999999999999645, -5.000000000000000000 ) ) ;
#49582=DIRECTION ( 'NONE',  ( 0.000000000000000000, 0.000000000000000000, 1.000000000000000000 ) ) ;
#49583=CARTESIAN_POINT ( 'NONE',  ( -4.458734124999999437, -27.56249999863440081, 0.000000000000000000 ) ) ;
#49594=CARTESIAN_POINT ( 'NONE',  ( 5.000000000000000000, -20.29166666393548368, -2.886751345948130876 ) ) ;
#49596=CARTESIAN_POINT ( 'NONE',  ( 9.457646018065525792E-16, -73.31249999863440792, 5.148502694627439702 ) ) ;
#49597=CARTESIAN_POINT ( 'NONE',  ( 1.975475456537005874E-15, -14.62499999726881228, 5.000000000000000000 ) ) ;
#49599=VERTEX_POINT ( 'NONE', #45673 ) ;
#49600=EDGE_CURVE ( 'NONE', #36859, #969, #35018, .T. ) ;
#49604=CARTESIAN_POINT ( 'NONE',  ( 4.458734124999998549, -5.979166665301073103, -2.574251347313721627 ) ) ;
#49605=ORIENTED_EDGE ( 'NONE', *, *, #23885, .T. ) ;
#49607=CARTESIAN_POINT ( 'NONE',  ( 0.000000000000000000, -120.0000000000000000, 0.000000000000000000 ) ) ;
#49609=EDGE_CURVE ( 'NONE', #8886, #43978, #6758, .T. ) ;
#49614=( BOUNDED_CURVE ( )  B_SPLINE_CURVE ( 2, ( #3715, #38725, #23331, #53536, #8533, #23949, #42936, #43863, #29378 ),
 .UNSPECIFIED., .F., .F. ) 
 B_SPLINE_CURVE_WITH_KNOTS ( ( 3, 2, 2, 2, 3 ),
 ( 0.3017857142857142683, 0.3023809523809523614, 0.3035714285714285476, 0.3047619047619047894, 0.3053571428571428825 ),
 .UNSPECIFIED. ) 
 CURVE ( )  GEOMETRIC_REPRESENTATION_ITEM ( )  RATIONAL_B_SPLINE_CURVE ( ( 0.9330127018922194093, 0.9330127018922194093, 1.000000000000000000, 0.8660254037844387076, 1.000000000000000000, 0.8660254037844387076, 1.000000000000000000, 0.9330127018922194093, 0.9330127018922194093 ) ) 
 REPRESENTATION_ITEM ( '' )  );
#49617=ADVANCED_FACE ( 'NONE', ( #5479 ), #45989, .T. ) ;
#49618=CARTESIAN_POINT ( 'NONE',  ( 2.229367062499998831, -83.64583333196773651, -3.861377020970580887 ) ) ;
#49621=CARTESIAN_POINT ( 'NONE',  ( 9.457646018065525792E-16, 3.937500001365595192, 5.148502694627439702 ) ) ;
#49622=CARTESIAN_POINT ( 'NONE',  ( 5.000000000000000888, -83.58333333333332860, 2.886751345948126879 ) ) ;
#49624=CARTESIAN_POINT ( 'NONE',  ( -4.458734124999999437, -66.56249999863440792, 0.000000000000000000 ) ) ;
#49625=CARTESIAN_POINT ( 'NONE',  ( 2.499999999999998668, -23.20833333060214443, -4.330127018922193649 ) ) ;
#49627=CARTESIAN_POINT ( 'NONE',  ( 4.458734124999999437, 27.18750000136559564, -5.460374474430324690E-16 ) ) ;
#49628=CARTESIAN_POINT ( 'NONE',  ( 1.975475456537005874E-15, -11.74999999999999645, 5.000000000000000000 ) ) ;
#49630=CARTESIAN_POINT ( 'NONE',  ( -4.458734124999998549, -45.22916666530106511, 2.574251347313722516 ) ) ;
#49631=CARTESIAN_POINT ( 'NONE',  ( -3.152548672688508926E-16, -30.81249999863440436, -5.148502694627439702 ) ) ;
#49633=CARTESIAN_POINT ( 'NONE',  ( 2.500000000000002220, 18.33333333333333215, 4.330127018922192761 ) ) ;
#49635=CARTESIAN_POINT ( 'NONE',  ( 1.975475456537005874E-15, -54.62499999726880873, 5.000000000000000000 ) ) ;
#49636=CARTESIAN_POINT ( 'NONE',  ( -2.229367062499996610, -38.14583333196773651, 3.861377020970582219 ) ) ;
#49637=CARTESIAN_POINT ( 'NONE',  ( -2.500000000000000444, -75.04166666393547303, -4.330127018922193649 ) ) ;
#49640=LINE ( 'NONE', #5577, #5934 ) ;
#49641=CARTESIAN_POINT ( 'NONE',  ( 4.458734124999998549, -80.97916666530106511, -2.574251347313721627 ) ) ;
#49645=CARTESIAN_POINT ( 'NONE',  ( -2.499999999999996447, -28.83333333333333570, 4.330127018922195425 ) ) ;
#49649=ORIENTED_EDGE ( 'NONE', *, *, #12582, .F. ) ;
#49652=CARTESIAN_POINT ( 'NONE',  ( 1.060575238724906964E-15, 23.37500000273118062, 5.773502691896257311 ) ) ;
#49663=CARTESIAN_POINT ( 'NONE',  ( -2.229367062500000163, -23.47916666530107221, -3.861377020970580443 ) ) ;
#49664=CARTESIAN_POINT ( 'NONE',  ( 3.044556291839386294E-14, 17.87500000273118417, -5.000000000000000000 ) ) ;
#49668=ORIENTED_EDGE ( 'NONE', *, *, #5962, .F. ) ;
#49669=DIRECTION ( 'NONE',  ( -0.000000000000000000, 1.000000000000000000, -0.000000000000000000 ) ) ;
#49671=ORIENTED_EDGE ( 'NONE', *, *, #51246, .F. ) ;
#49672=CARTESIAN_POINT ( 'NONE',  ( -2.499999999999996447, -27.83333333333333570, 4.330127018922195425 ) ) ;
#49673=DIRECTION ( 'NONE',  ( -0.000000000000000000, 1.000000000000000000, -0.000000000000000000 ) ) ;
#49675=ORIENTED_EDGE ( 'NONE', *, *, #6440, .T. ) ;
#49678=CARTESIAN_POINT ( 'NONE',  ( 5.000000000000000000, -86.50000000000000000, -6.123233995736766282E-16 ) ) ;
#49680=ORIENTED_EDGE ( 'NONE', *, *, #58177, .F. ) ;
#49682=CARTESIAN_POINT ( 'NONE',  ( 2.229367062499998831, 16.35416666803225993, -3.861377020970580887 ) ) ;
#49683=EDGE_CURVE ( 'NONE', #49750, #48396, #55503, .T. ) ;
#49686=CARTESIAN_POINT ( 'NONE',  ( 1.975475456537005874E-15, -44.74999999999999289, 5.000000000000000000 ) ) ;
#49688=CARTESIAN_POINT ( 'NONE',  ( 2.229367062500001939, -66.97916666530106511, 3.861377020970579999 ) ) ;
#49690=CARTESIAN_POINT ( 'NONE',  ( 4.458734124999999437, 17.18750000136559564, -5.460374474430324690E-16 ) ) ;
#49693=CARTESIAN_POINT ( 'NONE',  ( -2.229367062500000163, -48.72916666530106511, -3.861377020970580443 ) ) ;
#49694=CARTESIAN_POINT ( 'NONE',  ( 2.500000000000002220, -10.54166666393547835, 4.330127018922192761 ) ) ;
#49697=CARTESIAN_POINT ( 'NONE',  ( 0.000000000000000000, -120.0000000000000000, 0.000000000000000000 ) ) ;
#49699=CARTESIAN_POINT ( 'NONE',  ( -2.229367062499996610, -18.39583333196774007, 3.861377020970582219 ) ) ;
#49702=CARTESIAN_POINT ( 'NONE',  ( -4.458734124999998549, -101.2291666653010651, 2.574251347313722516 ) ) ;
#49704=ORIENTED_EDGE ( 'NONE', *, *, #21742, .T. ) ;
#49705=CARTESIAN_POINT ( 'NONE',  ( 2.229367062499998831, -96.89583333196773651, -3.861377020970580887 ) ) ;
#49707=CARTESIAN_POINT ( 'NONE',  ( -2.499999999999996447, -59.70833333060214443, 4.330127018922195425 ) ) ;
#49708=CYLINDRICAL_SURFACE ( 'NONE', #28416, 5.000000000000000000 ) ;
#49711=CARTESIAN_POINT ( 'NONE',  ( 2.229367062500001939, -18.97916666530106866, 3.861377020970579999 ) ) ;
#49712=CARTESIAN_POINT ( 'NONE',  ( 4.458734124999998549, 7.020833334698929562, -2.574251347313721627 ) ) ;
#49713=CARTESIAN_POINT ( 'NONE',  ( 4.458734124999998549, -64.97916666530106511, -2.574251347313721627 ) ) ;
#49716=FACE_OUTER_BOUND ( 'NONE', #60452, .T. ) ;
#49718=CARTESIAN_POINT ( 'NONE',  ( 2.500000000000002220, -10.66666666666666430, 4.330127018922192761 ) ) ;
#49722=CARTESIAN_POINT ( 'NONE',  ( 1.339745962155608039, 21.41965820146970501, 5.000000000000003553 ) ) ;
#49725=CARTESIAN_POINT ( 'NONE',  ( -2.229367062499996610, -92.14583333196773651, 3.861377020970582219 ) ) ;
#49728=CARTESIAN_POINT ( 'NONE',  ( -6.972266317189433020E-16, -0.2500000000000001665, -5.000000000000000000 ) ) ;
#49730=CARTESIAN_POINT ( 'NONE',  ( 1.975475456537005874E-15, -26.74999999999999645, 5.000000000000000000 ) ) ;
#49732=CARTESIAN_POINT ( 'NONE',  ( 5.000000000000000000, -76.50000000000000000, -6.123233995736766282E-16 ) ) ;
#49734=ORIENTED_EDGE ( 'NONE', *, *, #10698, .F. ) ;
#49735=CARTESIAN_POINT ( 'NONE',  ( -2.500000000000000444, -98.16666666666665719, -4.330127018922193649 ) ) ;
#49737=CARTESIAN_POINT ( 'NONE',  ( -2.500000000000000444, -51.16666666666666430, -4.330127018922193649 ) ) ;
#49741=ORIENTED_EDGE ( 'NONE', *, *, #62832, .T. ) ;
#49744=ORIENTED_EDGE ( 'NONE', *, *, #15425, .T. ) ;
#49747=CARTESIAN_POINT ( 'NONE',  ( -2.229367062499996610, -60.39583333196774362, 3.861377020970582219 ) ) ;
#49750=VERTEX_POINT ( 'NONE', #32139 ) ;
#49756=CARTESIAN_POINT ( 'NONE',  ( -3.152548672688508926E-16, 29.43750000136559564, -5.148502694627439702 ) ) ;
#49758=VERTEX_POINT ( 'NONE', #8030 ) ;
#49762=CARTESIAN_POINT ( 'NONE',  ( -2.229367062500000163, -46.47916666530106511, -3.861377020970580443 ) ) ;
#49765=CARTESIAN_POINT ( 'NONE',  ( 4.458734124999998549, -46.72916666530106511, -2.574251347313721627 ) ) ;
#49767=CARTESIAN_POINT ( 'NONE',  ( -3.152548672688508926E-16, -15.56249999863440614, -5.148502694627439702 ) ) ;
#49768=CARTESIAN_POINT ( 'NONE',  ( -4.999999999999999112, -101.9166666666666572, 2.886751345948131764 ) ) ;
#49770=CARTESIAN_POINT ( 'NONE',  ( -4.458734124999998549, -31.47916666530107221, 2.574251347313722516 ) ) ;
#49771=CARTESIAN_POINT ( 'NONE',  ( -2.499999999999996447, 8.291666669397852019, 4.330127018922195425 ) ) ;
#49777=DIRECTION ( 'NONE',  ( 0.000000000000000000, 0.000000000000000000, 1.000000000000000000 ) ) ;
#49778=CARTESIAN_POINT ( 'NONE',  ( -2.229367062500000163, 2.270833334698928230, -3.861377020970580443 ) ) ;
#49782=CARTESIAN_POINT ( 'NONE',  ( 9.457646018065525792E-16, -87.06249999863440792, 5.148502694627439702 ) ) ;
#49783=CARTESIAN_POINT ( 'NONE',  ( 9.457646018065525792E-16, -35.06249999863440792, 5.148502694627439702 ) ) ;
#49784=CARTESIAN_POINT ( 'NONE',  ( 5.000000000000000888, -9.583333333333332149, 2.886751345948126879 ) ) ;
#49785=CARTESIAN_POINT ( 'NONE',  ( -3.152548672688508926E-16, -80.81249999863440792, -5.148502694627439702 ) ) ;
#49787=CARTESIAN_POINT ( 'NONE',  ( -2.499999999999996447, -52.83333333333332860, 4.330127018922195425 ) ) ;
#49789=CARTESIAN_POINT ( 'NONE',  ( -4.458734124999999437, -0.3958333319677397322, -2.574251347313719407 ) ) ;
#49790=CARTESIAN_POINT ( 'NONE',  ( 2.229367062500001939, 19.77083333469892779, 3.861377020970579999 ) ) ;
#49791=CARTESIAN_POINT ( 'NONE',  ( 9.457646018065525792E-16, -46.31249999863440792, 5.148502694627439702 ) ) ;
#49792=( BOUNDED_CURVE ( )  B_SPLINE_CURVE ( 2, ( #17804, #2704, #41925, #32596, #51907, #62199, #18117, #38056, #37741 ),
 .UNSPECIFIED., .F., .F. ) 
 B_SPLINE_CURVE_WITH_KNOTS ( ( 3, 2, 2, 2, 3 ),
 ( 0.2589285714285714524, 0.2595238095238095455, 0.2607142857142857317, 0.2619047619047619180, 0.2625000000000000111 ),
 .UNSPECIFIED. ) 
 CURVE ( )  GEOMETRIC_REPRESENTATION_ITEM ( )  RATIONAL_B_SPLINE_CURVE ( ( 0.9330127018922194093, 0.9330127018922194093, 1.000000000000000000, 0.8660254037844387076, 1.000000000000000000, 0.8660254037844387076, 1.000000000000000000, 0.9330127018922194093, 0.9330127018922194093 ) ) 
 REPRESENTATION_ITEM ( '' )  );
#49793=CYLINDRICAL_SURFACE ( 'NONE', #46941, 5.000000000000000000 ) ;
#49798=CARTESIAN_POINT ( 'NONE',  ( 4.458734124999999437, -75.81249999863440792, -5.460374474430324690E-16 ) ) ;
#49799=CARTESIAN_POINT ( 'NONE',  ( 5.000000000000000000, -106.2916666639354730, -2.886751345948129988 ) ) ;
#49800=ADVANCED_FACE ( 'NONE', ( #41468 ), #61434, .T. ) ;
#49804=CARTESIAN_POINT ( 'NONE',  ( -2.500000000000000444, -61.16666666666666430, -4.330127018922193649 ) ) ;
#49805=CARTESIAN_POINT ( 'NONE',  ( -2.500000000000000444, -32.04166666393548724, -4.330127018922193649 ) ) ;
#49807=ORIENTED_EDGE ( 'NONE', *, *, #9100, .F. ) ;
#49808=DIRECTION ( 'NONE',  ( 0.000000000000000000, 0.000000000000000000, 1.000000000000000000 ) ) ;
#49816=CARTESIAN_POINT ( 'NONE',  ( -6.972266317189433020E-16, -76.12499999726880162, -5.000000000000000000 ) ) ;
#49824=CARTESIAN_POINT ( 'NONE',  ( -2.229367062500000163, -48.72916666530106511, -3.861377020970580443 ) ) ;
#49831=CYLINDRICAL_SURFACE ( 'NONE', #50924, 5.000000000000000000 ) ;
#49833=CARTESIAN_POINT ( 'NONE',  ( 4.458734124999998549, -92.97916666530106511, -2.574251347313721627 ) ) ;
#49834=CARTESIAN_POINT ( 'NONE',  ( 0.000000000000000000, -120.0000000000000000, 0.000000000000000000 ) ) ;
#49835=ORIENTED_EDGE ( 'NONE', *, *, #23163, .T. ) ;
#49839=( BOUNDED_CURVE ( )  B_SPLINE_CURVE ( 2, ( #46978, #2926, #42138, #12554, #12245, #57271, #7428, #46654, #2600 ),
 .UNSPECIFIED., .F., .F. ) 
 B_SPLINE_CURVE_WITH_KNOTS ( ( 3, 2, 2, 2, 3 ),
 ( 0.09821428571428571230, 0.09880952380952380543, 0.1000000000000000056, 0.1011904761904761918, 0.1017857142857142849 ),
 .UNSPECIFIED. ) 
 CURVE ( )  GEOMETRIC_REPRESENTATION_ITEM ( )  RATIONAL_B_SPLINE_CURVE ( ( 0.9330127018922194093, 0.9330127018922194093, 1.000000000000000000, 0.8660254037844387076, 1.000000000000000000, 0.8660254037844387076, 1.000000000000000000, 0.9330127018922194093, 0.9330127018922194093 ) ) 
 REPRESENTATION_ITEM ( '' )  );
#49842=CARTESIAN_POINT ( 'NONE',  ( 2.229367062499998831, 4.354166668032260823, -3.861377020970580887 ) ) ;
#49843=CARTESIAN_POINT ( 'NONE',  ( -4.458734124999999437, -16.56249999863440436, 0.000000000000000000 ) ) ;
#49844=VECTOR ( 'NONE', #25552, 1000.000000000000000 ) ;
#49845=CARTESIAN_POINT ( 'NONE',  ( -1.339745962155610925, -100.7946581987385315, 5.000000000000000000 ) ) ;
#49847=CARTESIAN_POINT ( 'NONE',  ( 5.000000000000000000, -55.29166666393548013, -2.886751345948130876 ) ) ;
#49849=CARTESIAN_POINT ( 'NONE',  ( -3.152548672688508926E-16, 14.18750000136559386, -5.148502694627439702 ) ) ;
#49852=CARTESIAN_POINT ( 'NONE',  ( 4.458734125000001214, -19.89583333196773651, 2.574251347313718519 ) ) ;
#49856=CARTESIAN_POINT ( 'NONE',  ( 5.000000000000000888, -48.45833333060215153, 2.886751345948126879 ) ) ;
#49858=CARTESIAN_POINT ( 'NONE',  ( 4.458734125000000326, 15.10416666803225993, 2.574251347313718519 ) ) ;
#49859=CARTESIAN_POINT ( 'NONE',  ( -2.500000000000000444, -9.041666663935483683, -4.330127018922193649 ) ) ;
#49862=CARTESIAN_POINT ( 'NONE',  ( -2.229367062500000163, -63.47916666530106511, -3.861377020970580443 ) ) ;
#49865=CARTESIAN_POINT ( 'NONE',  ( -5.000000000000000000, 3.916666666666665630, -2.886751345948128211 ) ) ;
#49867=CARTESIAN_POINT ( 'NONE',  ( -4.999999999999998224, 26.20833333606451632, 2.886751345948131764 ) ) ;
#49868=CARTESIAN_POINT ( 'NONE',  ( -3.152548672688508926E-16, -59.56249999863440081, -5.148502694627439702 ) ) ;
#49869=CARTESIAN_POINT ( 'NONE',  ( -5.000000000000000000, -91.95833333060214443, -2.886751345948128211 ) ) ;
#49870=EDGE_CURVE ( 'NONE', #49141, #56905, #42735, .T. ) ;
#49871=CARTESIAN_POINT ( 'NONE',  ( 9.457646018065525792E-16, -33.06249999863440792, 5.148502694627439702 ) ) ;
#49875=CARTESIAN_POINT ( 'NONE',  ( 1.339745962155612702, -16.16965819600733667, -5.000000000000000000 ) ) ;
#49877=CARTESIAN_POINT ( 'NONE',  ( -2.499999999999996447, -41.83333333333333570, 4.330127018922195425 ) ) ;
#49880=ORIENTED_EDGE ( 'NONE', *, *, #28330, .F. ) ;
#49881=CARTESIAN_POINT ( 'NONE',  ( 4.458734125000001214, -103.8958333319677365, 2.574251347313718519 ) ) ;
#49882=CARTESIAN_POINT ( 'NONE',  ( -4.458734124999999437, 4.354166668032260823, -2.574251347313719407 ) ) ;
#49885=EDGE_CURVE ( 'NONE', #32122, #60943, #56288, .T. ) ;
#49887=CARTESIAN_POINT ( 'NONE',  ( -2.500000000000000444, -26.16666666666666430, -4.330127018922193649 ) ) ;
#49890=ORIENTED_EDGE ( 'NONE', *, *, #57455, .T. ) ;
#49891=CARTESIAN_POINT ( 'NONE',  ( -6.972266317189433020E-16, -22.12499999726881228, -5.000000000000000000 ) ) ;
#49892=EDGE_CURVE ( 'NONE', #32964, #55487, #39503, .T. ) ;
#49894=CARTESIAN_POINT ( 'NONE',  ( 1.339745962155612702, -101.1696581960073331, -5.000000000000000000 ) ) ;
#49897=CARTESIAN_POINT ( 'NONE',  ( -2.229367062499996610, -29.39583333196774007, 3.861377020970582219 ) ) ;
#49905=VERTEX_POINT ( 'NONE', #27945 ) ;
#49908=CARTESIAN_POINT ( 'NONE',  ( 2.229367062499998831, -72.89583333196773651, -3.861377020970580887 ) ) ;
#49909=DIRECTION ( 'NONE',  ( -0.000000000000000000, 1.000000000000000000, -0.000000000000000000 ) ) ;
#49911=CARTESIAN_POINT ( 'NONE',  ( 2.499999999999998668, -16.33333333333333215, -4.330127018922193649 ) ) ;
#49914=CARTESIAN_POINT ( 'NONE',  ( -4.458734124999999437, -1.562499998634406140, 0.000000000000000000 ) ) ;
#49915=VERTEX_POINT ( 'NONE', #17976 ) ;
#49916=( BOUNDED_CURVE ( )  B_SPLINE_CURVE ( 2, ( #6257, #5612, #801, #5937, #10751, #35843, #40006, #15585, #49983 ),
 .UNSPECIFIED., .F., .F. ) 
 B_SPLINE_CURVE_WITH_KNOTS ( ( 3, 2, 2, 2, 3 ),
 ( 0.1160714285714285754, 0.1166666666666666685, 0.1178571428571428548, 0.1190476190476190410, 0.1196428571428571480 ),
 .UNSPECIFIED. ) 
 CURVE ( )  GEOMETRIC_REPRESENTATION_ITEM ( )  RATIONAL_B_SPLINE_CURVE ( ( 0.9330127018922194093, 0.9330127018922194093, 1.000000000000000000, 0.8660254037844387076, 1.000000000000000000, 0.8660254037844387076, 1.000000000000000000, 0.9330127018922185211, 0.9330127018922192983 ) ) 
 REPRESENTATION_ITEM ( '' )  );
#49917=CARTESIAN_POINT ( 'NONE',  ( 1.975475456537005874E-15, 8.375000002731187720, 5.000000000000000000 ) ) ;
#49918=EDGE_CURVE ( 'NONE', #44207, #13355, #4567, .T. ) ;
#49919=CARTESIAN_POINT ( 'NONE',  ( 5.000000000000000000, -27.49999999999999645, -6.123233995736766282E-16 ) ) ;
#49922=CARTESIAN_POINT ( 'NONE',  ( -6.972266317189433020E-16, -47.12499999726880873, -5.000000000000000000 ) ) ;
#49925=EDGE_LOOP ( 'NONE', ( #8552, #56164, #53711, #33075 ) ) ;
#49926=CARTESIAN_POINT ( 'NONE',  ( 4.458734124999999437, -79.81249999863440792, -5.460374474430324690E-16 ) ) ;
#49927=CARTESIAN_POINT ( 'NONE',  ( 1.339745962155612702, -29.16965819600733312, -5.000000000000000000 ) ) ;
#49928=CARTESIAN_POINT ( 'NONE',  ( 2.229367062499998831, -0.6458333319677399542, -3.861377020970580887 ) ) ;
#49932=CARTESIAN_POINT ( 'NONE',  ( -3.152548672688508926E-16, -68.81249999863439371, -5.148502694627439702 ) ) ;
#49933=CARTESIAN_POINT ( 'NONE',  ( 1.060575238724906964E-15, -27.62499999726881228, 5.773502691896257311 ) ) ;
#49935=CARTESIAN_POINT ( 'NONE',  ( 2.229367062499998831, 29.35416666803225993, -3.861377020970580887 ) ) ;
#49936=CARTESIAN_POINT ( 'NONE',  ( -5.000000000000000000, -55.99999999999999289, 0.000000000000000000 ) ) ;
#49937=CARTESIAN_POINT ( 'NONE',  ( 1.339745962155729053, -43.16965819600733312, -4.999999999999933387 ) ) ;
#49938=CARTESIAN_POINT ( 'NONE',  ( 4.458734124999999437, -47.81249999863440792, -5.460374474430324690E-16 ) ) ;
#49939=CARTESIAN_POINT ( 'NONE',  ( 4.458734125000000326, -30.14583333196773651, 2.574251347313718519 ) ) ;
#49943=CARTESIAN_POINT ( 'NONE',  ( 2.499999999999998668, 19.66666666666666430, -4.330127018922193649 ) ) ;
#49946=CARTESIAN_POINT ( 'NONE',  ( 2.229367062500001939, -40.97916666530107221, 3.861377020970579999 ) ) ;
#49947=CARTESIAN_POINT ( 'NONE',  ( -3.535250795749689387E-16, -75.12499999726880162, -5.773502691896257311 ) ) ;
#49948=AXIS2_PLACEMENT_3D ( 'NONE', #41548, #31598, #32867 ) ;
#49952=EDGE_CURVE ( 'NONE', #12052, #62764, #15276, .T. ) ;
#49955=CARTESIAN_POINT ( 'NONE',  ( 4.458734124999999437, -81.06249999863440792, -5.460374474430324690E-16 ) ) ;
#49957=CARTESIAN_POINT ( 'NONE',  ( 1.975475456537005874E-15, 18.37500000273118062, 5.000000000000000000 ) ) ;
#49959=CARTESIAN_POINT ( 'NONE',  ( -5.000000000000000000, -30.00000000000000000, 0.000000000000000000 ) ) ;
#49961=VERTEX_POINT ( 'NONE', #33408 ) ;
#49965=CARTESIAN_POINT ( 'NONE',  ( -5.000000000000000000, 24.12500000273118417, 0.000000000000000000 ) ) ;
#49975=CARTESIAN_POINT ( 'NONE',  ( 5.000000000000000000, -56.29166666393548013, -2.886751345948130876 ) ) ;
#49977=CARTESIAN_POINT ( 'NONE',  ( -3.152548672688508926E-16, -20.56249999863440081, -5.148502694627439702 ) ) ;
#49978=CARTESIAN_POINT ( 'NONE',  ( -2.500000000000000444, -78.04166666393547303, -4.330127018922193649 ) ) ;
#49982=EDGE_LOOP ( 'NONE', ( #5193, #51026, #29195, #49985 ) ) ;
#49983=CARTESIAN_POINT ( 'NONE',  ( -2.916731409357579869E-14, 13.25000000000000178, 5.000000000000000888 ) ) ;
#49985=ORIENTED_EDGE ( 'NONE', *, *, #31521, .T. ) ;
#49987=DIRECTION ( 'NONE',  ( 0.000000000000000000, 0.000000000000000000, 1.000000000000000000 ) ) ;
#49990=( BOUNDED_CURVE ( )  B_SPLINE_CURVE ( 2, ( #63349, #23792, #63666, #54322, #9927, #58514, #34061, #59474, #19899 ),
 .UNSPECIFIED., .F., .F. ) 
 B_SPLINE_CURVE_WITH_KNOTS ( ( 3, 2, 2, 2, 3 ),
 ( 0.4053571428571428603, 0.4059523809523809534, 0.4071428571428571397, 0.4083333333333333259, 0.4089285714285714191 ),
 .UNSPECIFIED. ) 
 CURVE ( )  GEOMETRIC_REPRESENTATION_ITEM ( )  RATIONAL_B_SPLINE_CURVE ( ( 0.9330127018922194093, 0.9330127018922194093, 1.000000000000000000, 0.8660254037844387076, 1.000000000000000000, 0.8660254037844387076, 1.000000000000000000, 0.9330127018922194093, 0.9330127018922194093 ) ) 
 REPRESENTATION_ITEM ( '' )  );
#49993=CARTESIAN_POINT ( 'NONE',  ( 5.000000000000000000, 15.50000000000000000, -6.123233995736766282E-16 ) ) ;
#49997=AXIS2_PLACEMENT_3D ( 'NONE', #282, #8971, #4456 ) ;
#49999=CARTESIAN_POINT ( 'NONE',  ( 4.458734124999999437, 15.18750000136559564, -5.460374474430324690E-16 ) ) ;
#50002=DIRECTION ( 'NONE',  ( -0.000000000000000000, 1.000000000000000000, -0.000000000000000000 ) ) ;
#50005=CARTESIAN_POINT ( 'NONE',  ( -4.458734124999999437, -67.39583333196773651, -2.574251347313719407 ) ) ;
#50006=CARTESIAN_POINT ( 'NONE',  ( -2.500000000000000444, -50.04166666393547303, -4.330127018922193649 ) ) ;
#50007=CARTESIAN_POINT ( 'NONE',  ( 2.229367062499998831, 19.35416666803225993, -3.861377020970580887 ) ) ;
#50008=CARTESIAN_POINT ( 'NONE',  ( -5.000000000000000000, 17.91666666666666430, -2.886751345948128211 ) ) ;
#50010=CARTESIAN_POINT ( 'NONE',  ( 4.458734124999998549, -48.97916666530107221, -2.574251347313721627 ) ) ;
#50011=CARTESIAN_POINT ( 'NONE',  ( -5.000000000000000000, -10.95833333060214621, -2.886751345948128211 ) ) ;
#50016=( BOUNDED_CURVE ( )  B_SPLINE_CURVE ( 2, ( #23611, #39323, #30314, #59609, #30639, #5563, #1400, #45437, #24869 ),
 .UNSPECIFIED., .F., .F. ) 
 B_SPLINE_CURVE_WITH_KNOTS ( ( 3, 2, 2, 2, 3 ),
 ( 0.5053571428571428381, 0.5059523809523809312, 0.5071428571428571175, 0.5083333333333333037, 0.5089285714285713969 ),
 .UNSPECIFIED. ) 
 CURVE ( )  GEOMETRIC_REPRESENTATION_ITEM ( )  RATIONAL_B_SPLINE_CURVE ( ( 0.9330127018922194093, 0.9330127018922194093, 1.000000000000000000, 0.8660254037844387076, 1.000000000000000000, 0.8660254037844387076, 1.000000000000000000, 0.9330127018922194093, 0.9330127018922194093 ) ) 
 REPRESENTATION_ITEM ( '' )  );
#50017=CARTESIAN_POINT ( 'NONE',  ( 4.458734124999998549, -15.97916666530107221, -2.574251347313721627 ) ) ;
#50020=CARTESIAN_POINT ( 'NONE',  ( -4.458734124999999437, -104.3124999986344079, 0.000000000000000000 ) ) ;
#50023=CARTESIAN_POINT ( 'NONE',  ( -2.229367062499996610, -99.39583333196773651, 3.861377020970582219 ) ) ;
#50024=CARTESIAN_POINT ( 'NONE',  ( 6.123233995736766282E-16, -120.0000000000000000, -5.000000000000000000 ) ) ;
#50025=CARTESIAN_POINT ( 'NONE',  ( -4.999999999999999112, -59.79166666393547303, 2.886751345948131764 ) ) ;
#50026=CARTESIAN_POINT ( 'NONE',  ( -1.339745962155613812, 18.91965820146970501, -5.000000000000000000 ) ) ;
#50030=CARTESIAN_POINT ( 'NONE',  ( -4.458734124999999437, -24.31249999863440436, 0.000000000000000000 ) ) ;
#50031=CARTESIAN_POINT ( 'NONE',  ( 4.458734124999998549, 6.020833334698928674, -2.574251347313721627 ) ) ;
#50032=CARTESIAN_POINT ( 'NONE',  ( 2.229367062499998831, -66.89583333196773651, -3.861377020970580887 ) ) ;
#50035=CARTESIAN_POINT ( 'NONE',  ( 0.000000000000000000, -120.0000000000000000, 0.000000000000000000 ) ) ;
#50037=CARTESIAN_POINT ( 'NONE',  ( -5.000000000000000000, -9.000000000000001776, 0.000000000000000000 ) ) ;
#50039=ORIENTED_EDGE ( 'NONE', *, *, #22815, .T. ) ;
#50042=CYLINDRICAL_SURFACE ( 'NONE', #2720, 5.000000000000000000 ) ;
#50043=CARTESIAN_POINT ( 'NONE',  ( 5.000000000000000888, -92.58333333333334281, 2.886751345948126879 ) ) ;
#50045=CIRCLE ( 'NONE', #4861, 5.000000000000000000 ) ;
#50048=AXIS2_PLACEMENT_3D ( 'NONE', #12064, #46488, #36839 ) ;
#50052=CARTESIAN_POINT ( 'NONE',  ( -2.500000000000000444, -74.16666666666665719, -4.330127018922193649 ) ) ;
#50054=EDGE_CURVE ( 'NONE', #53062, #53577, #34034, .T. ) ;
#50055=ORIENTED_EDGE ( 'NONE', *, *, #32316, .T. ) ;
#50056=CARTESIAN_POINT ( 'NONE',  ( -1.339745962155613812, -98.20534180126146850, -5.000000000000000000 ) ) ;
#50057=EDGE_LOOP ( 'NONE', ( #25471, #8242, #45089, #6512 ) ) ;
#50058=FACE_OUTER_BOUND ( 'NONE', #2321, .T. ) ;
#50061=EDGE_CURVE ( 'NONE', #39400, #57534, #42333, .T. ) ;
#50065=ORIENTED_EDGE ( 'NONE', *, *, #40068, .F. ) ;
#50069=DIRECTION ( 'NONE',  ( -0.000000000000000000, 1.000000000000000000, -0.000000000000000000 ) ) ;
#50073=CARTESIAN_POINT ( 'NONE',  ( -6.972266317189433020E-16, 3.749999999999999556, -5.000000000000000000 ) ) ;
#50074=ORIENTED_EDGE ( 'NONE', *, *, #26702, .F. ) ;
#50076=CARTESIAN_POINT ( 'NONE',  ( 4.458734124999998549, 28.27083333469892779, -2.574251347313721627 ) ) ;
#50078=ORIENTED_EDGE ( 'NONE', *, *, #42855, .F. ) ;
#50082=CARTESIAN_POINT ( 'NONE',  ( -4.458734124999997661, -42.22916666530107932, 2.574251347313722516 ) ) ;
#50084=VECTOR ( 'NONE', #50169, 1000.000000000000000 ) ;
#50086=CARTESIAN_POINT ( 'NONE',  ( -4.458734124999997661, -47.22916666530105800, 2.574251347313722516 ) ) ;
#50088=CARTESIAN_POINT ( 'NONE',  ( 6.123233995736766282E-16, -120.0000000000000000, -5.000000000000000000 ) ) ;
#50090=CARTESIAN_POINT ( 'NONE',  ( 9.457646018065525792E-16, -18.06249999863440436, 5.148502694627439702 ) ) ;
#50091=CARTESIAN_POINT ( 'NONE',  ( 1.060575238724906964E-15, -102.7500000000000142, 5.773502691896257311 ) ) ;
#50093=CARTESIAN_POINT ( 'NONE',  ( 2.229367062500001939, -34.22916666530107221, 3.861377020970579999 ) ) ;
#50094=CARTESIAN_POINT ( 'NONE',  ( -5.000000000000000000, 9.125000002731184168, 0.000000000000000000 ) ) ;
#50095=CARTESIAN_POINT ( 'NONE',  ( -1.339745962155610925, -6.669658196007334894, 5.000000000000000000 ) ) ;
#50099=CARTESIAN_POINT ( 'NONE',  ( 9.457646018065525792E-16, 0.6875000013655957476, 5.148502694627439702 ) ) ;
#50100=ORIENTED_EDGE ( 'NONE', *, *, #41324, .F. ) ;
#50102=CARTESIAN_POINT ( 'NONE',  ( -4.458734124999999437, -90.39583333196773651, -2.574251347313719407 ) ) ;
#50103=CARTESIAN_POINT ( 'NONE',  ( -2.229367062500000163, -34.47916666530107221, -3.861377020970580443 ) ) ;
#50104=CARTESIAN_POINT ( 'NONE',  ( 1.339745962155615144, -9.705341801261479162, 4.999999999999999112 ) ) ;
#50105=CARTESIAN_POINT ( 'NONE',  ( -2.229367062500000163, -80.72916666530106511, -3.861377020970580443 ) ) ;
#50109=CARTESIAN_POINT ( 'NONE',  ( 4.458734124999998549, -3.729166665301070438, -2.574251347313721627 ) ) ;
#50110=CARTESIAN_POINT ( 'NONE',  ( 9.457646018065525792E-16, 23.68750000136559564, 5.148502694627439702 ) ) ;
#50111=CARTESIAN_POINT ( 'NONE',  ( 4.458734125000000326, -48.14583333196773651, 2.574251347313718519 ) ) ;
#50118=CARTESIAN_POINT ( 'NONE',  ( -3.152548672688508926E-16, -76.56249999863440792, -5.148502694627439702 ) ) ;
#50119=CARTESIAN_POINT ( 'NONE',  ( 5.000000000000000888, -109.4583333306021586, 2.886751345948126879 ) ) ;
#50120=( BOUNDED_CURVE ( )  B_SPLINE_CURVE ( 2, ( #15762, #40201, #25085, #16078, #40514, #11564, #26050, #59837, #54999 ),
 .UNSPECIFIED., .F., .F. ) 
 B_SPLINE_CURVE_WITH_KNOTS ( ( 3, 2, 2, 2, 3 ),
 ( 0.1660714285714285643, 0.1666666666666666574, 0.1678571428571428437, 0.1690476190476190577, 0.1696428571428571508 ),
 .UNSPECIFIED. ) 
 CURVE ( )  GEOMETRIC_REPRESENTATION_ITEM ( )  RATIONAL_B_SPLINE_CURVE ( ( 0.9330127018922194093, 0.9330127018922194093, 1.000000000000000000, 0.8660254037844387076, 1.000000000000000000, 0.8660254037844387076, 1.000000000000000000, 0.9330127018922194093, 0.9330127018922194093 ) ) 
 REPRESENTATION_ITEM ( '' )  );
#50122=CARTESIAN_POINT ( 'NONE',  ( 1.975475456537005874E-15, 10.24999999999999822, 5.000000000000000000 ) ) ;
#50123=CARTESIAN_POINT ( 'NONE',  ( 0.000000000000000000, -120.0000000000000000, 0.000000000000000000 ) ) ;
#50125=CARTESIAN_POINT ( 'NONE',  ( -2.499999999999996447, -56.83333333333333570, 4.330127018922195425 ) ) ;
#50128=ORIENTED_EDGE ( 'NONE', *, *, #57123, .F. ) ;
#50129=CARTESIAN_POINT ( 'NONE',  ( 0.000000000000000000, -120.0000000000000000, 0.000000000000000000 ) ) ;
#50130=CARTESIAN_POINT ( 'NONE',  ( -6.972266317189433020E-16, -52.12499999726880873, -5.000000000000000000 ) ) ;
#50145=CARTESIAN_POINT ( 'NONE',  ( -4.458734124999998549, -44.47916666530106511, 2.574251347313722516 ) ) ;
#50148=CARTESIAN_POINT ( 'NONE',  ( 6.123233995736766282E-16, -120.0000000000000000, -5.000000000000000000 ) ) ;
#50151=AXIS2_PLACEMENT_3D ( 'NONE', #51621, #6922, #17525 ) ;
#50153=DIRECTION ( 'NONE',  ( 0.000000000000000000, 0.000000000000000000, 1.000000000000000000 ) ) ;
#50155=CARTESIAN_POINT ( 'NONE',  ( -4.458734124999999437, -95.56249999863440792, 0.000000000000000000 ) ) ;
#50157=ORIENTED_EDGE ( 'NONE', *, *, #15318, .F. ) ;
#50161=EDGE_CURVE ( 'NONE', #6339, #6165, #33100, .T. ) ;
#50163=CARTESIAN_POINT ( 'NONE',  ( 9.457646018065525792E-16, -2.062499998634407028, 5.148502694627439702 ) ) ;
#50164=CARTESIAN_POINT ( 'NONE',  ( 1.339745962155615144, -106.7053418012614543, 4.999999999999999112 ) ) ;
#50165=CARTESIAN_POINT ( 'NONE',  ( 2.229367062500001939, -19.22916666530106866, 3.861377020970579999 ) ) ;
#50166=( BOUNDED_CURVE ( )  B_SPLINE_CURVE ( 2, ( #55070, #10992, #6822, #30613, #26428, #45411, #46046, #2011, #1379 ),
 .UNSPECIFIED., .F., .F. ) 
 B_SPLINE_CURVE_WITH_KNOTS ( ( 3, 2, 2, 2, 3 ),
 ( 0.1125000000000000028, 0.1130952380952380959, 0.1142857142857142821, 0.1154761904761904823, 0.1160714285714285754 ),
 .UNSPECIFIED. ) 
 CURVE ( )  GEOMETRIC_REPRESENTATION_ITEM ( )  RATIONAL_B_SPLINE_CURVE ( ( 0.9330127018922194093, 0.9330127018922194093, 1.000000000000000000, 0.8660254037844387076, 1.000000000000000000, 0.8660254037844387076, 1.000000000000000000, 0.9330127018922194093, 0.9330127018922194093 ) ) 
 REPRESENTATION_ITEM ( '' )  );
#50169=DIRECTION ( 'NONE',  ( -0.000000000000000000, 1.000000000000000000, -0.000000000000000000 ) ) ;
#50172=AXIS2_PLACEMENT_3D ( 'NONE', #20678, #21307, #60869 ) ;
#50173=CARTESIAN_POINT ( 'NONE',  ( 4.458734124999999437, 16.93750000136559564, -5.460374474430324690E-16 ) ) ;
#50174=ORIENTED_EDGE ( 'NONE', *, *, #7679, .T. ) ;
#50175=CARTESIAN_POINT ( 'NONE',  ( -1.339745962155610925, -13.66965819600733489, 5.000000000000000000 ) ) ;
#50177=CARTESIAN_POINT ( 'NONE',  ( -2.229367062499996610, -21.14583333196774007, 3.861377020970582219 ) ) ;
#50181=CARTESIAN_POINT ( 'NONE',  ( -5.000000000000000000, -44.95833333060215153, -2.886751345948128211 ) ) ;
#50183=CARTESIAN_POINT ( 'NONE',  ( 2.229367062499998831, 14.35416666803226171, -3.861377020970580887 ) ) ;
#50187=CARTESIAN_POINT ( 'NONE',  ( 4.458734124999999437, -66.81249999863440792, -5.460374474430324690E-16 ) ) ;
#50188=VERTEX_POINT ( 'NONE', #14095 ) ;
#50190=CARTESIAN_POINT ( 'NONE',  ( 5.000000000000000000, 2.499999999999998668, -6.123233995736766282E-16 ) ) ;
#50193=CARTESIAN_POINT ( 'NONE',  ( -2.229367062499996610, -60.14583333196774362, 3.861377020970582219 ) ) ;
#50194=CARTESIAN_POINT ( 'NONE',  ( 5.000000000000000000, -95.37499999726881583, -6.123233995736766282E-16 ) ) ;
#50195=CARTESIAN_POINT ( 'NONE',  ( -2.229367062500000163, -33.47916666530107221, -3.861377020970580443 ) ) ;
#50197=CARTESIAN_POINT ( 'NONE',  ( -2.499999999999996447, -41.70833333060214443, 4.330127018922195425 ) ) ;
#50200=CARTESIAN_POINT ( 'NONE',  ( 5.000000000000000000, 1.583333333333332371, -2.886751345948130876 ) ) ;
#50202=( BOUNDED_CURVE ( )  B_SPLINE_CURVE ( 2, ( #28203, #4392, #49405, #4700, #34285, #5669, #9530, #24323, #19813 ),
 .UNSPECIFIED., .F., .F. ) 
 B_SPLINE_CURVE_WITH_KNOTS ( ( 3, 2, 2, 2, 3 ),
 ( 0.2767857142857143016, 0.2773809523809523947, 0.2785714285714285809, 0.2797619047619047672, 0.2803571428571428603 ),
 .UNSPECIFIED. ) 
 CURVE ( )  GEOMETRIC_REPRESENTATION_ITEM ( )  RATIONAL_B_SPLINE_CURVE ( ( 0.9330127018922194093, 0.9330127018922194093, 1.000000000000000000, 0.8660254037844387076, 1.000000000000000000, 0.8660254037844387076, 1.000000000000000000, 0.9330127018922194093, 0.9330127018922194093 ) ) 
 REPRESENTATION_ITEM ( '' )  );
#50203=CARTESIAN_POINT ( 'NONE',  ( 2.500000000000002220, -45.66666666666666430, 4.330127018922192761 ) ) ;
#50205=CARTESIAN_POINT ( 'NONE',  ( 5.000000000000000000, -86.37499999726880162, -6.123233995736766282E-16 ) ) ;
#50206=ORIENTED_EDGE ( 'NONE', *, *, #40089, .F. ) ;
#50207=CARTESIAN_POINT ( 'NONE',  ( 4.458734124999998549, -104.7291666653010509, -2.574251347313721627 ) ) ;
#50208=CARTESIAN_POINT ( 'NONE',  ( -3.152548672688508926E-16, 2.187500001365593416, -5.148502694627439702 ) ) ;
#50209=CARTESIAN_POINT ( 'NONE',  ( 2.499999999999998668, -59.33333333333333570, -4.330127018922193649 ) ) ;
#50219=ORIENTED_EDGE ( 'NONE', *, *, #39433, .T. ) ;
#50220=CARTESIAN_POINT ( 'NONE',  ( -2.499999999999996447, -48.70833333060213732, 4.330127018922195425 ) ) ;
#50222=CARTESIAN_POINT ( 'NONE',  ( -4.458734124999998549, -32.47916666530107221, 2.574251347313722516 ) ) ;
#50224=CARTESIAN_POINT ( 'NONE',  ( 0.000000000000000000, -120.0000000000000000, 5.000000000000000000 ) ) ;
#50232=VERTEX_POINT ( 'NONE', #8648 ) ;
#50234=EDGE_LOOP ( 'NONE', ( #10728, #55781, #13233 ) ) ;
#50235=CARTESIAN_POINT ( 'NONE',  ( 4.458734124999998549, -77.97916666530106511, -2.574251347313721627 ) ) ;
#50238=CARTESIAN_POINT ( 'NONE',  ( -2.500000000000000444, -15.04166666393548191, -4.330127018922193649 ) ) ;
#50239=CARTESIAN_POINT ( 'NONE',  ( -4.999999999999998224, 8.083333333333332149, 2.886751345948131764 ) ) ;
#50242=CARTESIAN_POINT ( 'NONE',  ( 4.458734125000001214, -3.145833331967738733, 2.574251347313718519 ) ) ;
#50252=CARTESIAN_POINT ( 'NONE',  ( 2.229367062500001939, -79.97916666530106511, 3.861377020970579999 ) ) ;
#50253=CARTESIAN_POINT ( 'NONE',  ( -2.499999999999996447, -96.83333333333332860, 4.330127018922195425 ) ) ;
#50254=CARTESIAN_POINT ( 'NONE',  ( 4.458734125000001214, -5.895833331967740953, 2.574251347313718519 ) ) ;
#50256=EDGE_CURVE ( 'NONE', #11403, #28956, #52672, .T. ) ;
#50258=CARTESIAN_POINT ( 'NONE',  ( 9.457646018065525792E-16, -71.31249999863439371, 5.148502694627439702 ) ) ;
#50259=CARTESIAN_POINT ( 'NONE',  ( 2.499999999999998668, -28.20833333060214798, -4.330127018922193649 ) ) ;
#50262=CARTESIAN_POINT ( 'NONE',  ( -1.336351044127974539E-14, 23.24999999999999645, 5.000000000000000000 ) ) ;
#50264=CARTESIAN_POINT ( 'NONE',  ( -2.229367062499996610, -51.14583333196772941, 3.861377020970582219 ) ) ;
#50265=CARTESIAN_POINT ( 'NONE',  ( 4.458734124999998549, -34.97916666530107221, -2.574251347313721627 ) ) ;
#50269=CARTESIAN_POINT ( 'NONE',  ( -5.000000000000000000, 20.99999999999999645, 0.000000000000000000 ) ) ;
#50272=AXIS2_PLACEMENT_3D ( 'NONE', #21336, #30660, #51250 ) ;
#50273=CARTESIAN_POINT ( 'NONE',  ( 9.457646018065525792E-16, -41.06249999863440792, 5.148502694627439702 ) ) ;
#50274=CARTESIAN_POINT ( 'NONE',  ( 1.060575238724906964E-15, -72.62499999726880162, 5.773502691896257311 ) ) ;
#50275=EDGE_CURVE ( 'NONE', #14167, #12673, #459, .T. ) ;
#50277=CARTESIAN_POINT ( 'NONE',  ( -4.458734124999999437, -110.3124999986343937, 0.000000000000000000 ) ) ;
#50279=CARTESIAN_POINT ( 'NONE',  ( 9.457646018065525792E-16, -79.31249999863440792, 5.148502694627439702 ) ) ;
#50281=CARTESIAN_POINT ( 'NONE',  ( 6.123233995736766282E-16, -120.0000000000000000, -5.000000000000000000 ) ) ;
#50282=CARTESIAN_POINT ( 'NONE',  ( 2.499999999999998668, -28.33333333333333570, -4.330127018922193649 ) ) ;
#50284=VERTEX_POINT ( 'NONE', #21156 ) ;
#50288=CARTESIAN_POINT ( 'NONE',  ( -2.499999999999996447, 21.29166666939785202, 4.330127018922195425 ) ) ;
#50296=FACE_OUTER_BOUND ( 'NONE', #19534, .T. ) ;
#50297=CARTESIAN_POINT ( 'NONE',  ( -5.000000000000000000, -74.95833333060214443, -2.886751345948128211 ) ) ;
#50300=CARTESIAN_POINT ( 'NONE',  ( -2.229367062500000163, -12.72916666530107044, -3.861377020970580443 ) ) ;
#50301=CARTESIAN_POINT ( 'NONE',  ( -2.499999999999996447, -77.70833333060214443, 4.330127018922195425 ) ) ;
#50305=( BOUNDED_CURVE ( )  B_SPLINE_CURVE ( 2, ( #25866, #25226, #45481, #6570, #59976, #34535, #15899, #35518, #44196 ),
 .UNSPECIFIED., .F., .F. ) 
 B_SPLINE_CURVE_WITH_KNOTS ( ( 3, 2, 2, 2, 3 ),
 ( 0.02678571428571428770, 0.02738095238095238082, 0.02857142857142857054, 0.02976190476190476025, 0.03035714285714285685 ),
 .UNSPECIFIED. ) 
 CURVE ( )  GEOMETRIC_REPRESENTATION_ITEM ( )  RATIONAL_B_SPLINE_CURVE ( ( 0.9330127018922194093, 0.9330127018922195203, 1.000000000000000000, 0.8660254037844387076, 1.000000000000000000, 0.8660254037844387076, 1.000000000000000000, 0.9330127018922194093, 0.9330127018922194093 ) ) 
 REPRESENTATION_ITEM ( '' )  );
#50307=ORIENTED_EDGE ( 'NONE', *, *, #52658, .T. ) ;
#50310=VERTEX_POINT ( 'NONE', #35957 ) ;
#50311=CARTESIAN_POINT ( 'NONE',  ( 1.339745962155615144, -21.70534180126147916, 4.999999999999999112 ) ) ;
#50312=CARTESIAN_POINT ( 'NONE',  ( 1.339745962155615144, 11.41965820146970501, 4.999999999999999112 ) ) ;
#50314=ORIENTED_EDGE ( 'NONE', *, *, #11054, .T. ) ;
#50318=CARTESIAN_POINT ( 'NONE',  ( 2.500000000000002220, -86.66666666666667140, 4.330127018922192761 ) ) ;
#50319=AXIS2_PLACEMENT_3D ( 'NONE', #33525, #9382, #33832 ) ;
#50321=EDGE_CURVE ( 'NONE', #10433, #44276, #59634, .T. ) ;
#50323=( BOUNDED_CURVE ( )  B_SPLINE_CURVE ( 2, ( #2225, #27587, #12484, #42378, #31146, #22145, #2847, #7036, #16997 ),
 .UNSPECIFIED., .F., .F. ) 
 B_SPLINE_CURVE_WITH_KNOTS ( ( 3, 2, 2, 2, 3 ),
 ( 0.1589285714285714191, 0.1595238095238095122, 0.1607142857142857262, 0.1619047619047619124, 0.1625000000000000056 ),
 .UNSPECIFIED. ) 
 CURVE ( )  GEOMETRIC_REPRESENTATION_ITEM ( )  RATIONAL_B_SPLINE_CURVE ( ( 0.9330127018922194093, 0.9330127018922194093, 1.000000000000000000, 0.8660254037844387076, 1.000000000000000000, 0.8660254037844387076, 1.000000000000000000, 0.9330127018922194093, 0.9330127018922194093 ) ) 
 REPRESENTATION_ITEM ( '' )  );
#50327=CARTESIAN_POINT ( 'NONE',  ( -4.458734124999999437, 11.68750000136559564, 0.000000000000000000 ) ) ;
#50330=CARTESIAN_POINT ( 'NONE',  ( 5.000000000000000888, 12.54166666939785557, 2.886751345948126879 ) ) ;
#50331=CARTESIAN_POINT ( 'NONE',  ( -6.972266317189433020E-16, -25.24999999999999645, -5.000000000000000000 ) ) ;
#50332=CARTESIAN_POINT ( 'NONE',  ( 4.458734124999998549, -63.72916666530106511, -2.574251347313721627 ) ) ;
#50334=CARTESIAN_POINT ( 'NONE',  ( 4.458734124999998549, 13.27083333469892779, -2.574251347313721627 ) ) ;
#50335=DIRECTION ( 'NONE',  ( -1.000000000000000000, -0.000000000000000000, -3.614007241618347908E-17 ) ) ;
#50337=CARTESIAN_POINT ( 'NONE',  ( 4.458734124999999437, -56.06249999863440081, -5.460374474430324690E-16 ) ) ;
#50338=CARTESIAN_POINT ( 'NONE',  ( 5.000000000000000000, -14.29166666393548191, -2.886751345948129988 ) ) ;
#50339=CARTESIAN_POINT ( 'NONE',  ( 2.500000000000002220, -25.54166666393547658, 4.330127018922192761 ) ) ;
#50341=CARTESIAN_POINT ( 'NONE',  ( 1.975475456537005874E-15, -65.62499999726881583, 5.000000000000000000 ) ) ;
#50343=CARTESIAN_POINT ( 'NONE',  ( 2.500000000000002220, -104.5416666639354730, 4.330127018922192761 ) ) ;
#50344=CARTESIAN_POINT ( 'NONE',  ( 4.458734124999999437, -16.06249999863440436, -5.460374474430324690E-16 ) ) ;
#50345=ORIENTED_EDGE ( 'NONE', *, *, #49683, .T. ) ;
#50347=CARTESIAN_POINT ( 'NONE',  ( -2.229367062500000163, -106.4791666653010651, -3.861377020970580443 ) ) ;
#50349=EDGE_LOOP ( 'NONE', ( #63614, #22869, #18960, #48509 ) ) ;
#50350=CARTESIAN_POINT ( 'NONE',  ( 2.229367062499998831, -101.8958333319677365, -3.861377020970580887 ) ) ;
#50351=CARTESIAN_POINT ( 'NONE',  ( 4.458734124999998549, -27.72916666530107221, -2.574251347313721627 ) ) ;
#50352=CARTESIAN_POINT ( 'NONE',  ( 2.500000000000002220, -59.54166666393546592, 4.330127018922192761 ) ) ;
#50355=CARTESIAN_POINT ( 'NONE',  ( -2.229367062499996610, -24.14583333196773651, 3.861377020970582219 ) ) ;
#50356=CARTESIAN_POINT ( 'NONE',  ( 9.457646018065525792E-16, -65.31249999863440792, 5.148502694627439702 ) ) ;
#50359=DIRECTION ( 'NONE',  ( -0.000000000000000000, 1.000000000000000000, -0.000000000000000000 ) ) ;
#50361=CARTESIAN_POINT ( 'NONE',  ( -5.000000000000000000, -10.00000000000000178, 0.000000000000000000 ) ) ;
#50367=CARTESIAN_POINT ( 'NONE',  ( 2.493747252781420335E-13, -90.25000000000000000, -5.000000000000000000 ) ) ;
#50372=CARTESIAN_POINT ( 'NONE',  ( 6.123233995736766282E-16, -120.0000000000000000, -5.000000000000000000 ) ) ;
#50374=CARTESIAN_POINT ( 'NONE',  ( 1.060575238724906964E-15, -78.75000000000001421, 5.773502691896257311 ) ) ;
#50378=VERTEX_POINT ( 'NONE', #10860 ) ;
#50379=( BOUNDED_CURVE ( )  B_SPLINE_CURVE ( 2, ( #16804, #6526, #35796, #55419, #16489, #11337, #36424, #30640, #50585 ),
 .UNSPECIFIED., .F., .F. ) 
 B_SPLINE_CURVE_WITH_KNOTS ( ( 3, 2, 2, 2, 3 ),
 ( 0.9589285714285714635, 0.9595238095238095566, 0.9607142857142857428, 0.9619047619047619291, 0.9625000000000000222 ),
 .UNSPECIFIED. ) 
 CURVE ( )  GEOMETRIC_REPRESENTATION_ITEM ( )  RATIONAL_B_SPLINE_CURVE ( ( 0.9330127018922194093, 0.9330127018922194093, 1.000000000000000000, 0.8660254037844387076, 1.000000000000000000, 0.8660254037844387076, 1.000000000000000000, 0.9330127018922194093, 0.9330127018922194093 ) ) 
 REPRESENTATION_ITEM ( '' )  );
#50380=CARTESIAN_POINT ( 'NONE',  ( 6.123233995736766282E-16, -120.0000000000000000, -5.000000000000000000 ) ) ;
#50386=ORIENTED_EDGE ( 'NONE', *, *, #3971, .T. ) ;
#50391=ORIENTED_EDGE ( 'NONE', *, *, #63066, .F. ) ;
#50394=CARTESIAN_POINT ( 'NONE',  ( -4.999999999999998224, -83.91666666666667140, 2.886751345948131764 ) ) ;
#50398=CARTESIAN_POINT ( 'NONE',  ( -4.458734124999998549, -76.22916666530107932, 2.574251347313722516 ) ) ;
#50399=CARTESIAN_POINT ( 'NONE',  ( 4.458734124999999437, -110.0624999986343937, -5.460374474430324690E-16 ) ) ;
#50402=VERTEX_POINT ( 'NONE', #28110 ) ;
#50403=CARTESIAN_POINT ( 'NONE',  ( -1.339745962155610925, 5.330341803992665994, 5.000000000000000000 ) ) ;
#50408=CARTESIAN_POINT ( 'NONE',  ( -3.152548672688508926E-16, -41.56249999863440081, -5.148502694627439702 ) ) ;
#50410=( BOUNDED_CURVE ( )  B_SPLINE_CURVE ( 2, ( #59665, #33934, #34894, #19454, #59337, #10122, #19130, #24602, #15270 ),
 .UNSPECIFIED., .F., .F. ) 
 B_SPLINE_CURVE_WITH_KNOTS ( ( 3, 2, 2, 2, 3 ),
 ( 0.9446428571428571175, 0.9452380952380952106, 0.9464285714285713969, 0.9476190476190475831, 0.9482142857142856762 ),
 .UNSPECIFIED. ) 
 CURVE ( )  GEOMETRIC_REPRESENTATION_ITEM ( )  RATIONAL_B_SPLINE_CURVE ( ( 0.9330127018922194093, 0.9330127018922194093, 1.000000000000000000, 0.8660254037844387076, 1.000000000000000000, 0.8660254037844387076, 1.000000000000000000, 0.9330127018922194093, 0.9330127018922194093 ) ) 
 REPRESENTATION_ITEM ( '' )  );
#50411=EDGE_CURVE ( 'NONE', #17652, #63145, #62851, .T. ) ;
#50413=CARTESIAN_POINT ( 'NONE',  ( 4.458734124999998549, -51.72916666530107221, -2.574251347313721627 ) ) ;
#50416=CARTESIAN_POINT ( 'NONE',  ( -4.458734124999998549, 28.77083333469892779, 2.574251347313722516 ) ) ;
#50417=EDGE_CURVE ( 'NONE', #47264, #57839, #13637, .T. ) ;
#50418=CARTESIAN_POINT ( 'NONE',  ( 2.229367062499998831, -18.64583333196774007, -3.861377020970580887 ) ) ;
#50420=CARTESIAN_POINT ( 'NONE',  ( -5.000000000000000000, -99.00000000000000000, 0.000000000000000000 ) ) ;
#50422=CARTESIAN_POINT ( 'NONE',  ( -4.458734124999998549, -38.47916666530107221, 2.574251347313722516 ) ) ;
#50423=CARTESIAN_POINT ( 'NONE',  ( -2.499999999999996447, 7.291666669397852019, 4.330127018922195425 ) ) ;
#50428=CARTESIAN_POINT ( 'NONE',  ( 5.000000000000000000, -71.41666666666667140, -2.886751345948130876 ) ) ;
#50429=CYLINDRICAL_SURFACE ( 'NONE', #11015, 5.000000000000000000 ) ;
#50430=CARTESIAN_POINT ( 'NONE',  ( -2.229367062499996610, 0.6041666680322611560, 3.861377020970582219 ) ) ;
#50435=CARTESIAN_POINT ( 'NONE',  ( 2.229367062500001939, -88.97916666530106511, 3.861377020970579999 ) ) ;
#50436=CARTESIAN_POINT ( 'NONE',  ( -4.458734124999998549, -36.22916666530106511, 2.574251347313722516 ) ) ;
#50437=CARTESIAN_POINT ( 'NONE',  ( 2.500000000000002220, 27.33333333333333215, 4.330127018922192761 ) ) ;
#50438=CARTESIAN_POINT ( 'NONE',  ( 2.229367062499998831, -79.89583333196773651, -3.861377020970580887 ) ) ;
#50444=CARTESIAN_POINT ( 'NONE',  ( 9.457646018065525792E-16, -9.062499998634407916, 5.148502694627439702 ) ) ;
#50445=CARTESIAN_POINT ( 'NONE',  ( 4.458734124999998549, 20.02083333469892779, -2.574251347313721627 ) ) ;
#50446=CARTESIAN_POINT ( 'NONE',  ( -4.458734124999999437, -49.56249999863440792, 0.000000000000000000 ) ) ;
#50447=CARTESIAN_POINT ( 'NONE',  ( -5.000000000000000000, -45.95833333060214443, -2.886751345948128211 ) ) ;
#50454=CARTESIAN_POINT ( 'NONE',  ( -4.458734124999999437, -73.31249999863439371, 0.000000000000000000 ) ) ;
#50455=CARTESIAN_POINT ( 'NONE',  ( 2.229367062500001939, 27.77083333469892779, 3.861377020970579999 ) ) ;
#50457=CARTESIAN_POINT ( 'NONE',  ( 4.769696007084727185, -114.9999999999999858, 1.500000000000000000 ) ) ;
#50460=CARTESIAN_POINT ( 'NONE',  ( -4.999999999999999112, -61.91666666666665719, 2.886751345948131764 ) ) ;
#50461=CARTESIAN_POINT ( 'NONE',  ( -5.000000000000000000, -75.00000000000000000, 0.000000000000000000 ) ) ;
#50463=ORIENTED_EDGE ( 'NONE', *, *, #25966, .T. ) ;
#50469=VECTOR ( 'NONE', #6490, 1000.000000000000000 ) ;
#50474=FACE_OUTER_BOUND ( 'NONE', #51904, .T. ) ;
#50477=VERTEX_POINT ( 'NONE', #31425 ) ;
#50480=CARTESIAN_POINT ( 'NONE',  ( 4.458734124999998549, -47.97916666530107221, -2.574251347313721627 ) ) ;
#50487=CARTESIAN_POINT ( 'NONE',  ( -1.339745962155610925, 1.205341801261479828, 5.000000000000000000 ) ) ;
#50489=CARTESIAN_POINT ( 'NONE',  ( -4.458734124999998549, -95.47916666530106511, 2.574251347313722516 ) ) ;
#50495=CARTESIAN_POINT ( 'NONE',  ( 1.339745962155615144, -60.70534180126147561, 4.999999999999999112 ) ) ;
#50496=ORIENTED_EDGE ( 'NONE', *, *, #8730, .T. ) ;
#50497=CARTESIAN_POINT ( 'NONE',  ( 4.458734125000001214, -3.895833331967739621, 2.574251347313718519 ) ) ;
#50498=CARTESIAN_POINT ( 'NONE',  ( 1.339745962155615144, -50.58034179853029144, 4.999999999999999112 ) ) ;
#50499=CARTESIAN_POINT ( 'NONE',  ( 2.229367062500001939, -17.22916666530106866, 3.861377020970579999 ) ) ;
#50502=CARTESIAN_POINT ( 'NONE',  ( 2.500000000000002220, 23.45833333606451632, 4.330127018922192761 ) ) ;
#50504=CARTESIAN_POINT ( 'NONE',  ( 4.458734124999999437, 15.93750000136559564, -5.460374474430324690E-16 ) ) ;
#50508=CARTESIAN_POINT ( 'NONE',  ( 2.229367062499998831, -17.64583333196773651, -3.861377020970580887 ) ) ;
#50511=CARTESIAN_POINT ( 'NONE',  ( 1.339745962155615144, -3.705341801261480494, 4.999999999999999112 ) ) ;
#50512=( BOUNDED_CURVE ( )  B_SPLINE_CURVE ( 2, ( #2511, #56861, #32401, #12467, #41409, #7970, #12779, #47202, #37864 ),
 .UNSPECIFIED., .F., .T. ) 
 B_SPLINE_CURVE_WITH_KNOTS ( ( 3, 2, 2, 2, 3 ),
 ( 0.4910714285714285476, 0.4916666666666666408, 0.4928571428571428825, 0.4940476190476190688, 0.4946428571428571619 ),
 .UNSPECIFIED. ) 
 CURVE ( )  GEOMETRIC_REPRESENTATION_ITEM ( )  RATIONAL_B_SPLINE_CURVE ( ( 0.9330127018922194093, 0.9330127018922194093, 1.000000000000000000, 0.8660254037844387076, 1.000000000000000000, 0.8660254037844387076, 1.000000000000000000, 0.9330127018922194093, 0.9330127018922194093 ) ) 
 REPRESENTATION_ITEM ( '' )  );
#50514=ADVANCED_FACE ( 'NONE', ( #38390 ), #2196, .T. ) ;
#50515=CARTESIAN_POINT ( 'NONE',  ( 5.000000000000000000, -46.37499999726880873, -6.123233995736766282E-16 ) ) ;
#50517=CARTESIAN_POINT ( 'NONE',  ( 2.229367062500001939, 11.02083333469892956, 3.861377020970579999 ) ) ;
#50518=CARTESIAN_POINT ( 'NONE',  ( 6.158835246850666199E-14, 8.749999999999998224, -4.999999999999999112 ) ) ;
#50519=CARTESIAN_POINT ( 'NONE',  ( 0.000000000000000000, -120.0000000000000000, 0.000000000000000000 ) ) ;
#50521=CARTESIAN_POINT ( 'NONE',  ( 4.458734124999998549, -68.72916666530106511, -2.574251347313721627 ) ) ;
#50523=CARTESIAN_POINT ( 'NONE',  ( -5.000000000000000000, 1.999999999999998224, 0.000000000000000000 ) ) ;
#50525=CARTESIAN_POINT ( 'NONE',  ( -2.229367062499996610, -61.14583333196774362, 3.861377020970582219 ) ) ;
#50526=CARTESIAN_POINT ( 'NONE',  ( 5.000000000000000000, -96.37499999726881583, -6.123233995736766282E-16 ) ) ;
#50528=CARTESIAN_POINT ( 'NONE',  ( -1.339745962155610925, -79.79465819873850307, 5.000000000000000000 ) ) ;
#50531=CARTESIAN_POINT ( 'NONE',  ( 5.000000000000000000, -41.41666666666667140, -2.886751345948129988 ) ) ;
#50533=CARTESIAN_POINT ( 'NONE',  ( -6.972266317189433020E-16, -6.124999997268813168, -5.000000000000000000 ) ) ;
#50534=VERTEX_POINT ( 'NONE', #28426 ) ;
#50535=CARTESIAN_POINT ( 'NONE',  ( 2.229367062499998831, -107.6458333319677365, -3.861377020970580887 ) ) ;
#50536=CARTESIAN_POINT ( 'NONE',  ( 4.458734125000001214, -2.145833331967737845, 2.574251347313718519 ) ) ;
#50537=CARTESIAN_POINT ( 'NONE',  ( -5.000000000000000000, -96.95833333060213022, -2.886751345948128211 ) ) ;
#50543=CARTESIAN_POINT ( 'NONE',  ( 5.000000000000000000, -6.499999999999999112, -6.123233995736766282E-16 ) ) ;
#50546=CARTESIAN_POINT ( 'NONE',  ( 2.500000000000002220, -101.6666666666666572, 4.330127018922192761 ) ) ;
#50548=CARTESIAN_POINT ( 'NONE',  ( 4.458734125000001214, -28.14583333196774007, 2.574251347313718519 ) ) ;
#50558=CARTESIAN_POINT ( 'NONE',  ( -3.152548672688508926E-16, -77.81249999863440792, -5.148502694627439702 ) ) ;
#50561=CARTESIAN_POINT ( 'NONE',  ( -4.999999999999998224, -14.79166666393548546, 2.886751345948131764 ) ) ;
#50563=DIRECTION ( 'NONE',  ( -0.000000000000000000, 1.000000000000000000, -0.000000000000000000 ) ) ;
#50565=CARTESIAN_POINT ( 'NONE',  ( 4.458734125000001214, -5.145833331967740065, 2.574251347313718519 ) ) ;
#50568=CARTESIAN_POINT ( 'NONE',  ( -1.339745962155613812, 2.919658201469706782, -5.000000000000000000 ) ) ;
#50569=ORIENTED_EDGE ( 'NONE', *, *, #60987, .F. ) ;
#50570=DIRECTION ( 'NONE',  ( 0.8660254037844410391, -0.4999999999999958367, -0.000000000000000000 ) ) ;
#50574=CARTESIAN_POINT ( 'NONE',  ( 1.975475456537005874E-15, -105.7500000000000000, 5.000000000000000000 ) ) ;
#50576=CARTESIAN_POINT ( 'NONE',  ( -2.229367062499996610, -79.14583333196773651, 3.861377020970582219 ) ) ;
#50577=CARTESIAN_POINT ( 'NONE',  ( 2.500000000000002220, -29.54166666393548013, 4.330127018922192761 ) ) ;
#50578=CARTESIAN_POINT ( 'NONE',  ( 4.458734124999998549, -2.729166665301069550, -2.574251347313721627 ) ) ;
#50580=DIRECTION ( 'NONE',  ( -0.000000000000000000, 1.000000000000000000, -0.000000000000000000 ) ) ;
#50581=CARTESIAN_POINT ( 'NONE',  ( 4.458734124999998549, -69.97916666530107932, -2.574251347313721627 ) ) ;
#50582=CARTESIAN_POINT ( 'NONE',  ( -5.000000000000000000, -29.95833333060214088, -2.886751345948128211 ) ) ;
#50584=CARTESIAN_POINT ( 'NONE',  ( -5.000000000000000000, -0.8749999972688139449, 0.000000000000000000 ) ) ;
#50585=CARTESIAN_POINT ( 'NONE',  ( 1.975475456537005874E-15, -104.7500000000000000, 5.000000000000000000 ) ) ;
#50587=CARTESIAN_POINT ( 'NONE',  ( 9.457646018065525792E-16, -52.06249999863440792, 5.148502694627439702 ) ) ;
#50588=CARTESIAN_POINT ( 'NONE',  ( -3.152548672688508926E-16, -35.81249999863440792, -5.148502694627439702 ) ) ;
#50590=CARTESIAN_POINT ( 'NONE',  ( -4.999999999999998224, 9.208333336064519870, 2.886751345948131764 ) ) ;
#50591=CARTESIAN_POINT ( 'NONE',  ( -5.000000000000000000, 22.91666666666666430, -2.886751345948128211 ) ) ;
#50593=CARTESIAN_POINT ( 'NONE',  ( 5.000000000000000000, -26.37499999726881583, -6.123233995736766282E-16 ) ) ;
#50594=CARTESIAN_POINT ( 'NONE',  ( 2.229367062500001939, -41.97916666530107932, 3.861377020970579999 ) ) ;
#50595=CARTESIAN_POINT ( 'NONE',  ( -2.499999999999996447, -77.70833333060214443, 4.330127018922195425 ) ) ;
#50598=CARTESIAN_POINT ( 'NONE',  ( -3.152548672688508926E-16, -80.81249999863440792, -5.148502694627439702 ) ) ;
#50601=CARTESIAN_POINT ( 'NONE',  ( 1.060575238724906964E-15, -26.74999999999999645, 5.773502691896257311 ) ) ;
#50605=ORIENTED_EDGE ( 'NONE', *, *, #30207, .T. ) ;
#50606=CARTESIAN_POINT ( 'NONE',  ( 2.229367062499998831, 13.10416666803226171, -3.861377020970580887 ) ) ;
#50607=CARTESIAN_POINT ( 'NONE',  ( 5.000000000000000000, 17.62500000273118417, -6.123233995736766282E-16 ) ) ;
#50608=( BOUNDED_CURVE ( )  B_SPLINE_CURVE ( 2, ( #14884, #49937, #29039, #43518, #15542, #10064, #5565, #20365, #14565 ),
 .UNSPECIFIED., .F., .F. ) 
 B_SPLINE_CURVE_WITH_KNOTS ( ( 3, 2, 2, 2, 3 ),
 ( 0.5160714285714286254, 0.5166666666666667185, 0.5178571428571429047, 0.5190476190476190910, 0.5196428571428571841 ),
 .UNSPECIFIED. ) 
 CURVE ( )  GEOMETRIC_REPRESENTATION_ITEM ( )  RATIONAL_B_SPLINE_CURVE ( ( 0.9330127018922194093, 0.9330127018922256266, 1.000000000000000000, 0.8660254037844387076, 1.000000000000000000, 0.8660254037844387076, 1.000000000000000000, 0.9330127018922194093, 0.9330127018922194093 ) ) 
 REPRESENTATION_ITEM ( '' )  );
#50611=ADVANCED_FACE ( 'NONE', ( #42897 ), #31754, .T. ) ;
#50615=CARTESIAN_POINT ( 'NONE',  ( 1.975475456537005874E-15, -51.75000000000000000, 5.000000000000000000 ) ) ;
#50616=CARTESIAN_POINT ( 'NONE',  ( 5.000000000000000888, 15.54166666939785202, 2.886751345948126879 ) ) ;
#50617=CARTESIAN_POINT ( 'NONE',  ( 5.000000000000000000, -1.416666666666663410, -2.886751345948130876 ) ) ;
#50620=CARTESIAN_POINT ( 'NONE',  ( 2.500000000000002220, -74.66666666666665719, 4.330127018922192761 ) ) ;
#50622=CARTESIAN_POINT ( 'NONE',  ( -3.152548672688508926E-16, -12.81249999863440259, -5.148502694627439702 ) ) ;
#50626=MANIFOLD_SOLID_BREP ( 'Cut-Extrude1', #12032 ) ;
#50629=EDGE_CURVE ( 'NONE', #43493, #28751, #50608, .T. ) ;
#50631=ORIENTED_EDGE ( 'NONE', *, *, #33776, .F. ) ;
#50635=CARTESIAN_POINT ( 'NONE',  ( 5.000000000000000000, -103.4166666666666430, -2.886751345948130876 ) ) ;
#50637=VERTEX_POINT ( 'NONE', #53809 ) ;
#50638=CARTESIAN_POINT ( 'NONE',  ( -1.339745962155610925, -9.794658198738520838, 5.000000000000000000 ) ) ;
#50640=FACE_OUTER_BOUND ( 'NONE', #56179, .T. ) ;
#50643=DIRECTION ( 'NONE',  ( -0.000000000000000000, -1.000000000000000000, -0.000000000000000000 ) ) ;
#50644=CARTESIAN_POINT ( 'NONE',  ( 4.458734124999998549, 15.27083333469893134, -2.574251347313721627 ) ) ;
#50647=CARTESIAN_POINT ( 'NONE',  ( 1.339745962155615144, -77.70534180126146850, 4.999999999999999112 ) ) ;
#50648=CARTESIAN_POINT ( 'NONE',  ( 1.339745962155557191, -25.70534180126148271, 5.000000000000032863 ) ) ;
#50650=CARTESIAN_POINT ( 'NONE',  ( -2.229367062499996610, -63.14583333196774362, 3.861377020970582219 ) ) ;
#50652=CARTESIAN_POINT ( 'NONE',  ( 4.458734124999999437, 13.18750000136559208, -5.460374474430324690E-16 ) ) ;
#50653=CARTESIAN_POINT ( 'NONE',  ( 5.000000000000000000, 7.625000002731186832, -6.123233995736766282E-16 ) ) ;
#50655=CARTESIAN_POINT ( 'NONE',  ( 2.229367062500001939, -54.22916666530107221, 3.861377020970579999 ) ) ;
#50656=CARTESIAN_POINT ( 'NONE',  ( 2.500000000000002220, -15.54166666393548191, 4.330127018922192761 ) ) ;
#50657=DIRECTION ( 'NONE',  ( -0.000000000000000000, 1.000000000000000000, -0.000000000000000000 ) ) ;
#50659=CARTESIAN_POINT ( 'NONE',  ( -6.972266317189433020E-16, -64.12499999726880162, -5.000000000000000000 ) ) ;
#50660=CARTESIAN_POINT ( 'NONE',  ( 4.458734125000000326, -17.14583333196773651, 2.574251347313718519 ) ) ;
#50661=EDGE_LOOP ( 'NONE', ( #63534, #21702, #61723, #27607 ) ) ;
#50663=CARTESIAN_POINT ( 'NONE',  ( -4.458734124999999437, -103.3958333319677365, -2.574251347313719407 ) ) ;
#50666=CARTESIAN_POINT ( 'NONE',  ( 2.229367062500001939, -101.2291666653010651, 3.861377020970579999 ) ) ;
#50667=CARTESIAN_POINT ( 'NONE',  ( -4.458734124999998549, -25.22916666530106866, 2.574251347313722516 ) ) ;
#50668=CARTESIAN_POINT ( 'NONE',  ( 5.000000000000000888, -60.45833333060213732, 2.886751345948126879 ) ) ;
#50671=CARTESIAN_POINT ( 'NONE',  ( 9.457646018065525792E-16, -22.06249999863440436, 5.148502694627439702 ) ) ;
#50672=CARTESIAN_POINT ( 'NONE',  ( -2.229367062500000163, -64.72916666530106511, -3.861377020970580443 ) ) ;
#50676=CARTESIAN_POINT ( 'NONE',  ( -5.000000000000000000, -10.08333333333333393, -2.886751345948128211 ) ) ;
#50678=VERTEX_POINT ( 'NONE', #35162 ) ;
#50680=CARTESIAN_POINT ( 'NONE',  ( 5.000000000000000000, 21.70833333606451987, -2.886751345948130876 ) ) ;
#50683=EDGE_CURVE ( 'NONE', #11557, #3938, #24226, .T. ) ;
#50684=( BOUNDED_CURVE ( )  B_SPLINE_CURVE ( 2, ( #23977, #59345, #14321, #15277, #34245, #9488, #10131, #43581, #53874 ),
 .UNSPECIFIED., .F., .F. ) 
 B_SPLINE_CURVE_WITH_KNOTS ( ( 3, 2, 2, 2, 3 ),
 ( 0.9482142857142856762, 0.9488095238095237693, 0.9499999999999999556, 0.9511904761904761418, 0.9517857142857142350 ),
 .UNSPECIFIED. ) 
 CURVE ( )  GEOMETRIC_REPRESENTATION_ITEM ( )  RATIONAL_B_SPLINE_CURVE ( ( 0.9330127018922194093, 0.9330127018922194093, 1.000000000000000000, 0.8660254037844387076, 1.000000000000000000, 0.8660254037844387076, 1.000000000000000000, 0.9330127018922194093, 0.9330127018922194093 ) ) 
 REPRESENTATION_ITEM ( '' )  );
#50686=CARTESIAN_POINT ( 'NONE',  ( 2.499999999999998668, 1.791666669397853795, -4.330127018922193649 ) ) ;
#50688=CARTESIAN_POINT ( 'NONE',  ( 4.330127018922258486, 45.00000000000000000, 7.499999999999910294 ) ) ;
#50690=CARTESIAN_POINT ( 'NONE',  ( -5.000000000000000000, -82.00000000000000000, 0.000000000000000000 ) ) ;
#50694=ORIENTED_EDGE ( 'NONE', *, *, #34461, .T. ) ;
#50698=EDGE_CURVE ( 'NONE', #62517, #15325, #57200, .T. ) ;
#50700=ORIENTED_EDGE ( 'NONE', *, *, #53535, .T. ) ;
#50702=ADVANCED_FACE ( 'NONE', ( #59280 ), #10709, .F. ) ;
#50707=CYLINDRICAL_SURFACE ( 'NONE', #21045, 5.000000000000000000 ) ;
#50708=ORIENTED_EDGE ( 'NONE', *, *, #1208, .F. ) ;
#50712=VERTEX_POINT ( 'NONE', #29996 ) ;
#50713=CARTESIAN_POINT ( 'NONE',  ( 4.458734124999999437, -75.81249999863440792, -5.460374474430324690E-16 ) ) ;
#50714=CARTESIAN_POINT ( 'NONE',  ( -4.458734124999998549, -108.4791666653010793, 2.574251347313722516 ) ) ;
#50716=ORIENTED_EDGE ( 'NONE', *, *, #34251, .F. ) ;
#50721=CARTESIAN_POINT ( 'NONE',  ( -2.229367062500000163, -42.47916666530107932, -3.861377020970580443 ) ) ;
#50724=CARTESIAN_POINT ( 'NONE',  ( 4.458734125000000326, -47.89583333196774362, 2.574251347313718519 ) ) ;
#50728=CARTESIAN_POINT ( 'NONE',  ( 1.060575238724906964E-15, -103.7500000000000000, 5.773502691896257311 ) ) ;
#50730=CARTESIAN_POINT ( 'NONE',  ( 4.458734124999998549, -36.97916666530107221, -2.574251347313721627 ) ) ;
#50731=CARTESIAN_POINT ( 'NONE',  ( -4.999999999999999112, 0.2083333360645180099, 2.886751345948131764 ) ) ;
#50732=CARTESIAN_POINT ( 'NONE',  ( 5.000000000000000000, -50.41666666666666430, -2.886751345948130876 ) ) ;
#50735=CARTESIAN_POINT ( 'NONE',  ( -6.972266317189433020E-16, -71.25000000000000000, -5.000000000000000000 ) ) ;
#50736=CARTESIAN_POINT ( 'NONE',  ( 4.458734124999999437, -94.81249999863440792, -5.460374474430324690E-16 ) ) ;
#50738=CARTESIAN_POINT ( 'NONE',  ( -3.152548672688508926E-16, -1.812499998634406584, -5.148502694627439702 ) ) ;
#50739=EDGE_LOOP ( 'NONE', ( #29132, #30843, #13758, #20446 ) ) ;
#50742=CARTESIAN_POINT ( 'NONE',  ( 4.458734125000001214, -86.89583333196773651, 2.574251347313718519 ) ) ;
#50744=CARTESIAN_POINT ( 'NONE',  ( 4.458734124999999437, -87.06249999863439371, -5.460374474430324690E-16 ) ) ;
#50746=FACE_OUTER_BOUND ( 'NONE', #12806, .T. ) ;
#50747=AXIS2_PLACEMENT_3D ( 'NONE', #11067, #20730, #60294 ) ;
#50749=CARTESIAN_POINT ( 'NONE',  ( 9.457646018065525792E-16, -6.062499998634404363, 5.148502694627439702 ) ) ;
#50750=CARTESIAN_POINT ( 'NONE',  ( 2.229367062499998831, 19.10416666803225993, -3.861377020970580887 ) ) ;
#50751=CARTESIAN_POINT ( 'NONE',  ( 4.458734124999998549, -49.97916666530106511, -2.574251347313721627 ) ) ;
#50755=DIRECTION ( 'NONE',  ( -0.4999999999999948375, 0.000000000000000000, 0.8660254037844415942 ) ) ;
#50756=ORIENTED_EDGE ( 'NONE', *, *, #25650, .T. ) ;
#50760=CARTESIAN_POINT ( 'NONE',  ( 2.229367062499998831, -75.64583333196773651, -3.861377020970580887 ) ) ;
#50761=CARTESIAN_POINT ( 'NONE',  ( -3.152548672688508926E-16, 27.18750000136559564, -5.148502694627439702 ) ) ;
#50763=ADVANCED_FACE ( 'NONE', ( #9429 ), #19074, .T. ) ;
#50765=LINE ( 'NONE', #51408, #45126 ) ;
#50768=CARTESIAN_POINT ( 'NONE',  ( 1.060575238724906964E-15, -66.75000000000000000, 5.773502691896257311 ) ) ;
#50770=CARTESIAN_POINT ( 'NONE',  ( -2.499999999999996447, -74.83333333333332860, 4.330127018922195425 ) ) ;
#50773=CARTESIAN_POINT ( 'NONE',  ( 1.975475456537005874E-15, -72.62499999726878741, 5.000000000000000000 ) ) ;
#50775=CARTESIAN_POINT ( 'NONE',  ( -5.000000000000000000, -106.8749999972687874, 0.000000000000000000 ) ) ;
#50783=VERTEX_POINT ( 'NONE', #36616 ) ;
#50784=CARTESIAN_POINT ( 'NONE',  ( 0.000000000000000000, -120.0000000000000000, 0.000000000000000000 ) ) ;
#50786=EDGE_CURVE ( 'NONE', #40505, #4115, #30876, .T. ) ;
#50788=ORIENTED_EDGE ( 'NONE', *, *, #36142, .T. ) ;
#50792=CARTESIAN_POINT ( 'NONE',  ( 9.457646018065525792E-16, -47.31249999863440792, 5.148502694627439702 ) ) ;
#50796=ADVANCED_FACE ( 'NONE', ( #3794 ), #13435, .T. ) ;
#50802=VECTOR ( 'NONE', #34871, 1000.000000000000000 ) ;
#50803=CARTESIAN_POINT ( 'NONE',  ( -2.500000000000000444, -59.04166666393546592, -4.330127018922193649 ) ) ;
#50805=CARTESIAN_POINT ( 'NONE',  ( 2.229367062499998831, -93.89583333196772230, -3.861377020970580887 ) ) ;
#50811=CARTESIAN_POINT ( 'NONE',  ( -3.152548672688508926E-16, -1.562499998634406140, -5.148502694627439702 ) ) ;
#50812=CARTESIAN_POINT ( 'NONE',  ( 1.339745962155615144, -1.580341798530293662, 4.999999999999999112 ) ) ;
#50813=CARTESIAN_POINT ( 'NONE',  ( 4.458734124999998549, -23.97916666530107221, -2.574251347313721627 ) ) ;
#50815=LINE ( 'NONE', #12835, #33293 ) ;
#50817=LINE ( 'NONE', #41464, #50084 ) ;
#50819=CARTESIAN_POINT ( 'NONE',  ( 4.458734124999998549, 18.02083333469892779, -2.574251347313721627 ) ) ;
#50820=ORIENTED_EDGE ( 'NONE', *, *, #49097, .T. ) ;
#50822=CARTESIAN_POINT ( 'NONE',  ( -5.000000000000000000, -12.99999999999999822, 0.000000000000000000 ) ) ;
#50823=CARTESIAN_POINT ( 'NONE',  ( 2.500000000000002220, -86.66666666666667140, 4.330127018922192761 ) ) ;
#50824=CARTESIAN_POINT ( 'NONE',  ( -2.229367062499996610, -17.14583333196773651, 3.861377020970582219 ) ) ;
#50826=CARTESIAN_POINT ( 'NONE',  ( 5.000000000000000888, -3.583333333333333925, 2.886751345948126879 ) ) ;
#50828=CARTESIAN_POINT ( 'NONE',  ( -5.000000000000000000, -46.95833333060215153, -2.886751345948128211 ) ) ;
#50829=CARTESIAN_POINT ( 'NONE',  ( 1.339745962155615144, -24.70534180126147561, 4.999999999999999112 ) ) ;
#50830=CARTESIAN_POINT ( 'NONE',  ( -4.458734124999999437, 10.60416666803225993, -2.574251347313719407 ) ) ;
#50832=PRODUCT_DEFINITION ( 'UNKNOWN', '', #13310, #38600 ) ;
#50835=CARTESIAN_POINT ( 'NONE',  ( -4.458734124999998549, -68.22916666530107932, 2.574251347313722516 ) ) ;
#50837=CARTESIAN_POINT ( 'NONE',  ( 5.000000000000000888, 0.4166666666666659080, 2.886751345948126879 ) ) ;
#50839=CARTESIAN_POINT ( 'NONE',  ( -5.000000000000000000, 26.04166666939784847, -2.886751345948128211 ) ) ;
#50840=CARTESIAN_POINT ( 'NONE',  ( -4.458734124999999437, -61.39583333196774362, -2.574251347313719407 ) ) ;
#50841=CARTESIAN_POINT ( 'NONE',  ( -5.000000000000000000, -96.87499999726881583, 0.000000000000000000 ) ) ;
#50843=CARTESIAN_POINT ( 'NONE',  ( 5.000000000000000000, 5.625000002731185056, -6.123233995736766282E-16 ) ) ;
#50846=CARTESIAN_POINT ( 'NONE',  ( -1.339745962155497683, -91.08034179853028434, -5.000000000000066613 ) ) ;
#50847=CARTESIAN_POINT ( 'NONE',  ( -3.535250795749689387E-16, -49.25000000000000000, -5.773502691896257311 ) ) ;
#50848=LINE ( 'NONE', #55998, #55202 ) ;
#50849=CARTESIAN_POINT ( 'NONE',  ( -6.972266317189433020E-16, -108.2499999999999858, -5.000000000000000000 ) ) ;
#50850=VERTEX_POINT ( 'NONE', #14921 ) ;
#50851=CARTESIAN_POINT ( 'NONE',  ( 4.458734125000001214, -104.8958333319677365, 2.574251347313718519 ) ) ;
#50852=CARTESIAN_POINT ( 'NONE',  ( -2.229367062500000163, -2.729166665301069550, -3.861377020970580443 ) ) ;
#50860=CARTESIAN_POINT ( 'NONE',  ( -5.000000000000000000, 28.12500000273118417, 0.000000000000000000 ) ) ;
#50863=CARTESIAN_POINT ( 'NONE',  ( -2.500000000000000444, 24.83333333333333215, -4.330127018922193649 ) ) ;
#50865=ADVANCED_FACE ( 'NONE', ( #18260 ), #2851, .T. ) ;
#50866=EDGE_CURVE ( 'NONE', #4573, #51626, #11145, .T. ) ;
#50867=CARTESIAN_POINT ( 'NONE',  ( 4.458734125000001214, -30.14583333196773296, 2.574251347313718519 ) ) ;
#50870=EDGE_CURVE ( 'NONE', #2056, #34626, #35384, .T. ) ;
#50873=( BOUNDED_CURVE ( )  B_SPLINE_CURVE ( 2, ( #7086, #35077, #54697, #55344, #55010, #50826, #10618, #50511, #6763 ),
 .UNSPECIFIED., .F., .F. ) 
 B_SPLINE_CURVE_WITH_KNOTS ( ( 3, 2, 2, 2, 3 ),
 ( 0.2374999999999999889, 0.2380952380952380820, 0.2392857142857142960, 0.2404761904761904823, 0.2410714285714285754 ),
 .UNSPECIFIED. ) 
 CURVE ( )  GEOMETRIC_REPRESENTATION_ITEM ( )  RATIONAL_B_SPLINE_CURVE ( ( 0.9330127018922194093, 0.9330127018922194093, 1.000000000000000000, 0.8660254037844387076, 1.000000000000000000, 0.8660254037844387076, 1.000000000000000000, 0.9330127018922194093, 0.9330127018922194093 ) ) 
 REPRESENTATION_ITEM ( '' )  );
#50876=CARTESIAN_POINT ( 'NONE',  ( -1.339745962155610925, -93.66965819600733312, 5.000000000000000000 ) ) ;
#50878=CARTESIAN_POINT ( 'NONE',  ( -3.152548672688508926E-16, -80.81249999863440792, -5.148502694627439702 ) ) ;
#50880=ORIENTED_EDGE ( 'NONE', *, *, #36142, .F. ) ;
#50881=CYLINDRICAL_SURFACE ( 'NONE', #12139, 5.000000000000000000 ) ;
#50884=CARTESIAN_POINT ( 'NONE',  ( -4.458734124999999437, -10.56249999863440792, 0.000000000000000000 ) ) ;
#50886=CARTESIAN_POINT ( 'NONE',  ( -4.999999999999998224, -9.791666663935476578, 2.886751345948131764 ) ) ;
#50888=CARTESIAN_POINT ( 'NONE',  ( -6.031010364368858512E-14, 3.375000002731183280, 5.000000000000000000 ) ) ;
#50890=CARTESIAN_POINT ( 'NONE',  ( -2.229367062499996610, -6.395833331967741842, 3.861377020970582219 ) ) ;
#50892=CARTESIAN_POINT ( 'NONE',  ( -4.999999999999998224, -11.79166666393547835, 2.886751345948131764 ) ) ;
#50894=CYLINDRICAL_SURFACE ( 'NONE', #50172, 5.000000000000000000 ) ;
#50896=CARTESIAN_POINT ( 'NONE',  ( 2.229367062499998831, -84.64583333196773651, -3.861377020970580887 ) ) ;
#50897=CARTESIAN_POINT ( 'NONE',  ( 5.000000000000000000, -75.41666666666667140, -2.886751345948130876 ) ) ;
#50898=CARTESIAN_POINT ( 'NONE',  ( -4.458734124999999437, -5.312499998634402587, 0.000000000000000000 ) ) ;
#50900=CARTESIAN_POINT ( 'NONE',  ( 1.060575238724906964E-15, -30.62499999726881228, 5.773502691896257311 ) ) ;
#50902=CARTESIAN_POINT ( 'NONE',  ( -2.229367062499996610, 21.85416666803226349, 3.861377020970582219 ) ) ;
#50903=CARTESIAN_POINT ( 'NONE',  ( -2.499999999999996447, -55.83333333333332860, 4.330127018922195425 ) ) ;
#50905=CARTESIAN_POINT ( 'NONE',  ( 2.229367062500001939, -50.97916666530107221, 3.861377020970579999 ) ) ;
#50906=CARTESIAN_POINT ( 'NONE',  ( 2.229367062499998831, -37.89583333196773651, -3.861377020970580887 ) ) ;
#50908=CARTESIAN_POINT ( 'NONE',  ( -2.500000000000000444, -18.16666666666666430, -4.330127018922193649 ) ) ;
#50909=CARTESIAN_POINT ( 'NONE',  ( -4.999999999999999112, 17.08333333333333215, 2.886751345948131764 ) ) ;
#50911=DIRECTION ( 'NONE',  ( -0.000000000000000000, 1.000000000000000000, -0.000000000000000000 ) ) ;
#50912=CARTESIAN_POINT ( 'NONE',  ( 2.229367062499998831, -44.64583333196774362, -3.861377020970580887 ) ) ;
#50913=CARTESIAN_POINT ( 'NONE',  ( 2.499999999999998668, -77.20833333060214443, -4.330127018922193649 ) ) ;
#50915=DIRECTION ( 'NONE',  ( -0.000000000000000000, 1.000000000000000000, -0.000000000000000000 ) ) ;
#50917=CARTESIAN_POINT ( 'NONE',  ( -1.339745962155613812, -64.08034179853029855, -5.000000000000000000 ) ) ;
#50918=CARTESIAN_POINT ( 'NONE',  ( 4.458734124999999437, -87.06249999863439371, -5.460374474430324690E-16 ) ) ;
#50921=CARTESIAN_POINT ( 'NONE',  ( -5.000000000000000000, -26.08333333333333215, -2.886751345948128211 ) ) ;
#50924=AXIS2_PLACEMENT_3D ( 'NONE', #980, #20583, #50153 ) ;
#50926=VERTEX_POINT ( 'NONE', #22788 ) ;
#50927=CARTESIAN_POINT ( 'NONE',  ( 4.458734125000001214, -91.89583333196773651, 2.574251347313718519 ) ) ;
#50928=CARTESIAN_POINT ( 'NONE',  ( 2.229367062499998831, 12.10416666803226171, -3.861377020970580887 ) ) ;
#50929=CARTESIAN_POINT ( 'NONE',  ( -4.999999999999999112, 18.20833333606451987, 2.886751345948131764 ) ) ;
#50930=CARTESIAN_POINT ( 'NONE',  ( -1.339745962155613812, -61.08034179853027723, -5.000000000000000000 ) ) ;
#50938=CYLINDRICAL_SURFACE ( 'NONE', #1499, 5.000000000000000000 ) ;
#50942=( BOUNDED_CURVE ( )  B_SPLINE_CURVE ( 2, ( #46902, #27582, #61072, #32732, #52359, #56241, #52045, #2221, #42374 ),
 .UNSPECIFIED., .F., .F. ) 
 B_SPLINE_CURVE_WITH_KNOTS ( ( 3, 2, 2, 2, 3 ),
 ( 0.6589285714285714191, 0.6595238095238095122, 0.6607142857142856984, 0.6619047619047618847, 0.6624999999999999778 ),
 .UNSPECIFIED. ) 
 CURVE ( )  GEOMETRIC_REPRESENTATION_ITEM ( )  RATIONAL_B_SPLINE_CURVE ( ( 0.9330127018922194093, 0.9330127018922194093, 1.000000000000000000, 0.8660254037844387076, 1.000000000000000000, 0.8660254037844387076, 1.000000000000000000, 0.9330127018922194093, 0.9330127018922194093 ) ) 
 REPRESENTATION_ITEM ( '' )  );
#50943=CARTESIAN_POINT ( 'NONE',  ( 4.458734124999998549, -16.97916666530107221, -2.574251347313721627 ) ) ;
#50944=CARTESIAN_POINT ( 'NONE',  ( 5.000000000000000888, 17.54166666939785557, 2.886751345948126879 ) ) ;
#50952=CARTESIAN_POINT ( 'NONE',  ( 0.000000000000000000, -120.0000000000000000, 0.000000000000000000 ) ) ;
#50954=CARTESIAN_POINT ( 'NONE',  ( 4.458734125000001214, -63.14583333196774362, 2.574251347313718519 ) ) ;
#50956=CARTESIAN_POINT ( 'NONE',  ( 5.000000000000000888, -58.58333333333333570, 2.886751345948126879 ) ) ;
#50958=ORIENTED_EDGE ( 'NONE', *, *, #2070, .T. ) ;
#50959=CARTESIAN_POINT ( 'NONE',  ( -4.999999999999998224, -7.791666663935482795, 2.886751345948131764 ) ) ;
#50963=EDGE_LOOP ( 'NONE', ( #14539, #10409, #32430, #40061 ) ) ;
#50964=CARTESIAN_POINT ( 'NONE',  ( -4.330127018922205195, 45.00000000000000000, -7.499999999999943157 ) ) ;
#50965=CARTESIAN_POINT ( 'NONE',  ( -4.458734124999999437, 7.687500001365594748, 0.000000000000000000 ) ) ;
#50970=VECTOR ( 'NONE', #19102, 1000.000000000000000 ) ;
#50972=CARTESIAN_POINT ( 'NONE',  ( 2.229367062499998831, -71.64583333196773651, -3.861377020970580887 ) ) ;
#50973=CARTESIAN_POINT ( 'NONE',  ( 1.975475456537005874E-15, -49.62499999726880873, 5.000000000000000000 ) ) ;
#50974=CARTESIAN_POINT ( 'NONE',  ( 2.229367062499998831, 14.35416666803226171, -3.861377020970580887 ) ) ;
#50977=VECTOR ( 'NONE', #25333, 1000.000000000000000 ) ;
#50978=CARTESIAN_POINT ( 'NONE',  ( -6.972266317189433020E-16, -70.12499999726880162, -5.000000000000000000 ) ) ;
#50980=CARTESIAN_POINT ( 'NONE',  ( -2.229367062499996610, -54.39583333196773651, 3.861377020970582219 ) ) ;
#50981=CARTESIAN_POINT ( 'NONE',  ( -2.499999999999996447, -13.70833333060214976, 4.330127018922195425 ) ) ;
#50983=DIRECTION ( 'NONE',  ( -0.000000000000000000, 1.000000000000000000, -0.000000000000000000 ) ) ;
#50985=CARTESIAN_POINT ( 'NONE',  ( -2.229367062499996610, -21.39583333196774007, 3.861377020970582219 ) ) ;
#50989=CARTESIAN_POINT ( 'NONE',  ( -2.229367062500000163, -102.4791666653010651, -3.861377020970580443 ) ) ;
#50992=CARTESIAN_POINT ( 'NONE',  ( -4.458734124999998549, -105.4791666653010793, 2.574251347313722516 ) ) ;
#50993=CARTESIAN_POINT ( 'NONE',  ( 9.457646018065525792E-16, -26.06249999863440792, 5.148502694627439702 ) ) ;
#50994=CARTESIAN_POINT ( 'NONE',  ( -5.000000000000000000, -61.95833333060215153, -2.886751345948128211 ) ) ;
#50997=CARTESIAN_POINT ( 'NONE',  ( 4.458734124999998549, -21.72916666530107221, -2.574251347313721627 ) ) ;
#50998=CARTESIAN_POINT ( 'NONE',  ( -4.458734124999997661, -66.47916666530106511, 2.574251347313722516 ) ) ;
#51001=CARTESIAN_POINT ( 'NONE',  ( 0.000000000000000000, -120.0000000000000000, 5.000000000000000000 ) ) ;
#51003=CARTESIAN_POINT ( 'NONE',  ( 5.000000000000000000, -10.50000000000000178, -6.123233995736766282E-16 ) ) ;
#51007=CARTESIAN_POINT ( 'NONE',  ( -2.500000000000000444, -87.04166666393547303, -4.330127018922193649 ) ) ;
#51010=CARTESIAN_POINT ( 'NONE',  ( -6.972266317189433020E-16, 25.74999999999999645, -5.000000000000000000 ) ) ;
#51016=ORIENTED_EDGE ( 'NONE', *, *, #29647, .F. ) ;
#51017=CARTESIAN_POINT ( 'NONE',  ( -6.972266317189433020E-16, -80.12499999726881583, -5.000000000000000000 ) ) ;
#51023=AXIS2_PLACEMENT_3D ( 'NONE', #34580, #53582, #44556 ) ;
#51024=AXIS2_PLACEMENT_3D ( 'NONE', #25246, #35222, #34247 ) ;
#51026=ORIENTED_EDGE ( 'NONE', *, *, #29535, .F. ) ;
#51032=VERTEX_POINT ( 'NONE', #54812 ) ;
#51037=CARTESIAN_POINT ( 'NONE',  ( -4.458734124999999437, -76.39583333196775072, -2.574251347313719407 ) ) ;
#51038=CARTESIAN_POINT ( 'NONE',  ( 9.457646018065525792E-16, 28.93750000136559564, 5.148502694627439702 ) ) ;
#51039=CARTESIAN_POINT ( 'NONE',  ( -2.500000000000000444, -54.16666666666667140, -4.330127018922193649 ) ) ;
#51040=ORIENTED_EDGE ( 'NONE', *, *, #29028, .T. ) ;
#51041=CARTESIAN_POINT ( 'NONE',  ( -2.499999999999996447, 5.291666669397853795, 4.330127018922195425 ) ) ;
#51048=CARTESIAN_POINT ( 'NONE',  ( 2.229367062500001939, -48.97916666530107221, 3.861377020970579999 ) ) ;
#51051=EDGE_CURVE ( 'NONE', #22073, #33230, #17733, .T. ) ;
#51052=CARTESIAN_POINT ( 'NONE',  ( 5.000000000000000888, -108.5833333333333428, 2.886751345948126879 ) ) ;
#51054=CARTESIAN_POINT ( 'NONE',  ( 4.458734124999999437, -40.06249999863440081, -5.460374474430324690E-16 ) ) ;
#51055=CARTESIAN_POINT ( 'NONE',  ( 5.000000000000000000, 3.625000002731186388, -6.123233995736766282E-16 ) ) ;
#51059=CARTESIAN_POINT ( 'NONE',  ( 1.339745962155615144, -71.70534180126148271, 4.999999999999999112 ) ) ;
#51060=CARTESIAN_POINT ( 'NONE',  ( -4.458734124999999437, -98.39583333196773651, -2.574251347313719407 ) ) ;
#51061=CARTESIAN_POINT ( 'NONE',  ( -2.229367062500000163, -3.729166665301070438, -3.861377020970580443 ) ) ;
#51062=ORIENTED_EDGE ( 'NONE', *, *, #32208, .F. ) ;
#51064=CARTESIAN_POINT ( 'NONE',  ( -1.339745962155613812, -86.08034179853028434, -5.000000000000000000 ) ) ;
#51065=CARTESIAN_POINT ( 'NONE',  ( 4.458734125000001214, -88.89583333196773651, 2.574251347313718519 ) ) ;
#51066=CARTESIAN_POINT ( 'NONE',  ( 7.204675194429079505E-15, 27.74999999999999645, -5.000000000000000000 ) ) ;
#51067=CARTESIAN_POINT ( 'NONE',  ( -4.458734124999998549, -87.47916666530107932, 2.574251347313722516 ) ) ;
#51068=AXIS2_PLACEMENT_3D ( 'NONE', #1078, #50580, #15850 ) ;
#51071=AXIS2_PLACEMENT_3D ( 'NONE', #38927, #39241, #29590 ) ;
#51075=AXIS2_PLACEMENT_3D ( 'NONE', #33658, #43607, #23391 ) ;
#51076=CARTESIAN_POINT ( 'NONE',  ( -2.229367062500000163, -6.479166665301072214, -3.861377020970580443 ) ) ;
#51077=CARTESIAN_POINT ( 'NONE',  ( 2.229367062500001939, 17.77083333469892779, 3.861377020970579999 ) ) ;
#51079=CARTESIAN_POINT ( 'NONE',  ( 4.458734124999998549, -48.97916666530107221, -2.574251347313721627 ) ) ;
#51084=VERTEX_POINT ( 'NONE', #29709 ) ;
#51087=CARTESIAN_POINT ( 'NONE',  ( -2.229367062500000163, -79.47916666530106511, -3.861377020970580443 ) ) ;
#51088=CARTESIAN_POINT ( 'NONE',  ( -4.458734124999999437, 28.35416666803226349, -2.574251347313719407 ) ) ;
#51094=CARTESIAN_POINT ( 'NONE',  ( -4.999999999999999112, -66.91666666666667140, 2.886751345948131764 ) ) ;
#51104=EDGE_CURVE ( 'NONE', #15979, #14724, #15891, .T. ) ;
#51106=ORIENTED_EDGE ( 'NONE', *, *, #35831, .F. ) ;
#51113=CARTESIAN_POINT ( 'NONE',  ( -4.458734124999999437, -44.64583333196773651, -2.574251347313719407 ) ) ;
#51116=CARTESIAN_POINT ( 'NONE',  ( -5.000000000000000000, -21.95833333060214798, -2.886751345948128211 ) ) ;
#51118=AXIS2_PLACEMENT_3D ( 'NONE', #60956, #16877, #12045 ) ;
#51120=AXIS2_PLACEMENT_3D ( 'NONE', #7329, #26940, #34836 ) ;
#51125=CARTESIAN_POINT ( 'NONE',  ( -4.458734124999999437, -93.56249999863440792, 0.000000000000000000 ) ) ;
#51127=( BOUNDED_CURVE ( )  B_SPLINE_CURVE ( 2, ( #52271, #23005, #57420, #18483, #13655, #25198, #9446, #33586, #33895 ),
 .UNSPECIFIED., .F., .F. ) 
 B_SPLINE_CURVE_WITH_KNOTS ( ( 3, 2, 2, 2, 3 ),
 ( 0.04464285714285714385, 0.04523809523809523697, 0.04642857142857143016, 0.04761904761904761640, 0.04821428571428571647 ),
 .UNSPECIFIED. ) 
 CURVE ( )  GEOMETRIC_REPRESENTATION_ITEM ( )  RATIONAL_B_SPLINE_CURVE ( ( 0.9330127018922194093, 0.9330127018922194093, 1.000000000000000000, 0.8660254037844387076, 1.000000000000000000, 0.8660254037844387076, 1.000000000000000000, 0.9330127018922189652, 0.9330127018922194093 ) ) 
 REPRESENTATION_ITEM ( '' )  );
#51134=CARTESIAN_POINT ( 'NONE',  ( -4.458734124999999437, -0.3124999986344051406, 0.000000000000000000 ) ) ;
#51135=CARTESIAN_POINT ( 'NONE',  ( 2.229367062499998831, -95.89583333196773651, -3.861377020970580887 ) ) ;
#51139=CARTESIAN_POINT ( 'NONE',  ( -3.152548672688508926E-16, -21.81249999863440436, -5.148502694627439702 ) ) ;
#51140=CARTESIAN_POINT ( 'NONE',  ( 2.499999999999998668, -46.33333333333333570, -4.330127018922193649 ) ) ;
#51143=CARTESIAN_POINT ( 'NONE',  ( 1.339745962155619807, 23.83034180399266688, -4.999999999999996447 ) ) ;
#51145=CARTESIAN_POINT ( 'NONE',  ( 4.458734125000000326, 13.85416666803225993, 2.574251347313718519 ) ) ;
#51147=DIRECTION ( 'NONE',  ( -1.000000000000000000, 0.000000000000000000, 3.305092117221761110E-15 ) ) ;
#51149=CARTESIAN_POINT ( 'NONE',  ( -3.535250795749689387E-16, -83.25000000000000000, -5.773502691896257311 ) ) ;
#51150=CARTESIAN_POINT ( 'NONE',  ( 2.229367062499998831, -19.64583333196774007, -3.861377020970580887 ) ) ;
#51152=EDGE_CURVE ( 'NONE', #35992, #35135, #37834, .T. ) ;
#51155=CARTESIAN_POINT ( 'NONE',  ( -4.999999999999999112, -47.79166666393548013, 2.886751345948131764 ) ) ;
#51156=CARTESIAN_POINT ( 'NONE',  ( 5.000000000000000000, -41.37499999726880162, -6.123233995736766282E-16 ) ) ;
#51157=CARTESIAN_POINT ( 'NONE',  ( 4.458734124999998549, 8.270833334698926009, -2.574251347313721627 ) ) ;
#51159=EDGE_CURVE ( 'NONE', #42322, #14985, #48526, .T. ) ;
#51160=DIRECTION ( 'NONE',  ( 0.000000000000000000, 0.000000000000000000, 1.000000000000000000 ) ) ;
#51162=CARTESIAN_POINT ( 'NONE',  ( -4.458734124999999437, -67.31249999863440792, 0.000000000000000000 ) ) ;
#51164=CARTESIAN_POINT ( 'NONE',  ( 2.500000000000002220, -0.6666666666666660745, 4.330127018922192761 ) ) ;
#51167=CARTESIAN_POINT ( 'NONE',  ( 4.458734125000001214, -56.89583333196774362, 2.574251347313718519 ) ) ;
#51168=CARTESIAN_POINT ( 'NONE',  ( -5.000000000000000000, -92.95833333060215864, -2.886751345948128211 ) ) ;
#51171=CARTESIAN_POINT ( 'NONE',  ( 1.339745962155615144, -56.70534180126148271, 4.999999999999999112 ) ) ;
#51174=CARTESIAN_POINT ( 'NONE',  ( -4.999999999999999112, -50.91666666666667140, 2.886751345948131764 ) ) ;
#51175=CARTESIAN_POINT ( 'NONE',  ( 6.123233995736766282E-16, -120.0000000000000000, -5.000000000000000000 ) ) ;
#51178=CARTESIAN_POINT ( 'NONE',  ( 4.458734125000001214, -108.8958333319677365, 2.574251347313718519 ) ) ;
#51179=CARTESIAN_POINT ( 'NONE',  ( -4.458734124999999437, -1.562499998634406140, 0.000000000000000000 ) ) ;
#51184=CARTESIAN_POINT ( 'NONE',  ( -5.000000000000000000, -26.00000000000000355, 0.000000000000000000 ) ) ;
#51188=CARTESIAN_POINT ( 'NONE',  ( 5.000000000000000000, -22.29166666393548013, -2.886751345948130876 ) ) ;
#51194=CARTESIAN_POINT ( 'NONE',  ( 2.229367062499998831, -31.89583333196773651, -3.861377020970580887 ) ) ;
#51201=CARTESIAN_POINT ( 'NONE',  ( 5.000000000000000000, -83.29166666393547303, -2.886751345948130876 ) ) ;
#51203=CARTESIAN_POINT ( 'NONE',  ( 2.229367062500001939, -78.22916666530106511, 3.861377020970579999 ) ) ;
#51204=CARTESIAN_POINT ( 'NONE',  ( 1.339745962155586056, 3.294658198738519506, 5.000000000000015987 ) ) ;
#51206=CYLINDRICAL_SURFACE ( 'NONE', #59384, 5.000000000000000000 ) ;
#51207=VECTOR ( 'NONE', #57509, 1000.000000000000000 ) ;
#51210=CARTESIAN_POINT ( 'NONE',  ( -2.229367062499996610, -9.395833331967736513, 3.861377020970582219 ) ) ;
#51211=ORIENTED_EDGE ( 'NONE', *, *, #26009, .T. ) ;
#51213=EDGE_CURVE ( 'NONE', #13355, #2572, #41270, .T. ) ;
#51214=ORIENTED_EDGE ( 'NONE', *, *, #39188, .F. ) ;
#51215=CARTESIAN_POINT ( 'NONE',  ( 4.458734125000001214, -8.145833331967736513, 2.574251347313718519 ) ) ;
#51216=DIRECTION ( 'NONE',  ( 0.000000000000000000, 0.000000000000000000, 1.000000000000000000 ) ) ;
#51220=ADVANCED_FACE ( 'NONE', ( #55770 ), #2074, .T. ) ;
#51221=CARTESIAN_POINT ( 'NONE',  ( 1.339745962155612702, -75.16965819600731891, -5.000000000000000000 ) ) ;
#51223=CARTESIAN_POINT ( 'NONE',  ( 4.458734124999998549, -85.72916666530107932, -2.574251347313721627 ) ) ;
#51224=DIRECTION ( 'NONE',  ( -0.000000000000000000, 1.000000000000000000, -0.000000000000000000 ) ) ;
#51225=CARTESIAN_POINT ( 'NONE',  ( -4.458734124999999437, -3.395833331967739177, -2.574251347313719407 ) ) ;
#51228=CARTESIAN_POINT ( 'NONE',  ( -2.500000000000000444, -29.04166666393548013, -4.330127018922193649 ) ) ;
#51230=CARTESIAN_POINT ( 'NONE',  ( 9.457646018065525792E-16, 24.93750000136559208, 5.148502694627439702 ) ) ;
#51234=CARTESIAN_POINT ( 'NONE',  ( 4.458734124999998549, -52.72916666530107221, -2.574251347313721627 ) ) ;
#51235=CARTESIAN_POINT ( 'NONE',  ( -3.152548672688508926E-16, -38.81249999863440081, -5.148502694627439702 ) ) ;
#51238=CARTESIAN_POINT ( 'NONE',  ( -2.500000000000000444, 14.83333333333333215, -4.330127018922193649 ) ) ;
#51242=CARTESIAN_POINT ( 'NONE',  ( -4.458734124999998549, -45.22916666530106511, 2.574251347313722516 ) ) ;
#51243=CARTESIAN_POINT ( 'NONE',  ( 5.000000000000000000, -80.29166666393545881, -2.886751345948129988 ) ) ;
#51246=EDGE_CURVE ( 'NONE', #12673, #15879, #32946, .T. ) ;
#51247=CARTESIAN_POINT ( 'NONE',  ( 2.499999999999998668, -36.33333333333332860, -4.330127018922193649 ) ) ;
#51248=CARTESIAN_POINT ( 'NONE',  ( 2.229367062499998831, -87.89583333196773651, -3.861377020970580887 ) ) ;
#51250=DIRECTION ( 'NONE',  ( 0.000000000000000000, 0.000000000000000000, 1.000000000000000000 ) ) ;
#51251=CARTESIAN_POINT ( 'NONE',  ( 1.060575238724906964E-15, -33.75000000000000000, 5.773502691896257311 ) ) ;
#51253=ORIENTED_EDGE ( 'NONE', *, *, #46011, .T. ) ;
#51256=CARTESIAN_POINT ( 'NONE',  ( 2.229367062499998831, -89.64583333196773651, -3.861377020970580887 ) ) ;
#51257=CARTESIAN_POINT ( 'NONE',  ( -4.458734124999998549, 11.52083333469892779, 2.574251347313722516 ) ) ;
#51259=CARTESIAN_POINT ( 'NONE',  ( 5.000000000000000000, 15.62500000273118417, -6.123233995736766282E-16 ) ) ;
#51260=CARTESIAN_POINT ( 'NONE',  ( -5.000000000000000000, -60.00000000000000000, 0.000000000000000000 ) ) ;
#51266=CARTESIAN_POINT ( 'NONE',  ( 5.000000000000000000, -40.29166666393548013, -2.886751345948130876 ) ) ;
#51268=CARTESIAN_POINT ( 'NONE',  ( -5.000000000000000000, 18.04166666939785557, -2.886751345948128211 ) ) ;
#51272=CARTESIAN_POINT ( 'NONE',  ( 4.458734124999999437, -13.06249999863440259, -5.460374474430324690E-16 ) ) ;
#51279=( BOUNDED_CURVE ( )  B_SPLINE_CURVE ( 2, ( #6293, #20443, #5004, #30723, #5645, #25898, #40684, #195, #508 ),
 .UNSPECIFIED., .F., .F. ) 
 B_SPLINE_CURVE_WITH_KNOTS ( ( 3, 2, 2, 2, 3 ),
 ( 0.04464285714285714385, 0.04523809523809523697, 0.04642857142857143016, 0.04761904761904761640, 0.04821428571428571647 ),
 .UNSPECIFIED. ) 
 CURVE ( )  GEOMETRIC_REPRESENTATION_ITEM ( )  RATIONAL_B_SPLINE_CURVE ( ( 0.9330127018922194093, 0.9330127018922194093, 1.000000000000000000, 0.8660254037844387076, 1.000000000000000000, 0.8660254037844387076, 1.000000000000000000, 0.9330127018922189652, 0.9330127018922194093 ) ) 
 REPRESENTATION_ITEM ( '' )  );
#51281=VERTEX_POINT ( 'NONE', #9082 ) ;
#51282=CARTESIAN_POINT ( 'NONE',  ( 2.500000000000002220, -85.54166666393547303, 4.330127018922192761 ) ) ;
#51284=CARTESIAN_POINT ( 'NONE',  ( -4.458734124999999437, -60.64583333196774362, -2.574251347313719407 ) ) ;
#51286=CARTESIAN_POINT ( 'NONE',  ( 1.975475456537005874E-15, -103.7500000000000000, 5.000000000000000000 ) ) ;
#51288=ORIENTED_EDGE ( 'NONE', *, *, #54601, .F. ) ;
#51289=CARTESIAN_POINT ( 'NONE',  ( -2.499999999999996447, -7.708333330602144429, 4.330127018922195425 ) ) ;
#51295=CARTESIAN_POINT ( 'NONE',  ( 2.229367062499998831, 7.354166668032259935, -3.861377020970580887 ) ) ;
#51298=CARTESIAN_POINT ( 'NONE',  ( 1.339745962155729053, -78.16965819600734733, -4.999999999999933387 ) ) ;
#51302=CARTESIAN_POINT ( 'NONE',  ( 2.229367062499998831, -69.64583333196773651, -3.861377020970580887 ) ) ;
#51304=CARTESIAN_POINT ( 'NONE',  ( -4.458734124999999437, 12.60416666803225993, -2.574251347313719407 ) ) ;
#51306=CARTESIAN_POINT ( 'NONE',  ( 4.458734124999998549, -53.97916666530107221, -2.574251347313721627 ) ) ;
#51307=CARTESIAN_POINT ( 'NONE',  ( 5.000000000000000000, -15.29166666393548368, -2.886751345948129988 ) ) ;
#51308=CARTESIAN_POINT ( 'NONE',  ( -6.972266317189433020E-16, -33.12499999726880873, -5.000000000000000000 ) ) ;
#51311=CARTESIAN_POINT ( 'NONE',  ( -2.229367062499996610, -20.39583333196774007, 3.861377020970582219 ) ) ;
#51313=CARTESIAN_POINT ( 'NONE',  ( -8.660254037844341113, 45.00000000000000000, 6.047423072554883697E-14 ) ) ;
#51314=CARTESIAN_POINT ( 'NONE',  ( -3.535250795749689387E-16, 29.74999999999999645, -5.773502691896257311 ) ) ;
#51317=CARTESIAN_POINT ( 'NONE',  ( -4.458734124999999437, -100.5624999986344079, 0.000000000000000000 ) ) ;
#51318=CARTESIAN_POINT ( 'NONE',  ( -4.458734124999999437, -24.39583333196773651, -2.574251347313719407 ) ) ;
#51319=CARTESIAN_POINT ( 'NONE',  ( 5.000000000000000000, -60.29166666393546592, -2.886751345948129988 ) ) ;
#51322=CARTESIAN_POINT ( 'NONE',  ( -4.458734124999999437, -25.31249999863440792, 0.000000000000000000 ) ) ;
#51323=CARTESIAN_POINT ( 'NONE',  ( 9.457646018065525792E-16, -69.31249999863439371, 5.148502694627439702 ) ) ;
#51326=LINE ( 'NONE', #31360, #31744 ) ;
#51328=CARTESIAN_POINT ( 'NONE',  ( 5.000000000000000000, -19.41666666666666075, -2.886751345948129988 ) ) ;
#51332=( BOUNDED_CURVE ( )  B_SPLINE_CURVE ( 2, ( #56321, #8374, #47901, #8675, #37953, #41816, #61463, #27662, #28289 ),
 .UNSPECIFIED., .F., .F. ) 
 B_SPLINE_CURVE_WITH_KNOTS ( ( 3, 2, 2, 2, 3 ),
 ( 0.7232142857142856984, 0.7238095238095237915, 0.7249999999999999778, 0.7261904761904761640, 0.7267857142857142572 ),
 .UNSPECIFIED. ) 
 CURVE ( )  GEOMETRIC_REPRESENTATION_ITEM ( )  RATIONAL_B_SPLINE_CURVE ( ( 0.9330127018922194093, 0.9330127018922194093, 1.000000000000000000, 0.8660254037844387076, 1.000000000000000000, 0.8660254037844387076, 1.000000000000000000, 0.9330127018922194093, 0.9330127018922194093 ) ) 
 REPRESENTATION_ITEM ( '' )  );
#51334=CARTESIAN_POINT ( 'NONE',  ( 1.339745962155615144, -92.70534180126148271, 4.999999999999999112 ) ) ;
#51336=CARTESIAN_POINT ( 'NONE',  ( -6.972266317189433020E-16, -76.12499999726880162, -5.000000000000000000 ) ) ;
#51340=CARTESIAN_POINT ( 'NONE',  ( 6.123233995736766282E-16, -120.0000000000000000, -5.000000000000000000 ) ) ;
#51359=CARTESIAN_POINT ( 'NONE',  ( -5.000000000000000000, 20.91666666666666785, -2.886751345948128211 ) ) ;
#51361=CARTESIAN_POINT ( 'NONE',  ( 2.229367062499998831, -75.64583333196773651, -3.861377020970580887 ) ) ;
#51362=CARTESIAN_POINT ( 'NONE',  ( 9.457646018065525792E-16, 26.93750000136559564, 5.148502694627439702 ) ) ;
#51369=CARTESIAN_POINT ( 'NONE',  ( -6.972266317189433020E-16, -74.12499999726878741, -5.000000000000000000 ) ) ;
#51371=( BOUNDED_CURVE ( )  B_SPLINE_CURVE ( 2, ( #43900, #62297, #14012, #63548, #8567, #28178, #47794, #19468, #23373 ),
 .UNSPECIFIED., .F., .F. ) 
 B_SPLINE_CURVE_WITH_KNOTS ( ( 3, 2, 2, 2, 3 ),
 ( 0.4375000000000000000, 0.4380952380952380931, 0.4392857142857142794, 0.4404761904761904656, 0.4410714285714285587 ),
 .UNSPECIFIED. ) 
 CURVE ( )  GEOMETRIC_REPRESENTATION_ITEM ( )  RATIONAL_B_SPLINE_CURVE ( ( 0.9330127018922194093, 0.9330127018922194093, 1.000000000000000000, 0.8660254037844387076, 1.000000000000000000, 0.8660254037844387076, 1.000000000000000000, 0.9330127018922194093, 0.9330127018922194093 ) ) 
 REPRESENTATION_ITEM ( '' )  );
#51373=CARTESIAN_POINT ( 'NONE',  ( 4.458734125000000326, -56.89583333196774362, 2.574251347313718519 ) ) ;
#51375=CARTESIAN_POINT ( 'NONE',  ( 4.458734124999999437, 28.18750000136559208, -5.460374474430324690E-16 ) ) ;
#51376=CARTESIAN_POINT ( 'NONE',  ( -5.000000000000000000, -105.9999999999999858, 0.000000000000000000 ) ) ;
#51378=CARTESIAN_POINT ( 'NONE',  ( 9.457646018065525792E-16, -39.31249999863439371, 5.148502694627439702 ) ) ;
#51379=CARTESIAN_POINT ( 'NONE',  ( 5.000000000000000000, 3.708333336064517205, -2.886751345948129988 ) ) ;
#51384=CARTESIAN_POINT ( 'NONE',  ( -2.229367062499996610, -105.1458333319677365, 3.861377020970582219 ) ) ;
#51385=CARTESIAN_POINT ( 'NONE',  ( 4.458734125000000326, -7.145833331967736513, 2.574251347313718519 ) ) ;
#51389=CARTESIAN_POINT ( 'NONE',  ( 4.458734124999998549, -92.72916666530107932, -2.574251347313721627 ) ) ;
#51391=CARTESIAN_POINT ( 'NONE',  ( 4.458734125000001214, -85.14583333196773651, 2.574251347313718519 ) ) ;
#51393=CARTESIAN_POINT ( 'NONE',  ( 0.000000000000000000, -120.0000000000000000, 0.000000000000000000 ) ) ;
#51395=CARTESIAN_POINT ( 'NONE',  ( 4.458734124999998549, -7.729166665301073991, -2.574251347313721627 ) ) ;
#51396=CARTESIAN_POINT ( 'NONE',  ( -2.229367062499996610, 15.60416666803225993, 3.861377020970582219 ) ) ;
#51397=CARTESIAN_POINT ( 'NONE',  ( 9.457646018065525792E-16, -53.31249999863440792, 5.148502694627439702 ) ) ;
#51401=ORIENTED_EDGE ( 'NONE', *, *, #32316, .F. ) ;
#51404=CARTESIAN_POINT ( 'NONE',  ( 9.457646018065525792E-16, -81.06249999863440792, 5.148502694627439702 ) ) ;
#51405=CARTESIAN_POINT ( 'NONE',  ( 2.500000000000002220, -109.5416666639354730, 4.330127018922192761 ) ) ;
#51408=CARTESIAN_POINT ( 'NONE',  ( 0.000000000000000000, -120.0000000000000000, 5.000000000000000000 ) ) ;
#51411=CARTESIAN_POINT ( 'NONE',  ( 5.000000000000000000, -67.41666666666665719, -2.886751345948129988 ) ) ;
#51412=CARTESIAN_POINT ( 'NONE',  ( 0.000000000000000000, -120.0000000000000000, 0.000000000000000000 ) ) ;
#51416=CARTESIAN_POINT ( 'NONE',  ( -5.000000000000000000, 9.000000000000001776, 0.000000000000000000 ) ) ;
#51417=DIRECTION ( 'NONE',  ( -0.000000000000000000, 1.000000000000000000, -0.000000000000000000 ) ) ;
#51431=CARTESIAN_POINT ( 'NONE',  ( 2.229367062500001939, -54.22916666530107221, 3.861377020970579999 ) ) ;
#51432=CARTESIAN_POINT ( 'NONE',  ( -6.972266317189433020E-16, -24.24999999999999645, -5.000000000000000000 ) ) ;
#51444=CARTESIAN_POINT ( 'NONE',  ( -2.229367062500000163, -101.7291666653010651, -3.861377020970580443 ) ) ;
#51450=EDGE_CURVE ( 'NONE', #9796, #49029, #59243, .T. ) ;
#51451=CARTESIAN_POINT ( 'NONE',  ( -2.229367062499996610, -2.145833331967737845, 3.861377020970582219 ) ) ;
#51453=CARTESIAN_POINT ( 'NONE',  ( 2.229367062500001939, -96.22916666530105090, 3.861377020970579999 ) ) ;
#51455=CARTESIAN_POINT ( 'NONE',  ( -3.152548672688508926E-16, -20.81249999863440081, -5.148502694627439702 ) ) ;
#51461=CARTESIAN_POINT ( 'NONE',  ( 9.457646018065525792E-16, 8.687500001365595637, 5.148502694627439702 ) ) ;
#51463=CARTESIAN_POINT ( 'NONE',  ( 6.123233995736766282E-16, -120.0000000000000000, -5.000000000000000000 ) ) ;
#51465=CARTESIAN_POINT ( 'NONE',  ( 5.000000000000000888, -88.58333333333332860, 2.886751345948126879 ) ) ;
#51466=CARTESIAN_POINT ( 'NONE',  ( -4.458734124999999437, -25.39583333196773651, -2.574251347313719407 ) ) ;
#51470=EDGE_CURVE ( 'NONE', #9470, #40984, #2162, .T. ) ;
#51471=CARTESIAN_POINT ( 'NONE',  ( 1.060575238724906964E-15, -51.62499999726881583, 5.773502691896257311 ) ) ;
#51472=FACE_OUTER_BOUND ( 'NONE', #41818, .T. ) ;
#51473=CARTESIAN_POINT ( 'NONE',  ( 4.458734124999999437, 9.187500001365592084, -5.460374474430324690E-16 ) ) ;
#51477=CARTESIAN_POINT ( 'NONE',  ( -3.152548672688508926E-16, -68.56249999863439371, -5.148502694627439702 ) ) ;
#51479=CARTESIAN_POINT ( 'NONE',  ( 2.499999999999998668, -3.333333333333333925, -4.330127018922193649 ) ) ;
#51483=CARTESIAN_POINT ( 'NONE',  ( -2.229367062500000163, -63.47916666530106511, -3.861377020970580443 ) ) ;
#51484=CARTESIAN_POINT ( 'NONE',  ( -2.499999999999996447, -92.70833333060214443, 4.330127018922195425 ) ) ;
#51485=CARTESIAN_POINT ( 'NONE',  ( 2.500000000000002220, 5.458333336064518981, 4.330127018922192761 ) ) ;
#51489=CARTESIAN_POINT ( 'NONE',  ( 5.000000000000000000, -47.41666666666666430, -2.886751345948129988 ) ) ;
#51490=CARTESIAN_POINT ( 'NONE',  ( -5.000000000000000000, 26.91666666666666430, -2.886751345948128211 ) ) ;
#51493=CARTESIAN_POINT ( 'NONE',  ( 4.458734125000001214, -105.8958333319677365, 2.574251347313718519 ) ) ;
#51494=CARTESIAN_POINT ( 'NONE',  ( 4.458734124999998549, -0.9791666653010713262, -2.574251347313721627 ) ) ;
#51502=ORIENTED_EDGE ( 'NONE', *, *, #51152, .T. ) ;
#51510=CARTESIAN_POINT ( 'NONE',  ( 4.458734124999998549, -34.97916666530107221, -2.574251347313721627 ) ) ;
#51511=CARTESIAN_POINT ( 'NONE',  ( -5.000000000000000000, -10.95833333060214621, -2.886751345948128211 ) ) ;
#51520=CARTESIAN_POINT ( 'NONE',  ( 4.458734124999999437, -77.06249999863440792, -5.460374474430324690E-16 ) ) ;
#51521=ORIENTED_EDGE ( 'NONE', *, *, #24466, .T. ) ;
#51526=CARTESIAN_POINT ( 'NONE',  ( -2.229367062500000163, -6.729166665301073103, -3.861377020970580443 ) ) ;
#51529=CARTESIAN_POINT ( 'NONE',  ( 2.229367062499998831, -8.895833331967736513, -3.861377020970580887 ) ) ;
#51530=FACE_OUTER_BOUND ( 'NONE', #3904, .T. ) ;
#51532=CARTESIAN_POINT ( 'NONE',  ( 1.975475456537005874E-15, -78.62499999726881583, 5.000000000000000000 ) ) ;
#51534=CARTESIAN_POINT ( 'NONE',  ( 2.229367062500001939, 26.77083333469892423, 3.861377020970579999 ) ) ;
#51535=VERTEX_POINT ( 'NONE', #20321 ) ;
#51536=CARTESIAN_POINT ( 'NONE',  ( -4.458734124999999437, -86.31249999863439371, 0.000000000000000000 ) ) ;
#51538=CARTESIAN_POINT ( 'NONE',  ( 2.229367062499998831, -6.645833331967741842, -3.861377020970580887 ) ) ;
#51540=CARTESIAN_POINT ( 'NONE',  ( -2.499999999999996447, -32.70833333060215153, 4.330127018922195425 ) ) ;
#51542=CARTESIAN_POINT ( 'NONE',  ( 4.458734125000000326, 26.10416666803225993, 2.574251347313718519 ) ) ;
#51543=CARTESIAN_POINT ( 'NONE',  ( 1.339745962155615144, -7.705341801261480938, 4.999999999999999112 ) ) ;
#51545=CARTESIAN_POINT ( 'NONE',  ( 4.458734124999999437, -49.81249999863440792, -5.460374474430324690E-16 ) ) ;
#51546=CARTESIAN_POINT ( 'NONE',  ( 4.458734124999999437, -38.06249999863440792, -5.460374474430324690E-16 ) ) ;
#51550=CARTESIAN_POINT ( 'NONE',  ( 2.499999999999998668, 13.66666666666666785, -4.330127018922193649 ) ) ;
#51553=CARTESIAN_POINT ( 'NONE',  ( 9.457646018065525792E-16, -46.06249999863440081, 5.148502694627439702 ) ) ;
#51554=CARTESIAN_POINT ( 'NONE',  ( 5.000000000000000888, -77.45833333060213022, 2.886751345948126879 ) ) ;
#51556=CARTESIAN_POINT ( 'NONE',  ( 5.000000000000000888, -65.45833333060213022, 2.886751345948126879 ) ) ;
#51558=CARTESIAN_POINT ( 'NONE',  ( -4.458734124999999437, -84.56249999863439371, 0.000000000000000000 ) ) ;
#51560=CARTESIAN_POINT ( 'NONE',  ( -5.000000000000000000, -35.08333333333332149, -2.886751345948128211 ) ) ;
#51565=CARTESIAN_POINT ( 'NONE',  ( 2.229367062499998831, -90.64583333196773651, -3.861377020970580887 ) ) ;
#51566=CARTESIAN_POINT ( 'NONE',  ( 4.458734124999999437, 15.93750000136559564, -5.460374474430324690E-16 ) ) ;
#51567=CARTESIAN_POINT ( 'NONE',  ( -5.000000000000000000, 17.12500000273118417, 0.000000000000000000 ) ) ;
#51571=CARTESIAN_POINT ( 'NONE',  ( 1.975475456537005874E-15, -61.62499999726880873, 5.000000000000000000 ) ) ;
#51572=ADVANCED_FACE ( 'NONE', ( #34796 ), #10347, .T. ) ;
#51576=CARTESIAN_POINT ( 'NONE',  ( 1.975475456537005874E-15, -33.62499999726880873, 5.000000000000000000 ) ) ;
#51577=ADVANCED_FACE ( 'NONE', ( #54739 ), #5207, .T. ) ;
#51580=CARTESIAN_POINT ( 'NONE',  ( 1.339745962155612702, -96.29465819873851729, -5.000000000000000000 ) ) ;
#51582=CARTESIAN_POINT ( 'NONE',  ( 9.457646018065525792E-16, -14.31249999863440259, 5.148502694627439702 ) ) ;
#51589=ADVANCED_FACE ( 'NONE', ( #11752 ), #17225, .F. ) ;
#51594=EDGE_CURVE ( 'NONE', #38517, #9564, #7037, .T. ) ;
#51595=ORIENTED_EDGE ( 'NONE', *, *, #30003, .F. ) ;
#51596=CARTESIAN_POINT ( 'NONE',  ( -4.458734124999998549, -61.47916666530107221, 2.574251347313722516 ) ) ;
#51600=ORIENTED_EDGE ( 'NONE', *, *, #9724, .F. ) ;
#51602=EDGE_CURVE ( 'NONE', #17309, #43124, #37479, .T. ) ;
#51603=CARTESIAN_POINT ( 'NONE',  ( 1.975475456537005874E-15, 0.3750000027311862216, 5.000000000000000000 ) ) ;
#51608=CARTESIAN_POINT ( 'NONE',  ( -1.339745962155640457, 2.330341803992662886, 4.999999999999984901 ) ) ;
#51609=CARTESIAN_POINT ( 'NONE',  ( 4.458734125000001214, 7.104166668032259047, 2.574251347313718519 ) ) ;
#51612=CARTESIAN_POINT ( 'NONE',  ( 2.493747252781420335E-13, -77.25000000000001421, -5.000000000000000000 ) ) ;
#51615=CARTESIAN_POINT ( 'NONE',  ( -4.458734124999999437, -69.39583333196773651, -2.574251347313719407 ) ) ;
#51617=CARTESIAN_POINT ( 'NONE',  ( 4.458734125000001214, 13.10416666803226171, 2.574251347313718519 ) ) ;
#51619=CARTESIAN_POINT ( 'NONE',  ( 4.458734125000001214, -56.14583333196774362, 2.574251347313718519 ) ) ;
#51620=CARTESIAN_POINT ( 'NONE',  ( -3.535250795749689387E-16, -14.12499999726881050, -5.773502691896257311 ) ) ;
#51621=CARTESIAN_POINT ( 'NONE',  ( 0.000000000000000000, -120.0000000000000000, 0.000000000000000000 ) ) ;
#51622=CARTESIAN_POINT ( 'NONE',  ( 1.975475456537005874E-15, -44.62499999726880162, 5.000000000000000000 ) ) ;
#51623=CARTESIAN_POINT ( 'NONE',  ( 1.975475456537005874E-15, -65.74999999999998579, 5.000000000000000000 ) ) ;
#51624=CARTESIAN_POINT ( 'NONE',  ( 9.457646018065525792E-16, -33.06249999863440792, 5.148502694627439702 ) ) ;
#51625=CARTESIAN_POINT ( 'NONE',  ( -4.458734124999997661, -22.47916666530107221, 2.574251347313722516 ) ) ;
#51626=VERTEX_POINT ( 'NONE', #61621 ) ;
#51628=CARTESIAN_POINT ( 'NONE',  ( -4.458734124999999437, -107.3124999986343937, 0.000000000000000000 ) ) ;
#51631=CARTESIAN_POINT ( 'NONE',  ( 2.229367062500001939, -100.2291666653010651, 3.861377020970579999 ) ) ;
#51632=CARTESIAN_POINT ( 'NONE',  ( 9.457646018065525792E-16, -28.06249999863440081, 5.148502694627439702 ) ) ;
#51633=CARTESIAN_POINT ( 'NONE',  ( -5.000000000000000000, -62.87499999726880873, 0.000000000000000000 ) ) ;
#51637=CARTESIAN_POINT ( 'NONE',  ( 9.457646018065525792E-16, -29.06249999863440436, 5.148502694627439702 ) ) ;
#51638=CARTESIAN_POINT ( 'NONE',  ( 4.458734124999998549, -69.97916666530107932, -2.574251347313721627 ) ) ;
#51639=CARTESIAN_POINT ( 'NONE',  ( 5.000000000000000000, 8.500000000000000000, -6.123233995736766282E-16 ) ) ;
#51643=CARTESIAN_POINT ( 'NONE',  ( 2.500000000000002220, -14.66666666666666785, 4.330127018922192761 ) ) ;
#51649=CARTESIAN_POINT ( 'NONE',  ( 1.975475456537005874E-15, -78.74999999999998579, 5.000000000000000000 ) ) ;
#51660=CARTESIAN_POINT ( 'NONE',  ( -4.999999999999998224, -29.79166666393548013, 2.886751345948131764 ) ) ;
#51661=ORIENTED_EDGE ( 'NONE', *, *, #52384, .T. ) ;
#51665=VERTEX_POINT ( 'NONE', #22059 ) ;
#51671=CARTESIAN_POINT ( 'NONE',  ( -1.339745962155610925, -50.66965819600732601, 5.000000000000000000 ) ) ;
#51677=CARTESIAN_POINT ( 'NONE',  ( 2.229367062499998831, -76.64583333196773651, -3.861377020970580887 ) ) ;
#51678=CARTESIAN_POINT ( 'NONE',  ( 4.458734124999999437, 22.18750000136559564, -5.460374474430324690E-16 ) ) ;
#51679=VERTEX_POINT ( 'NONE', #55837 ) ;
#51680=CARTESIAN_POINT ( 'NONE',  ( -6.972266317189433020E-16, 9.875000002731185944, -5.000000000000000000 ) ) ;
#51687=CARTESIAN_POINT ( 'NONE',  ( -4.458734124999999437, -55.31249999863440081, 0.000000000000000000 ) ) ;
#51689=CARTESIAN_POINT ( 'NONE',  ( 9.457646018065525792E-16, 28.93750000136559564, 5.148502694627439702 ) ) ;
#51690=CARTESIAN_POINT ( 'NONE',  ( 1.060575238724906964E-15, -106.7499999999999716, 5.773502691896257311 ) ) ;
#51692=CARTESIAN_POINT ( 'NONE',  ( 9.457646018065525792E-16, -41.31249999863440081, 5.148502694627439702 ) ) ;
#51693=CARTESIAN_POINT ( 'NONE',  ( -3.535250795749689387E-16, 2.875000002731185944, -5.773502691896257311 ) ) ;
#51694=CARTESIAN_POINT ( 'NONE',  ( -1.230605004983934782E-13, -36.75000000000000711, 5.000000000000000000 ) ) ;
#51697=CARTESIAN_POINT ( 'NONE',  ( 1.975475456537005874E-15, 24.24999999999999645, 5.000000000000000000 ) ) ;
#51698=CARTESIAN_POINT ( 'NONE',  ( -3.152548672688508926E-16, -102.5624999986344079, -5.148502694627439702 ) ) ;
#51699=CARTESIAN_POINT ( 'NONE',  ( -4.458734124999997661, -5.479166665301072214, 2.574251347313722516 ) ) ;
#51700=( BOUNDED_CURVE ( )  B_SPLINE_CURVE ( 2, ( #47760, #19107, #4331, #9462, #49011, #52908, #19434, #29072, #48695 ),
 .UNSPECIFIED., .F., .F. ) 
 B_SPLINE_CURVE_WITH_KNOTS ( ( 3, 2, 2, 2, 3 ),
 ( 0.8339285714285714635, 0.8345238095238095566, 0.8357142857142857428, 0.8369047619047619291, 0.8375000000000000222 ),
 .UNSPECIFIED. ) 
 CURVE ( )  GEOMETRIC_REPRESENTATION_ITEM ( )  RATIONAL_B_SPLINE_CURVE ( ( 0.9330127018922194093, 0.9330127018922194093, 1.000000000000000000, 0.8660254037844387076, 1.000000000000000000, 0.8660254037844387076, 1.000000000000000000, 0.9330127018922194093, 0.9330127018922194093 ) ) 
 REPRESENTATION_ITEM ( '' )  );
#51701=EDGE_LOOP ( 'NONE', ( #15092, #37966, #43940, #38339 ) ) ;
#51703=CARTESIAN_POINT ( 'NONE',  ( -4.458734124999998549, -91.22916666530106511, 2.574251347313722516 ) ) ;
#51705=CARTESIAN_POINT ( 'NONE',  ( 2.229367062500001939, -88.22916666530107932, 3.861377020970579999 ) ) ;
#51709=CARTESIAN_POINT ( 'NONE',  ( -4.458734124999999437, -6.312499998634403475, 0.000000000000000000 ) ) ;
#51710=CARTESIAN_POINT ( 'NONE',  ( 2.229367062500001939, 15.77083333469892601, 3.861377020970579999 ) ) ;
#51711=CARTESIAN_POINT ( 'NONE',  ( 9.457646018065525792E-16, -54.31249999863440792, 5.148502694627439702 ) ) ;
#51716=ORIENTED_EDGE ( 'NONE', *, *, #48011, .T. ) ;
#51719=CARTESIAN_POINT ( 'NONE',  ( 2.500000000000002220, -68.66666666666667140, 4.330127018922192761 ) ) ;
#51720=CARTESIAN_POINT ( 'NONE',  ( 4.458734124999998549, -82.72916666530106511, -2.574251347313721627 ) ) ;
#51721=CARTESIAN_POINT ( 'NONE',  ( -2.229367062499996610, 22.60416666803225993, 3.861377020970582219 ) ) ;
#51723=VECTOR ( 'NONE', #33165, 1000.000000000000000 ) ;
#51725=EDGE_CURVE ( 'NONE', #50678, #22715, #57574, .T. ) ;
#51728=CARTESIAN_POINT ( 'NONE',  ( 5.000000000000000888, -63.58333333333332149, 2.886751345948126879 ) ) ;
#51729=DIRECTION ( 'NONE',  ( -0.000000000000000000, 1.000000000000000000, -0.000000000000000000 ) ) ;
#51732=CARTESIAN_POINT ( 'NONE',  ( 5.000000000000000000, -18.29166666393547658, -2.886751345948130876 ) ) ;
#51735=DIRECTION ( 'NONE',  ( -0.000000000000000000, 1.000000000000000000, -0.000000000000000000 ) ) ;
#51740=ORIENTED_EDGE ( 'NONE', *, *, #57023, .F. ) ;
#51743=ORIENTED_EDGE ( 'NONE', *, *, #35440, .F. ) ;
#51746=CARTESIAN_POINT ( 'NONE',  ( -2.229367062499996610, -49.39583333196772941, 3.861377020970582219 ) ) ;
#51749=ORIENTED_EDGE ( 'NONE', *, *, #60522, .T. ) ;
#51753=CARTESIAN_POINT ( 'NONE',  ( 1.464175926609780648E-14, 22.74999999999999645, -5.000000000000000000 ) ) ;
#51756=CARTESIAN_POINT ( 'NONE',  ( 4.458734124999998549, -99.97916666530106511, -2.574251347313721627 ) ) ;
#51757=DIRECTION ( 'NONE',  ( 0.000000000000000000, 0.000000000000000000, 1.000000000000000000 ) ) ;
#51758=ORIENTED_EDGE ( 'NONE', *, *, #27890, .T. ) ;
#51762=CARTESIAN_POINT ( 'NONE',  ( -4.458734124999999437, -5.395833331967740953, -2.574251347313719407 ) ) ;
#51763=CARTESIAN_POINT ( 'NONE',  ( 2.229367062499998831, -93.89583333196772230, -3.861377020970580887 ) ) ;
#51765=CARTESIAN_POINT ( 'NONE',  ( 4.458734124999998549, -20.97916666530107221, -2.574251347313721627 ) ) ;
#51769=CARTESIAN_POINT ( 'NONE',  ( -6.972266317189433020E-16, -66.24999999999998579, -5.000000000000000000 ) ) ;
#51772=CARTESIAN_POINT ( 'NONE',  ( 4.458734125000000326, 11.85416666803225993, 2.574251347313718519 ) ) ;
#51773=ORIENTED_EDGE ( 'NONE', *, *, #2726, .T. ) ;
#51774=CARTESIAN_POINT ( 'NONE',  ( 2.500000000000002220, -61.66666666666666430, 4.330127018922192761 ) ) ;
#51775=CARTESIAN_POINT ( 'NONE',  ( -2.499999999999996447, -88.83333333333332860, 4.330127018922195425 ) ) ;
#51776=CARTESIAN_POINT ( 'NONE',  ( -4.458734124999998549, -26.22916666530106866, 2.574251347313722516 ) ) ;
#51778=CARTESIAN_POINT ( 'NONE',  ( -3.152548672688508926E-16, -71.81249999863439371, -5.148502694627439702 ) ) ;
#51779=EDGE_CURVE ( 'NONE', #42402, #45642, #41342, .T. ) ;
#51784=CARTESIAN_POINT ( 'NONE',  ( -4.458734124999999437, 6.604166668032259935, -2.574251347313719407 ) ) ;
#51788=CARTESIAN_POINT ( 'NONE',  ( 9.457646018065525792E-16, -74.06249999863440792, 5.148502694627439702 ) ) ;
#51790=CARTESIAN_POINT ( 'NONE',  ( 5.000000000000000000, 0.5833333333333314830, -2.886751345948129988 ) ) ;
#51793=CARTESIAN_POINT ( 'NONE',  ( -4.458734124999999437, -66.39583333196773651, -2.574251347313719407 ) ) ;
#51794=CARTESIAN_POINT ( 'NONE',  ( 5.000000000000000888, -101.4583333306021586, 2.886751345948126879 ) ) ;
#51795=CARTESIAN_POINT ( 'NONE',  ( 1.975475456537005874E-15, 5.375000002731185944, 5.000000000000000000 ) ) ;
#51797=LINE ( 'NONE', #45700, #20477 ) ;
#51799=CARTESIAN_POINT ( 'NONE',  ( 5.000000000000000000, -46.41666666666666430, -2.886751345948129988 ) ) ;
#51801=ORIENTED_EDGE ( 'NONE', *, *, #42411, .F. ) ;
#51802=CARTESIAN_POINT ( 'NONE',  ( -2.229367062500000163, -109.4791666653010651, -3.861377020970580443 ) ) ;
#51803=DIRECTION ( 'NONE',  ( 0.000000000000000000, -1.000000000000000000, 0.000000000000000000 ) ) ;
#51806=DIRECTION ( 'NONE',  ( -0.000000000000000000, 1.000000000000000000, -0.000000000000000000 ) ) ;
#51810=CARTESIAN_POINT ( 'NONE',  ( -6.972266317189433020E-16, -100.1249999972688016, -5.000000000000000000 ) ) ;
#51816=CARTESIAN_POINT ( 'NONE',  ( -2.229367062499996610, -37.39583333196773651, 3.861377020970582219 ) ) ;
#51817=CARTESIAN_POINT ( 'NONE',  ( 5.000000000000000888, -10.58333333333333393, 2.886751345948126879 ) ) ;
#51826=CARTESIAN_POINT ( 'NONE',  ( 2.229367062499998831, -84.89583333196773651, -3.861377020970580887 ) ) ;
#51830=CARTESIAN_POINT ( 'NONE',  ( 0.000000000000000000, -120.0000000000000000, 5.000000000000000000 ) ) ;
#51832=CARTESIAN_POINT ( 'NONE',  ( -3.152548672688508926E-16, -36.56249999863441502, -5.148502694627439702 ) ) ;
#51833=CARTESIAN_POINT ( 'NONE',  ( -4.458734124999998549, -10.47916666530107044, 2.574251347313722516 ) ) ;
#51836=CYLINDRICAL_SURFACE ( 'NONE', #11144, 5.000000000000000000 ) ;
#51837=CARTESIAN_POINT ( 'NONE',  ( 4.458734125000001214, -5.145833331967740065, 2.574251347313718519 ) ) ;
#51842=CARTESIAN_POINT ( 'NONE',  ( -2.229367062499996610, 27.60416666803225993, 3.861377020970582219 ) ) ;
#51844=CARTESIAN_POINT ( 'NONE',  ( -2.229367062499996610, -86.14583333196773651, 3.861377020970582219 ) ) ;
#51845=CARTESIAN_POINT ( 'NONE',  ( -1.339745962155610925, -30.79465819873851373, 5.000000000000000000 ) ) ;
#51846=CARTESIAN_POINT ( 'NONE',  ( 2.229367062499998831, -10.64583333196773829, -3.861377020970580887 ) ) ;
#51847=EDGE_CURVE ( 'NONE', #11867, #44276, #8839, .T. ) ;
#51849=CARTESIAN_POINT ( 'NONE',  ( -6.972266317189433020E-16, -48.24999999999999289, -5.000000000000000000 ) ) ;
#51852=CARTESIAN_POINT ( 'NONE',  ( -5.000000000000000000, -37.95833333060214443, -2.886751345948128211 ) ) ;
#51853=DIRECTION ( 'NONE',  ( -0.000000000000000000, 1.000000000000000000, -0.000000000000000000 ) ) ;
#51854=CARTESIAN_POINT ( 'NONE',  ( -2.229367062500000163, 25.52083333469892779, -3.861377020970580443 ) ) ;
#51855=CARTESIAN_POINT ( 'NONE',  ( -5.000000000000000000, -3.999999999999996447, 0.000000000000000000 ) ) ;
#51857=CARTESIAN_POINT ( 'NONE',  ( -4.458734124999999437, -55.31249999863440081, 0.000000000000000000 ) ) ;
#51859=CARTESIAN_POINT ( 'NONE',  ( -5.000000000000000000, 9.125000002731184168, 0.000000000000000000 ) ) ;
#51860=CARTESIAN_POINT ( 'NONE',  ( 5.000000000000000888, 14.41666666666666785, 2.886751345948126879 ) ) ;
#51864=CARTESIAN_POINT ( 'NONE',  ( 2.229367062500001939, -46.97916666530106511, 3.861377020970579999 ) ) ;
#51865=CARTESIAN_POINT ( 'NONE',  ( -5.000000000000000000, -83.95833333060214443, -2.886751345948128211 ) ) ;
#51868=CARTESIAN_POINT ( 'NONE',  ( 5.000000000000000888, -36.58333333333332149, 2.886751345948126879 ) ) ;
#51869=EDGE_CURVE ( 'NONE', #22249, #61639, #33905, .T. ) ;
#51870=CARTESIAN_POINT ( 'NONE',  ( -4.458734124999997661, -86.47916666530107932, 2.574251347313722516 ) ) ;
#51872=( BOUNDED_CURVE ( )  B_SPLINE_CURVE ( 2, ( #12789, #43003, #37551, #8912, #48144, #43315, #38484, #63581, #5354 ),
 .UNSPECIFIED., .F., .F. ) 
 B_SPLINE_CURVE_WITH_KNOTS ( ( 3, 2, 2, 2, 3 ),
 ( 0.5553571428571428825, 0.5559523809523809756, 0.5571428571428571619, 0.5583333333333333481, 0.5589285714285714413 ),
 .UNSPECIFIED. ) 
 CURVE ( )  GEOMETRIC_REPRESENTATION_ITEM ( )  RATIONAL_B_SPLINE_CURVE ( ( 0.9330127018922194093, 0.9330127018922194093, 1.000000000000000000, 0.8660254037844387076, 1.000000000000000000, 0.8660254037844387076, 1.000000000000000000, 0.9330127018922194093, 0.9330127018922194093 ) ) 
 REPRESENTATION_ITEM ( '' )  );
#51873=CARTESIAN_POINT ( 'NONE',  ( -5.000000000000000000, -31.08333333333332860, -2.886751345948128211 ) ) ;
#51878=CARTESIAN_POINT ( 'NONE',  ( 2.229367062500001939, -95.97916666530105090, 3.861377020970579999 ) ) ;
#51879=CARTESIAN_POINT ( 'NONE',  ( -4.458734124999999437, 14.35416666803226171, -2.574251347313719407 ) ) ;
#51880=CARTESIAN_POINT ( 'NONE',  ( -5.000000000000000000, 19.04166666939785202, -2.886751345948128211 ) ) ;
#51881=LINE ( 'NONE', #61864, #18591 ) ;
#51885=CARTESIAN_POINT ( 'NONE',  ( -2.500000000000000444, -81.16666666666667140, -4.330127018922193649 ) ) ;
#51887=CARTESIAN_POINT ( 'NONE',  ( 1.339745962155615144, -40.58034179853029144, 4.999999999999999112 ) ) ;
#51888=CARTESIAN_POINT ( 'NONE',  ( -6.972266317189433020E-16, -63.25000000000000000, -5.000000000000000000 ) ) ;
#51891=CARTESIAN_POINT ( 'NONE',  ( 5.000000000000000000, -107.4166666666666430, -2.886751345948130876 ) ) ;
#51892=CARTESIAN_POINT ( 'NONE',  ( -5.000000000000000000, 13.91666666666666785, -2.886751345948128211 ) ) ;
#51893=CARTESIAN_POINT ( 'NONE',  ( -4.458734124999998549, -19.47916666530107221, 2.574251347313722516 ) ) ;
#51903=DIRECTION ( 'NONE',  ( 0.000000000000000000, 0.000000000000000000, 1.000000000000000000 ) ) ;
#51904=EDGE_LOOP ( 'NONE', ( #49668, #37736, #33289, #39623 ) ) ;
#51906=CARTESIAN_POINT ( 'NONE',  ( -2.229367062499996610, -65.39583333196773651, 3.861377020970582219 ) ) ;
#51907=CARTESIAN_POINT ( 'NONE',  ( 5.000000000000000000, -7.374999997268813168, -6.123233995736766282E-16 ) ) ;
#51908=VERTEX_POINT ( 'NONE', #38719 ) ;
#51914=CARTESIAN_POINT ( 'NONE',  ( -4.999999999999998224, -54.91666666666667140, 2.886751345948131764 ) ) ;
#51915=CARTESIAN_POINT ( 'NONE',  ( -2.229367062499996610, 8.854166668032261711, 3.861377020970582219 ) ) ;
#51918=CARTESIAN_POINT ( 'NONE',  ( 5.000000000000000000, -78.37499999726881583, -6.123233995736766282E-16 ) ) ;
#51922=CARTESIAN_POINT ( 'NONE',  ( -4.458734124999997661, -69.22916666530107932, 2.574251347313722516 ) ) ;
#51924=CARTESIAN_POINT ( 'NONE',  ( 4.458734124999998549, 6.270833334698928674, -2.574251347313721627 ) ) ;
#51925=EDGE_CURVE ( 'NONE', #59890, #53853, #39873, .T. ) ;
#51927=CARTESIAN_POINT ( 'NONE',  ( 9.457646018065525792E-16, -61.31249999863440792, 5.148502694627439702 ) ) ;
#51928=CARTESIAN_POINT ( 'NONE',  ( -2.500000000000000444, -18.04166666393547658, -4.330127018922193649 ) ) ;
#51930=DIRECTION ( 'NONE',  ( 0.000000000000000000, 0.000000000000000000, 1.000000000000000000 ) ) ;
#51932=CARTESIAN_POINT ( 'NONE',  ( -5.000000000000000000, -83.87499999726880162, 0.000000000000000000 ) ) ;
#51933=CARTESIAN_POINT ( 'NONE',  ( -4.458734124999999437, -36.39583333196772941, -2.574251347313719407 ) ) ;
#51934=CARTESIAN_POINT ( 'NONE',  ( -2.229367062499996610, -23.39583333196773651, 3.861377020970582219 ) ) ;
#51935=ORIENTED_EDGE ( 'NONE', *, *, #2413, .T. ) ;
#51937=CARTESIAN_POINT ( 'NONE',  ( -5.000000000000000000, 28.91666666666666430, -2.886751345948128211 ) ) ;
#51939=ORIENTED_EDGE ( 'NONE', *, *, #29898, .F. ) ;
#51940=CARTESIAN_POINT ( 'NONE',  ( -4.458734124999999437, -108.5624999986343937, 0.000000000000000000 ) ) ;
#51941=CARTESIAN_POINT ( 'NONE',  ( 9.457646018065525792E-16, -33.06249999863440792, 5.148502694627439702 ) ) ;
#51942=CARTESIAN_POINT ( 'NONE',  ( -2.499999999999996447, -60.70833333060214443, 4.330127018922195425 ) ) ;
#51944=AXIS2_PLACEMENT_3D ( 'NONE', #27314, #47561, #37592 ) ;
#51947=CARTESIAN_POINT ( 'NONE',  ( 4.458734124999998549, -30.72916666530107221, -2.574251347313721627 ) ) ;
#51949=CARTESIAN_POINT ( 'NONE',  ( 2.229367062499998831, -68.89583333196773651, -3.861377020970580887 ) ) ;
#51954=CARTESIAN_POINT ( 'NONE',  ( 1.060575238724906964E-15, -18.75000000000000000, 5.773502691896257311 ) ) ;
#51957=DIRECTION ( 'NONE',  ( 0.000000000000000000, 0.000000000000000000, 1.000000000000000000 ) ) ;
#51959=CARTESIAN_POINT ( 'NONE',  ( 2.500000000000002220, -84.54166666393547303, 4.330127018922192761 ) ) ;
#51960=CARTESIAN_POINT ( 'NONE',  ( -1.339745962155610925, -0.7946581987385198387, 5.000000000000000000 ) ) ;
#51969=DIRECTION ( 'NONE',  ( 0.000000000000000000, 0.000000000000000000, 1.000000000000000000 ) ) ;
#51971=CYLINDRICAL_SURFACE ( 'NONE', #30672, 5.000000000000000000 ) ;
#51986=CARTESIAN_POINT ( 'NONE',  ( 4.458734124999998549, -84.72916666530106511, -2.574251347313721627 ) ) ;
#51987=CARTESIAN_POINT ( 'NONE',  ( 4.458734124999998549, 25.27083333469892779, -2.574251347313721627 ) ) ;
#51988=DIRECTION ( 'NONE',  ( -0.000000000000000000, 1.000000000000000000, -0.000000000000000000 ) ) ;
#51995=FACE_OUTER_BOUND ( 'NONE', #14613, .T. ) ;
#51996=CARTESIAN_POINT ( 'NONE',  ( -6.031010364368858512E-14, 4.249999999999995559, 5.000000000000000000 ) ) ;
#51997=CARTESIAN_POINT ( 'NONE',  ( -4.458734124999999437, -54.39583333196773651, -2.574251347313719407 ) ) ;
#51998=APPLICATION_CONTEXT ( 'automotive_design' ) ;
#52000=CARTESIAN_POINT ( 'NONE',  ( 2.229367062500001939, 21.02083333469892779, 3.861377020970579999 ) ) ;
#52002=CARTESIAN_POINT ( 'NONE',  ( -4.999999999999999112, -105.9166666666666714, 2.886751345948131764 ) ) ;
#52005=CARTESIAN_POINT ( 'NONE',  ( 4.458734124999999437, -45.06249999863440081, -5.460374474430324690E-16 ) ) ;
#52006=CARTESIAN_POINT ( 'NONE',  ( 2.499999999999998668, 0.7916666693978530178, -4.330127018922193649 ) ) ;
#52010=CARTESIAN_POINT ( 'NONE',  ( 2.229367062499998831, -102.6458333319677365, -3.861377020970580887 ) ) ;
#52011=CARTESIAN_POINT ( 'NONE',  ( 4.458734124999998549, -5.979166665301071326, -2.574251347313721627 ) ) ;
#52014=CARTESIAN_POINT ( 'NONE',  ( 2.229367062499998831, -90.64583333196773651, -3.861377020970580887 ) ) ;
#52016=CARTESIAN_POINT ( 'NONE',  ( 4.458734124999998549, -85.97916666530107932, -2.574251347313721627 ) ) ;
#52018=CARTESIAN_POINT ( 'NONE',  ( 5.000000000000000888, -2.458333330602146205, 2.886751345948126879 ) ) ;
#52021=CARTESIAN_POINT ( 'NONE',  ( -4.458734124999997661, -10.22916666530106866, 2.574251347313722516 ) ) ;
#52022=CARTESIAN_POINT ( 'NONE',  ( 4.458734124999999437, 17.93750000136559208, -5.460374474430324690E-16 ) ) ;
#52023=CARTESIAN_POINT ( 'NONE',  ( -3.152548672688508926E-16, -54.81249999863440081, -5.148502694627439702 ) ) ;
#52025=CARTESIAN_POINT ( 'NONE',  ( -4.999999999999998224, -105.9166666666666572, 2.886751345948131764 ) ) ;
#52028=ADVANCED_FACE ( 'NONE', ( #43235 ), #23325, .T. ) ;
#52033=FACE_OUTER_BOUND ( 'NONE', #56710, .T. ) ;
#52034=CARTESIAN_POINT ( 'NONE',  ( 4.458734124999998549, -78.72916666530106511, -2.574251347313721627 ) ) ;
#52035=CARTESIAN_POINT ( 'NONE',  ( -2.229367062499996610, 26.60416666803225993, 3.861377020970582219 ) ) ;
#52037=AXIS2_PLACEMENT_3D ( 'NONE', #49542, #5483, #39882 ) ;
#52040=EDGE_CURVE ( 'NONE', #50678, #52441, #19657, .T. ) ;
#52044=CARTESIAN_POINT ( 'NONE',  ( -5.000000000000000000, -63.00000000000000000, 0.000000000000000000 ) ) ;
#52045=CARTESIAN_POINT ( 'NONE',  ( 2.500000000000002220, -63.54166666393547303, 4.330127018922192761 ) ) ;
#52047=ORIENTED_EDGE ( 'NONE', *, *, #13101, .T. ) ;
#52056=ORIENTED_EDGE ( 'NONE', *, *, #60053, .T. ) ;
#52057=CARTESIAN_POINT ( 'NONE',  ( -6.972266317189433020E-16, -28.25000000000000000, -5.000000000000000000 ) ) ;
#52059=ORIENTED_EDGE ( 'NONE', *, *, #2093, .T. ) ;
#52062=CARTESIAN_POINT ( 'NONE',  ( 9.457646018065525792E-16, -52.31249999863440792, 5.148502694627439702 ) ) ;
#52069=CYLINDRICAL_SURFACE ( 'NONE', #42642, 5.000000000000000000 ) ;
#52071=CARTESIAN_POINT ( 'NONE',  ( -4.458734124999999437, -100.6458333319677223, -2.574251347313719407 ) ) ;
#52073=ORIENTED_EDGE ( 'NONE', *, *, #48087, .T. ) ;
#52076=( BOUNDED_CURVE ( )  B_SPLINE_CURVE ( 2, ( #2073, #51580, #12006, #36148, #61554, #21990, #37108, #32262, #12338 ),
 .UNSPECIFIED., .F., .F. ) 
 B_SPLINE_CURVE_WITH_KNOTS ( ( 3, 2, 2, 2, 3 ),
 ( 0.9017857142857143016, 0.9023809523809523947, 0.9035714285714285809, 0.9047619047619047672, 0.9053571428571428603 ),
 .UNSPECIFIED. ) 
 CURVE ( )  GEOMETRIC_REPRESENTATION_ITEM ( )  RATIONAL_B_SPLINE_CURVE ( ( 0.9330127018922194093, 0.9330127018922194093, 1.000000000000000000, 0.8660254037844387076, 1.000000000000000000, 0.8660254037844387076, 1.000000000000000000, 0.9330127018922194093, 0.9330127018922194093 ) ) 
 REPRESENTATION_ITEM ( '' )  );
#52077=VECTOR ( 'NONE', #21458, 1000.000000000000000 ) ;
#52080=CARTESIAN_POINT ( 'NONE',  ( 4.458734124999999437, -5.812499998634403475, -5.460374474430324690E-16 ) ) ;
#52081=CARTESIAN_POINT ( 'NONE',  ( 4.458734124999998549, -94.97916666530106511, -2.574251347313721627 ) ) ;
#52083=CARTESIAN_POINT ( 'NONE',  ( 4.458734125000001214, -22.14583333196773296, 2.574251347313718519 ) ) ;
#52088=CARTESIAN_POINT ( 'NONE',  ( -6.972266317189433020E-16, 1.750000000000000444, -5.000000000000000000 ) ) ;
#52090=CARTESIAN_POINT ( 'NONE',  ( -4.458734124999999437, 9.354166668032261711, -2.574251347313719407 ) ) ;
#52091=VERTEX_POINT ( 'NONE', #58591 ) ;
#52094=CARTESIAN_POINT ( 'NONE',  ( -2.499999999999996447, -90.83333333333332860, 4.330127018922195425 ) ) ;
#52095=CARTESIAN_POINT ( 'NONE',  ( -4.458734124999999437, -24.31249999863440436, 0.000000000000000000 ) ) ;
#52096=CARTESIAN_POINT ( 'NONE',  ( 1.339745962155612702, -73.29465819873851729, -5.000000000000000000 ) ) ;
#52097=CARTESIAN_POINT ( 'NONE',  ( -4.458734124999998549, -71.47916666530107932, 2.574251347313722516 ) ) ;
#52100=CARTESIAN_POINT ( 'NONE',  ( 4.458734124999998549, 2.270833334698928230, -2.574251347313721627 ) ) ;
#52104=CARTESIAN_POINT ( 'NONE',  ( 2.229367062500001939, -70.97916666530107932, 3.861377020970579999 ) ) ;
#52106=CARTESIAN_POINT ( 'NONE',  ( 5.000000000000000000, 1.500000000000001332, -6.123233995736766282E-16 ) ) ;
#52109=CARTESIAN_POINT ( 'NONE',  ( 9.457646018065525792E-16, -62.06249999863440792, 5.148502694627439702 ) ) ;
#52110=CARTESIAN_POINT ( 'NONE',  ( -2.499999999999996447, -102.7083333306021444, 4.330127018922195425 ) ) ;
#52113=CARTESIAN_POINT ( 'NONE',  ( -4.458734124999997661, -106.4791666653010793, 2.574251347313722516 ) ) ;
#52115=CARTESIAN_POINT ( 'NONE',  ( -5.000000000000000000, -51.08333333333332860, -2.886751345948128211 ) ) ;
#52117=CARTESIAN_POINT ( 'NONE',  ( -6.000000000000000000, -114.9999999999999858, 1.499999999999999556 ) ) ;
#52119=CARTESIAN_POINT ( 'NONE',  ( 9.457646018065525792E-16, -110.0624999986343795, 5.148502694627439702 ) ) ;
#52121=CARTESIAN_POINT ( 'NONE',  ( -4.999999999999998224, -99.79166666393545881, 2.886751345948131764 ) ) ;
#52124=VECTOR ( 'NONE', #7108, 1000.000000000000000 ) ;
#52137=CARTESIAN_POINT ( 'NONE',  ( 2.229367062499998831, -37.89583333196773651, -3.861377020970580887 ) ) ;
#52138=CARTESIAN_POINT ( 'NONE',  ( -6.972266317189433020E-16, -11.12499999726881406, -5.000000000000000000 ) ) ;
#52141=CARTESIAN_POINT ( 'NONE',  ( -1.339745962155613812, -30.20534180126148271, -5.000000000000000000 ) ) ;
#52145=CARTESIAN_POINT ( 'NONE',  ( -5.000000000000000000, -24.87499999726881583, 0.000000000000000000 ) ) ;
#52146=CARTESIAN_POINT ( 'NONE',  ( -2.229367062500000163, -84.72916666530107932, -3.861377020970580443 ) ) ;
#52152=CARTESIAN_POINT ( 'NONE',  ( 2.229367062500001939, -7.229166665301073103, 3.861377020970579999 ) ) ;
#52155=FACE_OUTER_BOUND ( 'NONE', #35632, .T. ) ;
#52156=CARTESIAN_POINT ( 'NONE',  ( -3.152548672688508926E-16, -4.812499998634402587, -5.148502694627439702 ) ) ;
#52159=CARTESIAN_POINT ( 'NONE',  ( -2.500000000000000444, -12.04166666393547835, -4.330127018922193649 ) ) ;
#52161=CARTESIAN_POINT ( 'NONE',  ( 9.457646018065525792E-16, 27.68750000136559208, 5.148502694627439702 ) ) ;
#52163=CARTESIAN_POINT ( 'NONE',  ( -4.458734124999997661, -87.22916666530107932, 2.574251347313722516 ) ) ;
#52164=CARTESIAN_POINT ( 'NONE',  ( 9.457646018065525792E-16, -6.062499998634403475, 5.148502694627439702 ) ) ;
#52165=CARTESIAN_POINT ( 'NONE',  ( 6.123233995736766282E-16, -120.0000000000000000, -5.000000000000000000 ) ) ;
#52166=CARTESIAN_POINT ( 'NONE',  ( 2.499999999999998668, -48.33333333333332860, -4.330127018922193649 ) ) ;
#52168=CARTESIAN_POINT ( 'NONE',  ( 5.000000000000000000, -34.29166666393547303, -2.886751345948129988 ) ) ;
#52169=FACE_OUTER_BOUND ( 'NONE', #26415, .T. ) ;
#52170=CARTESIAN_POINT ( 'NONE',  ( -2.229367062500000163, 21.52083333469892779, -3.861377020970580443 ) ) ;
#52171=CYLINDRICAL_SURFACE ( 'NONE', #49948, 5.000000000000000000 ) ;
#52173=CARTESIAN_POINT ( 'NONE',  ( 9.457646018065525792E-16, -58.06249999863440081, 5.148502694627439702 ) ) ;
#52176=CARTESIAN_POINT ( 'NONE',  ( 2.499999999999998668, 15.66666666666666607, -4.330127018922193649 ) ) ;
#52178=CARTESIAN_POINT ( 'NONE',  ( -6.972266317189433020E-16, -46.24999999999999289, -5.000000000000000000 ) ) ;
#52179=CARTESIAN_POINT ( 'NONE',  ( -2.229367062499996610, -50.14583333196772941, 3.861377020970582219 ) ) ;
#52180=CARTESIAN_POINT ( 'NONE',  ( -5.000000000000000000, -82.95833333060213022, -2.886751345948128211 ) ) ;
#52184=CARTESIAN_POINT ( 'NONE',  ( -4.458734124999999437, -85.64583333196773651, -2.574251347313719407 ) ) ;
#52186=CARTESIAN_POINT ( 'NONE',  ( 1.060575238724906964E-15, -31.75000000000000000, 5.773502691896257311 ) ) ;
#52187=CARTESIAN_POINT ( 'NONE',  ( -2.499999999999996447, 24.16666666666666785, 4.330127018922195425 ) ) ;
#52191=CARTESIAN_POINT ( 'NONE',  ( 2.229367062499998831, -94.64583333196773651, -3.861377020970580887 ) ) ;
#52192=CARTESIAN_POINT ( 'NONE',  ( 9.457646018065525792E-16, 7.687500001365596525, 5.148502694627439702 ) ) ;
#52193=CARTESIAN_POINT ( 'NONE',  ( 5.000000000000000888, 11.54166666939785202, 2.886751345948126879 ) ) ;
#52194=CARTESIAN_POINT ( 'NONE',  ( -2.500000000000000444, -29.04166666393548013, -4.330127018922193649 ) ) ;
#52199=CARTESIAN_POINT ( 'NONE',  ( 2.499999999999998668, -80.33333333333332860, -4.330127018922193649 ) ) ;
#52201=CARTESIAN_POINT ( 'NONE',  ( 6.158835246850666199E-14, -3.124999997268815388, -4.999999999999999112 ) ) ;
#52202=DIRECTION ( 'NONE',  ( -0.000000000000000000, 1.000000000000000000, -0.000000000000000000 ) ) ;
#52207=CARTESIAN_POINT ( 'NONE',  ( 9.457646018065525792E-16, -22.31249999863440792, 5.148502694627439702 ) ) ;
#52208=AXIS2_PLACEMENT_3D ( 'NONE', #30137, #19542, #20187 ) ;
#52214=VECTOR ( 'NONE', #18639, 1000.000000000000000 ) ;
#52218=ORIENTED_EDGE ( 'NONE', *, *, #17254, .T. ) ;
#52221=CARTESIAN_POINT ( 'NONE',  ( 4.458734124999998549, -65.97916666530106511, -2.574251347313721627 ) ) ;
#52223=CYLINDRICAL_SURFACE ( 'NONE', #62592, 5.000000000000000000 ) ;
#52229=AXIS2_PLACEMENT_3D ( 'NONE', #4999, #49377, #54201 ) ;
#52231=CARTESIAN_POINT ( 'NONE',  ( -4.999999999999998224, 2.208333336064519870, 2.886751345948131764 ) ) ;
#52233=CARTESIAN_POINT ( 'NONE',  ( 2.229367062499998831, 8.354166668032261711, -3.861377020970580887 ) ) ;
#52239=CARTESIAN_POINT ( 'NONE',  ( -4.458734124999997661, -68.22916666530106511, 2.574251347313722516 ) ) ;
#52240=CARTESIAN_POINT ( 'NONE',  ( 1.339745962155615144, -10.58034179853029144, 4.999999999999999112 ) ) ;
#52241=CARTESIAN_POINT ( 'NONE',  ( -2.229367062500000163, 7.520833334698929562, -3.861377020970580443 ) ) ;
#52244=CARTESIAN_POINT ( 'NONE',  ( 4.458734124999999437, -59.06249999863440081, -5.460374474430324690E-16 ) ) ;
#52245=CARTESIAN_POINT ( 'NONE',  ( -2.499999999999996447, -20.70833333060214798, 4.330127018922195425 ) ) ;
#52249=( BOUNDED_CURVE ( )  B_SPLINE_CURVE ( 2, ( #37583, #26991, #61417, #26350, #7701, #31482, #61731, #27304, #46929 ),
 .UNSPECIFIED., .F., .F. ) 
 B_SPLINE_CURVE_WITH_KNOTS ( ( 3, 2, 2, 2, 3 ),
 ( 0.2303571428571428714, 0.2309523809523809645, 0.2321428571428571508, 0.2333333333333333370, 0.2339285714285714302 ),
 .UNSPECIFIED. ) 
 CURVE ( )  GEOMETRIC_REPRESENTATION_ITEM ( )  RATIONAL_B_SPLINE_CURVE ( ( 0.9330127018922194093, 0.9330127018922209636, 1.000000000000000000, 0.8660254037844387076, 1.000000000000000000, 0.8660254037844387076, 1.000000000000000000, 0.9330127018922194093, 0.9330127018922194093 ) ) 
 REPRESENTATION_ITEM ( '' )  );
#52250=CARTESIAN_POINT ( 'NONE',  ( 5.000000000000000000, -65.50000000000000000, -6.123233995736766282E-16 ) ) ;
#52251=CARTESIAN_POINT ( 'NONE',  ( 4.458734124999998549, -41.72916666530107932, -2.574251347313721627 ) ) ;
#52252=CARTESIAN_POINT ( 'NONE',  ( -2.229367062500000163, -21.72916666530107221, -3.861377020970580443 ) ) ;
#52253=( BOUNDED_CURVE ( )  B_SPLINE_CURVE ( 2, ( #2091, #45807, #30694, #26832, #59980, #1134, #20733, #15903, #16540 ),
 .UNSPECIFIED., .F., .F. ) 
 B_SPLINE_CURVE_WITH_KNOTS ( ( 3, 2, 2, 2, 3 ),
 ( 0.8267857142857142350, 0.8273809523809523281, 0.8285714285714286254, 0.8297619047619048116, 0.8303571428571429047 ),
 .UNSPECIFIED. ) 
 CURVE ( )  GEOMETRIC_REPRESENTATION_ITEM ( )  RATIONAL_B_SPLINE_CURVE ( ( 0.9330127018922194093, 0.9330127018922194093, 1.000000000000000000, 0.8660254037844387076, 1.000000000000000000, 0.8660254037844387076, 1.000000000000000000, 0.9330127018922194093, 0.9330127018922194093 ) ) 
 REPRESENTATION_ITEM ( '' )  );
#52254=VERTEX_POINT ( 'NONE', #23862 ) ;
#52256=CARTESIAN_POINT ( 'NONE',  ( 4.458734124999999437, -109.8124999986343937, -5.460374474430324690E-16 ) ) ;
#52258=EDGE_LOOP ( 'NONE', ( #70, #35602, #55936, #42777 ) ) ;
#52259=CARTESIAN_POINT ( 'NONE',  ( 2.229367062500001939, -108.2291666653010651, 3.861377020970579999 ) ) ;
#52261=CARTESIAN_POINT ( 'NONE',  ( 4.458734124999999437, -30.81249999863440436, -5.460374474430324690E-16 ) ) ;
#52262=CARTESIAN_POINT ( 'NONE',  ( 5.000000000000000000, -67.37499999726881583, -6.123233995736766282E-16 ) ) ;
#52265=EDGE_CURVE ( 'NONE', #24051, #37866, #53042, .T. ) ;
#52266=CARTESIAN_POINT ( 'NONE',  ( -4.458734124999997661, -29.22916666530107221, 2.574251347313722516 ) ) ;
#52267=CARTESIAN_POINT ( 'NONE',  ( -4.458734124999999437, -67.64583333196773651, -2.574251347313719407 ) ) ;
#52271=CARTESIAN_POINT ( 'NONE',  ( -6.972266317189433020E-16, 22.87500000273118417, -5.000000000000000000 ) ) ;
#52272=CARTESIAN_POINT ( 'NONE',  ( 2.499999999999998668, -15.33333333333333037, -4.330127018922193649 ) ) ;
#52275=CARTESIAN_POINT ( 'NONE',  ( -2.500000000000000444, -82.16666666666667140, -4.330127018922193649 ) ) ;
#52277=CARTESIAN_POINT ( 'NONE',  ( -5.000000000000000000, -2.958333330602146649, -2.886751345948128211 ) ) ;
#52278=CARTESIAN_POINT ( 'NONE',  ( 2.499999999999998668, -81.20833333060213022, -4.330127018922193649 ) ) ;
#52285=( BOUNDED_CURVE ( )  B_SPLINE_CURVE ( 2, ( #55745, #36123, #15222, #11662, #45130, #54791, #10720, #30327, #44483 ),
 .UNSPECIFIED., .F., .F. ) 
 B_SPLINE_CURVE_WITH_KNOTS ( ( 3, 2, 2, 2, 3 ),
 ( 0.3803571428571428381, 0.3809523809523809312, 0.3821428571428571175, 0.3833333333333333592, 0.3839285714285714524 ),
 .UNSPECIFIED. ) 
 CURVE ( )  GEOMETRIC_REPRESENTATION_ITEM ( )  RATIONAL_B_SPLINE_CURVE ( ( 0.9330127018922194093, 0.9330127018922194093, 1.000000000000000000, 0.8660254037844387076, 1.000000000000000000, 0.8660254037844387076, 1.000000000000000000, 0.9330127018922194093, 0.9330127018922194093 ) ) 
 REPRESENTATION_ITEM ( '' )  );
#52286=VERTEX_POINT ( 'NONE', #43777 ) ;
#52295=EDGE_CURVE ( 'NONE', #44414, #34309, #6278, .T. ) ;
#52303=CARTESIAN_POINT ( 'NONE',  ( -1.339745962155610925, -38.66965819600732601, 5.000000000000000000 ) ) ;
#52308=VERTEX_POINT ( 'NONE', #35106 ) ;
#52309=CARTESIAN_POINT ( 'NONE',  ( 2.229367062500001939, -84.97916666530107932, 3.861377020970579999 ) ) ;
#52310=ADVANCED_FACE ( 'NONE', ( #5828 ), #20306, .T. ) ;
#52311=CARTESIAN_POINT ( 'NONE',  ( -2.229367062500000163, 24.52083333469892779, -3.861377020970580443 ) ) ;
#52313=ORIENTED_EDGE ( 'NONE', *, *, #5512, .T. ) ;
#52314=CARTESIAN_POINT ( 'NONE',  ( 1.975475456537005874E-15, 14.25000000000000000, 5.000000000000000000 ) ) ;
#52320=CARTESIAN_POINT ( 'NONE',  ( 2.499999999999998668, -13.20833333060214976, -4.330127018922193649 ) ) ;
#52321=CARTESIAN_POINT ( 'NONE',  ( 4.458734124999999437, -55.81249999863440081, -5.460374474430324690E-16 ) ) ;
#52322=CARTESIAN_POINT ( 'NONE',  ( 1.975475456537005874E-15, 21.24999999999999289, 5.000000000000000000 ) ) ;
#52323=CARTESIAN_POINT ( 'NONE',  ( -3.152548672688508926E-16, 25.43750000136559208, -5.148502694627439702 ) ) ;
#52324=CARTESIAN_POINT ( 'NONE',  ( 5.000000000000000888, -107.5833333333333428, 2.886751345948126879 ) ) ;
#52325=CARTESIAN_POINT ( 'NONE',  ( -5.000000000000000000, -44.00000000000000000, 0.000000000000000000 ) ) ;
#52326=CARTESIAN_POINT ( 'NONE',  ( -4.458734124999999437, -42.64583333196773651, -2.574251347313719407 ) ) ;
#52327=CARTESIAN_POINT ( 'NONE',  ( -4.999999999999999112, -5.791666663935480130, 2.886751345948131764 ) ) ;
#52331=CARTESIAN_POINT ( 'NONE',  ( 2.229367062500001939, -100.9791666653010651, 3.861377020970579999 ) ) ;
#52332=CARTESIAN_POINT ( 'NONE',  ( 4.458734124999999437, -7.062499998634404363, -5.460374474430324690E-16 ) ) ;
#52334=DIRECTION ( 'NONE',  ( 0.000000000000000000, 0.000000000000000000, 1.000000000000000000 ) ) ;
#52335=CARTESIAN_POINT ( 'NONE',  ( 4.458734124999998549, -90.72916666530106511, -2.574251347313721627 ) ) ;
#52337=CARTESIAN_POINT ( 'NONE',  ( 2.229367062500001939, -93.22916666530106511, 3.861377020970579999 ) ) ;
#52341=CARTESIAN_POINT ( 'NONE',  ( 4.458734125000000326, -13.89583333196774007, 2.574251347313718519 ) ) ;
#52342=CARTESIAN_POINT ( 'NONE',  ( -3.152548672688508926E-16, 10.18750000136559564, -5.148502694627439702 ) ) ;
#52343=CARTESIAN_POINT ( 'NONE',  ( 2.229367062499998831, -54.89583333196773651, -3.861377020970580887 ) ) ;
#52345=CARTESIAN_POINT ( 'NONE',  ( -1.339745962155613812, -106.2053418012614685, -5.000000000000000000 ) ) ;
#52351=CYLINDRICAL_SURFACE ( 'NONE', #12120, 5.000000000000000000 ) ;
#52352=CARTESIAN_POINT ( 'NONE',  ( 2.229367062500001939, -80.97916666530106511, 3.861377020970579999 ) ) ;
#52353=CARTESIAN_POINT ( 'NONE',  ( 9.457646018065525792E-16, 21.68750000136559208, 5.148502694627439702 ) ) ;
#52356=CARTESIAN_POINT ( 'NONE',  ( -4.769696007084728073, -120.0000000000000000, -1.500000000000000000 ) ) ;
#52358=CARTESIAN_POINT ( 'NONE',  ( 5.000000000000000000, -71.50000000000000000, -6.123233995736766282E-16 ) ) ;
#52359=CARTESIAN_POINT ( 'NONE',  ( 5.000000000000000000, -63.37499999726880873, -6.123233995736766282E-16 ) ) ;
#52364=CARTESIAN_POINT ( 'NONE',  ( -2.480964764533239819E-13, -108.6249999972688016, 5.000000000000000000 ) ) ;
#52370=EDGE_CURVE ( 'NONE', #55212, #55214, #12470, .T. ) ;
#52375=ORIENTED_EDGE ( 'NONE', *, *, #43639, .F. ) ;
#52376=EDGE_CURVE ( 'NONE', #22588, #15620, #27684, .T. ) ;
#52379=CARTESIAN_POINT ( 'NONE',  ( 2.229367062500001939, -52.22916666530107221, 3.861377020970579999 ) ) ;
#52382=ORIENTED_EDGE ( 'NONE', *, *, #16773, .T. ) ;
#52384=EDGE_CURVE ( 'NONE', #7754, #45000, #58854, .T. ) ;
#52392=CARTESIAN_POINT ( 'NONE',  ( 2.229367062499998831, -97.89583333196773651, -3.861377020970580887 ) ) ;
#52394=ORIENTED_EDGE ( 'NONE', *, *, #50411, .F. ) ;
#52395=ADVANCED_FACE ( 'NONE', ( #17705 ), #62408, .T. ) ;
#52401=CARTESIAN_POINT ( 'NONE',  ( -4.999999999999998224, 1.208333336064518981, 2.886751345948131764 ) ) ;
#52402=CARTESIAN_POINT ( 'NONE',  ( -2.229367062500000163, -9.479166665301068662, -3.861377020970580443 ) ) ;
#52403=CARTESIAN_POINT ( 'NONE',  ( -4.458734124999997661, -95.47916666530106511, 2.574251347313722516 ) ) ;
#52406=CARTESIAN_POINT ( 'NONE',  ( 4.458734124999998549, -29.97916666530107577, -2.574251347313721627 ) ) ;
#52407=CARTESIAN_POINT ( 'NONE',  ( 1.975475456537005874E-15, -1.624999997268813834, 5.000000000000000000 ) ) ;
#52410=CARTESIAN_POINT ( 'NONE',  ( 5.000000000000000888, -21.45833333060214798, 2.886751345948126879 ) ) ;
#52411=CARTESIAN_POINT ( 'NONE',  ( 5.000000000000000000, -88.37499999726880162, -6.123233995736766282E-16 ) ) ;
#52413=CARTESIAN_POINT ( 'NONE',  ( 4.458734124999999437, 9.937500001365593860, -5.460374474430324690E-16 ) ) ;
#52416=CARTESIAN_POINT ( 'NONE',  ( -2.500000000000000444, -89.16666666666665719, -4.330127018922193649 ) ) ;
#52417=CARTESIAN_POINT ( 'NONE',  ( 4.458734124999998549, -25.72916666530107221, -2.574251347313721627 ) ) ;
#52419=CARTESIAN_POINT ( 'NONE',  ( -2.229367062500000163, -75.72916666530106511, -3.861377020970580443 ) ) ;
#52421=CARTESIAN_POINT ( 'NONE',  ( 5.000000000000000000, -79.29166666393547303, -2.886751345948130876 ) ) ;
#52423=CARTESIAN_POINT ( 'NONE',  ( -3.152548672688508926E-16, 1.437500001365596525, -5.148502694627439702 ) ) ;
#52424=CARTESIAN_POINT ( 'NONE',  ( -5.000000000000000000, -62.95833333060215153, -2.886751345948128211 ) ) ;
#52425=CARTESIAN_POINT ( 'NONE',  ( -6.972266317189433020E-16, 16.74999999999999645, -5.000000000000000000 ) ) ;
#52427=CARTESIAN_POINT ( 'NONE',  ( 2.229367062500001939, -73.97916666530106511, 3.861377020970579999 ) ) ;
#52429=CARTESIAN_POINT ( 'NONE',  ( -4.999999999999999112, -7.916666666666668739, 2.886751345948131764 ) ) ;
#52432=CARTESIAN_POINT ( 'NONE',  ( -2.229367062499996610, -64.14583333196773651, 3.861377020970582219 ) ) ;
#52433=CARTESIAN_POINT ( 'NONE',  ( 5.000000000000000888, -97.45833333060214443, 2.886751345948126879 ) ) ;
#52436=CARTESIAN_POINT ( 'NONE',  ( 2.499999999999998668, 9.791666669397850242, -4.330127018922193649 ) ) ;
#52437=CARTESIAN_POINT ( 'NONE',  ( 4.458734124999999437, -106.0624999986344221, -5.460374474430324690E-16 ) ) ;
#52439=CARTESIAN_POINT ( 'NONE',  ( 1.060575238724906964E-15, -53.74999999999998579, 5.773502691896257311 ) ) ;
#52441=VERTEX_POINT ( 'NONE', #7742 ) ;
#52448=CARTESIAN_POINT ( 'NONE',  ( -5.000000000000000000, -4.958333330602148870, -2.886751345948128211 ) ) ;
#52454=ORIENTED_EDGE ( 'NONE', *, *, #22790, .T. ) ;
#52458=CARTESIAN_POINT ( 'NONE',  ( -2.229367062499996610, -33.39583333196772941, 3.861377020970582219 ) ) ;
#52460=( BOUNDED_CURVE ( )  B_SPLINE_CURVE ( 2, ( #756, #30960, #5564, #26139, #29995, #45759, #10386, #1711, #20364 ),
 .UNSPECIFIED., .F., .F. ) 
 B_SPLINE_CURVE_WITH_KNOTS ( ( 3, 2, 2, 2, 3 ),
 ( 0.4767857142857143127, 0.4773809523809524058, 0.4785714285714285920, 0.4797619047619047783, 0.4803571428571428714 ),
 .UNSPECIFIED. ) 
 CURVE ( )  GEOMETRIC_REPRESENTATION_ITEM ( )  RATIONAL_B_SPLINE_CURVE ( ( 0.9330127018922194093, 0.9330127018922225179, 1.000000000000000000, 0.8660254037844387076, 1.000000000000000000, 0.8660254037844387076, 1.000000000000000000, 0.9330127018922194093, 0.9330127018922194093 ) ) 
 REPRESENTATION_ITEM ( '' )  );
#52466=CARTESIAN_POINT ( 'NONE',  ( 1.975475456537005874E-15, -24.62499999726881583, 5.000000000000000000 ) ) ;
#52467=CARTESIAN_POINT ( 'NONE',  ( 2.229367062500001939, -85.22916666530107932, 3.861377020970579999 ) ) ;
#52468=DIRECTION ( 'NONE',  ( -0.000000000000000000, 1.000000000000000000, -0.000000000000000000 ) ) ;
#52469=VERTEX_POINT ( 'NONE', #12870 ) ;
#52471=CARTESIAN_POINT ( 'NONE',  ( -6.972266317189433020E-16, -102.1249999972688158, -5.000000000000000000 ) ) ;
#52477=CARTESIAN_POINT ( 'NONE',  ( -1.339745962155610925, -1.794658198738520616, 5.000000000000000000 ) ) ;
#52478=CARTESIAN_POINT ( 'NONE',  ( -4.458734124999999437, -14.56249999863440436, 0.000000000000000000 ) ) ;
#52479=CARTESIAN_POINT ( 'NONE',  ( -4.999999999999998224, -34.91666666666666430, 2.886751345948131764 ) ) ;
#52481=CARTESIAN_POINT ( 'NONE',  ( -1.339745962155613812, -96.08034179853028434, -5.000000000000000000 ) ) ;
#52484=CARTESIAN_POINT ( 'NONE',  ( -3.152548672688508926E-16, 27.18750000136559564, -5.148502694627439702 ) ) ;
#52486=CARTESIAN_POINT ( 'NONE',  ( -4.458734124999999437, -94.39583333196773651, -2.574251347313719407 ) ) ;
#52488=CARTESIAN_POINT ( 'NONE',  ( -1.339745962155613812, -63.20534180126146850, -5.000000000000000000 ) ) ;
#52489=CARTESIAN_POINT ( 'NONE',  ( 4.458734124999999437, -8.812499998634406140, -5.460374474430324690E-16 ) ) ;
#52490=VECTOR ( 'NONE', #32015, 1000.000000000000000 ) ;
#52491=LINE ( 'NONE', #52165, #5700 ) ;
#52492=CARTESIAN_POINT ( 'NONE',  ( 2.500000000000002220, -48.66666666666666430, 4.330127018922192761 ) ) ;
#52494=CARTESIAN_POINT ( 'NONE',  ( -2.499999999999996447, -33.70833333060213732, 4.330127018922195425 ) ) ;
#52495=DIRECTION ( 'NONE',  ( -0.000000000000000000, 1.000000000000000000, -0.000000000000000000 ) ) ;
#52496=CARTESIAN_POINT ( 'NONE',  ( -4.458734124999999437, 16.60416666803225993, -2.574251347313719407 ) ) ;
#52498=CARTESIAN_POINT ( 'NONE',  ( -4.458734124999998549, -57.22916666530107932, 2.574251347313722516 ) ) ;
#52501=CARTESIAN_POINT ( 'NONE',  ( 2.499999999999998668, 11.66666666666666607, -4.330127018922193649 ) ) ;
#52504=CARTESIAN_POINT ( 'NONE',  ( -4.458734124999999437, -47.39583333196774362, -2.574251347313719407 ) ) ;
#52505=CARTESIAN_POINT ( 'NONE',  ( 2.500000000000002220, -83.54166666393547303, 4.330127018922192761 ) ) ;
#52507=CARTESIAN_POINT ( 'NONE',  ( 5.000000000000000000, -14.37499999726881228, -6.123233995736766282E-16 ) ) ;
#52508=CARTESIAN_POINT ( 'NONE',  ( -5.000000000000000000, -104.8749999972688158, 0.000000000000000000 ) ) ;
#52509=CARTESIAN_POINT ( 'NONE',  ( -4.458734124999997661, -90.47916666530106511, 2.574251347313722516 ) ) ;
#52511=CARTESIAN_POINT ( 'NONE',  ( 5.000000000000000000, -32.41666666666665719, -2.886751345948129988 ) ) ;
#52513=ORIENTED_EDGE ( 'NONE', *, *, #55150, .T. ) ;
#52515=ORIENTED_EDGE ( 'NONE', *, *, #44391, .T. ) ;
#52516=CARTESIAN_POINT ( 'NONE',  ( 2.229367062499998831, -96.64583333196773651, -3.861377020970580887 ) ) ;
#52517=CARTESIAN_POINT ( 'NONE',  ( 4.458734125000001214, 6.854166668032259935, 2.574251347313718519 ) ) ;
#52518=CARTESIAN_POINT ( 'NONE',  ( 5.000000000000000000, 13.62500000273118417, -6.123233995736766282E-16 ) ) ;
#52519=CARTESIAN_POINT ( 'NONE',  ( -6.972266317189433020E-16, -60.24999999999999289, -5.000000000000000000 ) ) ;
#52525=CARTESIAN_POINT ( 'NONE',  ( -2.500000000000000444, -26.04166666393547658, -4.330127018922193649 ) ) ;
#52526=DIRECTION ( 'NONE',  ( 0.000000000000000000, 0.000000000000000000, 1.000000000000000000 ) ) ;
#52529=CARTESIAN_POINT ( 'NONE',  ( 1.339745962155612702, 6.830341803992665994, -5.000000000000000000 ) ) ;
#52530=CARTESIAN_POINT ( 'NONE',  ( -4.458734124999999437, -21.64583333196774362, -2.574251347313719407 ) ) ;
#52538=ORIENTED_EDGE ( 'NONE', *, *, #50870, .T. ) ;
#52540=ORIENTED_EDGE ( 'NONE', *, *, #51602, .F. ) ;
#52541=CARTESIAN_POINT ( 'NONE',  ( -4.458734124999999437, -68.56249999863439371, 0.000000000000000000 ) ) ;
#52542=CARTESIAN_POINT ( 'NONE',  ( -1.975475456537005874E-15, 29.25000000000000000, 5.000000000000000000 ) ) ;
#52544=ORIENTED_EDGE ( 'NONE', *, *, #48439, .T. ) ;
#52548=CARTESIAN_POINT ( 'NONE',  ( -2.229367062499996610, 1.604166668032262155, 3.861377020970582219 ) ) ;
#52549=ORIENTED_EDGE ( 'NONE', *, *, #33419, .F. ) ;
#52550=CARTESIAN_POINT ( 'NONE',  ( 5.000000000000000888, -45.58333333333333570, 2.886751345948126879 ) ) ;
#52551=CARTESIAN_POINT ( 'NONE',  ( -3.152548672688508926E-16, 3.437500001365594748, -5.148502694627439702 ) ) ;
#52554=CARTESIAN_POINT ( 'NONE',  ( 1.339745962155612702, 16.70534180126147916, -5.000000000000000000 ) ) ;
#52556=ORIENTED_EDGE ( 'NONE', *, *, #36256, .T. ) ;
#52557=CARTESIAN_POINT ( 'NONE',  ( -2.229367062500000163, -77.47916666530106511, -3.861377020970580443 ) ) ;
#52559=CARTESIAN_POINT ( 'NONE',  ( 2.229367062500001939, 7.020833334698928674, 3.861377020970579999 ) ) ;
#52561=CARTESIAN_POINT ( 'NONE',  ( 4.458734124999999437, -58.06249999863440081, -5.460374474430324690E-16 ) ) ;
#52562=CARTESIAN_POINT ( 'NONE',  ( 1.060575238724906964E-15, -19.62499999726881583, 5.773502691896257311 ) ) ;
#52564=CARTESIAN_POINT ( 'NONE',  ( -6.972266317189433020E-16, -42.12499999726880873, -5.000000000000000000 ) ) ;
#52565=CARTESIAN_POINT ( 'NONE',  ( 1.975475456537005874E-15, 19.37500000273118772, 5.000000000000000000 ) ) ;
#52566=DIRECTION ( 'NONE',  ( -0.000000000000000000, 1.000000000000000000, -0.000000000000000000 ) ) ;
#52568=CARTESIAN_POINT ( 'NONE',  ( -3.152548672688508926E-16, -38.56249999863439371, -5.148502694627439702 ) ) ;
#52569=CARTESIAN_POINT ( 'NONE',  ( 2.229367062500001939, -27.22916666530106866, 3.861377020970579999 ) ) ;
#52571=CARTESIAN_POINT ( 'NONE',  ( 2.499999999999998668, 25.66666666666666430, -4.330127018922193649 ) ) ;
#52574=CARTESIAN_POINT ( 'NONE',  ( -2.229367062499996610, -106.3958333319677365, 3.861377020970582219 ) ) ;
#52576=CARTESIAN_POINT ( 'NONE',  ( 4.458734125000001214, -29.89583333196773651, 2.574251347313718519 ) ) ;
#52577=CARTESIAN_POINT ( 'NONE',  ( -3.535250795749689387E-16, -70.12499999726880162, -5.773502691896257311 ) ) ;
#52581=CARTESIAN_POINT ( 'NONE',  ( -4.458734124999997661, -30.22916666530106866, 2.574251347313722516 ) ) ;
#52582=CARTESIAN_POINT ( 'NONE',  ( 2.229367062499998831, -73.89583333196773651, -3.861377020970580887 ) ) ;
#52586=CARTESIAN_POINT ( 'NONE',  ( 2.500000000000002220, -18.66666666666666430, 4.330127018922192761 ) ) ;
#52588=ORIENTED_EDGE ( 'NONE', *, *, #4795, .F. ) ;
#52591=CARTESIAN_POINT ( 'NONE',  ( 5.000000000000000888, 25.54166666939784847, 2.886751345948126879 ) ) ;
#52595=CARTESIAN_POINT ( 'NONE',  ( -6.972266317189433020E-16, -45.12499999726880162, -5.000000000000000000 ) ) ;
#52599=CARTESIAN_POINT ( 'NONE',  ( 0.000000000000000000, -120.0000000000000000, 5.000000000000000000 ) ) ;
#52608=CARTESIAN_POINT ( 'NONE',  ( 5.000000000000000888, -34.58333333333332860, 2.886751345948126879 ) ) ;
#52610=CARTESIAN_POINT ( 'NONE',  ( 0.000000000000000000, -120.0000000000000000, 0.000000000000000000 ) ) ;
#52613=ORIENTED_EDGE ( 'NONE', *, *, #29018, .T. ) ;
#52614=CARTESIAN_POINT ( 'NONE',  ( -2.229367062499996610, -83.14583333196773651, 3.861377020970582219 ) ) ;
#52615=CARTESIAN_POINT ( 'NONE',  ( 4.458734124999998549, 23.27083333469892423, -2.574251347313721627 ) ) ;
#52616=CARTESIAN_POINT ( 'NONE',  ( -2.499999999999996447, -17.70833333060214443, 4.330127018922195425 ) ) ;
#52623=CARTESIAN_POINT ( 'NONE',  ( -6.972266317189433020E-16, 2.875000002731185500, -5.000000000000000000 ) ) ;
#52626=CARTESIAN_POINT ( 'NONE',  ( -2.229367062500000163, -60.47916666530106511, -3.861377020970580443 ) ) ;
#52628=CARTESIAN_POINT ( 'NONE',  ( 4.458734124999998549, 21.27083333469892779, -2.574251347313721627 ) ) ;
#52630=CARTESIAN_POINT ( 'NONE',  ( -4.999999999999998224, -43.91666666666665719, 2.886751345948131764 ) ) ;
#52631=CARTESIAN_POINT ( 'NONE',  ( -2.229367062500000163, -42.72916666530107932, -3.861377020970580443 ) ) ;
#52632=CARTESIAN_POINT ( 'NONE',  ( 2.500000000000002220, -6.541666663935481019, 4.330127018922192761 ) ) ;
#52636=CARTESIAN_POINT ( 'NONE',  ( -3.152548672688508926E-16, -104.5624999986343937, -5.148502694627439702 ) ) ;
#52637=CARTESIAN_POINT ( 'NONE',  ( -2.229367062499996610, -8.395833331967736513, 3.861377020970582219 ) ) ;
#52640=CARTESIAN_POINT ( 'NONE',  ( -4.458734124999998549, -93.22916666530107932, 2.574251347313722516 ) ) ;
#52642=CARTESIAN_POINT ( 'NONE',  ( -4.458734124999999437, -94.56249999863440792, 0.000000000000000000 ) ) ;
#52643=ADVANCED_FACE ( 'NONE', ( #17396 ), #56640, .F. ) ;
#52644=CARTESIAN_POINT ( 'NONE',  ( 2.499999999999998668, -50.20833333060213732, -4.330127018922193649 ) ) ;
#52645=CARTESIAN_POINT ( 'NONE',  ( 6.123233995736766282E-16, -120.0000000000000000, -5.000000000000000000 ) ) ;
#52647=CARTESIAN_POINT ( 'NONE',  ( 2.229367062500001939, -14.97916666530107399, 3.861377020970579999 ) ) ;
#52648=CARTESIAN_POINT ( 'NONE',  ( -2.229367062500000163, 13.27083333469892779, -3.861377020970580443 ) ) ;
#52649=CARTESIAN_POINT ( 'NONE',  ( -2.229367062499996610, -54.39583333196773651, 3.861377020970582219 ) ) ;
#52653=FACE_OUTER_BOUND ( 'NONE', #6199, .T. ) ;
#52657=CARTESIAN_POINT ( 'NONE',  ( -5.926426369611017623E-15, 26.37500000273118417, 5.000000000000000000 ) ) ;
#52658=EDGE_CURVE ( 'NONE', #11867, #49354, #49839, .T. ) ;
#52659=DIRECTION ( 'NONE',  ( -0.000000000000000000, 1.000000000000000000, -0.000000000000000000 ) ) ;
#52660=CARTESIAN_POINT ( 'NONE',  ( -3.152548672688508926E-16, -86.56249999863440792, -5.148502694627439702 ) ) ;
#52661=CARTESIAN_POINT ( 'NONE',  ( -4.458734124999999437, 25.35416666803225993, -2.574251347313719407 ) ) ;
#52667=CARTESIAN_POINT ( 'NONE',  ( -2.499999999999996447, -68.83333333333332860, 4.330127018922195425 ) ) ;
#52671=CARTESIAN_POINT ( 'NONE',  ( 2.493747252781420335E-13, -90.25000000000000000, -5.000000000000000000 ) ) ;
#52672=( BOUNDED_CURVE ( )  B_SPLINE_CURVE ( 2, ( #10229, #11180, #34671, #30803, #5406, #59768, #30476, #16009, #40446 ),
 .UNSPECIFIED., .F., .F. ) 
 B_SPLINE_CURVE_WITH_KNOTS ( ( 3, 2, 2, 2, 3 ),
 ( 0.4303571428571428825, 0.4309523809523809756, 0.4321428571428571619, 0.4333333333333333481, 0.4339285714285714413 ),
 .UNSPECIFIED. ) 
 CURVE ( )  GEOMETRIC_REPRESENTATION_ITEM ( )  RATIONAL_B_SPLINE_CURVE ( ( 0.9330127018922194093, 0.9330127018922194093, 1.000000000000000000, 0.8660254037844387076, 1.000000000000000000, 0.8660254037844387076, 1.000000000000000000, 0.9330127018922194093, 0.9330127018922194093 ) ) 
 REPRESENTATION_ITEM ( '' )  );
#52673=CARTESIAN_POINT ( 'NONE',  ( -1.339745962155610925, -71.79465819873850307, 5.000000000000000000 ) ) ;
#52682=ORIENTED_EDGE ( 'NONE', *, *, #2082, .T. ) ;
#52685=CARTESIAN_POINT ( 'NONE',  ( -2.229367062500000163, -49.72916666530107221, -3.861377020970580443 ) ) ;
#52687=EDGE_LOOP ( 'NONE', ( #1141, #33610, #23791, #43539 ) ) ;
#52694=CARTESIAN_POINT ( 'NONE',  ( 4.458734124999999437, -102.0624999986344079, -5.460374474430324690E-16 ) ) ;
#52695=CARTESIAN_POINT ( 'NONE',  ( -2.499999999999996447, -26.70833333060214798, 4.330127018922195425 ) ) ;
#52700=CARTESIAN_POINT ( 'NONE',  ( 1.975475456537005874E-15, 1.375000002731185500, 5.000000000000000000 ) ) ;
#52701=CARTESIAN_POINT ( 'NONE',  ( -3.152548672688508926E-16, -9.562499998634406140, -5.148502694627439702 ) ) ;
#52702=CARTESIAN_POINT ( 'NONE',  ( 9.457646018065525792E-16, -99.31249999863439371, 5.148502694627439702 ) ) ;
#52705=CARTESIAN_POINT ( 'NONE',  ( -4.458734124999999437, -26.56249999863440792, 0.000000000000000000 ) ) ;
#52706=CARTESIAN_POINT ( 'NONE',  ( -1.339745962155610925, 12.20534180126148094, 5.000000000000000000 ) ) ;
#52709=LINE ( 'NONE', #43051, #42520 ) ;
#52710=CARTESIAN_POINT ( 'NONE',  ( 5.000000000000000888, -88.45833333060214443, 2.886751345948126879 ) ) ;
#52712=CARTESIAN_POINT ( 'NONE',  ( 2.229367062500001939, 7.770833334698926009, 3.861377020970579999 ) ) ;
#52713=ORIENTED_EDGE ( 'NONE', *, *, #2516, .F. ) ;
#52715=CARTESIAN_POINT ( 'NONE',  ( 2.499999999999998668, 2.666666666666667851, -4.330127018922193649 ) ) ;
#52716=CARTESIAN_POINT ( 'NONE',  ( 5.000000000000000888, -91.58333333333332860, 2.886751345948126879 ) ) ;
#52717=CARTESIAN_POINT ( 'NONE',  ( -3.152548672688508926E-16, -26.56249999863440792, -5.148502694627439702 ) ) ;
#52719=CARTESIAN_POINT ( 'NONE',  ( 4.458734124999999437, -75.06249999863440792, -5.460374474430324690E-16 ) ) ;
#52724=ADVANCED_FACE ( 'NONE', ( #28914 ), #38267, .T. ) ;
#52725=CARTESIAN_POINT ( 'NONE',  ( -4.458734124999999437, 5.604166668032261711, -2.574251347313719407 ) ) ;
#52726=CARTESIAN_POINT ( 'NONE',  ( -2.229367062499996610, 26.60416666803225993, 3.861377020970582219 ) ) ;
#52727=CARTESIAN_POINT ( 'NONE',  ( -2.229367062500000163, -39.72916666530107221, -3.861377020970580443 ) ) ;
#52728=CYLINDRICAL_SURFACE ( 'NONE', #26412, 5.000000000000000000 ) ;
#52731=CARTESIAN_POINT ( 'NONE',  ( 4.458734124999999437, -72.81249999863439371, -5.460374474430324690E-16 ) ) ;
#52733=CARTESIAN_POINT ( 'NONE',  ( -5.000000000000000000, -6.083333333333336590, -2.886751345948128211 ) ) ;
#52736=CARTESIAN_POINT ( 'NONE',  ( 2.229367062500001939, -65.97916666530106511, 3.861377020970579999 ) ) ;
#52737=CARTESIAN_POINT ( 'NONE',  ( 1.060575238724906964E-15, -100.6249999972688158, 5.773502691896257311 ) ) ;
#52743=CARTESIAN_POINT ( 'NONE',  ( 2.229367062499998831, -105.8958333319677365, -3.861377020970580887 ) ) ;
#52745=CARTESIAN_POINT ( 'NONE',  ( 5.000000000000000888, -56.58333333333332860, 2.886751345948126879 ) ) ;
#52749=DIRECTION ( 'NONE',  ( -0.000000000000000000, 1.000000000000000000, -0.000000000000000000 ) ) ;
#52752=ADVANCED_FACE ( 'NONE', ( #34256 ), #63550, .T. ) ;
#52759=CARTESIAN_POINT ( 'NONE',  ( 5.000000000000000000, -100.3749999972688158, -6.123233995736766282E-16 ) ) ;
#52765=CARTESIAN_POINT ( 'NONE',  ( -3.152548672688508926E-16, -33.81249999863440792, -5.148502694627439702 ) ) ;
#52773=CARTESIAN_POINT ( 'NONE',  ( 5.000000000000000888, -83.45833333060213022, 2.886751345948126879 ) ) ;
#52775=CARTESIAN_POINT ( 'NONE',  ( 9.457646018065525792E-16, -81.31249999863440792, 5.148502694627439702 ) ) ;
#52777=ORIENTED_EDGE ( 'NONE', *, *, #62138, .T. ) ;
#52779=CARTESIAN_POINT ( 'NONE',  ( -1.339745962155610925, -104.7946581987385315, 5.000000000000000000 ) ) ;
#52783=CYLINDRICAL_SURFACE ( 'NONE', #23664, 5.000000000000000000 ) ;
#52784=CARTESIAN_POINT ( 'NONE',  ( -4.458734124999998549, -12.47916666530107221, 2.574251347313722516 ) ) ;
#52785=CARTESIAN_POINT ( 'NONE',  ( -2.500000000000000444, -35.16666666666666430, -4.330127018922193649 ) ) ;
#52787=CARTESIAN_POINT ( 'NONE',  ( -2.500000000000000444, -96.04166666393548724, -4.330127018922193649 ) ) ;
#52789=CARTESIAN_POINT ( 'NONE',  ( 9.457646018065525792E-16, 28.68750000136559208, 5.148502694627439702 ) ) ;
#52791=CARTESIAN_POINT ( 'NONE',  ( -4.458734124999999437, -90.31249999863440792, 0.000000000000000000 ) ) ;
#52792=CARTESIAN_POINT ( 'NONE',  ( -1.339745962155613812, -97.20534180126145429, -5.000000000000000000 ) ) ;
#52793=CARTESIAN_POINT ( 'NONE',  ( 1.339745962155499015, -60.58034179853027723, 5.000000000000065725 ) ) ;
#52794=CARTESIAN_POINT ( 'NONE',  ( 2.229367062500001939, -9.979166665301068662, 3.861377020970579999 ) ) ;
#52798=EDGE_CURVE ( 'NONE', #27444, #58830, #60570, .T. ) ;
#52799=CARTESIAN_POINT ( 'NONE',  ( 5.000000000000000000, -36.29166666393547303, -2.886751345948129988 ) ) ;
#52801=CARTESIAN_POINT ( 'NONE',  ( -2.229367062500000163, 20.52083333469892779, -3.861377020970580443 ) ) ;
#52803=CARTESIAN_POINT ( 'NONE',  ( -2.229367062499996610, -55.14583333196773651, 3.861377020970582219 ) ) ;
#52806=CARTESIAN_POINT ( 'NONE',  ( 2.500000000000002220, 10.33333333333333393, 4.330127018922192761 ) ) ;
#52808=CARTESIAN_POINT ( 'NONE',  ( 1.339745962155615144, -69.70534180126148271, 4.999999999999999112 ) ) ;
#52809=CARTESIAN_POINT ( 'NONE',  ( -3.152548672688508926E-16, -50.56249999863440792, -5.148502694627439702 ) ) ;
#52810=CARTESIAN_POINT ( 'NONE',  ( 2.500000000000002220, -81.54166666393547303, 4.330127018922192761 ) ) ;
#52814=CARTESIAN_POINT ( 'NONE',  ( -2.229367062499996610, -88.39583333196773651, 3.861377020970582219 ) ) ;
#52816=CARTESIAN_POINT ( 'NONE',  ( -5.000000000000000000, -38.08333333333333570, -2.886751345948128211 ) ) ;
#52817=ORIENTED_EDGE ( 'NONE', *, *, #38485, .T. ) ;
#52818=ADVANCED_FACE ( 'NONE', ( #39397 ), #59031, .T. ) ;
#52821=CARTESIAN_POINT ( 'NONE',  ( -4.458734124999998549, -96.22916666530106511, 2.574251347313722516 ) ) ;
#52822=CARTESIAN_POINT ( 'NONE',  ( 4.458734124999998549, 6.020833334698928674, -2.574251347313721627 ) ) ;
#52823=CARTESIAN_POINT ( 'NONE',  ( 1.060575238724906964E-15, 13.37500000273118594, 5.773502691896257311 ) ) ;
#52826=EDGE_CURVE ( 'NONE', #19379, #46887, #10012, .T. ) ;
#52838=CARTESIAN_POINT ( 'NONE',  ( 2.229367062499998831, -19.89583333196774007, -3.861377020970580887 ) ) ;
#52846=VERTEX_POINT ( 'NONE', #12919 ) ;
#52849=CARTESIAN_POINT ( 'NONE',  ( 2.229367062499998831, -68.89583333196773651, -3.861377020970580887 ) ) ;
#52850=CARTESIAN_POINT ( 'NONE',  ( 1.975475456537005874E-15, -9.624999997268814056, 5.000000000000000000 ) ) ;
#52851=CARTESIAN_POINT ( 'NONE',  ( 1.975475456537005874E-15, -5.624999997268812280, 5.000000000000000000 ) ) ;
#52852=ORIENTED_EDGE ( 'NONE', *, *, #21385, .T. ) ;
#52854=DIRECTION ( 'NONE',  ( -0.000000000000000000, 1.000000000000000000, -0.000000000000000000 ) ) ;
#52856=CARTESIAN_POINT ( 'NONE',  ( 2.229367062500001939, 2.770833334698928674, 3.861377020970579999 ) ) ;
#52859=CARTESIAN_POINT ( 'NONE',  ( -6.972266317189433020E-16, 1.875000002731185722, -5.000000000000000000 ) ) ;
#52860=CARTESIAN_POINT ( 'NONE',  ( 2.229367062499998831, 1.354166668032261933, -3.861377020970580887 ) ) ;
#52863=CARTESIAN_POINT ( 'NONE',  ( 1.975475456537005874E-15, -92.62499999726881583, 5.000000000000000000 ) ) ;
#52866=CARTESIAN_POINT ( 'NONE',  ( 9.457646018065525792E-16, -78.06249999863440792, 5.148502694627439702 ) ) ;
#52868=CARTESIAN_POINT ( 'NONE',  ( 4.458734124999999437, 8.187500001365595637, -5.460374474430324690E-16 ) ) ;
#52871=CARTESIAN_POINT ( 'NONE',  ( 2.229367062500001939, -58.22916666530107932, 3.861377020970579999 ) ) ;
#52872=CARTESIAN_POINT ( 'NONE',  ( -2.500000000000000444, -20.04166666393548013, -4.330127018922193649 ) ) ;
#52874=CARTESIAN_POINT ( 'NONE',  ( 1.975475456537005874E-15, -42.62499999726880873, 5.000000000000000000 ) ) ;
#52877=CARTESIAN_POINT ( 'NONE',  ( -2.229367062500000163, -39.47916666530107221, -3.861377020970580443 ) ) ;
#52878=CARTESIAN_POINT ( 'NONE',  ( 2.229367062500001939, -26.22916666530106866, 3.861377020970579999 ) ) ;
#52879=DIRECTION ( 'NONE',  ( -0.000000000000000000, 1.000000000000000000, -0.000000000000000000 ) ) ;
#52880=CARTESIAN_POINT ( 'NONE',  ( -3.535250795749689387E-16, 24.75000000000000355, -5.773502691896257311 ) ) ;
#52882=ORIENTED_EDGE ( 'NONE', *, *, #7242, .T. ) ;
#52883=CARTESIAN_POINT ( 'NONE',  ( 9.457646018065525792E-16, -109.3124999986343937, 5.148502694627439702 ) ) ;
#52884=AXIS2_PLACEMENT_3D ( 'NONE', #19845, #20812, #59739 ) ;
#52885=CARTESIAN_POINT ( 'NONE',  ( -2.229367062500000163, -30.47916666530107221, -3.861377020970580443 ) ) ;
#52886=CARTESIAN_POINT ( 'NONE',  ( 5.000000000000000888, -69.45833333060214443, 2.886751345948126879 ) ) ;
#52889=CARTESIAN_POINT ( 'NONE',  ( 4.458734124999999437, -28.81249999863440436, -5.460374474430324690E-16 ) ) ;
#52890=CARTESIAN_POINT ( 'NONE',  ( 4.458734125000000326, -76.14583333196773651, 2.574251347313718519 ) ) ;
#52893=CARTESIAN_POINT ( 'NONE',  ( -6.972266317189433020E-16, 5.749999999999999112, -5.000000000000000000 ) ) ;
#52895=CARTESIAN_POINT ( 'NONE',  ( 2.500000000000002220, -24.66666666666666430, 4.330127018922192761 ) ) ;
#52898=CARTESIAN_POINT ( 'NONE',  ( 5.000000000000000888, -16.45833333060214443, 2.886751345948126879 ) ) ;
#52900=CARTESIAN_POINT ( 'NONE',  ( -5.000000000000000000, 29.12500000273118417, 0.000000000000000000 ) ) ;
#52906=CARTESIAN_POINT ( 'NONE',  ( 1.975475456537005874E-15, -15.75000000000000000, 5.000000000000000000 ) ) ;
#52908=CARTESIAN_POINT ( 'NONE',  ( -5.000000000000000000, -87.95833333060213022, -2.886751345948128211 ) ) ;
#52916=CARTESIAN_POINT ( 'NONE',  ( -1.339745962155610925, 0.3303418039926660499, 5.000000000000000000 ) ) ;
#52917=DIRECTION ( 'NONE',  ( 0.000000000000000000, 0.000000000000000000, 1.000000000000000000 ) ) ;
#52919=EDGE_LOOP ( 'NONE', ( #38808, #45237, #55327, #6894 ) ) ;
#52922=EDGE_CURVE ( 'NONE', #19776, #19094, #57325, .T. ) ;
#52925=( BOUNDED_CURVE ( )  B_SPLINE_CURVE ( 2, ( #15702, #55269, #49787, #1561, #60094, #25987, #41085, #10547, #39811 ),
 .UNSPECIFIED., .F., .F. ) 
 B_SPLINE_CURVE_WITH_KNOTS ( ( 3, 2, 2, 2, 3 ),
 ( 0.5910714285714285809, 0.5916666666666666741, 0.5928571428571428603, 0.5940476190476190466, 0.5946428571428571397 ),
 .UNSPECIFIED. ) 
 CURVE ( )  GEOMETRIC_REPRESENTATION_ITEM ( )  RATIONAL_B_SPLINE_CURVE ( ( 0.9330127018922194093, 0.9330127018922194093, 1.000000000000000000, 0.8660254037844387076, 1.000000000000000000, 0.8660254037844387076, 1.000000000000000000, 0.9330127018922194093, 0.9330127018922194093 ) ) 
 REPRESENTATION_ITEM ( '' )  );
#52926=CARTESIAN_POINT ( 'NONE',  ( -3.152548672688508926E-16, -82.56249999863442213, -5.148502694627439702 ) ) ;
#52927=CARTESIAN_POINT ( 'NONE',  ( 4.458734124999998549, 17.27083333469892779, -2.574251347313721627 ) ) ;
#52928=CARTESIAN_POINT ( 'NONE',  ( 5.000000000000000888, -12.45833333060214976, 2.886751345948126879 ) ) ;
#52935=CARTESIAN_POINT ( 'NONE',  ( 1.339745962155612702, -13.16965819600733489, -5.000000000000000000 ) ) ;
#52936=CARTESIAN_POINT ( 'NONE',  ( 4.458734124999998549, -61.72916666530106511, -2.574251347313721627 ) ) ;
#52937=CARTESIAN_POINT ( 'NONE',  ( 5.000000000000000888, 10.41666666666666785, 2.886751345948126879 ) ) ;
#52938=CARTESIAN_POINT ( 'NONE',  ( -2.229367062499996610, 24.85416666803225993, 3.861377020970582219 ) ) ;
#52939=CARTESIAN_POINT ( 'NONE',  ( 2.500000000000002220, -109.6666666666666572, 4.330127018922192761 ) ) ;
#52941=( BOUNDED_CURVE ( )  B_SPLINE_CURVE ( 2, ( #12048, #22669, #42268, #62221, #32620, #31988, #27168, #57082, #61908 ),
 .UNSPECIFIED., .F., .F. ) 
 B_SPLINE_CURVE_WITH_KNOTS ( ( 3, 2, 2, 2, 3 ),
 ( 0.3482142857142856984, 0.3488095238095237915, 0.3499999999999999778, 0.3511904761904761640, 0.3517857142857143127 ),
 .UNSPECIFIED. ) 
 CURVE ( )  GEOMETRIC_REPRESENTATION_ITEM ( )  RATIONAL_B_SPLINE_CURVE ( ( 0.9330127018922194093, 0.9330127018922194093, 1.000000000000000000, 0.8660254037844387076, 1.000000000000000000, 0.8660254037844387076, 1.000000000000000000, 0.9330127018922163007, 0.9330127018922194093 ) ) 
 REPRESENTATION_ITEM ( '' )  );
#52943=CARTESIAN_POINT ( 'NONE',  ( -4.458734124999999437, -43.56249999863440081, 0.000000000000000000 ) ) ;
#52944=CARTESIAN_POINT ( 'NONE',  ( -5.000000000000000000, -4.958333330602147981, -2.886751345948128211 ) ) ;
#52947=CARTESIAN_POINT ( 'NONE',  ( -4.458734124999999437, -109.3124999986343937, 0.000000000000000000 ) ) ;
#52948=CARTESIAN_POINT ( 'NONE',  ( 4.458734125000000326, -11.14583333196773829, 2.574251347313718519 ) ) ;
#52950=CARTESIAN_POINT ( 'NONE',  ( 5.000000000000000000, -52.41666666666666430, -2.886751345948130876 ) ) ;
#52951=CARTESIAN_POINT ( 'NONE',  ( 4.458734124999998549, -99.72916666530105090, -2.574251347313721627 ) ) ;
#52953=CARTESIAN_POINT ( 'NONE',  ( -4.458734124999998549, -91.47916666530106511, 2.574251347313722516 ) ) ;
#52954=CARTESIAN_POINT ( 'NONE',  ( 2.500000000000002220, -50.54166666393547303, 4.330127018922192761 ) ) ;
#52957=CARTESIAN_POINT ( 'NONE',  ( -4.458734124999999437, -10.31249999863440792, 0.000000000000000000 ) ) ;
#52958=CARTESIAN_POINT ( 'NONE',  ( -4.458734124999999437, 11.35416666803225993, -2.574251347313719407 ) ) ;
#52959=CARTESIAN_POINT ( 'NONE',  ( 2.229367062500001939, -57.22916666530107932, 3.861377020970579999 ) ) ;
#52960=DIRECTION ( 'NONE',  ( -0.000000000000000000, 1.000000000000000000, -0.000000000000000000 ) ) ;
#52967=CYLINDRICAL_SURFACE ( 'NONE', #24689, 5.000000000000000000 ) ;
#52969=CARTESIAN_POINT ( 'NONE',  ( -4.458734124999999437, -84.31249999863439371, 0.000000000000000000 ) ) ;
#52970=CARTESIAN_POINT ( 'NONE',  ( 4.458734124999999437, 20.93750000136559208, -5.460374474430324690E-16 ) ) ;
#52975=CARTESIAN_POINT ( 'NONE',  ( -3.535250795749689387E-16, -72.24999999999998579, -5.773502691896257311 ) ) ;
#52980=CARTESIAN_POINT ( 'NONE',  ( -6.972266317189433020E-16, -72.25000000000000000, -5.000000000000000000 ) ) ;
#52985=ORIENTED_EDGE ( 'NONE', *, *, #46347, .F. ) ;
#52988=EDGE_LOOP ( 'NONE', ( #9868, #61918, #55685, #52777 ) ) ;
#52991=CARTESIAN_POINT ( 'NONE',  ( 2.229367062499998831, -54.89583333196773651, -3.861377020970580887 ) ) ;
#52992=( BOUNDED_CURVE ( )  B_SPLINE_CURVE ( 2, ( #15720, #6401, #35339, #54958, #26010, #1902, #45627, #10888, #59471 ),
 .UNSPECIFIED., .F., .F. ) 
 B_SPLINE_CURVE_WITH_KNOTS ( ( 3, 2, 2, 2, 3 ),
 ( 0.8517857142857142572, 0.8523809523809523503, 0.8535714285714285365, 0.8547619047619047228, 0.8553571428571428159 ),
 .UNSPECIFIED. ) 
 CURVE ( )  GEOMETRIC_REPRESENTATION_ITEM ( )  RATIONAL_B_SPLINE_CURVE ( ( 0.9330127018922194093, 0.9330127018922194093, 1.000000000000000000, 0.8660254037844387076, 1.000000000000000000, 0.8660254037844387076, 1.000000000000000000, 0.9330127018922194093, 0.9330127018922194093 ) ) 
 REPRESENTATION_ITEM ( '' )  );
#53002=CARTESIAN_POINT ( 'NONE',  ( -4.458734124999999437, -104.5624999986344079, 0.000000000000000000 ) ) ;
#53007=CARTESIAN_POINT ( 'NONE',  ( 4.458734125000000326, -36.89583333196773651, 2.574251347313718519 ) ) ;
#53009=CARTESIAN_POINT ( 'NONE',  ( -4.458734124999999437, -8.395833331967736513, -2.574251347313719407 ) ) ;
#53010=CARTESIAN_POINT ( 'NONE',  ( -4.458734124999999437, -99.56249999863440792, 0.000000000000000000 ) ) ;
#53011=EDGE_CURVE ( 'NONE', #60996, #15028, #28028, .T. ) ;
#53013=CARTESIAN_POINT ( 'NONE',  ( 4.458734124999999437, -30.06249999863440436, -5.460374474430324690E-16 ) ) ;
#53018=CARTESIAN_POINT ( 'NONE',  ( -5.000000000000000000, -16.00000000000000000, 0.000000000000000000 ) ) ;
#53019=CARTESIAN_POINT ( 'NONE',  ( -6.972266317189433020E-16, -34.25000000000000000, -5.000000000000000000 ) ) ;
#53021=CARTESIAN_POINT ( 'NONE',  ( 4.458734125000000326, 3.854166668032260823, 2.574251347313718519 ) ) ;
#53022=VERTEX_POINT ( 'NONE', #21075 ) ;
#53023=( GEOMETRIC_REPRESENTATION_CONTEXT ( 3 ) GLOBAL_UNCERTAINTY_ASSIGNED_CONTEXT ( ( #18243 ) ) GLOBAL_UNIT_ASSIGNED_CONTEXT ( ( #54126, #14257, #431 ) ) REPRESENTATION_CONTEXT ( 'NONE', 'WORKASPACE' ) );
#53025=CARTESIAN_POINT ( 'NONE',  ( -1.339745962155613812, 15.91965820146970501, -5.000000000000000000 ) ) ;
#53026=CARTESIAN_POINT ( 'NONE',  ( -4.999999999999999112, -96.91666666666665719, 2.886751345948131764 ) ) ;
#53027=CARTESIAN_POINT ( 'NONE',  ( 2.229367062500001939, -27.97916666530107221, 3.861377020970579999 ) ) ;
#53028=CARTESIAN_POINT ( 'NONE',  ( -2.499999999999996447, -76.70833333060214443, 4.330127018922195425 ) ) ;
#53029=CARTESIAN_POINT ( 'NONE',  ( 2.229367062499998831, -74.89583333196773651, -3.861377020970580887 ) ) ;
#53032=CARTESIAN_POINT ( 'NONE',  ( -2.499999999999996447, -101.7083333306021444, 4.330127018922195425 ) ) ;
#53033=EDGE_CURVE ( 'NONE', #51665, #25684, #55499, .T. ) ;
#53036=CARTESIAN_POINT ( 'NONE',  ( 4.458734124999999437, 5.187500001365596525, -5.460374474430324690E-16 ) ) ;
#53037=CARTESIAN_POINT ( 'NONE',  ( -4.458734124999999437, 25.43750000136559208, 0.000000000000000000 ) ) ;
#53038=CARTESIAN_POINT ( 'NONE',  ( 4.458734125000000326, -42.14583333196773651, 2.574251347313718519 ) ) ;
#53039=CARTESIAN_POINT ( 'NONE',  ( -1.339745962155613812, -4.080341798530293218, -5.000000000000000000 ) ) ;
#53042=( BOUNDED_CURVE ( )  B_SPLINE_CURVE ( 2, ( #33823, #53442, #9685, #43154, #24173, #38636, #3937, #48609, #58897 ),
 .UNSPECIFIED., .F., .F. ) 
 B_SPLINE_CURVE_WITH_KNOTS ( ( 3, 2, 2, 2, 3 ),
 ( 0.3732142857142857206, 0.3738095238095238138, 0.3750000000000000000, 0.3761904761904761862, 0.3767857142857142794 ),
 .UNSPECIFIED. ) 
 CURVE ( )  GEOMETRIC_REPRESENTATION_ITEM ( )  RATIONAL_B_SPLINE_CURVE ( ( 0.9330127018922194093, 0.9330127018922194093, 1.000000000000000000, 0.8660254037844387076, 1.000000000000000000, 0.8660254037844387076, 1.000000000000000000, 0.9330127018922194093, 0.9330127018922194093 ) ) 
 REPRESENTATION_ITEM ( '' )  );
#53044=CARTESIAN_POINT ( 'NONE',  ( -2.229367062500000163, -70.47916666530107932, -3.861377020970580443 ) ) ;
#53045=CARTESIAN_POINT ( 'NONE',  ( -3.535250795749689387E-16, -99.12499999726881583, -5.773502691896257311 ) ) ;
#53047=FACE_OUTER_BOUND ( 'NONE', #59735, .T. ) ;
#53048=ADVANCED_FACE ( 'NONE', ( #2650 ), #22269, .T. ) ;
#53049=CARTESIAN_POINT ( 'NONE',  ( 9.457646018065525792E-16, -105.3124999986344221, 5.148502694627439702 ) ) ;
#53051=CARTESIAN_POINT ( 'NONE',  ( 5.000000000000000000, -56.41666666666666430, -2.886751345948129988 ) ) ;
#53053=ORIENTED_EDGE ( 'NONE', *, *, #37048, .F. ) ;
#53054=LINE ( 'NONE', #14752, #59185 ) ;
#53055=CARTESIAN_POINT ( 'NONE',  ( -2.500000000000000444, 12.83333333333333215, -4.330127018922193649 ) ) ;
#53062=VERTEX_POINT ( 'NONE', #9663 ) ;
#53063=CARTESIAN_POINT ( 'NONE',  ( 5.000000000000000000, -45.29166666393547303, -2.886751345948130876 ) ) ;
#53065=VERTEX_POINT ( 'NONE', #44390 ) ;
#53069=CARTESIAN_POINT ( 'NONE',  ( 4.458734124999998549, -40.97916666530107932, -2.574251347313721627 ) ) ;
#53074=EDGE_CURVE ( 'NONE', #42260, #54554, #53108, .T. ) ;
#53077=AXIS2_PLACEMENT_3D ( 'NONE', #54623, #11508, #35963 ) ;
#53079=EDGE_CURVE ( 'NONE', #100, #56685, #32572, .T. ) ;
#53081=CARTESIAN_POINT ( 'NONE',  ( 5.000000000000000000, -26.49999999999999645, -6.123233995736766282E-16 ) ) ;
#53083=AXIS2_PLACEMENT_3D ( 'NONE', #42119, #17689, #55983 ) ;
#53084=CARTESIAN_POINT ( 'NONE',  ( 4.458734124999999437, -86.06249999863439371, -5.460374474430324690E-16 ) ) ;
#53086=ORIENTED_EDGE ( 'NONE', *, *, #53178, .F. ) ;
#53087=CARTESIAN_POINT ( 'NONE',  ( 1.339745962155615144, -99.70534180126146850, 4.999999999999999112 ) ) ;
#53091=EDGE_LOOP ( 'NONE', ( #4644, #23158, #11451, #41223 ) ) ;
#53093=CARTESIAN_POINT ( 'NONE',  ( -5.000000000000000000, -70.87499999726880162, 0.000000000000000000 ) ) ;
#53094=CARTESIAN_POINT ( 'NONE',  ( -4.458734124999999437, -12.64583333196774007, -2.574251347313719407 ) ) ;
#53096=FACE_OUTER_BOUND ( 'NONE', #55479, .T. ) ;
#53100=CARTESIAN_POINT ( 'NONE',  ( 2.229367062499998831, 19.10416666803225993, -3.861377020970580887 ) ) ;
#53102=CARTESIAN_POINT ( 'NONE',  ( 2.229367062499998831, -89.64583333196773651, -3.861377020970580887 ) ) ;
#53103=CARTESIAN_POINT ( 'NONE',  ( 1.339745962155615144, -47.70534180126147561, 4.999999999999999112 ) ) ;
#53104=DIRECTION ( 'NONE',  ( -0.000000000000000000, 1.000000000000000000, -0.000000000000000000 ) ) ;
#53105=CARTESIAN_POINT ( 'NONE',  ( 9.457646018065525792E-16, -12.06249999863440081, 5.148502694627439702 ) ) ;
#53108=LINE ( 'NONE', #63089, #2769 ) ;
#53109=CARTESIAN_POINT ( 'NONE',  ( -5.000000000000000000, -34.87499999726881583, 0.000000000000000000 ) ) ;
#53110=CARTESIAN_POINT ( 'NONE',  ( 1.975475456537005874E-15, -49.62499999726880873, 5.000000000000000000 ) ) ;
#53111=CARTESIAN_POINT ( 'NONE',  ( 4.458734124999999437, 19.18750000136559564, -5.460374474430324690E-16 ) ) ;
#53114=CARTESIAN_POINT ( 'NONE',  ( -2.229367062500000163, -57.47916666530107932, -3.861377020970580443 ) ) ;
#53118=CARTESIAN_POINT ( 'NONE',  ( -5.000000000000000000, 11.91666666666666607, -2.886751345948128211 ) ) ;
#53121=CARTESIAN_POINT ( 'NONE',  ( 2.229367062500001939, -51.97916666530107221, 3.861377020970579999 ) ) ;
#53122=CARTESIAN_POINT ( 'NONE',  ( 5.000000000000000888, -81.45833333060213022, 2.886751345948126879 ) ) ;
#53123=AXIS2_PLACEMENT_3D ( 'NONE', #39491, #10864, #59127 ) ;
#53125=( BOUNDED_CURVE ( )  B_SPLINE_CURVE ( 2, ( #37595, #33094, #18614, #57860, #63007, #52410, #13155, #4143, #8341 ),
 .UNSPECIFIED., .F., .F. ) 
 B_SPLINE_CURVE_WITH_KNOTS ( ( 3, 2, 2, 2, 3 ),
 ( 0.3589285714285714302, 0.3595238095238095233, 0.3607142857142857095, 0.3619047619047618958, 0.3624999999999999889 ),
 .UNSPECIFIED. ) 
 CURVE ( )  GEOMETRIC_REPRESENTATION_ITEM ( )  RATIONAL_B_SPLINE_CURVE ( ( 0.9330127018922194093, 0.9330127018922194093, 1.000000000000000000, 0.8660254037844387076, 1.000000000000000000, 0.8660254037844387076, 1.000000000000000000, 0.9330127018922194093, 0.9330127018922194093 ) ) 
 REPRESENTATION_ITEM ( '' )  );
#53127=CARTESIAN_POINT ( 'NONE',  ( -1.339745962155613812, -92.20534180126149693, -5.000000000000000000 ) ) ;
#53128=AXIS2_PLACEMENT_3D ( 'NONE', #30736, #41330, #17212 ) ;
#53129=CARTESIAN_POINT ( 'NONE',  ( -2.229367062499996610, -91.39583333196773651, 3.861377020970582219 ) ) ;
#53131=CARTESIAN_POINT ( 'NONE',  ( -3.535250795749689387E-16, -38.24999999999999289, -5.773502691896257311 ) ) ;
#53132=CARTESIAN_POINT ( 'NONE',  ( 1.975475456537005874E-15, -19.62499999726881228, 5.000000000000000000 ) ) ;
#53134=ORIENTED_EDGE ( 'NONE', *, *, #21746, .F. ) ;
#53135=CARTESIAN_POINT ( 'NONE',  ( 4.458734124999999437, -93.81249999863440792, -5.460374474430324690E-16 ) ) ;
#53136=CARTESIAN_POINT ( 'NONE',  ( -4.458734124999999437, 7.354166668032259935, -2.574251347313719407 ) ) ;
#53137=CARTESIAN_POINT ( 'NONE',  ( 1.060575238724906964E-15, 10.37500000273118594, 5.773502691896257311 ) ) ;
#53143=CARTESIAN_POINT ( 'NONE',  ( -5.000000000000000000, -11.08333333333333393, -2.886751345948128211 ) ) ;
#53144=CYLINDRICAL_SURFACE ( 'NONE', #17913, 5.000000000000000000 ) ;
#53145=CARTESIAN_POINT ( 'NONE',  ( 2.500000000000002220, -20.66666666666666785, 4.330127018922192761 ) ) ;
#53148=CARTESIAN_POINT ( 'NONE',  ( 9.457646018065525792E-16, -25.31249999863440792, 5.148502694627439702 ) ) ;
#53157=ORIENTED_EDGE ( 'NONE', *, *, #30714, .T. ) ;
#53158=CARTESIAN_POINT ( 'NONE',  ( 1.339745962155612702, -93.16965819600733312, -5.000000000000000000 ) ) ;
#53159=VERTEX_POINT ( 'NONE', #9528 ) ;
#53160=CARTESIAN_POINT ( 'NONE',  ( -4.458734124999999437, -66.56249999863440792, 0.000000000000000000 ) ) ;
#53167=EDGE_CURVE ( 'NONE', #43365, #37277, #13727, .T. ) ;
#53168=CARTESIAN_POINT ( 'NONE',  ( -4.458734124999998549, -0.4791666653010707710, 2.574251347313722516 ) ) ;
#53170=ADVANCED_FACE ( 'NONE', ( #29134 ), #28202, .T. ) ;
#53171=CARTESIAN_POINT ( 'NONE',  ( 0.000000000000000000, -120.0000000000000000, 0.000000000000000000 ) ) ;
#53178=EDGE_CURVE ( 'NONE', #10376, #17008, #36712, .T. ) ;
#53179=CARTESIAN_POINT ( 'NONE',  ( -3.152548672688508926E-16, -76.56249999863440792, -5.148502694627439702 ) ) ;
#53181=CARTESIAN_POINT ( 'NONE',  ( 4.458734125000001214, 7.104166668032259047, 2.574251347313718519 ) ) ;
#53184=CARTESIAN_POINT ( 'NONE',  ( -2.229367062499996610, -59.39583333196773651, 3.861377020970582219 ) ) ;
#53185=CARTESIAN_POINT ( 'NONE',  ( -2.499999999999996447, -19.70833333060214798, 4.330127018922195425 ) ) ;
#53186=DIRECTION ( 'NONE',  ( 0.000000000000000000, 0.000000000000000000, 1.000000000000000000 ) ) ;
#53187=CARTESIAN_POINT ( 'NONE',  ( -6.972266317189433020E-16, -65.12499999726880162, -5.000000000000000000 ) ) ;
#53189=DIRECTION ( 'NONE',  ( -0.000000000000000000, 1.000000000000000000, -0.000000000000000000 ) ) ;
#53190=CARTESIAN_POINT ( 'NONE',  ( -4.458734124999998549, -38.22916666530107932, 2.574251347313722516 ) ) ;
#53191=CARTESIAN_POINT ( 'NONE',  ( -4.458734124999997661, -29.47916666530106866, 2.574251347313722516 ) ) ;
#53194=CARTESIAN_POINT ( 'NONE',  ( -2.500000000000000444, 26.83333333333333570, -4.330127018922193649 ) ) ;
#53196=CARTESIAN_POINT ( 'NONE',  ( 9.457646018065525792E-16, -107.3124999986343937, 5.148502694627439702 ) ) ;
#53197=CARTESIAN_POINT ( 'NONE',  ( 9.457646018065525792E-16, -30.06249999863440081, 5.148502694627439702 ) ) ;
#53198=CARTESIAN_POINT ( 'NONE',  ( -5.000000000000000000, -68.87499999726880162, 0.000000000000000000 ) ) ;
#53201=CARTESIAN_POINT ( 'NONE',  ( -4.458734124999999437, -77.64583333196773651, -2.574251347313719407 ) ) ;
#53205=DIRECTION ( 'NONE',  ( -0.000000000000000000, 1.000000000000000000, -0.000000000000000000 ) ) ;
#53206=CARTESIAN_POINT ( 'NONE',  ( -5.000000000000000000, -23.08333333333332860, -2.886751345948128211 ) ) ;
#53208=ORIENTED_EDGE ( 'NONE', *, *, #8234, .F. ) ;
#53210=CARTESIAN_POINT ( 'NONE',  ( 5.000000000000000888, 1.416666666666666741, 2.886751345948126879 ) ) ;
#53212=AXIS2_PLACEMENT_3D ( 'NONE', #46784, #22670, #51930 ) ;
#53213=CARTESIAN_POINT ( 'NONE',  ( -3.535250795749689387E-16, 24.87500000273118417, -5.773502691896257311 ) ) ;
#53220=CARTESIAN_POINT ( 'NONE',  ( -5.000000000000000000, -77.08333333333334281, -2.886751345948128211 ) ) ;
#53224=( BOUNDED_CURVE ( )  B_SPLINE_CURVE ( 2, ( #43505, #32931, #18448, #28716, #63150, #63466, #19385, #19061, #52863 ),
 .UNSPECIFIED., .F., .F. ) 
 B_SPLINE_CURVE_WITH_KNOTS ( ( 3, 2, 2, 2, 3 ),
 ( 0.8660714285714286031, 0.8666666666666666963, 0.8678571428571428825, 0.8690476190476190688, 0.8696428571428571619 ),
 .UNSPECIFIED. ) 
 CURVE ( )  GEOMETRIC_REPRESENTATION_ITEM ( )  RATIONAL_B_SPLINE_CURVE ( ( 0.9330127018922194093, 0.9330127018922194093, 1.000000000000000000, 0.8660254037844387076, 1.000000000000000000, 0.8660254037844387076, 1.000000000000000000, 0.9330127018922194093, 0.9330127018922194093 ) ) 
 REPRESENTATION_ITEM ( '' )  );
#53225=CARTESIAN_POINT ( 'NONE',  ( 5.000000000000000888, 10.54166666939785202, 2.886751345948126879 ) ) ;
#53231=ORIENTED_EDGE ( 'NONE', *, *, #21624, .T. ) ;
#53232=CARTESIAN_POINT ( 'NONE',  ( 1.339745962155612702, -87.29465819873851729, -5.000000000000000000 ) ) ;
#53235=ORIENTED_EDGE ( 'NONE', *, *, #33833, .F. ) ;
#53242=CARTESIAN_POINT ( 'NONE',  ( 4.458734125000001214, -80.89583333196773651, 2.574251347313718519 ) ) ;
#53243=CARTESIAN_POINT ( 'NONE',  ( -4.458734124999999437, 16.60416666803225993, -2.574251347313719407 ) ) ;
#53245=ORIENTED_EDGE ( 'NONE', *, *, #48430, .T. ) ;
#53251=CARTESIAN_POINT ( 'NONE',  ( 2.229367062499998831, -62.64583333196774362, -3.861377020970580887 ) ) ;
#53253=CARTESIAN_POINT ( 'NONE',  ( -4.458734124999998549, 23.77083333469892423, 2.574251347313722516 ) ) ;
#53255=CARTESIAN_POINT ( 'NONE',  ( -5.000000000000000000, -109.9999999999999858, 0.000000000000000000 ) ) ;
#53257=CARTESIAN_POINT ( 'NONE',  ( 9.457646018065525792E-16, -46.31249999863440792, 5.148502694627439702 ) ) ;
#53258=CARTESIAN_POINT ( 'NONE',  ( -5.000000000000000000, -2.958333330602146649, -2.886751345948128211 ) ) ;
#53259=CARTESIAN_POINT ( 'NONE',  ( -5.926426369611017623E-15, 26.37500000273118417, 5.000000000000000000 ) ) ;
#53262=LINE ( 'NONE', #4371, #28546 ) ;
#53263=CARTESIAN_POINT ( 'NONE',  ( -2.229367062499996610, -11.39583333196773829, 3.861377020970582219 ) ) ;
#53266=CARTESIAN_POINT ( 'NONE',  ( -2.229367062499996610, -96.14583333196773651, 3.861377020970582219 ) ) ;
#53268=CARTESIAN_POINT ( 'NONE',  ( 4.458734124999998549, -92.97916666530106511, -2.574251347313721627 ) ) ;
#53269=CARTESIAN_POINT ( 'NONE',  ( -5.000000000000000000, -50.95833333060213732, -2.886751345948128211 ) ) ;
#53273=CARTESIAN_POINT ( 'NONE',  ( -2.229367062499996610, -18.14583333196773651, 3.861377020970582219 ) ) ;
#53274=CARTESIAN_POINT ( 'NONE',  ( -4.458734124999999437, 9.354166668032261711, -2.574251347313719407 ) ) ;
#53275=CARTESIAN_POINT ( 'NONE',  ( -4.458734124999999437, -60.64583333196774362, -2.574251347313719407 ) ) ;
#53276=DIRECTION ( 'NONE',  ( -0.000000000000000000, 1.000000000000000000, -0.000000000000000000 ) ) ;
#53282=CARTESIAN_POINT ( 'NONE',  ( -2.499999999999996447, -91.70833333060214443, 4.330127018922195425 ) ) ;
#53283=CARTESIAN_POINT ( 'NONE',  ( -5.000000000000000000, -25.00000000000000000, 0.000000000000000000 ) ) ;
#53284=CARTESIAN_POINT ( 'NONE',  ( 9.457646018065525792E-16, -88.06249999863439371, 5.148502694627439702 ) ) ;
#53285=CARTESIAN_POINT ( 'NONE',  ( -2.229367062500000163, 21.27083333469892779, -3.861377020970580443 ) ) ;
#53287=DIRECTION ( 'NONE',  ( -0.000000000000000000, 1.000000000000000000, -0.000000000000000000 ) ) ;
#53288=CARTESIAN_POINT ( 'NONE',  ( -2.499999999999996447, -6.833333333333330373, 4.330127018922195425 ) ) ;
#53290=CARTESIAN_POINT ( 'NONE',  ( -5.000000000000000000, -72.00000000000000000, 0.000000000000000000 ) ) ;
#53293=CYLINDRICAL_SURFACE ( 'NONE', #3778, 5.000000000000000000 ) ;
#53297=CARTESIAN_POINT ( 'NONE',  ( -4.999999999999998224, -103.9166666666666572, 2.886751345948131764 ) ) ;
#53301=( BOUNDED_CURVE ( )  B_SPLINE_CURVE ( 2, ( #9808, #13703, #28807, #33325, #58712, #53882, #28494, #48113, #23684 ),
 .UNSPECIFIED., .F., .F. ) 
 B_SPLINE_CURVE_WITH_KNOTS ( ( 3, 2, 2, 2, 3 ),
 ( 0.8767857142857142794, 0.8773809523809523725, 0.8785714285714285587, 0.8797619047619047450, 0.8803571428571428381 ),
 .UNSPECIFIED. ) 
 CURVE ( )  GEOMETRIC_REPRESENTATION_ITEM ( )  RATIONAL_B_SPLINE_CURVE ( ( 0.9330127018922194093, 0.9330127018922194093, 1.000000000000000000, 0.8660254037844387076, 1.000000000000000000, 0.8660254037844387076, 1.000000000000000000, 0.9330127018922194093, 0.9330127018922194093 ) ) 
 REPRESENTATION_ITEM ( '' )  );
#53304=ORIENTED_EDGE ( 'NONE', *, *, #60231, .T. ) ;
#53307=EDGE_LOOP ( 'NONE', ( #62259, #58053, #21133, #7994 ) ) ;
#53309=CARTESIAN_POINT ( 'NONE',  ( -6.972266317189433020E-16, 23.75000000000000000, -5.000000000000000000 ) ) ;
#53310=CARTESIAN_POINT ( 'NONE',  ( -4.458734124999999437, -54.56249999863440081, 0.000000000000000000 ) ) ;
#53317=ORIENTED_EDGE ( 'NONE', *, *, #6629, .F. ) ;
#53318=( BOUNDED_CURVE ( )  B_SPLINE_CURVE ( 2, ( #16876, #21069, #33178, #62458, #22024, #62136, #46466, #52793, #16559 ),
 .UNSPECIFIED., .F., .F. ) 
 B_SPLINE_CURVE_WITH_KNOTS ( ( 3, 2, 2, 2, 3 ),
 ( 0.6374999999999999556, 0.6380952380952380487, 0.6392857142857142350, 0.6404761904761904212, 0.6410714285714286254 ),
 .UNSPECIFIED. ) 
 CURVE ( )  GEOMETRIC_REPRESENTATION_ITEM ( )  RATIONAL_B_SPLINE_CURVE ( ( 0.9330127018922194093, 0.9330127018922194093, 1.000000000000000000, 0.8660254037844387076, 1.000000000000000000, 0.8660254037844387076, 1.000000000000000000, 0.9330127018922130810, 0.9330127018922194093 ) ) 
 REPRESENTATION_ITEM ( '' )  );
#53321=CARTESIAN_POINT ( 'NONE',  ( -2.229367062499996610, -105.3958333319677365, 3.861377020970582219 ) ) ;
#53326=CARTESIAN_POINT ( 'NONE',  ( -4.458734124999999437, -39.39583333196773651, -2.574251347313719407 ) ) ;
#53328=CARTESIAN_POINT ( 'NONE',  ( -4.458734124999999437, -15.39583333196773474, -2.574251347313719407 ) ) ;
#53329=CARTESIAN_POINT ( 'NONE',  ( -4.458734124999999437, -99.64583333196773651, -2.574251347313719407 ) ) ;
#53331=CARTESIAN_POINT ( 'NONE',  ( -4.458734124999999437, -27.56249999863440081, 0.000000000000000000 ) ) ;
#53335=DIRECTION ( 'NONE',  ( 0.000000000000000000, 0.000000000000000000, 1.000000000000000000 ) ) ;
#53336=CARTESIAN_POINT ( 'NONE',  ( 1.975475456537005874E-15, -109.6249999972688016, 5.000000000000000000 ) ) ;
#53338=CARTESIAN_POINT ( 'NONE',  ( -3.152548672688508926E-16, 3.187500001365594304, -5.148502694627439702 ) ) ;
#53340=CARTESIAN_POINT ( 'NONE',  ( -2.500000000000000444, 1.833333333333332593, -4.330127018922193649 ) ) ;
#53341=CARTESIAN_POINT ( 'NONE',  ( 2.500000000000002220, -93.66666666666665719, 4.330127018922192761 ) ) ;
#53342=CARTESIAN_POINT ( 'NONE',  ( 4.458734124999999437, -27.81249999863440081, -5.460374474430324690E-16 ) ) ;
#53344=CARTESIAN_POINT ( 'NONE',  ( 4.458734124999998549, -73.97916666530106511, -2.574251347313721627 ) ) ;
#53348=CARTESIAN_POINT ( 'NONE',  ( 4.458734124999999437, 1.187500001365596081, -5.460374474430324690E-16 ) ) ;
#53349=CARTESIAN_POINT ( 'NONE',  ( -4.458734124999999437, 27.35416666803225993, -2.574251347313719407 ) ) ;
#53350=CARTESIAN_POINT ( 'NONE',  ( 9.457646018065525792E-16, -43.31249999863440792, 5.148502694627439702 ) ) ;
#53355=CARTESIAN_POINT ( 'NONE',  ( 9.457646018065525792E-16, -69.06249999863439371, 5.148502694627439702 ) ) ;
#53356=CARTESIAN_POINT ( 'NONE',  ( -2.500000000000000444, -104.0416666639354730, -4.330127018922193649 ) ) ;
#53357=ADVANCED_FACE ( 'NONE', ( #40703 ), #50042, .T. ) ;
#53360=CARTESIAN_POINT ( 'NONE',  ( 2.229367062500001939, -108.2291666653010651, 3.861377020970579999 ) ) ;
#53362=CARTESIAN_POINT ( 'NONE',  ( -5.000000000000000000, -52.08333333333332860, -2.886751345948128211 ) ) ;
#53365=VERTEX_POINT ( 'NONE', #11439 ) ;
#53368=CARTESIAN_POINT ( 'NONE',  ( 1.975475456537005874E-15, -27.62499999726881228, 5.000000000000000000 ) ) ;
#53378=ADVANCED_FACE ( 'NONE', ( #10166 ), #55527, .T. ) ;
#53384=CARTESIAN_POINT ( 'NONE',  ( 4.458734125000001214, -43.14583333196773651, 2.574251347313718519 ) ) ;
#53388=CARTESIAN_POINT ( 'NONE',  ( 6.123233995736766282E-16, -120.0000000000000000, -5.000000000000000000 ) ) ;
#53395=CARTESIAN_POINT ( 'NONE',  ( -4.458734124999999437, -91.64583333196773651, -2.574251347313719407 ) ) ;
#53396=CARTESIAN_POINT ( 'NONE',  ( 1.339745962155615144, -34.58034179853028434, 4.999999999999999112 ) ) ;
#53397=ORIENTED_EDGE ( 'NONE', *, *, #23969, .T. ) ;
#53403=EDGE_CURVE ( 'NONE', #17776, #30563, #8344, .T. ) ;
#53404=CARTESIAN_POINT ( 'NONE',  ( 9.457646018065525792E-16, -10.31249999863440614, 5.148502694627439702 ) ) ;
#53407=CYLINDRICAL_SURFACE ( 'NONE', #46981, 5.000000000000000000 ) ;
#53409=( BOUNDED_CURVE ( )  B_SPLINE_CURVE ( 2, ( #35948, #35626, #44955, #50732, #21472, #20520, #44625, #59115, #1236 ),
 .UNSPECIFIED., .F., .F. ) 
 B_SPLINE_CURVE_WITH_KNOTS ( ( 3, 2, 2, 2, 3 ),
 ( 0.5732142857142856762, 0.5738095238095237693, 0.5749999999999999556, 0.5761904761904761418, 0.5767857142857142350 ),
 .UNSPECIFIED. ) 
 CURVE ( )  GEOMETRIC_REPRESENTATION_ITEM ( )  RATIONAL_B_SPLINE_CURVE ( ( 0.9330127018922194093, 0.9330127018922194093, 1.000000000000000000, 0.8660254037844387076, 1.000000000000000000, 0.8660254037844387076, 1.000000000000000000, 0.9330127018922194093, 0.9330127018922194093 ) ) 
 REPRESENTATION_ITEM ( '' )  );
#53410=CARTESIAN_POINT ( 'NONE',  ( -2.229367062500000163, 20.27083333469892779, -3.861377020970580443 ) ) ;
#53411=ORIENTED_EDGE ( 'NONE', *, *, #18866, .F. ) ;
#53412=CARTESIAN_POINT ( 'NONE',  ( 9.457646018065525792E-16, -94.06249999863439371, 5.148502694627439702 ) ) ;
#53415=CARTESIAN_POINT ( 'NONE',  ( -4.458734124999999437, -12.31249999863440259, 0.000000000000000000 ) ) ;
#53416=DIRECTION ( 'NONE',  ( -0.000000000000000000, 1.000000000000000000, -0.000000000000000000 ) ) ;
#53417=DIRECTION ( 'NONE',  ( -0.000000000000000000, 1.000000000000000000, -0.000000000000000000 ) ) ;
#53419=CARTESIAN_POINT ( 'NONE',  ( -5.000000000000000000, -38.87499999726880162, 0.000000000000000000 ) ) ;
#53420=CARTESIAN_POINT ( 'NONE',  ( 2.229367062500001939, 17.02083333469892779, 3.861377020970579999 ) ) ;
#53421=CARTESIAN_POINT ( 'NONE',  ( 2.499999999999998668, -46.20833333060214443, -4.330127018922193649 ) ) ;
#53422=ORIENTED_EDGE ( 'NONE', *, *, #57397, .T. ) ;
#53424=CARTESIAN_POINT ( 'NONE',  ( 9.457646018065525792E-16, -62.06249999863440792, 5.148502694627439702 ) ) ;
#53425=VECTOR ( 'NONE', #57715, 1000.000000000000000 ) ;
#53428=CARTESIAN_POINT ( 'NONE',  ( -4.999999999999999112, 9.083333333333333925, 2.886751345948131764 ) ) ;
#53432=CARTESIAN_POINT ( 'NONE',  ( 4.458734125000001214, -52.89583333196772941, 2.574251347313718519 ) ) ;
#53433=CARTESIAN_POINT ( 'NONE',  ( 2.500000000000002220, -87.54166666393547303, 4.330127018922192761 ) ) ;
#53436=FACE_OUTER_BOUND ( 'NONE', #57142, .T. ) ;
#53438=CARTESIAN_POINT ( 'NONE',  ( 4.458734125000000326, -90.14583333196773651, 2.574251347313718519 ) ) ;
#53440=CARTESIAN_POINT ( 'NONE',  ( 2.500000000000002220, -35.66666666666666430, 4.330127018922192761 ) ) ;
#53442=CARTESIAN_POINT ( 'NONE',  ( 1.339745962155612702, -22.29465819873851729, -5.000000000000000000 ) ) ;
#53444=CARTESIAN_POINT ( 'NONE',  ( -2.229367062500000163, -100.4791666653010651, -3.861377020970580443 ) ) ;
#53445=CARTESIAN_POINT ( 'NONE',  ( -3.152548672688508926E-16, 9.187500001365593860, -5.148502694627439702 ) ) ;
#53448=EDGE_CURVE ( 'NONE', #57369, #43327, #45218, .T. ) ;
#53456=CARTESIAN_POINT ( 'NONE',  ( 1.975475456537005874E-15, -20.74999999999999645, 5.000000000000000000 ) ) ;
#53459=CARTESIAN_POINT ( 'NONE',  ( -2.499999999999996447, -89.70833333060214443, 4.330127018922195425 ) ) ;
#53460=CARTESIAN_POINT ( 'NONE',  ( -4.458734124999998549, -23.47916666530107577, 2.574251347313722516 ) ) ;
#53461=LINE ( 'NONE', #48002, #48108 ) ;
#53471=CARTESIAN_POINT ( 'NONE',  ( 2.229367062499998831, -71.89583333196773651, -3.861377020970580887 ) ) ;
#53474=VECTOR ( 'NONE', #17455, 1000.000000000000000 ) ;
#53475=FACE_OUTER_BOUND ( 'NONE', #15259, .T. ) ;
#53480=CARTESIAN_POINT ( 'NONE',  ( 4.458734124999998549, 0.02083333469892617584, -2.574251347313721627 ) ) ;
#53483=CARTESIAN_POINT ( 'NONE',  ( -5.000000000000000000, 29.04166666939785557, -2.886751345948128211 ) ) ;
#53487=ORIENTED_EDGE ( 'NONE', *, *, #8612, .F. ) ;
#53488=CARTESIAN_POINT ( 'NONE',  ( -2.229367062500000163, -74.47916666530106511, -3.861377020970580443 ) ) ;
#53489=CARTESIAN_POINT ( 'NONE',  ( 5.000000000000000888, -0.4583333306021481479, 2.886751345948126879 ) ) ;
#53490=CARTESIAN_POINT ( 'NONE',  ( -2.229367062500000163, 2.520833334698928230, -3.861377020970580443 ) ) ;
#53493=CARTESIAN_POINT ( 'NONE',  ( 4.458734124999998549, -64.97916666530106511, -2.574251347313721627 ) ) ;
#53494=CARTESIAN_POINT ( 'NONE',  ( -3.535250795749689387E-16, -24.12499999726881583, -5.773502691896257311 ) ) ;
#53496=CARTESIAN_POINT ( 'NONE',  ( 5.000000000000000000, -44.29166666393546592, -2.886751345948130876 ) ) ;
#53497=CARTESIAN_POINT ( 'NONE',  ( 1.975475456537005874E-15, -49.74999999999999289, 5.000000000000000000 ) ) ;
#53498=CARTESIAN_POINT ( 'NONE',  ( -2.499999999999996447, -105.7083333306021444, 4.330127018922195425 ) ) ;
#53499=CARTESIAN_POINT ( 'NONE',  ( 5.000000000000000000, -3.291666663935478354, -2.886751345948130876 ) ) ;
#53500=CARTESIAN_POINT ( 'NONE',  ( 4.458734124999999437, -44.81249999863440081, -5.460374474430324690E-16 ) ) ;
#53501=CARTESIAN_POINT ( 'NONE',  ( -3.152548672688508926E-16, -26.81249999863440436, -5.148502694627439702 ) ) ;
#53504=CARTESIAN_POINT ( 'NONE',  ( 1.060575238724906964E-15, 23.25000000000000000, 5.773502691896257311 ) ) ;
#53507=CARTESIAN_POINT ( 'NONE',  ( 4.458734124999999437, -38.81249999863440081, -5.460374474430324690E-16 ) ) ;
#53508=CARTESIAN_POINT ( 'NONE',  ( -4.999999999999999112, -66.79166666393548724, 2.886751345948131764 ) ) ;
#53511=EDGE_CURVE ( 'NONE', #55695, #47768, #25618, .T. ) ;
#53512=EDGE_CURVE ( 'NONE', #4271, #38750, #2445, .T. ) ;
#53513=CARTESIAN_POINT ( 'NONE',  ( 4.458734124999999437, -74.06249999863440792, -5.460374474430324690E-16 ) ) ;
#53517=DIRECTION ( 'NONE',  ( 0.000000000000000000, 0.000000000000000000, 1.000000000000000000 ) ) ;
#53518=DIRECTION ( 'NONE',  ( 0.000000000000000000, 0.000000000000000000, 1.000000000000000000 ) ) ;
#53519=CARTESIAN_POINT ( 'NONE',  ( 2.499999999999998668, -22.33333333333332860, -4.330127018922193649 ) ) ;
#53521=ORIENTED_EDGE ( 'NONE', *, *, #24694, .F. ) ;
#53525=CARTESIAN_POINT ( 'NONE',  ( -2.499999999999996447, 28.29166666939785202, 4.330127018922195425 ) ) ;
#53531=CARTESIAN_POINT ( 'NONE',  ( -2.500000000000000444, 3.833333333333334370, -4.330127018922193649 ) ) ;
#53534=EDGE_CURVE ( 'NONE', #34309, #59250, #43255, .T. ) ;
#53535=EDGE_CURVE ( 'NONE', #43806, #62517, #3831, .T. ) ;
#53536=CARTESIAN_POINT ( 'NONE',  ( 5.000000000000000000, -12.41666666666666607, -2.886751345948130876 ) ) ;
#53537=CARTESIAN_POINT ( 'NONE',  ( -2.229367062500000163, -21.47916666530107221, -3.861377020970580443 ) ) ;
#53547=CARTESIAN_POINT ( 'NONE',  ( 0.000000000000000000, -120.0000000000000000, 0.000000000000000000 ) ) ;
#53548=CARTESIAN_POINT ( 'NONE',  ( -4.999999999999998224, -67.79166666393547303, 2.886751345948131764 ) ) ;
#53550=ORIENTED_EDGE ( 'NONE', *, *, #27265, .T. ) ;
#53555=EDGE_LOOP ( 'NONE', ( #51106, #54239, #1915, #35446 ) ) ;
#53556=CARTESIAN_POINT ( 'NONE',  ( 0.000000000000000000, -120.0000000000000000, 5.000000000000000000 ) ) ;
#53557=CARTESIAN_POINT ( 'NONE',  ( -4.458734124999999437, 18.68750000136559564, 0.000000000000000000 ) ) ;
#53563=LINE ( 'NONE', #39705, #9639 ) ;
#53564=CARTESIAN_POINT ( 'NONE',  ( 2.229367062499998831, -60.64583333196774362, -3.861377020970580887 ) ) ;
#53567=CARTESIAN_POINT ( 'NONE',  ( -3.152548672688508926E-16, 18.43750000136559564, -5.148502694627439702 ) ) ;
#53568=CARTESIAN_POINT ( 'NONE',  ( 1.339745962155615144, -102.5803417985302843, 4.999999999999999112 ) ) ;
#53569=CARTESIAN_POINT ( 'NONE',  ( -1.339745962155613812, -44.20534180126147561, -5.000000000000000000 ) ) ;
#53570=CARTESIAN_POINT ( 'NONE',  ( 2.229367062499998831, -48.89583333196772941, -3.861377020970580887 ) ) ;
#53571=CARTESIAN_POINT ( 'NONE',  ( -2.500000000000000444, -3.041666663935477910, -4.330127018922193649 ) ) ;
#53575=CARTESIAN_POINT ( 'NONE',  ( 2.229367062500001939, -105.9791666653010651, 3.861377020970579999 ) ) ;
#53576=CARTESIAN_POINT ( 'NONE',  ( -4.458734124999999437, -10.64583333196773829, -2.574251347313719407 ) ) ;
#53577=VERTEX_POINT ( 'NONE', #48064 ) ;
#53579=CARTESIAN_POINT ( 'NONE',  ( 4.458734125000001214, -96.89583333196772230, 2.574251347313718519 ) ) ;
#53581=CARTESIAN_POINT ( 'NONE',  ( -4.458734124999998549, -93.47916666530106511, 2.574251347313722516 ) ) ;
#53582=DIRECTION ( 'NONE',  ( -0.000000000000000000, 1.000000000000000000, -0.000000000000000000 ) ) ;
#53583=CARTESIAN_POINT ( 'NONE',  ( 5.000000000000000000, -54.37499999726880162, -6.123233995736766282E-16 ) ) ;
#53584=CARTESIAN_POINT ( 'NONE',  ( -6.972266317189433020E-16, -40.12499999726880162, -5.000000000000000000 ) ) ;
#53587=CARTESIAN_POINT ( 'NONE',  ( 4.458734124999998549, -17.72916666530106866, -2.574251347313721627 ) ) ;
#53588=CARTESIAN_POINT ( 'NONE',  ( 2.229367062500001939, 9.770833334698927786, 3.861377020970579999 ) ) ;
#53589=CARTESIAN_POINT ( 'NONE',  ( 4.458734124999999437, -59.06249999863440081, -5.460374474430324690E-16 ) ) ;
#53590=CARTESIAN_POINT ( 'NONE',  ( 0.000000000000000000, -120.0000000000000000, 0.000000000000000000 ) ) ;
#53594=VERTEX_POINT ( 'NONE', #33902 ) ;
#53599=CARTESIAN_POINT ( 'NONE',  ( 6.123233995736766282E-16, -120.0000000000000000, -5.000000000000000000 ) ) ;
#53600=CARTESIAN_POINT ( 'NONE',  ( -2.229367062499996610, -86.14583333196773651, 3.861377020970582219 ) ) ;
#53601=CARTESIAN_POINT ( 'NONE',  ( -2.229367062500000163, 18.27083333469892779, -3.861377020970580443 ) ) ;
#53603=CARTESIAN_POINT ( 'NONE',  ( 2.500000000000002220, -93.66666666666665719, 4.330127018922192761 ) ) ;
#53604=DIRECTION ( 'NONE',  ( -0.000000000000000000, 1.000000000000000000, -0.000000000000000000 ) ) ;
#53607=CARTESIAN_POINT ( 'NONE',  ( 2.500000000000002220, -72.66666666666667140, 4.330127018922192761 ) ) ;
#53612=ORIENTED_EDGE ( 'NONE', *, *, #43702, .T. ) ;
#53616=ADVANCED_FACE ( 'NONE', ( #4322 ), #14513, .T. ) ;
#53617=EDGE_CURVE ( 'NONE', #47264, #3800, #47406, .T. ) ;
#53626=CARTESIAN_POINT ( 'NONE',  ( 6.123233995736766282E-16, -120.0000000000000000, -5.000000000000000000 ) ) ;
#53627=CARTESIAN_POINT ( 'NONE',  ( -3.152548672688508926E-16, -57.81249999863440081, -5.148502694627439702 ) ) ;
#53635=CARTESIAN_POINT ( 'NONE',  ( 4.458734124999999437, -105.0624999986344079, -5.460374474430324690E-16 ) ) ;
#53639=CARTESIAN_POINT ( 'NONE',  ( 9.457646018065525792E-16, -36.06249999863440792, 5.148502694627439702 ) ) ;
#53641=CARTESIAN_POINT ( 'NONE',  ( -5.000000000000000000, -2.083333333333333037, -2.886751345948128211 ) ) ;
#53642=CARTESIAN_POINT ( 'NONE',  ( 4.458734124999998549, -13.72916666530107399, -2.574251347313721627 ) ) ;
#53643=CARTESIAN_POINT ( 'NONE',  ( -2.229367062499996610, -99.39583333196773651, 3.861377020970582219 ) ) ;
#53644=ORIENTED_EDGE ( 'NONE', *, *, #25966, .F. ) ;
#53646=CARTESIAN_POINT ( 'NONE',  ( -2.229367062500000163, -28.72916666530107221, -3.861377020970580443 ) ) ;
#53650=CARTESIAN_POINT ( 'NONE',  ( -6.972266317189433020E-16, -16.25000000000000000, -5.000000000000000000 ) ) ;
#53653=CARTESIAN_POINT ( 'NONE',  ( -4.458734124999999437, 2.437500001365593860, 0.000000000000000000 ) ) ;
#53656=LINE ( 'NONE', #38536, #34050 ) ;
#53657=CARTESIAN_POINT ( 'NONE',  ( 2.499999999999998668, -95.33333333333332860, -4.330127018922193649 ) ) ;
#53658=CARTESIAN_POINT ( 'NONE',  ( -3.152548672688508926E-16, -29.56249999863440436, -5.148502694627439702 ) ) ;
#53660=CARTESIAN_POINT ( 'NONE',  ( -4.458734124999999437, -77.64583333196773651, -2.574251347313719407 ) ) ;
#53662=CARTESIAN_POINT ( 'NONE',  ( 1.975475456537005874E-15, -101.6249999972688158, 5.000000000000000000 ) ) ;
#53664=EDGE_CURVE ( 'NONE', #3550, #7844, #54786, .T. ) ;
#53665=CARTESIAN_POINT ( 'NONE',  ( 4.458734124999999437, -3.812499998634408360, -5.460374474430324690E-16 ) ) ;
#53666=CARTESIAN_POINT ( 'NONE',  ( 4.458734124999998549, 25.02083333469892423, -2.574251347313721627 ) ) ;
#53667=CARTESIAN_POINT ( 'NONE',  ( -2.229367062499996610, -44.39583333196774362, 3.861377020970582219 ) ) ;
#53672=CARTESIAN_POINT ( 'NONE',  ( -4.458734124999999437, -69.31249999863439371, 0.000000000000000000 ) ) ;
#53673=CARTESIAN_POINT ( 'NONE',  ( -5.000000000000000000, -107.8749999972687874, 0.000000000000000000 ) ) ;
#53674=( BOUNDED_CURVE ( )  B_SPLINE_CURVE ( 2, ( #13135, #33693, #8934, #22800, #48483, #61722, #18273, #62978, #37899 ),
 .UNSPECIFIED., .F., .F. ) 
 B_SPLINE_CURVE_WITH_KNOTS ( ( 3, 2, 2, 2, 3 ),
 ( 0.1339285714285714246, 0.1345238095238095177, 0.1357142857142857040, 0.1369047619047619180, 0.1375000000000000111 ),
 .UNSPECIFIED. ) 
 CURVE ( )  GEOMETRIC_REPRESENTATION_ITEM ( )  RATIONAL_B_SPLINE_CURVE ( ( 0.9330127018922194093, 0.9330127018922194093, 1.000000000000000000, 0.8660254037844387076, 1.000000000000000000, 0.8660254037844387076, 1.000000000000000000, 0.9330127018922194093, 0.9330127018922194093 ) ) 
 REPRESENTATION_ITEM ( '' )  );
#53679=CARTESIAN_POINT ( 'NONE',  ( 5.000000000000000000, -53.41666666666667140, -2.886751345948129988 ) ) ;
#53680=CARTESIAN_POINT ( 'NONE',  ( -4.999999999999998224, -65.91666666666667140, 2.886751345948131764 ) ) ;
#53681=DIRECTION ( 'NONE',  ( -0.000000000000000000, 1.000000000000000000, -0.000000000000000000 ) ) ;
#53682=ORIENTED_EDGE ( 'NONE', *, *, #44729, .F. ) ;
#53684=CARTESIAN_POINT ( 'NONE',  ( -5.000000000000000000, 12.91666666666666607, -2.886751345948128211 ) ) ;
#53692=EDGE_LOOP ( 'NONE', ( #39457, #63209, #18123, #41768 ) ) ;
#53700=CARTESIAN_POINT ( 'NONE',  ( -2.229367062499996610, -42.39583333196773651, 3.861377020970582219 ) ) ;
#53709=CARTESIAN_POINT ( 'NONE',  ( 4.458734125000001214, -90.14583333196773651, 2.574251347313718519 ) ) ;
#53711=ORIENTED_EDGE ( 'NONE', *, *, #42579, .T. ) ;
#53712=CARTESIAN_POINT ( 'NONE',  ( -5.000000000000000000, -47.00000000000000000, 0.000000000000000000 ) ) ;
#53715=CARTESIAN_POINT ( 'NONE',  ( 1.339745962155612702, -82.16965819600734733, -5.000000000000000000 ) ) ;
#53717=ORIENTED_EDGE ( 'NONE', *, *, #48287, .T. ) ;
#53718=CARTESIAN_POINT ( 'NONE',  ( 1.339745962155612702, -78.29465819873851729, -5.000000000000000000 ) ) ;
#53719=CARTESIAN_POINT ( 'NONE',  ( 4.458734124999998549, -13.97916666530107221, -2.574251347313721627 ) ) ;
#53724=CARTESIAN_POINT ( 'NONE',  ( -2.229367062500000163, 22.27083333469892423, -3.861377020970580443 ) ) ;
#53725=ORIENTED_EDGE ( 'NONE', *, *, #25215, .T. ) ;
#53726=CARTESIAN_POINT ( 'NONE',  ( -4.458734124999999437, -95.39583333196773651, -2.574251347313719407 ) ) ;
#53727=CARTESIAN_POINT ( 'NONE',  ( 1.975475456537005874E-15, -33.62499999726880873, 5.000000000000000000 ) ) ;
#53729=CARTESIAN_POINT ( 'NONE',  ( 2.229367062499998831, -16.64583333196773651, -3.861377020970580887 ) ) ;
#53730=CARTESIAN_POINT ( 'NONE',  ( -2.499999999999996447, -84.70833333060214443, 4.330127018922195425 ) ) ;
#53731=CARTESIAN_POINT ( 'NONE',  ( -2.499999999999996447, -42.70833333060214443, 4.330127018922195425 ) ) ;
#53732=CYLINDRICAL_SURFACE ( 'NONE', #46242, 5.000000000000000000 ) ;
#53733=CARTESIAN_POINT ( 'NONE',  ( 4.458734125000000326, 13.10416666803226171, 2.574251347313718519 ) ) ;
#53734=CARTESIAN_POINT ( 'NONE',  ( 1.975475456537005874E-15, -46.62499999726880873, 5.000000000000000000 ) ) ;
#53737=CARTESIAN_POINT ( 'NONE',  ( -3.152548672688508926E-16, -60.56249999863440792, -5.148502694627439702 ) ) ;
#53739=( BOUNDED_CURVE ( )  B_SPLINE_CURVE ( 2, ( #35738, #30905, #60508, #11597, #6789, #45703, #55683, #46018, #11913 ),
 .UNSPECIFIED., .F., .F. ) 
 B_SPLINE_CURVE_WITH_KNOTS ( ( 3, 2, 2, 2, 3 ),
 ( 0.3089285714285714413, 0.3095238095238095344, 0.3107142857142857206, 0.3119047619047619069, 0.3125000000000000000 ),
 .UNSPECIFIED. ) 
 CURVE ( )  GEOMETRIC_REPRESENTATION_ITEM ( )  RATIONAL_B_SPLINE_CURVE ( ( 0.9330127018922194093, 0.9330127018922194093, 1.000000000000000000, 0.8660254037844387076, 1.000000000000000000, 0.8660254037844387076, 1.000000000000000000, 0.9330127018922194093, 0.9330127018922194093 ) ) 
 REPRESENTATION_ITEM ( '' )  );
#53741=CARTESIAN_POINT ( 'NONE',  ( -4.999999999999999112, 12.08333333333333037, 2.886751345948131764 ) ) ;
#53743=DIRECTION ( 'NONE',  ( -0.000000000000000000, 1.000000000000000000, -0.000000000000000000 ) ) ;
#53744=CARTESIAN_POINT ( 'NONE',  ( 2.229367062499998831, -55.64583333196773651, -3.861377020970580887 ) ) ;
#53745=CARTESIAN_POINT ( 'NONE',  ( 2.500000000000002220, -91.54166666393547303, 4.330127018922192761 ) ) ;
#53746=CARTESIAN_POINT ( 'NONE',  ( 0.000000000000000000, -120.0000000000000000, 0.000000000000000000 ) ) ;
#53747=CARTESIAN_POINT ( 'NONE',  ( -5.926426369611017623E-15, 25.37500000273118062, 5.000000000000000000 ) ) ;
#53748=LINE ( 'NONE', #54065, #38774 ) ;
#53750=CARTESIAN_POINT ( 'NONE',  ( 5.000000000000000000, -35.50000000000000711, -6.123233995736766282E-16 ) ) ;
#53754=CARTESIAN_POINT ( 'NONE',  ( 9.457646018065525792E-16, -102.0624999986344079, 5.148502694627439702 ) ) ;
#53755=CARTESIAN_POINT ( 'NONE',  ( -4.458734124999999437, 3.354166668032260823, -2.574251347313719407 ) ) ;
#53759=CARTESIAN_POINT ( 'NONE',  ( -6.031010364368858512E-14, 3.249999999999997335, 5.000000000000000000 ) ) ;
#53763=CARTESIAN_POINT ( 'NONE',  ( 0.000000000000000000, -120.0000000000000000, 0.000000000000000000 ) ) ;
#53764=CARTESIAN_POINT ( 'NONE',  ( 1.975475456537005874E-15, -59.62499999726880873, 5.000000000000000000 ) ) ;
#53770=CARTESIAN_POINT ( 'NONE',  ( -2.229367062499996610, -26.39583333196774007, 3.861377020970582219 ) ) ;
#53771=CARTESIAN_POINT ( 'NONE',  ( -5.000000000000000000, 22.04166666939785202, -2.886751345948128211 ) ) ;
#53781=CARTESIAN_POINT ( 'NONE',  ( -4.458734124999998549, -75.47916666530107932, 2.574251347313722516 ) ) ;
#53783=( LENGTH_UNIT ( ) NAMED_UNIT ( * ) SI_UNIT ( .MILLI., .METRE. ) );
#53784=ORIENTED_EDGE ( 'NONE', *, *, #40874, .F. ) ;
#53785=CARTESIAN_POINT ( 'NONE',  ( 1.243387493232115550E-13, -20.12499999726881228, -5.000000000000000000 ) ) ;
#53788=EDGE_CURVE ( 'NONE', #16917, #47768, #58965, .T. ) ;
#53789=CARTESIAN_POINT ( 'NONE',  ( 2.229367062499998831, 2.104166668032262599, -3.861377020970580887 ) ) ;
#53795=CARTESIAN_POINT ( 'NONE',  ( 0.000000000000000000, -120.0000000000000000, 0.000000000000000000 ) ) ;
#53797=ORIENTED_EDGE ( 'NONE', *, *, #13362, .T. ) ;
#53798=CARTESIAN_POINT ( 'NONE',  ( 4.458734124999999437, -76.81249999863440792, -5.460374474430324690E-16 ) ) ;
#53800=CARTESIAN_POINT ( 'NONE',  ( 4.458734125000001214, 3.104166668032260379, 2.574251347313718519 ) ) ;
#53801=VECTOR ( 'NONE', #16850, 1000.000000000000000 ) ;
#53802=CARTESIAN_POINT ( 'NONE',  ( 2.493747252781420335E-13, -43.12499999726882294, -5.000000000000000000 ) ) ;
#53803=CARTESIAN_POINT ( 'NONE',  ( 4.458734124999998549, -66.97916666530107932, -2.574251347313721627 ) ) ;
#53804=CARTESIAN_POINT ( 'NONE',  ( 5.000000000000000888, -23.45833333060214443, 2.886751345948126879 ) ) ;
#53805=EDGE_CURVE ( 'NONE', #52846, #36859, #10716, .T. ) ;
#53807=CARTESIAN_POINT ( 'NONE',  ( 1.339745962155612702, -44.16965819600732601, -5.000000000000000000 ) ) ;
#53809=CARTESIAN_POINT ( 'NONE',  ( 1.975475456537005874E-15, -20.74999999999999645, 5.000000000000000000 ) ) ;
#53810=CARTESIAN_POINT ( 'NONE',  ( -2.229367062500000163, -44.47916666530106511, -3.861377020970580443 ) ) ;
#53812=CARTESIAN_POINT ( 'NONE',  ( -4.458734124999999437, -25.64583333196773651, -2.574251347313719407 ) ) ;
#53815=CARTESIAN_POINT ( 'NONE',  ( -2.499999999999996447, 25.16666666666666430, 4.330127018922195425 ) ) ;
#53818=CARTESIAN_POINT ( 'NONE',  ( 4.458734125000001214, -39.89583333196772941, 2.574251347313718519 ) ) ;
#53819=CARTESIAN_POINT ( 'NONE',  ( -2.499999999999996447, -74.70833333060214443, 4.330127018922195425 ) ) ;
#53823=CARTESIAN_POINT ( 'NONE',  ( -4.458734124999999437, -73.64583333196773651, -2.574251347313719407 ) ) ;
#53828=CARTESIAN_POINT ( 'NONE',  ( 5.000000000000000000, -23.41666666666667140, -2.886751345948129988 ) ) ;
#53832=ORIENTED_EDGE ( 'NONE', *, *, #4022, .F. ) ;
#53834=CARTESIAN_POINT ( 'NONE',  ( 2.500000000000002220, 27.45833333606451632, 4.330127018922192761 ) ) ;
#53835=CARTESIAN_POINT ( 'NONE',  ( 1.975475456537005874E-15, -29.74999999999999645, 5.000000000000000000 ) ) ;
#53837=CARTESIAN_POINT ( 'NONE',  ( -1.339745962155585168, 7.919658201469705006, -5.000000000000015987 ) ) ;
#53842=CARTESIAN_POINT ( 'NONE',  ( 1.339745962155729053, -91.16965819600733312, -4.999999999999933387 ) ) ;
#53845=CARTESIAN_POINT ( 'NONE',  ( 4.458734124999999437, -21.81249999863440436, -5.460374474430324690E-16 ) ) ;
#53846=CARTESIAN_POINT ( 'NONE',  ( 1.975475456537005874E-15, -71.62499999726878741, 5.000000000000000000 ) ) ;
#53851=ORIENTED_EDGE ( 'NONE', *, *, #58253, .F. ) ;
#53853=VERTEX_POINT ( 'NONE', #25506 ) ;
#53856=ORIENTED_EDGE ( 'NONE', *, *, #22740, .F. ) ;
#53857=CARTESIAN_POINT ( 'NONE',  ( 1.975475456537005874E-15, 11.24999999999999822, 5.000000000000000000 ) ) ;
#53861=EDGE_CURVE ( 'NONE', #50378, #11950, #12838, .T. ) ;
#53863=( BOUNDED_CURVE ( )  B_SPLINE_CURVE ( 2, ( #51753, #35692, #36957, #12192, #26347, #60142, #11863, #31479, #30858 ),
 .UNSPECIFIED., .F., .F. ) 
 B_SPLINE_CURVE_WITH_KNOTS ( ( 3, 2, 2, 2, 3 ),
 ( 0.05178571428571428908, 0.05238095238095238221, 0.05357142857142856845, 0.05476190476190476164, 0.05535714285714286170 ),
 .UNSPECIFIED. ) 
 CURVE ( )  GEOMETRIC_REPRESENTATION_ITEM ( )  RATIONAL_B_SPLINE_CURVE ( ( 0.9330127018922194093, 0.9330127018922197424, 1.000000000000000000, 0.8660254037844387076, 1.000000000000000000, 0.8660254037844387076, 1.000000000000000000, 0.9330127018922189652, 0.9330127018922194093 ) ) 
 REPRESENTATION_ITEM ( '' )  );
#53867=CARTESIAN_POINT ( 'NONE',  ( -2.229367062499996610, 18.85416666803225993, 3.861377020970582219 ) ) ;
#53869=ORIENTED_EDGE ( 'NONE', *, *, #23584, .F. ) ;
#53874=CARTESIAN_POINT ( 'NONE',  ( -6.972266317189433020E-16, -103.2500000000000000, -5.000000000000000000 ) ) ;
#53875=CARTESIAN_POINT ( 'NONE',  ( -3.152548672688508926E-16, -61.56249999863440081, -5.148502694627439702 ) ) ;
#53877=CARTESIAN_POINT ( 'NONE',  ( 4.458734124999999437, 19.18750000136559564, -5.460374474430324690E-16 ) ) ;
#53880=CARTESIAN_POINT ( 'NONE',  ( -4.458734124999999437, -51.56249999863440792, 0.000000000000000000 ) ) ;
#53881=CARTESIAN_POINT ( 'NONE',  ( -2.500000000000000444, -10.04166666393547658, -4.330127018922193649 ) ) ;
#53882=CARTESIAN_POINT ( 'NONE',  ( -5.000000000000000000, -93.08333333333332860, -2.886751345948128211 ) ) ;
#53883=ADVANCED_FACE ( 'NONE', ( #6218 ), #7176, .T. ) ;
#53886=CARTESIAN_POINT ( 'NONE',  ( 4.458734124999999437, -108.8124999986343937, -5.460374474430324690E-16 ) ) ;
#53887=CARTESIAN_POINT ( 'NONE',  ( -2.229367062499996610, -10.39583333196773829, 3.861377020970582219 ) ) ;
#53888=ORIENTED_EDGE ( 'NONE', *, *, #3233, .F. ) ;
#53890=CARTESIAN_POINT ( 'NONE',  ( 2.229367062499998831, -98.64583333196773651, -3.861377020970580887 ) ) ;
#53892=CARTESIAN_POINT ( 'NONE',  ( 4.458734124999999437, -96.06249999863440792, -5.460374474430324690E-16 ) ) ;
#53893=CARTESIAN_POINT ( 'NONE',  ( -2.499999999999996447, -57.70833333060214443, 4.330127018922195425 ) ) ;
#53894=CARTESIAN_POINT ( 'NONE',  ( 5.000000000000000888, -5.583333333333336590, 2.886751345948126879 ) ) ;
#53895=AXIS2_PLACEMENT_3D ( 'NONE', #42470, #18030, #9948 ) ;
#53898=CARTESIAN_POINT ( 'NONE',  ( -4.458734124999999437, -18.31249999863440792, 0.000000000000000000 ) ) ;
#53899=CARTESIAN_POINT ( 'NONE',  ( 4.458734125000001214, 6.854166668032259935, 2.574251347313718519 ) ) ;
#53900=CARTESIAN_POINT ( 'NONE',  ( -2.229367062499996610, -56.39583333196773651, 3.861377020970582219 ) ) ;
#53904=CARTESIAN_POINT ( 'NONE',  ( 2.499999999999998668, -8.333333333333332149, -4.330127018922193649 ) ) ;
#53905=ORIENTED_EDGE ( 'NONE', *, *, #31517, .T. ) ;
#53908=CARTESIAN_POINT ( 'NONE',  ( -4.999999999999998224, -91.79166666393547303, 2.886751345948131764 ) ) ;
#53910=CARTESIAN_POINT ( 'NONE',  ( 2.229367062499998831, -85.64583333196773651, -3.861377020970580887 ) ) ;
#53911=CARTESIAN_POINT ( 'NONE',  ( -4.458734124999998549, 16.52083333469892779, 2.574251347313722516 ) ) ;
#53913=CARTESIAN_POINT ( 'NONE',  ( 1.339745962155612702, -0.2946581987385212820, -5.000000000000000000 ) ) ;
#53914=CARTESIAN_POINT ( 'NONE',  ( -2.500000000000000444, -7.166666666666668739, -4.330127018922193649 ) ) ;
#53917=CARTESIAN_POINT ( 'NONE',  ( -5.000000000000000000, -76.08333333333332860, -2.886751345948128211 ) ) ;
#53920=ORIENTED_EDGE ( 'NONE', *, *, #51594, .T. ) ;
#53921=CARTESIAN_POINT ( 'NONE',  ( 0.000000000000000000, -120.0000000000000000, 0.000000000000000000 ) ) ;
#53935=CARTESIAN_POINT ( 'NONE',  ( -4.458734124999999437, -59.64583333196773651, -2.574251347313719407 ) ) ;
#53938=EDGE_LOOP ( 'NONE', ( #13767, #12412, #24910, #50345 ) ) ;
#53946=CARTESIAN_POINT ( 'NONE',  ( -4.458734124999999437, -102.5624999986344079, 0.000000000000000000 ) ) ;
#53951=CARTESIAN_POINT ( 'NONE',  ( 4.458734124999999437, -37.81249999863440792, -5.460374474430324690E-16 ) ) ;
#53954=CARTESIAN_POINT ( 'NONE',  ( -5.000000000000000000, -71.00000000000000000, 0.000000000000000000 ) ) ;
#53955=CARTESIAN_POINT ( 'NONE',  ( 9.457646018065525792E-16, -12.06249999863440081, 5.148502694627439702 ) ) ;
#53956=CARTESIAN_POINT ( 'NONE',  ( -4.458734124999997661, -101.4791666653010651, 2.574251347313722516 ) ) ;
#53959=CARTESIAN_POINT ( 'NONE',  ( 2.229367062499998831, -30.89583333196773651, -3.861377020970580887 ) ) ;
#53960=CARTESIAN_POINT ( 'NONE',  ( 5.000000000000000000, 8.625000002731184168, -6.123233995736766282E-16 ) ) ;
#53967=CARTESIAN_POINT ( 'NONE',  ( -6.972266317189433020E-16, 12.87500000273118417, -5.000000000000000000 ) ) ;
#53968=( BOUNDED_CURVE ( )  B_SPLINE_CURVE ( 2, ( #44404, #49555, #14186, #19648, #63100, #363, #43767, #19966, #54392 ),
 .UNSPECIFIED., .F., .F. ) 
 B_SPLINE_CURVE_WITH_KNOTS ( ( 3, 2, 2, 2, 3 ),
 ( 0.6339285714285713969, 0.6345238095238094900, 0.6357142857142856762, 0.6369047619047618625, 0.6374999999999999556 ),
 .UNSPECIFIED. ) 
 CURVE ( )  GEOMETRIC_REPRESENTATION_ITEM ( )  RATIONAL_B_SPLINE_CURVE ( ( 0.9330127018922194093, 0.9330127018922194093, 1.000000000000000000, 0.8660254037844387076, 1.000000000000000000, 0.8660254037844387076, 1.000000000000000000, 0.9330127018922194093, 0.9330127018922194093 ) ) 
 REPRESENTATION_ITEM ( '' )  );
#53969=CARTESIAN_POINT ( 'NONE',  ( 2.229367062499998831, 5.104166668032261711, -3.861377020970580887 ) ) ;
#53970=EDGE_LOOP ( 'NONE', ( #53134, #29966, #33168, #16242 ) ) ;
#53972=EDGE_CURVE ( 'NONE', #19776, #42151, #26468, .T. ) ;
#53973=CARTESIAN_POINT ( 'NONE',  ( 1.339745962155612702, 2.705341801261480050, -5.000000000000000000 ) ) ;
#53974=CARTESIAN_POINT ( 'NONE',  ( 5.000000000000000000, -96.50000000000000000, -6.123233995736766282E-16 ) ) ;
#53975=CARTESIAN_POINT ( 'NONE',  ( 4.458734124999999437, -28.81249999863440436, -5.460374474430324690E-16 ) ) ;
#53976=CARTESIAN_POINT ( 'NONE',  ( 5.000000000000000888, -95.58333333333334281, 2.886751345948126879 ) ) ;
#53977=CARTESIAN_POINT ( 'NONE',  ( -2.229367062500000163, -81.72916666530106511, -3.861377020970580443 ) ) ;
#53982=CARTESIAN_POINT ( 'NONE',  ( 4.458734124999999437, -1.812499998634406584, -5.460374474430324690E-16 ) ) ;
#53983=CARTESIAN_POINT ( 'NONE',  ( 1.975475456537005874E-15, -81.62499999726881583, 5.000000000000000000 ) ) ;
#53984=CARTESIAN_POINT ( 'NONE',  ( -2.229367062500000163, -41.72916666530107932, -3.861377020970580443 ) ) ;
#53985=CARTESIAN_POINT ( 'NONE',  ( -4.999999999999998224, -45.79166666393547303, 2.886751345948131764 ) ) ;
#53988=CARTESIAN_POINT ( 'NONE',  ( -4.458734124999999437, -70.31249999863439371, 0.000000000000000000 ) ) ;
#53989=CARTESIAN_POINT ( 'NONE',  ( 5.000000000000000000, -105.3749999972688158, -6.123233995736766282E-16 ) ) ;
#53990=AXIS2_PLACEMENT_3D ( 'NONE', #15959, #24974, #21104 ) ;
#53992=CARTESIAN_POINT ( 'NONE',  ( -1.339745962155613812, -65.20534180126146850, -5.000000000000000000 ) ) ;
#53993=CARTESIAN_POINT ( 'NONE',  ( 6.123233995736766282E-16, -120.0000000000000000, -5.000000000000000000 ) ) ;
#53995=CARTESIAN_POINT ( 'NONE',  ( 2.499999999999998668, -58.33333333333333570, -4.330127018922193649 ) ) ;
#53996=DIRECTION ( 'NONE',  ( -1.000000000000000000, 0.000000000000000000, 1.061635649774262822E-14 ) ) ;
#54006=ORIENTED_EDGE ( 'NONE', *, *, #45205, .F. ) ;
#54007=CARTESIAN_POINT ( 'NONE',  ( -6.972266317189433020E-16, -35.12499999726880873, -5.000000000000000000 ) ) ;
#54010=ORIENTED_EDGE ( 'NONE', *, *, #62138, .F. ) ;
#54014=CARTESIAN_POINT ( 'NONE',  ( -4.458734124999998549, -42.47916666530107932, 2.574251347313722516 ) ) ;
#54020=LINE ( 'NONE', #9954, #2059 ) ;
#54022=CARTESIAN_POINT ( 'NONE',  ( -2.229367062499996610, -90.39583333196773651, 3.861377020970582219 ) ) ;
#54025=DIRECTION ( 'NONE',  ( -0.000000000000000000, 1.000000000000000000, -0.000000000000000000 ) ) ;
#54030=CARTESIAN_POINT ( 'NONE',  ( 4.458734124999998549, 3.270833334698929118, -2.574251347313721627 ) ) ;
#54031=AXIS2_PLACEMENT_3D ( 'NONE', #6595, #17445, #13563 ) ;
#54032=CARTESIAN_POINT ( 'NONE',  ( 9.457646018065525792E-16, -17.31249999863440436, 5.148502694627439702 ) ) ;
#54035=CARTESIAN_POINT ( 'NONE',  ( -1.339745962155613812, -74.08034179853029855, -5.000000000000000000 ) ) ;
#54037=CARTESIAN_POINT ( 'NONE',  ( -3.152548672688508926E-16, 23.18750000136559564, -5.148502694627439702 ) ) ;
#54038=VERTEX_POINT ( 'NONE', #56385 ) ;
#54039=CARTESIAN_POINT ( 'NONE',  ( -2.229367062499996610, -95.14583333196773651, 3.861377020970582219 ) ) ;
#54040=CARTESIAN_POINT ( 'NONE',  ( -6.972266317189433020E-16, -47.24999999999999289, -5.000000000000000000 ) ) ;
#54042=CARTESIAN_POINT ( 'NONE',  ( 2.229367062499998831, -11.64583333196774007, -3.861377020970580887 ) ) ;
#54043=CYLINDRICAL_SURFACE ( 'NONE', #6764, 5.000000000000000000 ) ;
#54047=CARTESIAN_POINT ( 'NONE',  ( 5.000000000000000000, -40.29166666393548013, -2.886751345948129988 ) ) ;
#54048=CARTESIAN_POINT ( 'NONE',  ( -4.999999999999998224, 21.20833333606451987, 2.886751345948131764 ) ) ;
#54049=CARTESIAN_POINT ( 'NONE',  ( 4.458734124999999437, 14.18750000136559386, -5.460374474430324690E-16 ) ) ;
#54051=ORIENTED_EDGE ( 'NONE', *, *, #40459, .T. ) ;
#54053=CARTESIAN_POINT ( 'NONE',  ( 2.229367062500001939, -59.97916666530106511, 3.861377020970579999 ) ) ;
#54056=CARTESIAN_POINT ( 'NONE',  ( 2.499999999999998668, 4.666666666666666075, -4.330127018922193649 ) ) ;
#54059=CARTESIAN_POINT ( 'NONE',  ( -2.229367062500000163, -54.47916666530107221, -3.861377020970580443 ) ) ;
#54060=CARTESIAN_POINT ( 'NONE',  ( -5.000000000000000000, -89.87499999726880162, 0.000000000000000000 ) ) ;
#54061=CARTESIAN_POINT ( 'NONE',  ( -2.229367062499996610, -35.14583333196772941, 3.861377020970582219 ) ) ;
#54063=( BOUNDED_CURVE ( )  B_SPLINE_CURVE ( 2, ( #20310, #15490, #50209, #1663, #49570, #44737, #40869, #378, #26088 ),
 .UNSPECIFIED., .F., .F. ) 
 B_SPLINE_CURVE_WITH_KNOTS ( ( 3, 2, 2, 2, 3 ),
 ( 0.6374999999999999556, 0.6380952380952380487, 0.6392857142857142350, 0.6404761904761904212, 0.6410714285714286254 ),
 .UNSPECIFIED. ) 
 CURVE ( )  GEOMETRIC_REPRESENTATION_ITEM ( )  RATIONAL_B_SPLINE_CURVE ( ( 0.9330127018922194093, 0.9330127018922194093, 1.000000000000000000, 0.8660254037844387076, 1.000000000000000000, 0.8660254037844387076, 1.000000000000000000, 0.9330127018922130810, 0.9330127018922194093 ) ) 
 REPRESENTATION_ITEM ( '' )  );
#54064=CARTESIAN_POINT ( 'NONE',  ( 2.500000000000002220, 25.45833333606451987, 4.330127018922192761 ) ) ;
#54065=CARTESIAN_POINT ( 'NONE',  ( -8.660254037844341113, 30.00000000000000000, 6.047423072554883697E-14 ) ) ;
#54067=CARTESIAN_POINT ( 'NONE',  ( 5.000000000000000000, -39.49999999999999289, -6.123233995736766282E-16 ) ) ;
#54068=CARTESIAN_POINT ( 'NONE',  ( 1.975475456537005874E-15, -98.62499999726880162, 5.000000000000000000 ) ) ;
#54070=ORIENTED_EDGE ( 'NONE', *, *, #9786, .T. ) ;
#54071=CARTESIAN_POINT ( 'NONE',  ( -3.152548672688508926E-16, -99.56249999863440792, -5.148502694627439702 ) ) ;
#54072=CARTESIAN_POINT ( 'NONE',  ( 4.458734125000001214, 1.854166668032262155, 2.574251347313718519 ) ) ;
#54074=CARTESIAN_POINT ( 'NONE',  ( 1.339745962155615144, -80.70534180126146850, 4.999999999999999112 ) ) ;
#54078=VECTOR ( 'NONE', #36181, 1000.000000000000000 ) ;
#54082=ORIENTED_EDGE ( 'NONE', *, *, #26823, .F. ) ;
#54085=CARTESIAN_POINT ( 'NONE',  ( 1.339745962155612702, -20.29465819873851729, -5.000000000000000000 ) ) ;
#54087=CARTESIAN_POINT ( 'NONE',  ( 4.458734125000001214, -27.14583333196774717, 2.574251347313718519 ) ) ;
#54088=CARTESIAN_POINT ( 'NONE',  ( -5.000000000000000000, 22.12500000273118417, 0.000000000000000000 ) ) ;
#54096=DIRECTION ( 'NONE',  ( -0.000000000000000000, 1.000000000000000000, -0.000000000000000000 ) ) ;
#54097=VERTEX_POINT ( 'NONE', #11977 ) ;
#54098=CARTESIAN_POINT ( 'NONE',  ( -4.458734124999999437, -70.64583333196773651, -2.574251347313719407 ) ) ;
#54103=CARTESIAN_POINT ( 'NONE',  ( 1.975475456537005874E-15, -48.74999999999999289, 5.000000000000000000 ) ) ;
#54105=CARTESIAN_POINT ( 'NONE',  ( -4.458734124999998549, -1.479166665301071770, 2.574251347313722516 ) ) ;
#54107=CYLINDRICAL_SURFACE ( 'NONE', #28590, 5.000000000000000000 ) ;
#54108=CARTESIAN_POINT ( 'NONE',  ( -4.999999999999998224, -44.91666666666666430, 2.886751345948131764 ) ) ;
#54114=VECTOR ( 'NONE', #21890, 1000.000000000000000 ) ;
#54115=ORIENTED_EDGE ( 'NONE', *, *, #61459, .F. ) ;
#54116=CARTESIAN_POINT ( 'NONE',  ( 2.229367062500001939, -82.97916666530106511, 3.861377020970579999 ) ) ;
#54118=CARTESIAN_POINT ( 'NONE',  ( 4.458734124999999437, 3.187500001365594304, -5.460374474430324690E-16 ) ) ;
#54119=CARTESIAN_POINT ( 'NONE',  ( 5.000000000000000888, -87.58333333333332860, 2.886751345948126879 ) ) ;
#54120=CARTESIAN_POINT ( 'NONE',  ( -1.339745962155497683, -43.08034179853029855, -5.000000000000066613 ) ) ;
#54121=CARTESIAN_POINT ( 'NONE',  ( 2.229367062499998831, -62.89583333196774362, -3.861377020970580887 ) ) ;
#54122=CARTESIAN_POINT ( 'NONE',  ( 5.000000000000000000, -25.37499999726881583, -6.123233995736766282E-16 ) ) ;
#54124=CARTESIAN_POINT ( 'NONE',  ( -4.458734124999999437, 27.68750000136559208, 0.000000000000000000 ) ) ;
#54125=CARTESIAN_POINT ( 'NONE',  ( 5.000000000000000000, -49.50000000000000000, -6.123233995736766282E-16 ) ) ;
#54126=( LENGTH_UNIT ( ) NAMED_UNIT ( * ) SI_UNIT ( .MILLI., .METRE. ) );
#54127=CARTESIAN_POINT ( 'NONE',  ( 2.229367062500001939, -43.97916666530106511, 3.861377020970579999 ) ) ;
#54128=CARTESIAN_POINT ( 'NONE',  ( 2.229367062499998831, -30.89583333196773651, -3.861377020970580887 ) ) ;
#54131=CARTESIAN_POINT ( 'NONE',  ( 2.499999999999998668, 18.66666666666666430, -4.330127018922193649 ) ) ;
#54133=CARTESIAN_POINT ( 'NONE',  ( -4.999999999999998224, -49.91666666666667140, 2.886751345948131764 ) ) ;
#54134=CARTESIAN_POINT ( 'NONE',  ( 4.458734125000001214, -35.89583333196773651, 2.574251347313718519 ) ) ;
#54135=CARTESIAN_POINT ( 'NONE',  ( 2.499999999999998668, -71.20833333060214443, -4.330127018922193649 ) ) ;
#54139=CARTESIAN_POINT ( 'NONE',  ( -3.152548672688508926E-16, -82.81249999863442213, -5.148502694627439702 ) ) ;
#54142=CARTESIAN_POINT ( 'NONE',  ( 1.975475456537005874E-15, -18.74999999999999645, 5.000000000000000000 ) ) ;
#54144=CARTESIAN_POINT ( 'NONE',  ( 5.000000000000000000, -22.41666666666666785, -2.886751345948129988 ) ) ;
#54150=CARTESIAN_POINT ( 'NONE',  ( 1.060575238724906964E-15, 20.37500000273119127, 5.773502691896257311 ) ) ;
#54159=CARTESIAN_POINT ( 'NONE',  ( -6.972266317189433020E-16, -79.24999999999998579, -5.000000000000000000 ) ) ;
#54160=CARTESIAN_POINT ( 'NONE',  ( -4.458734124999999437, -19.31249999863440081, 0.000000000000000000 ) ) ;
#54162=CARTESIAN_POINT ( 'NONE',  ( 5.000000000000000888, 0.4166666666666659080, 2.886751345948126879 ) ) ;
#54165=AXIS2_PLACEMENT_3D ( 'NONE', #39828, #1271, #60751 ) ;
#54167=ADVANCED_FACE ( 'NONE', ( #25830 ), #46716, .T. ) ;
#54170=LINE ( 'NONE', #30361, #29139 ) ;
#54173=EDGE_CURVE ( 'NONE', #41437, #11139, #32188, .T. ) ;
#54178=CARTESIAN_POINT ( 'NONE',  ( -1.339745962155613812, 10.79465819873852084, -5.000000000000000000 ) ) ;
#54183=EDGE_CURVE ( 'NONE', #29896, #143, #31277, .T. ) ;
#54185=CARTESIAN_POINT ( 'NONE',  ( 2.229367062500001939, 17.02083333469892779, 3.861377020970579999 ) ) ;
#54187=ORIENTED_EDGE ( 'NONE', *, *, #37550, .F. ) ;
#54190=CARTESIAN_POINT ( 'NONE',  ( 5.000000000000000000, 12.70833333606451809, -2.886751345948130876 ) ) ;
#54193=CARTESIAN_POINT ( 'NONE',  ( 4.458734124999998549, -65.72916666530106511, -2.574251347313721627 ) ) ;
#54195=CARTESIAN_POINT ( 'NONE',  ( 2.229367062499998831, 16.35416666803225993, -3.861377020970580887 ) ) ;
#54197=CARTESIAN_POINT ( 'NONE',  ( -3.152548672688508926E-16, -50.81249999863440792, -5.148502694627439702 ) ) ;
#54199=CARTESIAN_POINT ( 'NONE',  ( -4.999999999999999112, -11.79166666393547835, 2.886751345948131764 ) ) ;
#54201=DIRECTION ( 'NONE',  ( 0.000000000000000000, 0.000000000000000000, -1.000000000000000000 ) ) ;
#54203=CARTESIAN_POINT ( 'NONE',  ( -4.458734124999997661, -107.2291666653010651, 2.574251347313722516 ) ) ;
#54204=CARTESIAN_POINT ( 'NONE',  ( 2.229367062499998831, -13.89583333196774184, -3.861377020970580887 ) ) ;
#54205=ORIENTED_EDGE ( 'NONE', *, *, #17820, .F. ) ;
#54208=CARTESIAN_POINT ( 'NONE',  ( 2.229367062500001939, -98.97916666530105090, 3.861377020970579999 ) ) ;
#54210=CARTESIAN_POINT ( 'NONE',  ( 4.458734125000001214, -100.1458333319677365, 2.574251347313718519 ) ) ;
#54213=CARTESIAN_POINT ( 'NONE',  ( 1.060575238724906964E-15, -59.62499999726880873, 5.773502691896257311 ) ) ;
#54217=CARTESIAN_POINT ( 'NONE',  ( -4.458734124999999437, -17.31249999863440792, 0.000000000000000000 ) ) ;
#54218=CARTESIAN_POINT ( 'NONE',  ( -2.229367062500000163, 8.270833334698926009, -3.861377020970580443 ) ) ;
#54219=CARTESIAN_POINT ( 'NONE',  ( -2.229367062499996610, -61.39583333196774362, 3.861377020970582219 ) ) ;
#54224=CARTESIAN_POINT ( 'NONE',  ( -4.999999999999999112, -5.916666666666666963, 2.886751345948131764 ) ) ;
#54228=CARTESIAN_POINT ( 'NONE',  ( 2.500000000000002220, -66.66666666666667140, 4.330127018922192761 ) ) ;
#54229=CARTESIAN_POINT ( 'NONE',  ( -4.999999999999998224, -66.79166666393547303, 2.886751345948131764 ) ) ;
#54230=CARTESIAN_POINT ( 'NONE',  ( 9.457646018065525792E-16, -92.06249999863439371, 5.148502694627439702 ) ) ;
#54231=CARTESIAN_POINT ( 'NONE',  ( 9.457646018065525792E-16, 18.68750000136559208, 5.148502694627439702 ) ) ;
#54232=EDGE_CURVE ( 'NONE', #44900, #23690, #39124, .T. ) ;
#54237=CARTESIAN_POINT ( 'NONE',  ( -5.000000000000000000, -74.00000000000000000, 0.000000000000000000 ) ) ;
#54239=ORIENTED_EDGE ( 'NONE', *, *, #6119, .T. ) ;
#54240=CARTESIAN_POINT ( 'NONE',  ( 2.499999999999998668, -79.33333333333332860, -4.330127018922193649 ) ) ;
#54247=EDGE_LOOP ( 'NONE', ( #12255, #25616, #35252, #39368 ) ) ;
#54255=CARTESIAN_POINT ( 'NONE',  ( 2.229367062499998831, -59.89583333196774362, -3.861377020970580887 ) ) ;
#54258=CARTESIAN_POINT ( 'NONE',  ( -6.972266317189433020E-16, 3.875000002731185500, -5.000000000000000000 ) ) ;
#54266=CARTESIAN_POINT ( 'NONE',  ( 2.229367062500001939, -107.2291666653010651, 3.861377020970579999 ) ) ;
#54272=CARTESIAN_POINT ( 'NONE',  ( 4.458734125000000326, -45.89583333196774362, 2.574251347313718519 ) ) ;
#54276=CARTESIAN_POINT ( 'NONE',  ( 9.457646018065525792E-16, -13.06249999863440259, 5.148502694627439702 ) ) ;
#54277=CARTESIAN_POINT ( 'NONE',  ( -4.999999999999999112, -99.91666666666665719, 2.886751345948131764 ) ) ;
#54280=CARTESIAN_POINT ( 'NONE',  ( -4.458734124999998549, -33.47916666530107221, 2.574251347313722516 ) ) ;
#54281=CARTESIAN_POINT ( 'NONE',  ( -5.000000000000000000, 8.125000002731187720, 0.000000000000000000 ) ) ;
#54282=PLANE ( 'NONE',  #33524 ) ;
#54285=DIRECTION ( 'NONE',  ( 0.000000000000000000, 0.000000000000000000, 1.000000000000000000 ) ) ;
#54286=FACE_OUTER_BOUND ( 'NONE', #54568, .T. ) ;
#54288=CARTESIAN_POINT ( 'NONE',  ( -2.229367062499996610, 4.604166668032261711, 3.861377020970582219 ) ) ;
#54292=CARTESIAN_POINT ( 'NONE',  ( -5.000000000000000000, -98.08333333333332860, -2.886751345948128211 ) ) ;
#54293=CARTESIAN_POINT ( 'NONE',  ( -4.458734124999999437, -28.31249999863440081, 0.000000000000000000 ) ) ;
#54294=CARTESIAN_POINT ( 'NONE',  ( -4.999999999999998224, -22.79166666393548013, 2.886751345948131764 ) ) ;
#54295=CARTESIAN_POINT ( 'NONE',  ( 4.458734125000001214, -83.14583333196773651, 2.574251347313718519 ) ) ;
#54297=DIRECTION ( 'NONE',  ( -0.000000000000000000, 1.000000000000000000, -0.000000000000000000 ) ) ;
#54299=CARTESIAN_POINT ( 'NONE',  ( 2.229367062499998831, -3.645833331967739177, -3.861377020970580887 ) ) ;
#54300=CARTESIAN_POINT ( 'NONE',  ( 9.457646018065525792E-16, 20.68750000136559564, 5.148502694627439702 ) ) ;
#54301=CARTESIAN_POINT ( 'NONE',  ( -4.458734124999997661, -40.47916666530107221, 2.574251347313722516 ) ) ;
#54302=( BOUNDED_CURVE ( )  B_SPLINE_CURVE ( 2, ( #57848, #28242, #52695, #23113, #32763, #9255, #4429, #43038, #47856 ),
 .UNSPECIFIED., .F., .F. ) 
 B_SPLINE_CURVE_WITH_KNOTS ( ( 3, 2, 2, 2, 3 ),
 ( 0.3982142857142857428, 0.3988095238095238360, 0.4000000000000000222, 0.4011904761904762085, 0.4017857142857143016 ),
 .UNSPECIFIED. ) 
 CURVE ( )  GEOMETRIC_REPRESENTATION_ITEM ( )  RATIONAL_B_SPLINE_CURVE ( ( 0.9330127018922194093, 0.9330127018922225179, 1.000000000000000000, 0.8660254037844387076, 1.000000000000000000, 0.8660254037844387076, 1.000000000000000000, 0.9330127018922194093, 0.9330127018922194093 ) ) 
 REPRESENTATION_ITEM ( '' )  );
#54303=CARTESIAN_POINT ( 'NONE',  ( 5.000000000000000888, -15.58333333333332860, 2.886751345948126879 ) ) ;
#54307=VECTOR ( 'NONE', #46495, 1000.000000000000000 ) ;
#54308=CARTESIAN_POINT ( 'NONE',  ( -4.458734124999999437, -68.39583333196773651, -2.574251347313719407 ) ) ;
#54309=CARTESIAN_POINT ( 'NONE',  ( 5.000000000000000000, -105.2916666639354730, -2.886751345948129988 ) ) ;
#54310=VECTOR ( 'NONE', #60610, 1000.000000000000000 ) ;
#54312=EDGE_CURVE ( 'NONE', #28777, #27512, #14888, .T. ) ;
#54314=CARTESIAN_POINT ( 'NONE',  ( 1.975475456537005874E-15, -58.62499999726879452, 5.000000000000000000 ) ) ;
#54315=CARTESIAN_POINT ( 'NONE',  ( 9.457646018065525792E-16, -109.3124999986343937, 5.148502694627439702 ) ) ;
#54317=CARTESIAN_POINT ( 'NONE',  ( 5.000000000000000000, -59.41666666666665719, -2.886751345948129988 ) ) ;
#54319=CARTESIAN_POINT ( 'NONE',  ( 1.975475456537005874E-15, -21.75000000000000000, 5.000000000000000000 ) ) ;
#54322=CARTESIAN_POINT ( 'NONE',  ( -4.999999999999998224, -26.91666666666666430, 2.886751345948131764 ) ) ;
#54330=VECTOR ( 'NONE', #55192, 1000.000000000000000 ) ;
#54338=( BOUNDED_CURVE ( )  B_SPLINE_CURVE ( 2, ( #7660, #33352, #37546, #12783, #56865, #3150, #17296, #42679, #27889 ),
 .UNSPECIFIED., .F., .F. ) 
 B_SPLINE_CURVE_WITH_KNOTS ( ( 3, 2, 2, 2, 3 ),
 ( 0.7589285714285713969, 0.7595238095238094900, 0.7607142857142856762, 0.7619047619047618625, 0.7624999999999999556 ),
 .UNSPECIFIED. ) 
 CURVE ( )  GEOMETRIC_REPRESENTATION_ITEM ( )  RATIONAL_B_SPLINE_CURVE ( ( 0.9330127018922194093, 0.9330127018922194093, 1.000000000000000000, 0.8660254037844387076, 1.000000000000000000, 0.8660254037844387076, 1.000000000000000000, 0.9330127018922194093, 0.9330127018922194093 ) ) 
 REPRESENTATION_ITEM ( '' )  );
#54343=CARTESIAN_POINT ( 'NONE',  ( -2.229367062500000163, -39.72916666530107221, -3.861377020970580443 ) ) ;
#54348=CARTESIAN_POINT ( 'NONE',  ( 0.000000000000000000, -120.0000000000000000, 0.000000000000000000 ) ) ;
#54352=DIRECTION ( 'NONE',  ( -0.000000000000000000, 1.000000000000000000, -0.000000000000000000 ) ) ;
#54354=CARTESIAN_POINT ( 'NONE',  ( 2.229367062499998831, -89.89583333196773651, -3.861377020970580887 ) ) ;
#54363=VECTOR ( 'NONE', #63377, 1000.000000000000000 ) ;
#54364=ORIENTED_EDGE ( 'NONE', *, *, #46874, .F. ) ;
#54365=CARTESIAN_POINT ( 'NONE',  ( 4.458734124999999437, 5.187500001365596525, -5.460374474430324690E-16 ) ) ;
#54367=CARTESIAN_POINT ( 'NONE',  ( 4.458734125000001214, -19.14583333196774007, 2.574251347313718519 ) ) ;
#54372=CARTESIAN_POINT ( 'NONE',  ( -3.152548672688508926E-16, 20.18750000136559208, -5.148502694627439702 ) ) ;
#54374=CARTESIAN_POINT ( 'NONE',  ( 4.458734125000000326, -99.89583333196773651, 2.574251347313718519 ) ) ;
#54377=CARTESIAN_POINT ( 'NONE',  ( 2.229367062500001939, -13.97916666530107221, 3.861377020970579999 ) ) ;
#54379=CARTESIAN_POINT ( 'NONE',  ( 6.123233995736766282E-16, -120.0000000000000000, -5.000000000000000000 ) ) ;
#54381=CARTESIAN_POINT ( 'NONE',  ( -3.535250795749689387E-16, -39.12499999726880162, -5.773502691896257311 ) ) ;
#54382=CARTESIAN_POINT ( 'NONE',  ( -6.972266317189433020E-16, -67.12499999726881583, -5.000000000000000000 ) ) ;
#54383=CARTESIAN_POINT ( 'NONE',  ( 4.458734124999998549, 11.27083333469893134, -2.574251347313721627 ) ) ;
#54387=CARTESIAN_POINT ( 'NONE',  ( 9.457646018065525792E-16, -60.06249999863440792, 5.148502694627439702 ) ) ;
#54390=CARTESIAN_POINT ( 'NONE',  ( 5.000000000000000000, 6.499999999999999112, -6.123233995736766282E-16 ) ) ;
#54392=CARTESIAN_POINT ( 'NONE',  ( -6.972266317189433020E-16, -60.12499999726880873, -5.000000000000000000 ) ) ;
#54393=CARTESIAN_POINT ( 'NONE',  ( 4.458734124999998549, -52.72916666530107221, -2.574251347313721627 ) ) ;
#54394=CARTESIAN_POINT ( 'NONE',  ( -5.000000000000000000, -88.95833333060214443, -2.886751345948128211 ) ) ;
#54395=CARTESIAN_POINT ( 'NONE',  ( 4.458734124999998549, -31.72916666530107577, -2.574251347313721627 ) ) ;
#54397=CARTESIAN_POINT ( 'NONE',  ( 1.975475456537005874E-15, -8.750000000000000000, 5.000000000000000000 ) ) ;
#54399=CARTESIAN_POINT ( 'NONE',  ( 5.000000000000000888, -45.58333333333333570, 2.886751345948126879 ) ) ;
#54403=CARTESIAN_POINT ( 'NONE',  ( 4.458734124999999437, -102.8124999986344079, -5.460374474430324690E-16 ) ) ;
#54404=CARTESIAN_POINT ( 'NONE',  ( -4.458734124999999437, 4.437500001365595637, 0.000000000000000000 ) ) ;
#54407=AXIS2_PLACEMENT_3D ( 'NONE', #3388, #43227, #27496 ) ;
#54412=ORIENTED_EDGE ( 'NONE', *, *, #50683, .T. ) ;
#54413=CARTESIAN_POINT ( 'NONE',  ( 1.339745962155615144, -33.70534180126148271, 4.999999999999999112 ) ) ;
#54414=CARTESIAN_POINT ( 'NONE',  ( 5.000000000000000888, 19.41666666666666785, 2.886751345948126879 ) ) ;
#54418=ADVANCED_FACE ( 'NONE', ( #5181 ), #58885, .T. ) ;
#54420=CARTESIAN_POINT ( 'NONE',  ( -2.229367062499996610, -23.39583333196773651, 3.861377020970582219 ) ) ;
#54428=EDGE_CURVE ( 'NONE', #39986, #56905, #53968, .T. ) ;
#54431=ORIENTED_EDGE ( 'NONE', *, *, #11031, .T. ) ;
#54432=CARTESIAN_POINT ( 'NONE',  ( 2.229367062500001939, -72.22916666530107932, 3.861377020970579999 ) ) ;
#54434=SURFACE_STYLE_USAGE ( .BOTH. , #4275 ) ;
#54435=ORIENTED_EDGE ( 'NONE', *, *, #43018, .F. ) ;
#54439=CARTESIAN_POINT ( 'NONE',  ( -2.229367062500000163, -5.729166665301072214, -3.861377020970580443 ) ) ;
#54441=( BOUNDED_CURVE ( )  B_SPLINE_CURVE ( 2, ( #40487, #55625, #40174, #36310, #630, #39842, #25380, #30516, #41118 ),
 .UNSPECIFIED., .F., .F. ) 
 B_SPLINE_CURVE_WITH_KNOTS ( ( 3, 2, 2, 2, 3 ),
 ( 0.1267857142857142794, 0.1273809523809523725, 0.1285714285714285587, 0.1297619047619047727, 0.1303571428571428659 ),
 .UNSPECIFIED. ) 
 CURVE ( )  GEOMETRIC_REPRESENTATION_ITEM ( )  RATIONAL_B_SPLINE_CURVE ( ( 0.9330127018922194093, 0.9330127018922194093, 1.000000000000000000, 0.8660254037844387076, 1.000000000000000000, 0.8660254037844387076, 1.000000000000000000, 0.9330127018922194093, 0.9330127018922194093 ) ) 
 REPRESENTATION_ITEM ( '' )  );
#54446=CARTESIAN_POINT ( 'NONE',  ( 2.500000000000002220, -47.54166666393547303, 4.330127018922192761 ) ) ;
#54449=CARTESIAN_POINT ( 'NONE',  ( 4.458734124999998549, -79.72916666530106511, -2.574251347313721627 ) ) ;
#54451=CARTESIAN_POINT ( 'NONE',  ( -4.458734124999998549, 1.770833334698927786, 2.574251347313722516 ) ) ;
#54452=VECTOR ( 'NONE', #51806, 1000.000000000000000 ) ;
#54453=( BOUNDED_CURVE ( )  B_SPLINE_CURVE ( 2, ( #7673, #31458, #21513, #26647, #51416, #46267, #21830, #41740, #47221 ),
 .UNSPECIFIED., .F., .F. ) 
 B_SPLINE_CURVE_WITH_KNOTS ( ( 3, 2, 2, 2, 3 ),
 ( 0.1482142857142857151, 0.1488095238095238082, 0.1499999999999999944, 0.1511904761904761807, 0.1517857142857143016 ),
 .UNSPECIFIED. ) 
 CURVE ( )  GEOMETRIC_REPRESENTATION_ITEM ( )  RATIONAL_B_SPLINE_CURVE ( ( 0.9330127018922194093, 0.9330127018922194093, 1.000000000000000000, 0.8660254037844387076, 1.000000000000000000, 0.8660254037844387076, 1.000000000000000000, 0.9330127018922178550, 0.9330127018922194093 ) ) 
 REPRESENTATION_ITEM ( '' )  );
#54454=CARTESIAN_POINT ( 'NONE',  ( -5.000000000000000000, -87.08333333333331439, -2.886751345948128211 ) ) ;
#54456=CARTESIAN_POINT ( 'NONE',  ( -4.458734124999999437, -64.64583333196772230, -2.574251347313719407 ) ) ;
#54457=CARTESIAN_POINT ( 'NONE',  ( 5.000000000000000888, -24.45833333060214088, 2.886751345948126879 ) ) ;
#54459=CARTESIAN_POINT ( 'NONE',  ( 2.229367062499998831, 27.35416666803225993, -3.861377020970580887 ) ) ;
#54462=CARTESIAN_POINT ( 'NONE',  ( 2.229367062499998831, -48.64583333196772941, -3.861377020970580887 ) ) ;
#54463=CARTESIAN_POINT ( 'NONE',  ( -2.229367062499996610, -31.39583333196773651, 3.861377020970582219 ) ) ;
#54466=CARTESIAN_POINT ( 'NONE',  ( -2.499999999999996447, 20.16666666666666430, 4.330127018922195425 ) ) ;
#54468=DIRECTION ( 'NONE',  ( -0.000000000000000000, 1.000000000000000000, -0.000000000000000000 ) ) ;
#54469=CARTESIAN_POINT ( 'NONE',  ( -2.229367062500000163, -37.47916666530107221, -3.861377020970580443 ) ) ;
#54470=CARTESIAN_POINT ( 'NONE',  ( -2.500000000000000444, -74.04166666393547303, -4.330127018922193649 ) ) ;
#54473=CARTESIAN_POINT ( 'NONE',  ( 5.000000000000000000, -15.29166666393548191, -2.886751345948130876 ) ) ;
#54474=CARTESIAN_POINT ( 'NONE',  ( -2.229367062500000163, -82.72916666530106511, -3.861377020970580443 ) ) ;
#54477=DIRECTION ( 'NONE',  ( -0.000000000000000000, 1.000000000000000000, -0.000000000000000000 ) ) ;
#54478=CARTESIAN_POINT ( 'NONE',  ( 2.500000000000002220, -25.66666666666666430, 4.330127018922192761 ) ) ;
#54484=CARTESIAN_POINT ( 'NONE',  ( 5.000000000000000000, 19.70833333606451987, -2.886751345948129988 ) ) ;
#54495=CARTESIAN_POINT ( 'NONE',  ( -2.499999999999996447, -78.83333333333332860, 4.330127018922195425 ) ) ;
#54496=CARTESIAN_POINT ( 'NONE',  ( 2.229367062499998831, -20.64583333196774007, -3.861377020970580887 ) ) ;
#54502=ORIENTED_EDGE ( 'NONE', *, *, #59861, .F. ) ;
#54507=CARTESIAN_POINT ( 'NONE',  ( 1.975475456537005874E-15, -2.750000000000000888, 5.000000000000000000 ) ) ;
#54510=( BOUNDED_CURVE ( )  B_SPLINE_CURVE ( 2, ( #19320, #14178, #28967, #33805, #9355, #4531, #38936, #14491, #49547 ),
 .UNSPECIFIED., .F., .F. ) 
 B_SPLINE_CURVE_WITH_KNOTS ( ( 3, 2, 2, 2, 3 ),
 ( 0.1196428571428571480, 0.1202380952380952411, 0.1214285714285714274, 0.1226190476190476136, 0.1232142857142857206 ),
 .UNSPECIFIED. ) 
 CURVE ( )  GEOMETRIC_REPRESENTATION_ITEM ( )  RATIONAL_B_SPLINE_CURVE ( ( 0.9330127018922192983, 0.9330127018922200755, 1.000000000000000000, 0.8660254037844387076, 1.000000000000000000, 0.8660254037844387076, 1.000000000000000000, 0.9330127018922185211, 0.9330127018922192983 ) ) 
 REPRESENTATION_ITEM ( '' )  );
#54517=CARTESIAN_POINT ( 'NONE',  ( -3.152548672688508926E-16, 13.43750000136559386, -5.148502694627439702 ) ) ;
#54520=CARTESIAN_POINT ( 'NONE',  ( 2.499999999999998668, -44.33333333333333570, -4.330127018922193649 ) ) ;
#54522=CARTESIAN_POINT ( 'NONE',  ( -6.972266317189433020E-16, -15.25000000000000000, -5.000000000000000000 ) ) ;
#54523=CARTESIAN_POINT ( 'NONE',  ( 4.458734124999999437, -63.81249999863440792, -5.460374474430324690E-16 ) ) ;
#54525=CARTESIAN_POINT ( 'NONE',  ( 2.229367062499998831, 17.35416666803225993, -3.861377020970580887 ) ) ;
#54526=EDGE_CURVE ( 'NONE', #11325, #43978, #21499, .T. ) ;
#54528=CARTESIAN_POINT ( 'NONE',  ( -4.458734124999998549, -50.47916666530107221, 2.574251347313722516 ) ) ;
#54529=CARTESIAN_POINT ( 'NONE',  ( 5.000000000000000000, -7.291666663935481907, -2.886751345948129988 ) ) ;
#54530=CARTESIAN_POINT ( 'NONE',  ( -5.000000000000000000, -109.0833333333333428, -2.886751345948128211 ) ) ;
#54534=( BOUNDED_CURVE ( )  B_SPLINE_CURVE ( 2, ( #835, #16252, #35872, #11415, #35551, #30720, #50343, #15613, #54850 ),
 .UNSPECIFIED., .F., .F. ) 
 B_SPLINE_CURVE_WITH_KNOTS ( ( 3, 2, 2, 2, 3 ),
 ( 0.9517857142857142350, 0.9523809523809523281, 0.9535714285714286254, 0.9547619047619048116, 0.9553571428571429047 ),
 .UNSPECIFIED. ) 
 CURVE ( )  GEOMETRIC_REPRESENTATION_ITEM ( )  RATIONAL_B_SPLINE_CURVE ( ( 0.9330127018922194093, 0.9330127018922194093, 1.000000000000000000, 0.8660254037844387076, 1.000000000000000000, 0.8660254037844387076, 1.000000000000000000, 0.9330127018922194093, 0.9330127018922194093 ) ) 
 REPRESENTATION_ITEM ( '' )  );
#54535=CARTESIAN_POINT ( 'NONE',  ( -2.229367062500000163, -15.72916666530107399, -3.861377020970580443 ) ) ;
#54537=CARTESIAN_POINT ( 'NONE',  ( 4.458734124999999437, -104.8124999986344079, -5.460374474430324690E-16 ) ) ;
#54540=CARTESIAN_POINT ( 'NONE',  ( -4.458734124999999437, -96.56249999863440792, 0.000000000000000000 ) ) ;
#54542=CARTESIAN_POINT ( 'NONE',  ( 2.500000000000002220, -58.54166666393548013, 4.330127018922192761 ) ) ;
#54545=CARTESIAN_POINT ( 'NONE',  ( -4.458734124999999437, -18.39583333196774007, -2.574251347313719407 ) ) ;
#54546=CARTESIAN_POINT ( 'NONE',  ( -3.152548672688508926E-16, 7.187500001365594748, -5.148502694627439702 ) ) ;
#54547=CARTESIAN_POINT ( 'NONE',  ( -2.229367062499996610, -63.39583333196774362, 3.861377020970582219 ) ) ;
#54552=CARTESIAN_POINT ( 'NONE',  ( 2.500000000000002220, -9.666666666666664298, 4.330127018922192761 ) ) ;
#54554=VERTEX_POINT ( 'NONE', #60181 ) ;
#54557=CARTESIAN_POINT ( 'NONE',  ( -5.000000000000000000, -91.87499999726880162, 0.000000000000000000 ) ) ;
#54559=CARTESIAN_POINT ( 'NONE',  ( 4.458734124999999437, -90.81249999863440792, -5.460374474430324690E-16 ) ) ;
#54560=CARTESIAN_POINT ( 'NONE',  ( -4.458734124999998549, 15.52083333469892779, 2.574251347313722516 ) ) ;
#54562=CARTESIAN_POINT ( 'NONE',  ( 5.000000000000000888, -82.58333333333334281, 2.886751345948126879 ) ) ;
#54563=DIRECTION ( 'NONE',  ( 0.000000000000000000, 0.000000000000000000, 1.000000000000000000 ) ) ;
#54566=CARTESIAN_POINT ( 'NONE',  ( 5.000000000000000000, -74.41666666666665719, -2.886751345948129988 ) ) ;
#54568=EDGE_LOOP ( 'NONE', ( #47292, #16436, #6111, #50569, #29010, #25486, #18646, #51214 ) ) ;
#54569=CARTESIAN_POINT ( 'NONE',  ( 5.000000000000000000, -80.37499999726881583, -6.123233995736766282E-16 ) ) ;
#54571=DIRECTION ( 'NONE',  ( -0.000000000000000000, 1.000000000000000000, -0.000000000000000000 ) ) ;
#54580=CARTESIAN_POINT ( 'NONE',  ( 4.458734124999999437, -65.06249999863440792, -5.460374474430324690E-16 ) ) ;
#54583=VERTEX_POINT ( 'NONE', #16742 ) ;
#54588=VERTEX_POINT ( 'NONE', #1018 ) ;
#54591=CARTESIAN_POINT ( 'NONE',  ( 4.458734124999998549, -109.9791666653010793, -2.574251347313721627 ) ) ;
#54592=CARTESIAN_POINT ( 'NONE',  ( 5.000000000000000888, 20.41666666666666785, 2.886751345948126879 ) ) ;
#54597=CARTESIAN_POINT ( 'NONE',  ( 9.457646018065525792E-16, -43.06249999863440081, 5.148502694627439702 ) ) ;
#54600=CARTESIAN_POINT ( 'NONE',  ( 4.458734124999998549, -49.72916666530107221, -2.574251347313721627 ) ) ;
#54601=EDGE_CURVE ( 'NONE', #45912, #52441, #34615, .T. ) ;
#54602=CARTESIAN_POINT ( 'NONE',  ( -2.229367062500000163, -12.47916666530107044, -3.861377020970580443 ) ) ;
#54603=CARTESIAN_POINT ( 'NONE',  ( -2.500000000000000444, -102.1666666666666572, -4.330127018922193649 ) ) ;
#54605=CARTESIAN_POINT ( 'NONE',  ( 9.457646018065525792E-16, -32.31249999863440792, 5.148502694627439702 ) ) ;
#54606=CARTESIAN_POINT ( 'NONE',  ( -5.000000000000000000, 4.125000002731186832, 0.000000000000000000 ) ) ;
#54607=CARTESIAN_POINT ( 'NONE',  ( -2.500000000000000444, -7.041666663935481907, -4.330127018922193649 ) ) ;
#54610=DIRECTION ( 'NONE',  ( -0.000000000000000000, 1.000000000000000000, -0.000000000000000000 ) ) ;
#54612=DIRECTION ( 'NONE',  ( -0.000000000000000000, 1.000000000000000000, -0.000000000000000000 ) ) ;
#54613=CARTESIAN_POINT ( 'NONE',  ( -2.229367062499996610, -1.395833331967737179, 3.861377020970582219 ) ) ;
#54615=CARTESIAN_POINT ( 'NONE',  ( 5.000000000000000000, 24.70833333606452342, -2.886751345948130876 ) ) ;
#54616=CARTESIAN_POINT ( 'NONE',  ( -2.500000000000000444, -76.16666666666665719, -4.330127018922193649 ) ) ;
#54617=CARTESIAN_POINT ( 'NONE',  ( -4.458734124999999437, -85.31249999863439371, 0.000000000000000000 ) ) ;
#54618=CARTESIAN_POINT ( 'NONE',  ( -2.229367062499996610, -33.14583333196772941, 3.861377020970582219 ) ) ;
#54620=CARTESIAN_POINT ( 'NONE',  ( 2.493747252781420335E-13, -77.25000000000001421, -5.000000000000000000 ) ) ;
#54621=CARTESIAN_POINT ( 'NONE',  ( -2.229367062500000163, -83.72916666530106511, -3.861377020970580443 ) ) ;
#54623=CARTESIAN_POINT ( 'NONE',  ( 0.000000000000000000, -120.0000000000000000, 0.000000000000000000 ) ) ;
#54625=CARTESIAN_POINT ( 'NONE',  ( -4.458734124999999437, -1.395833331967737179, -2.574251347313719407 ) ) ;
#54626=CARTESIAN_POINT ( 'NONE',  ( -4.458734124999999437, 20.35416666803225993, -2.574251347313719407 ) ) ;
#54628=CARTESIAN_POINT ( 'NONE',  ( 9.457646018065525792E-16, -48.31249999863440792, 5.148502694627439702 ) ) ;
#54629=CARTESIAN_POINT ( 'NONE',  ( -2.499999999999996447, -45.70833333060214443, 4.330127018922195425 ) ) ;
#54633=CARTESIAN_POINT ( 'NONE',  ( 2.229367062500001939, -74.97916666530106511, 3.861377020970579999 ) ) ;
#54634=CARTESIAN_POINT ( 'NONE',  ( 5.000000000000000888, -104.4583333306021302, 2.886751345948126879 ) ) ;
#54637=CARTESIAN_POINT ( 'NONE',  ( 2.500000000000002220, -58.54166666393548013, 4.330127018922192761 ) ) ;
#54640=CARTESIAN_POINT ( 'NONE',  ( 5.000000000000000888, -61.58333333333334281, 2.886751345948126879 ) ) ;
#54641=CARTESIAN_POINT ( 'NONE',  ( -4.999999999999998224, -31.79166666393548724, 2.886751345948131764 ) ) ;
#54643=ORIENTED_EDGE ( 'NONE', *, *, #43360, .F. ) ;
#54644=DIRECTION ( 'NONE',  ( 0.000000000000000000, 0.000000000000000000, 1.000000000000000000 ) ) ;
#54652=ORIENTED_EDGE ( 'NONE', *, *, #7863, .T. ) ;
#54653=CARTESIAN_POINT ( 'NONE',  ( -5.000000000000000000, -75.95833333060214443, -2.886751345948128211 ) ) ;
#54660=CARTESIAN_POINT ( 'NONE',  ( -3.152548672688508926E-16, -46.81249999863440081, -5.148502694627439702 ) ) ;
#54669=CARTESIAN_POINT ( 'NONE',  ( -4.458734124999998549, -89.47916666530106511, 2.574251347313722516 ) ) ;
#54671=ORIENTED_EDGE ( 'NONE', *, *, #43417, .T. ) ;
#54672=LINE ( 'NONE', #14, #31353 ) ;
#54677=CARTESIAN_POINT ( 'NONE',  ( 2.229367062500001939, 5.020833334698926897, 3.861377020970579999 ) ) ;
#54678=EDGE_CURVE ( 'NONE', #3563, #37393, #60498, .T. ) ;
#54680=CARTESIAN_POINT ( 'NONE',  ( 2.499999999999998668, -106.3333333333333286, -4.330127018922193649 ) ) ;
#54681=CARTESIAN_POINT ( 'NONE',  ( -3.152548672688508926E-16, -16.81249999863440436, -5.148502694627439702 ) ) ;
#54689=CARTESIAN_POINT ( 'NONE',  ( 4.458734125000000326, 14.85416666803225993, 2.574251347313718519 ) ) ;
#54690=ORIENTED_EDGE ( 'NONE', *, *, #49168, .F. ) ;
#54691=CARTESIAN_POINT ( 'NONE',  ( 4.458734124999998549, -94.72916666530106511, -2.574251347313721627 ) ) ;
#54692=CARTESIAN_POINT ( 'NONE',  ( -5.000000000000000000, -18.95833333060214798, -2.886751345948128211 ) ) ;
#54693=CARTESIAN_POINT ( 'NONE',  ( 5.000000000000000000, -71.37499999726880162, -6.123233995736766282E-16 ) ) ;
#54694=CARTESIAN_POINT ( 'NONE',  ( -4.458734124999998549, -17.22916666530106866, 2.574251347313722516 ) ) ;
#54696=EDGE_CURVE ( 'NONE', #48706, #20975, #29722, .T. ) ;
#54697=CARTESIAN_POINT ( 'NONE',  ( 2.499999999999998668, -3.333333333333333925, -4.330127018922193649 ) ) ;
#54699=CARTESIAN_POINT ( 'NONE',  ( -5.000000000000000000, -43.95833333060214443, -2.886751345948128211 ) ) ;
#54700=CARTESIAN_POINT ( 'NONE',  ( 6.123233995736766282E-16, -120.0000000000000000, -5.000000000000000000 ) ) ;
#54701=CARTESIAN_POINT ( 'NONE',  ( -3.152548672688508926E-16, 12.43750000136559208, -5.148502694627439702 ) ) ;
#54702=CARTESIAN_POINT ( 'NONE',  ( -4.458734124999999437, -110.5624999986343937, 0.000000000000000000 ) ) ;
#54706=CARTESIAN_POINT ( 'NONE',  ( 4.458734125000001214, -61.89583333196773651, 2.574251347313718519 ) ) ;
#54707=EDGE_LOOP ( 'NONE', ( #51595, #2173, #34806, #62316 ) ) ;
#54709=CARTESIAN_POINT ( 'NONE',  ( -5.000000000000000000, 4.000000000000000000, 0.000000000000000000 ) ) ;
#54713=CARTESIAN_POINT ( 'NONE',  ( -2.229367062500000163, -59.47916666530106511, -3.861377020970580443 ) ) ;
#54714=CARTESIAN_POINT ( 'NONE',  ( -3.535250795749689387E-16, -90.12499999726881583, -5.773502691896257311 ) ) ;
#54715=CARTESIAN_POINT ( 'NONE',  ( 4.458734124999999437, -31.81249999863440436, -5.460374474430324690E-16 ) ) ;
#54716=CYLINDRICAL_SURFACE ( 'NONE', #41128, 5.000000000000000000 ) ;
#54721=CARTESIAN_POINT ( 'NONE',  ( 2.499999999999998668, -41.33333333333333570, -4.330127018922193649 ) ) ;
#54723=CARTESIAN_POINT ( 'NONE',  ( 1.975475456537005874E-15, -6.624999997268813168, 5.000000000000000000 ) ) ;
#54724=VERTEX_POINT ( 'NONE', #37003 ) ;
#54725=CARTESIAN_POINT ( 'NONE',  ( 2.229367062500001939, -99.97916666530106511, 3.861377020970579999 ) ) ;
#54726=CARTESIAN_POINT ( 'NONE',  ( -2.229367062499996610, 0.6041666680322611560, 3.861377020970582219 ) ) ;
#54734=CARTESIAN_POINT ( 'NONE',  ( 2.499999999999998668, -33.33333333333332860, -4.330127018922193649 ) ) ;
#54735=CARTESIAN_POINT ( 'NONE',  ( -2.500000000000000444, -17.04166666393548368, -4.330127018922193649 ) ) ;
#54737=CARTESIAN_POINT ( 'NONE',  ( -1.339745962155497683, -56.08034179853028434, -5.000000000000066613 ) ) ;
#54739=FACE_OUTER_BOUND ( 'NONE', #15166, .T. ) ;
#54740=CARTESIAN_POINT ( 'NONE',  ( -2.229367062500000163, -29.72916666530107221, -3.861377020970580443 ) ) ;
#54751=CARTESIAN_POINT ( 'NONE',  ( -4.458734124999999437, -74.64583333196773651, -2.574251347313719407 ) ) ;
#54752=LINE ( 'NONE', #15829, #34847 ) ;
#54753=VERTEX_POINT ( 'NONE', #7419 ) ;
#54755=DIRECTION ( 'NONE',  ( 0.000000000000000000, 0.000000000000000000, 1.000000000000000000 ) ) ;
#54757=CARTESIAN_POINT ( 'NONE',  ( 4.458734124999998549, -1.979166665301068662, -2.574251347313721627 ) ) ;
#54761=CARTESIAN_POINT ( 'NONE',  ( -2.499999999999996447, -44.83333333333333570, 4.330127018922195425 ) ) ;
#54767=CARTESIAN_POINT ( 'NONE',  ( -2.229367062500000163, -79.47916666530106511, -3.861377020970580443 ) ) ;
#54768=CARTESIAN_POINT ( 'NONE',  ( -6.972266317189433020E-16, -90.12499999726880162, -5.000000000000000000 ) ) ;
#54769=CARTESIAN_POINT ( 'NONE',  ( 4.458734124999998549, 0.2708333346989263979, -2.574251347313721627 ) ) ;
#54772=CARTESIAN_POINT ( 'NONE',  ( -2.229367062500000163, -66.72916666530106511, -3.861377020970580443 ) ) ;
#54773=CARTESIAN_POINT ( 'NONE',  ( -5.000000000000000000, -26.87499999726881583, 0.000000000000000000 ) ) ;
#54775=CARTESIAN_POINT ( 'NONE',  ( -4.458734124999999437, 29.60416666803225993, -2.574251347313719407 ) ) ;
#54776=CARTESIAN_POINT ( 'NONE',  ( 1.339745962155615144, -110.5803417985302985, 4.999999999999999112 ) ) ;
#54777=CARTESIAN_POINT ( 'NONE',  ( 1.339745962155615144, -3.580341798530293662, 4.999999999999999112 ) ) ;
#54779=CARTESIAN_POINT ( 'NONE',  ( -2.229367062500000163, -47.47916666530106511, -3.861377020970580443 ) ) ;
#54780=CARTESIAN_POINT ( 'NONE',  ( -2.229367062500000163, -34.72916666530107221, -3.861377020970580443 ) ) ;
#54783=CARTESIAN_POINT ( 'NONE',  ( -5.000000000000000000, 19.00000000000000000, 0.000000000000000000 ) ) ;
#54786=LINE ( 'NONE', #44479, #61356 ) ;
#54787=CARTESIAN_POINT ( 'NONE',  ( 4.458734125000001214, -37.89583333196772941, 2.574251347313718519 ) ) ;
#54788=CARTESIAN_POINT ( 'NONE',  ( 5.000000000000000888, -73.45833333060214443, 2.886751345948126879 ) ) ;
#54791=CARTESIAN_POINT ( 'NONE',  ( 5.000000000000000888, -24.45833333060214798, 2.886751345948126879 ) ) ;
#54793=CARTESIAN_POINT ( 'NONE',  ( 1.339745962155612702, -37.29465819873852439, -5.000000000000000000 ) ) ;
#54794=CARTESIAN_POINT ( 'NONE',  ( -4.458734124999999437, -81.56249999863440792, 0.000000000000000000 ) ) ;
#54798=CARTESIAN_POINT ( 'NONE',  ( -5.000000000000000000, -26.99999999999999645, 0.000000000000000000 ) ) ;
#54802=ORIENTED_EDGE ( 'NONE', *, *, #30666, .T. ) ;
#54804=CARTESIAN_POINT ( 'NONE',  ( -4.999999999999999112, 19.20833333606451632, 2.886751345948131764 ) ) ;
#54810=CARTESIAN_POINT ( 'NONE',  ( -6.972266317189433020E-16, -0.2500000000000001665, -5.000000000000000000 ) ) ;
#54812=CARTESIAN_POINT ( 'NONE',  ( 1.975475456537005874E-15, -40.74999999999999289, 5.000000000000000000 ) ) ;
#54813=CARTESIAN_POINT ( 'NONE',  ( 9.457646018065525792E-16, -24.06249999863440436, 5.148502694627439702 ) ) ;
#54817=( BOUNDED_CURVE ( )  B_SPLINE_CURVE ( 2, ( #14771, #48868, #45328, #34719, #20894, #4814, #5135, #49196, #44038 ),
 .UNSPECIFIED., .F., .F. ) 
 B_SPLINE_CURVE_WITH_KNOTS ( ( 3, 2, 2, 2, 3 ),
 ( 0.6125000000000000444, 0.6130952380952381375, 0.6142857142857143238, 0.6154761904761905100, 0.6160714285714286031 ),
 .UNSPECIFIED. ) 
 CURVE ( )  GEOMETRIC_REPRESENTATION_ITEM ( )  RATIONAL_B_SPLINE_CURVE ( ( 0.9330127018922194093, 0.9330127018922194093, 1.000000000000000000, 0.8660254037844387076, 1.000000000000000000, 0.8660254037844387076, 1.000000000000000000, 0.9330127018922194093, 0.9330127018922194093 ) ) 
 REPRESENTATION_ITEM ( '' )  );
#54822=ORIENTED_EDGE ( 'NONE', *, *, #27890, .F. ) ;
#54824=CARTESIAN_POINT ( 'NONE',  ( -2.500000000000000444, -3.166666666666664742, -4.330127018922193649 ) ) ;
#54835=CARTESIAN_POINT ( 'NONE',  ( -2.229367062499996610, 14.85416666803226171, 3.861377020970582219 ) ) ;
#54838=FACE_OUTER_BOUND ( 'NONE', #17234, .T. ) ;
#54841=CARTESIAN_POINT ( 'NONE',  ( 4.458734125000000326, -65.89583333196773651, 2.574251347313718519 ) ) ;
#54842=LINE ( 'NONE', #29411, #4769 ) ;
#54843=CARTESIAN_POINT ( 'NONE',  ( -4.458734124999998549, 19.77083333469892779, 2.574251347313722516 ) ) ;
#54846=CARTESIAN_POINT ( 'NONE',  ( 2.229367062500001939, -51.22916666530107221, 3.861377020970579999 ) ) ;
#54847=CARTESIAN_POINT ( 'NONE',  ( -2.499999999999996447, -10.70833333060214621, 4.330127018922195425 ) ) ;
#54850=CARTESIAN_POINT ( 'NONE',  ( 1.975475456537005874E-15, -104.6249999972688016, 5.000000000000000000 ) ) ;
#54851=CARTESIAN_POINT ( 'NONE',  ( 9.457646018065525792E-16, -15.31249999863440436, 5.148502694627439702 ) ) ;
#54854=CARTESIAN_POINT ( 'NONE',  ( -4.458734124999999437, -103.3124999986344079, 0.000000000000000000 ) ) ;
#54857=CARTESIAN_POINT ( 'NONE',  ( 4.458734124999999437, -99.06249999863440792, -5.460374474430324690E-16 ) ) ;
#54858=DIRECTION ( 'NONE',  ( -0.000000000000000000, 1.000000000000000000, -0.000000000000000000 ) ) ;
#54859=CARTESIAN_POINT ( 'NONE',  ( -2.499999999999996447, -55.70833333060214443, 4.330127018922195425 ) ) ;
#54860=CARTESIAN_POINT ( 'NONE',  ( 0.000000000000000000, -120.0000000000000000, 0.000000000000000000 ) ) ;
#54863=CARTESIAN_POINT ( 'NONE',  ( -2.229367062499996610, -23.14583333196773651, 3.861377020970582219 ) ) ;
#54864=CARTESIAN_POINT ( 'NONE',  ( 9.457646018065525792E-16, 5.687500001365592972, 5.148502694627439702 ) ) ;
#54865=CARTESIAN_POINT ( 'NONE',  ( 9.457646018065525792E-16, -66.31249999863440792, 5.148502694627439702 ) ) ;
#54866=CARTESIAN_POINT ( 'NONE',  ( 1.339745962155615144, -94.58034179853028434, 4.999999999999999112 ) ) ;
#54868=CARTESIAN_POINT ( 'NONE',  ( 1.975475456537005874E-15, -32.74999999999999289, 5.000000000000000000 ) ) ;
#54870=CARTESIAN_POINT ( 'NONE',  ( 5.000000000000000888, -10.58333333333333393, 2.886751345948126879 ) ) ;
#54872=ORIENTED_EDGE ( 'NONE', *, *, #35751, .T. ) ;
#54874=CARTESIAN_POINT ( 'NONE',  ( 5.000000000000000888, 21.54166666939785202, 2.886751345948126879 ) ) ;
#54875=CARTESIAN_POINT ( 'NONE',  ( -6.972266317189433020E-16, -38.12499999726880873, -5.000000000000000000 ) ) ;
#54877=AXIS2_PLACEMENT_3D ( 'NONE', #28256, #18916, #53335 ) ;
#54879=CARTESIAN_POINT ( 'NONE',  ( 5.000000000000000000, -82.41666666666667140, -2.886751345948130876 ) ) ;
#54880=DIRECTION ( 'NONE',  ( 0.000000000000000000, 0.000000000000000000, 1.000000000000000000 ) ) ;
#54883=CARTESIAN_POINT ( 'NONE',  ( -2.500000000000000444, -77.16666666666665719, -4.330127018922193649 ) ) ;
#54885=VERTEX_POINT ( 'NONE', #7734 ) ;
#54887=EDGE_LOOP ( 'NONE', ( #25278, #60314, #35237, #40045 ) ) ;
#54898=CARTESIAN_POINT ( 'NONE',  ( 2.229367062500001939, -63.22916666530106511, 3.861377020970579999 ) ) ;
#54905=VERTEX_POINT ( 'NONE', #17994 ) ;
#54908=CARTESIAN_POINT ( 'NONE',  ( -4.458734124999998549, 27.77083333469892423, 2.574251347313722516 ) ) ;
#54910=ORIENTED_EDGE ( 'NONE', *, *, #18261, .F. ) ;
#54914=CARTESIAN_POINT ( 'NONE',  ( 2.229367062499998831, -45.64583333196774362, -3.861377020970580887 ) ) ;
#54918=CARTESIAN_POINT ( 'NONE',  ( 2.229367062499998831, -49.64583333196772941, -3.861377020970580887 ) ) ;
#54919=CARTESIAN_POINT ( 'NONE',  ( -1.339745962155610925, -70.79465819873850307, 5.000000000000000000 ) ) ;
#54920=CARTESIAN_POINT ( 'NONE',  ( 4.458734124999998549, -17.72916666530106866, -2.574251347313721627 ) ) ;
#54921=CARTESIAN_POINT ( 'NONE',  ( -3.535250795749689387E-16, -103.2500000000000000, -5.773502691896257311 ) ) ;
#54924=CARTESIAN_POINT ( 'NONE',  ( 9.457646018065525792E-16, -33.31249999863440792, 5.148502694627439702 ) ) ;
#54925=CARTESIAN_POINT ( 'NONE',  ( -4.999999999999999112, 5.208333336064518981, 2.886751345948131764 ) ) ;
#54930=CARTESIAN_POINT ( 'NONE',  ( -4.999999999999998224, -44.79166666393547303, 2.886751345948131764 ) ) ;
#54932=CARTESIAN_POINT ( 'NONE',  ( 4.458734125000000326, -0.1458333319677394824, 2.574251347313718519 ) ) ;
#54933=ORIENTED_EDGE ( 'NONE', *, *, #4895, .T. ) ;
#54936=CARTESIAN_POINT ( 'NONE',  ( 2.229367062500001939, -87.97916666530107932, 3.861377020970579999 ) ) ;
#54937=CARTESIAN_POINT ( 'NONE',  ( -2.229367062500000163, -35.47916666530107221, -3.861377020970580443 ) ) ;
#54938=FACE_OUTER_BOUND ( 'NONE', #35328, .T. ) ;
#54939=CARTESIAN_POINT ( 'NONE',  ( -4.458734124999999437, -82.64583333196772230, -2.574251347313719407 ) ) ;
#54941=CYLINDRICAL_SURFACE ( 'NONE', #21223, 5.000000000000000000 ) ;
#54943=CARTESIAN_POINT ( 'NONE',  ( 9.457646018065525792E-16, -3.062499998634407472, 5.148502694627439702 ) ) ;
#54944=CARTESIAN_POINT ( 'NONE',  ( 2.229367062499998831, 20.10416666803225993, -3.861377020970580887 ) ) ;
#54945=CARTESIAN_POINT ( 'NONE',  ( -4.458734124999997661, -47.47916666530106511, 2.574251347313722516 ) ) ;
#54946=CARTESIAN_POINT ( 'NONE',  ( 5.000000000000000888, -105.5833333333333286, 2.886751345948126879 ) ) ;
#54951=CARTESIAN_POINT ( 'NONE',  ( -4.458734124999999437, -72.39583333196775072, -2.574251347313719407 ) ) ;
#54952=CARTESIAN_POINT ( 'NONE',  ( -5.000000000000000000, -110.8749999972688016, 0.000000000000000000 ) ) ;
#54954=CARTESIAN_POINT ( 'NONE',  ( 6.123233995736766282E-16, -120.0000000000000000, -5.000000000000000000 ) ) ;
#54957=CARTESIAN_POINT ( 'NONE',  ( -5.000000000000000000, -61.00000000000000000, 0.000000000000000000 ) ) ;
#54958=CARTESIAN_POINT ( 'NONE',  ( 5.000000000000000000, -90.29166666393547303, -2.886751345948130876 ) ) ;
#54960=ORIENTED_EDGE ( 'NONE', *, *, #1208, .T. ) ;
#54961=CARTESIAN_POINT ( 'NONE',  ( 4.648177544792955347E-16, 28.87500000273118417, -5.000000000000000000 ) ) ;
#54962=CARTESIAN_POINT ( 'NONE',  ( -1.339745962155613812, -99.20534180126146850, -5.000000000000000000 ) ) ;
#54968=AXIS2_PLACEMENT_3D ( 'NONE', #44930, #19525, #34006 ) ;
#54971=ORIENTED_EDGE ( 'NONE', *, *, #12667, .T. ) ;
#54972=CARTESIAN_POINT ( 'NONE',  ( 3.253724281355068545E-15, 27.87500000273118417, -5.000000000000000000 ) ) ;
#54974=EDGE_LOOP ( 'NONE', ( #34441, #12383, #38073, #41923 ) ) ;
#54978=CARTESIAN_POINT ( 'NONE',  ( 4.458734124999999437, -44.06249999863440081, -5.460374474430324690E-16 ) ) ;
#54979=CARTESIAN_POINT ( 'NONE',  ( 1.339745962155612702, -68.16965819600733312, -5.000000000000000000 ) ) ;
#54981=CARTESIAN_POINT ( 'NONE',  ( 1.975475456537005874E-15, -81.62499999726881583, 5.000000000000000000 ) ) ;
#54986=CARTESIAN_POINT ( 'NONE',  ( -6.972266317189433020E-16, -24.12499999726881228, -5.000000000000000000 ) ) ;
#54988=ADVANCED_FACE ( 'NONE', ( #6352 ), #56511, .T. ) ;
#54989=CARTESIAN_POINT ( 'NONE',  ( -4.458734124999999437, -93.64583333196773651, -2.574251347313719407 ) ) ;
#54990=CARTESIAN_POINT ( 'NONE',  ( 1.975475456537005874E-15, -106.7499999999999858, 5.000000000000000000 ) ) ;
#54995=CARTESIAN_POINT ( 'NONE',  ( -5.926426369611017623E-15, 27.24999999999999645, 5.000000000000000000 ) ) ;
#54997=EDGE_CURVE ( 'NONE', #20011, #44517, #11785, .T. ) ;
#54998=CARTESIAN_POINT ( 'NONE',  ( 2.229367062499998831, -3.645833331967739177, -3.861377020970580887 ) ) ;
#54999=CARTESIAN_POINT ( 'NONE',  ( 1.975475456537005874E-15, 6.249999999999998224, 5.000000000000000000 ) ) ;
#55000=CARTESIAN_POINT ( 'NONE',  ( -4.458734124999999437, -19.64583333196774362, -2.574251347313719407 ) ) ;
#55002=CARTESIAN_POINT ( 'NONE',  ( 1.975475456537005874E-15, 4.375000002731185056, 5.000000000000000000 ) ) ;
#55004=CARTESIAN_POINT ( 'NONE',  ( -4.458734124999999437, 13.43750000136559386, 0.000000000000000000 ) ) ;
#55007=CARTESIAN_POINT ( 'NONE',  ( -2.499999999999996447, -20.83333333333333570, 4.330127018922195425 ) ) ;
#55008=CARTESIAN_POINT ( 'NONE',  ( 4.458734124999998549, -18.72916666530106866, -2.574251347313721627 ) ) ;
#55010=CARTESIAN_POINT ( 'NONE',  ( 5.000000000000000000, -3.500000000000003109, -6.123233995736766282E-16 ) ) ;
#55012=( BOUNDED_CURVE ( )  B_SPLINE_CURVE ( 2, ( #60475, #6120, #54680, #36018, #29900, #20267, #10603, #50164, #25733 ),
 .UNSPECIFIED., .F., .F. ) 
 B_SPLINE_CURVE_WITH_KNOTS ( ( 3, 2, 2, 2, 3 ),
 ( 0.9732142857142856984, 0.9738095238095237915, 0.9749999999999999778, 0.9761904761904761640, 0.9767857142857142572 ),
 .UNSPECIFIED. ) 
 CURVE ( )  GEOMETRIC_REPRESENTATION_ITEM ( )  RATIONAL_B_SPLINE_CURVE ( ( 0.9330127018922194093, 0.9330127018922194093, 1.000000000000000000, 0.8660254037844387076, 1.000000000000000000, 0.8660254037844387076, 1.000000000000000000, 0.9330127018922194093, 0.9330127018922194093 ) ) 
 REPRESENTATION_ITEM ( '' )  );
#55015=CARTESIAN_POINT ( 'NONE',  ( -2.499999999999996447, -48.70833333060213732, 4.330127018922195425 ) ) ;
#55017=CARTESIAN_POINT ( 'NONE',  ( 4.458734124999999437, 15.18750000136559564, -5.460374474430324690E-16 ) ) ;
#55018=CARTESIAN_POINT ( 'NONE',  ( 2.499999999999998668, -35.33333333333332860, -4.330127018922193649 ) ) ;
#55021=CARTESIAN_POINT ( 'NONE',  ( 2.229367062499998831, -67.64583333196773651, -3.861377020970580887 ) ) ;
#55022=VERTEX_POINT ( 'NONE', #41058 ) ;
#55024=CARTESIAN_POINT ( 'NONE',  ( 5.000000000000000888, 3.416666666666665186, 2.886751345948126879 ) ) ;
#55026=CARTESIAN_POINT ( 'NONE',  ( -2.499999999999996447, 22.16666666666666785, 4.330127018922195425 ) ) ;
#55027=CARTESIAN_POINT ( 'NONE',  ( -2.229367062499996610, -58.14583333196773651, 3.861377020970582219 ) ) ;
#55028=CARTESIAN_POINT ( 'NONE',  ( -2.500000000000000444, -95.04166666393547303, -4.330127018922193649 ) ) ;
#55029=CARTESIAN_POINT ( 'NONE',  ( -4.458734124999999437, -35.39583333196772941, -2.574251347313719407 ) ) ;
#55030=CARTESIAN_POINT ( 'NONE',  ( -5.000000000000000000, 20.04166666939785202, -2.886751345948128211 ) ) ;
#55033=CARTESIAN_POINT ( 'NONE',  ( 2.500000000000002220, 1.333333333333332149, 4.330127018922192761 ) ) ;
#55035=CARTESIAN_POINT ( 'NONE',  ( 2.499999999999998668, -44.33333333333333570, -4.330127018922193649 ) ) ;
#55038=CARTESIAN_POINT ( 'NONE',  ( 4.458734124999998549, -108.7291666653010651, -2.574251347313721627 ) ) ;
#55039=CARTESIAN_POINT ( 'NONE',  ( 4.458734125000001214, 4.854166668032262599, 2.574251347313718519 ) ) ;
#55042=VECTOR ( 'NONE', #51853, 1000.000000000000000 ) ;
#55045=CARTESIAN_POINT ( 'NONE',  ( 0.000000000000000000, 30.00000000000000000, 0.000000000000000000 ) ) ;
#55046=EDGE_CURVE ( 'NONE', #55022, #12016, #17357, .T. ) ;
#55047=ADVANCED_FACE ( 'NONE', ( #46535 ), #31735, .T. ) ;
#55052=CARTESIAN_POINT ( 'NONE',  ( -1.339745962155612258, 27.91965820146970856, -5.000000000000000888 ) ) ;
#55054=ORIENTED_EDGE ( 'NONE', *, *, #40980, .T. ) ;
#55057=CARTESIAN_POINT ( 'NONE',  ( 2.229367062500001939, -31.22916666530107221, 3.861377020970579999 ) ) ;
#55063=AXIS2_PLACEMENT_3D ( 'NONE', #10303, #1324, #41157 ) ;
#55066=LINE ( 'NONE', #5860, #29972 ) ;
#55067=VERTEX_POINT ( 'NONE', #51680 ) ;
#55069=CARTESIAN_POINT ( 'NONE',  ( -4.458734124999999437, -78.64583333196773651, -2.574251347313719407 ) ) ;
#55070=CARTESIAN_POINT ( 'NONE',  ( 1.975475456537005874E-15, 13.37500000273118417, 5.000000000000000000 ) ) ;
#55071=ORIENTED_EDGE ( 'NONE', *, *, #49164, .F. ) ;
#55072=FACE_OUTER_BOUND ( 'NONE', #4647, .T. ) ;
#55073=( BOUNDED_CURVE ( )  B_SPLINE_CURVE ( 2, ( #5297, #24915, #44519, #481, #45165, #46449, #31321, #50312, #6896 ),
 .UNSPECIFIED., .F., .F. ) 
 B_SPLINE_CURVE_WITH_KNOTS ( ( 3, 2, 2, 2, 3 ),
 ( 0.1232142857142857206, 0.1238095238095238138, 0.1250000000000000000, 0.1261904761904761862, 0.1267857142857142794 ),
 .UNSPECIFIED. ) 
 CURVE ( )  GEOMETRIC_REPRESENTATION_ITEM ( )  RATIONAL_B_SPLINE_CURVE ( ( 0.9330127018922192983, 0.9330127018922200755, 1.000000000000000000, 0.8660254037844387076, 1.000000000000000000, 0.8660254037844387076, 1.000000000000000000, 0.9330127018922194093, 0.9330127018922194093 ) ) 
 REPRESENTATION_ITEM ( '' )  );
#55074=CARTESIAN_POINT ( 'NONE',  ( -6.972266317189433020E-16, 7.750000000000000000, -5.000000000000000000 ) ) ;
#55076=CARTESIAN_POINT ( 'NONE',  ( -4.458734124999999437, -2.645833331967737845, -2.574251347313719407 ) ) ;
#55084=CARTESIAN_POINT ( 'NONE',  ( 5.000000000000000000, -75.37499999726880162, -6.123233995736766282E-16 ) ) ;
#55085=ORIENTED_EDGE ( 'NONE', *, *, #49600, .F. ) ;
#55086=CARTESIAN_POINT ( 'NONE',  ( 2.229367062500001939, -78.97916666530106511, 3.861377020970579999 ) ) ;
#55087=CARTESIAN_POINT ( 'NONE',  ( 4.458734124999999437, -5.812499998634403475, -5.460374474430324690E-16 ) ) ;
#55090=CARTESIAN_POINT ( 'NONE',  ( -2.229367062500000163, -70.72916666530107932, -3.861377020970580443 ) ) ;
#55091=CARTESIAN_POINT ( 'NONE',  ( -5.000000000000000000, -32.87499999726880873, 0.000000000000000000 ) ) ;
#55093=CARTESIAN_POINT ( 'NONE',  ( 9.457646018065525792E-16, 27.93750000136559208, 5.148502694627439702 ) ) ;
#55095=CARTESIAN_POINT ( 'NONE',  ( 2.229367062500001939, -52.97916666530107221, 3.861377020970579999 ) ) ;
#55096=CARTESIAN_POINT ( 'NONE',  ( -4.458734124999999437, -31.56249999863440436, 0.000000000000000000 ) ) ;
#55099=CARTESIAN_POINT ( 'NONE',  ( 0.000000000000000000, -120.0000000000000000, 5.000000000000000000 ) ) ;
#55100=CARTESIAN_POINT ( 'NONE',  ( -5.000000000000000000, 18.91666666666666430, -2.886751345948128211 ) ) ;
#55103=CARTESIAN_POINT ( 'NONE',  ( -4.458734124999999437, -44.39583333196773651, -2.574251347313719407 ) ) ;
#55104=CARTESIAN_POINT ( 'NONE',  ( -4.999999999999999112, -71.79166666393547303, 2.886751345948131764 ) ) ;
#55105=VECTOR ( 'NONE', #52749, 1000.000000000000000 ) ;
#55106=AXIS2_PLACEMENT_3D ( 'NONE', #40999, #8110, #3911 ) ;
#55109=CARTESIAN_POINT ( 'NONE',  ( -3.152548672688508926E-16, -77.81249999863440792, -5.148502694627439702 ) ) ;
#55111=DIRECTION ( 'NONE',  ( -0.000000000000000000, 1.000000000000000000, -0.000000000000000000 ) ) ;
#55112=CARTESIAN_POINT ( 'NONE',  ( 1.339745962155612702, 13.83034180399266333, -5.000000000000000000 ) ) ;
#55113=CARTESIAN_POINT ( 'NONE',  ( 5.000000000000000000, -25.41666666666666430, -2.886751345948129988 ) ) ;
#55119=CARTESIAN_POINT ( 'NONE',  ( -2.500000000000000444, 20.95833333606451987, -4.330127018922193649 ) ) ;
#55127=CARTESIAN_POINT ( 'NONE',  ( 5.000000000000000000, -99.29166666393545881, -2.886751345948130876 ) ) ;
#55128=CARTESIAN_POINT ( 'NONE',  ( 1.339745962155613146, 28.83034180399266688, -4.999999999999999112 ) ) ;
#55131=CARTESIAN_POINT ( 'NONE',  ( -2.229367062500000163, -13.72916666530107221, -3.861377020970580443 ) ) ;
#55132=EDGE_CURVE ( 'NONE', #46887, #35992, #56817, .T. ) ;
#55133=CARTESIAN_POINT ( 'NONE',  ( 5.000000000000000000, 17.70833333606451632, -2.886751345948130876 ) ) ;
#55138=EDGE_CURVE ( 'NONE', #10824, #14367, #63382, .T. ) ;
#55140=ORIENTED_EDGE ( 'NONE', *, *, #26597, .T. ) ;
#55143=ORIENTED_EDGE ( 'NONE', *, *, #50256, .T. ) ;
#55144=CARTESIAN_POINT ( 'NONE',  ( 5.000000000000000000, -21.50000000000000000, -6.123233995736766282E-16 ) ) ;
#55150=EDGE_CURVE ( 'NONE', #2700, #4593, #11323, .T. ) ;
#55155=ORIENTED_EDGE ( 'NONE', *, *, #12741, .F. ) ;
#55159=VECTOR ( 'NONE', #55669, 1000.000000000000000 ) ;
#55160=CARTESIAN_POINT ( 'NONE',  ( 4.458734124999998549, 13.27083333469892779, -2.574251347313721627 ) ) ;
#55161=EDGE_CURVE ( 'NONE', #10267, #39251, #2814, .T. ) ;
#55164=CARTESIAN_POINT ( 'NONE',  ( 1.339745962155615144, -44.70534180126146850, 4.999999999999999112 ) ) ;
#55166=CARTESIAN_POINT ( 'NONE',  ( -4.458734124999999437, -64.39583333196773651, -2.574251347313719407 ) ) ;
#55168=CARTESIAN_POINT ( 'NONE',  ( -2.229367062499996610, 14.85416666803226171, 3.861377020970582219 ) ) ;
#55170=CARTESIAN_POINT ( 'NONE',  ( 1.975475456537005874E-15, -68.62499999726881583, 5.000000000000000000 ) ) ;
#55171=CARTESIAN_POINT ( 'NONE',  ( 4.458734124999998549, -54.97916666530107221, -2.574251347313721627 ) ) ;
#55172=CARTESIAN_POINT ( 'NONE',  ( 2.499999999999998668, -11.20833333060214798, -4.330127018922193649 ) ) ;
#55173=CARTESIAN_POINT ( 'NONE',  ( -2.499999999999996447, -108.8333333333333428, 4.330127018922195425 ) ) ;
#55177=CARTESIAN_POINT ( 'NONE',  ( -3.152548672688508926E-16, -13.81249999863440259, -5.148502694627439702 ) ) ;
#55179=CARTESIAN_POINT ( 'NONE',  ( 4.458734125000001214, -101.8958333319677365, 2.574251347313718519 ) ) ;
#55181=VERTEX_POINT ( 'NONE', #103 ) ;
#55182=CARTESIAN_POINT ( 'NONE',  ( -3.152548672688508926E-16, -99.81249999863442213, -5.148502694627439702 ) ) ;
#55183=CARTESIAN_POINT ( 'NONE',  ( -2.229367062499996610, -27.14583333196774007, 3.861377020970582219 ) ) ;
#55184=CARTESIAN_POINT ( 'NONE',  ( 2.499999999999998668, -59.20833333060214443, -4.330127018922193649 ) ) ;
#55185=CARTESIAN_POINT ( 'NONE',  ( 5.000000000000000000, -62.37499999726880873, -6.123233995736766282E-16 ) ) ;
#55188=CARTESIAN_POINT ( 'NONE',  ( 9.457646018065525792E-16, -21.06249999863440436, 5.148502694627439702 ) ) ;
#55189=CARTESIAN_POINT ( 'NONE',  ( 9.457646018065525792E-16, -64.31249999863440792, 5.148502694627439702 ) ) ;
#55192=DIRECTION ( 'NONE',  ( -0.000000000000000000, 1.000000000000000000, -0.000000000000000000 ) ) ;
#55194=CARTESIAN_POINT ( 'NONE',  ( -5.000000000000000000, -12.08333333333333393, -2.886751345948128211 ) ) ;
#55196=ORIENTED_EDGE ( 'NONE', *, *, #30578, .F. ) ;
#55198=VECTOR ( 'NONE', #30222, 1000.000000000000000 ) ;
#55199=CARTESIAN_POINT ( 'NONE',  ( 0.000000000000000000, -120.0000000000000000, 0.000000000000000000 ) ) ;
#55202=VECTOR ( 'NONE', #25442, 1000.000000000000000 ) ;
#55203=AXIS2_PLACEMENT_3D ( 'NONE', #36416, #45752, #20681 ) ;
#55204=( BOUNDED_CURVE ( )  B_SPLINE_CURVE ( 2, ( #23189, #28946, #43739, #18674, #8407, #48252, #63069, #58227, #14156 ),
 .UNSPECIFIED., .F., .F. ) 
 B_SPLINE_CURVE_WITH_KNOTS ( ( 3, 2, 2, 2, 3 ),
 ( 0.5232142857142857428, 0.5238095238095238360, 0.5250000000000000222, 0.5261904761904762085, 0.5267857142857143016 ),
 .UNSPECIFIED. ) 
 CURVE ( )  GEOMETRIC_REPRESENTATION_ITEM ( )  RATIONAL_B_SPLINE_CURVE ( ( 0.9330127018922194093, 0.9330127018922194093, 1.000000000000000000, 0.8660254037844387076, 1.000000000000000000, 0.8660254037844387076, 1.000000000000000000, 0.9330127018922194093, 0.9330127018922194093 ) ) 
 REPRESENTATION_ITEM ( '' )  );
#55206=CARTESIAN_POINT ( 'NONE',  ( 5.000000000000000000, 1.625000002731184834, -6.123233995736766282E-16 ) ) ;
#55207=VECTOR ( 'NONE', #39484, 1000.000000000000000 ) ;
#55210=CARTESIAN_POINT ( 'NONE',  ( -3.535250795749689387E-16, -74.25000000000000000, -5.773502691896257311 ) ) ;
#55212=VERTEX_POINT ( 'NONE', #19700 ) ;
#55213=CARTESIAN_POINT ( 'NONE',  ( 0.000000000000000000, -120.0000000000000000, 5.000000000000000000 ) ) ;
#55214=VERTEX_POINT ( 'NONE', #39310 ) ;
#55215=CARTESIAN_POINT ( 'NONE',  ( -6.972266317189433020E-16, -54.12499999726880162, -5.000000000000000000 ) ) ;
#55233=CARTESIAN_POINT ( 'NONE',  ( -4.458734124999999437, -75.31249999863440792, 0.000000000000000000 ) ) ;
#55234=CARTESIAN_POINT ( 'NONE',  ( -4.458734124999998549, -109.4791666653010651, 2.574251347313722516 ) ) ;
#55241=CARTESIAN_POINT ( 'NONE',  ( 2.229367062499998831, -44.64583333196774362, -3.861377020970580887 ) ) ;
#55245=CARTESIAN_POINT ( 'NONE',  ( -4.458734124999999437, -51.39583333196773651, -2.574251347313719407 ) ) ;
#55247=CARTESIAN_POINT ( 'NONE',  ( -6.972266317189433020E-16, -73.25000000000000000, -5.000000000000000000 ) ) ;
#55249=CARTESIAN_POINT ( 'NONE',  ( -3.152548672688508926E-16, -18.56249999863440792, -5.148502694627439702 ) ) ;
#55250=CARTESIAN_POINT ( 'NONE',  ( 5.000000000000000888, -102.5833333333333428, 2.886751345948126879 ) ) ;
#55252=CARTESIAN_POINT ( 'NONE',  ( 9.457646018065525792E-16, -40.31249999863440081, 5.148502694627439702 ) ) ;
#55253=CARTESIAN_POINT ( 'NONE',  ( 2.499999999999998668, 4.791666669397852907, -4.330127018922193649 ) ) ;
#55254=DIRECTION ( 'NONE',  ( 0.000000000000000000, 0.000000000000000000, 1.000000000000000000 ) ) ;
#55258=CARTESIAN_POINT ( 'NONE',  ( 2.499999999999998668, -30.20833333060214443, -4.330127018922193649 ) ) ;
#55260=CARTESIAN_POINT ( 'NONE',  ( -2.229367062500000163, -1.729166665301071992, -3.861377020970580443 ) ) ;
#55262=CARTESIAN_POINT ( 'NONE',  ( -6.972266317189433020E-16, 24.87500000273118417, -5.000000000000000000 ) ) ;
#55263=CARTESIAN_POINT ( 'NONE',  ( 2.500000000000002220, -57.66666666666667140, 4.330127018922192761 ) ) ;
#55264=CARTESIAN_POINT ( 'NONE',  ( -4.458734124999999437, -89.39583333196773651, -2.574251347313719407 ) ) ;
#55265=CARTESIAN_POINT ( 'NONE',  ( 4.458734124999998549, -35.72916666530107221, -2.574251347313721627 ) ) ;
#55266=DIRECTION ( 'NONE',  ( -0.000000000000000000, 1.000000000000000000, -0.000000000000000000 ) ) ;
#55267=CARTESIAN_POINT ( 'NONE',  ( 4.458734124999999437, -81.06249999863440792, -5.460374474430324690E-16 ) ) ;
#55269=CARTESIAN_POINT ( 'NONE',  ( -1.339745962155610925, -52.79465819873851729, 5.000000000000000000 ) ) ;
#55271=CARTESIAN_POINT ( 'NONE',  ( -4.458734124999997661, -9.229166665301068662, 2.574251347313722516 ) ) ;
#55272=CARTESIAN_POINT ( 'NONE',  ( -2.229367062499996610, 20.60416666803225993, 3.861377020970582219 ) ) ;
#55273=CARTESIAN_POINT ( 'NONE',  ( -2.229367062499996610, -47.39583333196774362, 3.861377020970582219 ) ) ;
#55277=CARTESIAN_POINT ( 'NONE',  ( -4.330127018922205195, 30.00000000000000000, -7.499999999999943157 ) ) ;
#55282=CARTESIAN_POINT ( 'NONE',  ( -4.458734124999999437, -74.31249999863440792, 0.000000000000000000 ) ) ;
#55283=CARTESIAN_POINT ( 'NONE',  ( -4.458734124999998549, 28.52083333469892423, 2.574251347313722516 ) ) ;
#55285=DIRECTION ( 'NONE',  ( -0.000000000000000000, 1.000000000000000000, -0.000000000000000000 ) ) ;
#55288=CARTESIAN_POINT ( 'NONE',  ( 1.060575238724906964E-15, -59.74999999999999289, 5.773502691896257311 ) ) ;
#55292=CARTESIAN_POINT ( 'NONE',  ( 1.975475456537005874E-15, -56.75000000000000000, 5.000000000000000000 ) ) ;
#55299=CIRCLE ( 'NONE', #59362, 5.000000000000000000 ) ;
#55311=CARTESIAN_POINT ( 'NONE',  ( 2.229367062500001939, -44.22916666530106511, 3.861377020970579999 ) ) ;
#55312=CARTESIAN_POINT ( 'NONE',  ( -1.339745962155610925, -15.66965819600733134, 5.000000000000000000 ) ) ;
#55319=CARTESIAN_POINT ( 'NONE',  ( -2.500000000000000444, 0.8333333333333317050, -4.330127018922193649 ) ) ;
#55321=CARTESIAN_POINT ( 'NONE',  ( 4.458734124999998549, -96.97916666530106511, -2.574251347313721627 ) ) ;
#55324=DIRECTION ( 'NONE',  ( 0.000000000000000000, 0.000000000000000000, -1.000000000000000000 ) ) ;
#55327=ORIENTED_EDGE ( 'NONE', *, *, #48437, .T. ) ;
#55328=CARTESIAN_POINT ( 'NONE',  ( -2.229367062500000163, -3.479166665301069994, -3.861377020970580443 ) ) ;
#55330=CARTESIAN_POINT ( 'NONE',  ( 9.457646018065525792E-16, -16.31249999863440436, 5.148502694627439702 ) ) ;
#55333=DIRECTION ( 'NONE',  ( -0.000000000000000000, 1.000000000000000000, -0.000000000000000000 ) ) ;
#55336=CARTESIAN_POINT ( 'NONE',  ( 2.229367062500001939, 16.77083333469892779, 3.861377020970579999 ) ) ;
#55339=CARTESIAN_POINT ( 'NONE',  ( -2.500000000000000444, -13.16666666666666607, -4.330127018922193649 ) ) ;
#55340=CARTESIAN_POINT ( 'NONE',  ( -3.152548672688508926E-16, -17.56249999863440792, -5.148502694627439702 ) ) ;
#55342=VECTOR ( 'NONE', #6493, 1000.000000000000000 ) ;
#55343=FACE_OUTER_BOUND ( 'NONE', #18450, .T. ) ;
#55344=CARTESIAN_POINT ( 'NONE',  ( 5.000000000000000000, -3.416666666666665186, -2.886751345948130876 ) ) ;
#55346=CARTESIAN_POINT ( 'NONE',  ( 5.000000000000000000, -49.29166666393547303, -2.886751345948129988 ) ) ;
#55348=CARTESIAN_POINT ( 'NONE',  ( -3.152548672688508926E-16, 9.437500001365593860, -5.148502694627439702 ) ) ;
#55349=CARTESIAN_POINT ( 'NONE',  ( -1.339745962155555858, -9.080341798530296771, -5.000000000000032863 ) ) ;
#55350=CARTESIAN_POINT ( 'NONE',  ( 0.000000000000000000, -120.0000000000000000, 0.000000000000000000 ) ) ;
#55352=CARTESIAN_POINT ( 'NONE',  ( 2.229367062500001939, -68.97916666530107932, 3.861377020970579999 ) ) ;
#55354=CARTESIAN_POINT ( 'NONE',  ( 2.499999999999998668, 3.666666666666665186, -4.330127018922193649 ) ) ;
#55357=CARTESIAN_POINT ( 'NONE',  ( -3.152548672688508926E-16, -57.56249999863439371, -5.148502694627439702 ) ) ;
#55358=CARTESIAN_POINT ( 'NONE',  ( 2.500000000000002220, -95.54166666393547303, 4.330127018922192761 ) ) ;
#55359=LINE ( 'NONE', #11273, #40111 ) ;
#55360=ADVANCED_FACE ( 'NONE', ( #35781 ), #20345, .T. ) ;
#55361=CYLINDRICAL_SURFACE ( 'NONE', #41917, 5.000000000000000000 ) ;
#55364=CARTESIAN_POINT ( 'NONE',  ( -5.000000000000000000, -43.08333333333332860, -2.886751345948128211 ) ) ;
#55365=CARTESIAN_POINT ( 'NONE',  ( -4.999999999999998224, -107.9166666666666572, 2.886751345948131764 ) ) ;
#55367=CARTESIAN_POINT ( 'NONE',  ( 2.229367062500001939, -106.9791666653010651, 3.861377020970579999 ) ) ;
#55368=CARTESIAN_POINT ( 'NONE',  ( -4.458734124999999437, -3.645833331967739621, -2.574251347313719407 ) ) ;
#55372=DIRECTION ( 'NONE',  ( 0.000000000000000000, 1.000000000000000000, 0.000000000000000000 ) ) ;
#55375=ORIENTED_EDGE ( 'NONE', *, *, #62111, .T. ) ;
#55376=CARTESIAN_POINT ( 'NONE',  ( 1.339745962155615144, -22.58034179853029144, 4.999999999999999112 ) ) ;
#55380=CARTESIAN_POINT ( 'NONE',  ( -2.229367062499996610, -32.39583333196773651, 3.861377020970582219 ) ) ;
#55386=( BOUNDED_CURVE ( )  B_SPLINE_CURVE ( 2, ( #37933, #37300, #32791, #52421, #12850, #8655, #57565, #12222, #3841 ),
 .UNSPECIFIED., .F., .F. ) 
 B_SPLINE_CURVE_WITH_KNOTS ( ( 3, 2, 2, 2, 3 ),
 ( 0.7732142857142857428, 0.7738095238095238360, 0.7750000000000000222, 0.7761904761904762085, 0.7767857142857143016 ),
 .UNSPECIFIED. ) 
 CURVE ( )  GEOMETRIC_REPRESENTATION_ITEM ( )  RATIONAL_B_SPLINE_CURVE ( ( 0.9330127018922194093, 0.9330127018922194093, 1.000000000000000000, 0.8660254037844387076, 1.000000000000000000, 0.8660254037844387076, 1.000000000000000000, 0.9330127018922194093, 0.9330127018922194093 ) ) 
 REPRESENTATION_ITEM ( '' )  );
#55388=ORIENTED_EDGE ( 'NONE', *, *, #53805, .F. ) ;
#55389=FACE_OUTER_BOUND ( 'NONE', #33330, .T. ) ;
#55390=ORIENTED_EDGE ( 'NONE', *, *, #46144, .F. ) ;
#55391=CARTESIAN_POINT ( 'NONE',  ( -3.152548672688508926E-16, -76.81249999863440792, -5.148502694627439702 ) ) ;
#55392=FACE_OUTER_BOUND ( 'NONE', #34933, .T. ) ;
#55394=CARTESIAN_POINT ( 'NONE',  ( -5.000000000000000000, -14.95833333060214621, -2.886751345948128211 ) ) ;
#55395=CARTESIAN_POINT ( 'NONE',  ( 5.000000000000000000, -31.29166666393548724, -2.886751345948130876 ) ) ;
#55397=CARTESIAN_POINT ( 'NONE',  ( -2.229367062500000163, -2.729166665301069550, -3.861377020970580443 ) ) ;
#55398=ORIENTED_EDGE ( 'NONE', *, *, #31398, .T. ) ;
#55401=LINE ( 'NONE', #26437, #36827 ) ;
#55403=DIRECTION ( 'NONE',  ( 0.000000000000000000, 0.000000000000000000, 1.000000000000000000 ) ) ;
#55409=CARTESIAN_POINT ( 'NONE',  ( 4.458734125000000326, -82.89583333196773651, 2.574251347313718519 ) ) ;
#55410=DIRECTION ( 'NONE',  ( -0.000000000000000000, 1.000000000000000000, -0.000000000000000000 ) ) ;
#55411=CARTESIAN_POINT ( 'NONE',  ( 2.229367062500001939, -4.979166665301071326, 3.861377020970579999 ) ) ;
#55412=EDGE_CURVE ( 'NONE', #28777, #43561, #44456, .T. ) ;
#55415=CARTESIAN_POINT ( 'NONE',  ( -4.458734124999999437, -68.64583333196773651, -2.574251347313719407 ) ) ;
#55416=CARTESIAN_POINT ( 'NONE',  ( 5.000000000000000888, -30.45833333060214443, 2.886751345948126879 ) ) ;
#55418=CARTESIAN_POINT ( 'NONE',  ( 2.229367062500001939, 29.02083333469892779, 3.861377020970579999 ) ) ;
#55419=CARTESIAN_POINT ( 'NONE',  ( 5.000000000000000000, -104.4166666666666572, -2.886751345948130876 ) ) ;
#55421=CARTESIAN_POINT ( 'NONE',  ( -3.152548672688508926E-16, -51.56249999863441502, -5.148502694627439702 ) ) ;
#55422=CARTESIAN_POINT ( 'NONE',  ( 2.229367062499998831, -33.89583333196772941, -3.861377020970580887 ) ) ;
#55426=CARTESIAN_POINT ( 'NONE',  ( -2.499999999999996447, 19.16666666666666430, 4.330127018922195425 ) ) ;
#55429=EDGE_CURVE ( 'NONE', #63665, #6339, #49464, .T. ) ;
#55430=CARTESIAN_POINT ( 'NONE',  ( 2.229367062500001939, -43.97916666530106511, 3.861377020970579999 ) ) ;
#55431=CARTESIAN_POINT ( 'NONE',  ( -5.000000000000000000, -80.87499999726881583, 0.000000000000000000 ) ) ;
#55434=CARTESIAN_POINT ( 'NONE',  ( 5.000000000000000000, -37.41666666666666430, -2.886751345948130876 ) ) ;
#55435=EDGE_CURVE ( 'NONE', #43959, #20764, #60234, .T. ) ;
#55436=CARTESIAN_POINT ( 'NONE',  ( 2.229367062499998831, -78.89583333196773651, -3.861377020970580887 ) ) ;
#55438=DIRECTION ( 'NONE',  ( -0.000000000000000000, 1.000000000000000000, -0.000000000000000000 ) ) ;
#55439=CARTESIAN_POINT ( 'NONE',  ( -3.535250795749689387E-16, -28.24999999999999645, -5.773502691896257311 ) ) ;
#55441=ORIENTED_EDGE ( 'NONE', *, *, #3507, .F. ) ;
#55444=CARTESIAN_POINT ( 'NONE',  ( 2.500000000000002220, 23.45833333606451632, 4.330127018922192761 ) ) ;
#55450=CARTESIAN_POINT ( 'NONE',  ( -1.339745962155610925, 20.20534180126147916, 5.000000000000000000 ) ) ;
#55453=CARTESIAN_POINT ( 'NONE',  ( -6.972266317189433020E-16, -62.24999999999999289, -5.000000000000000000 ) ) ;
#55457=( BOUNDED_CURVE ( )  B_SPLINE_CURVE ( 2, ( #1582, #59799, #50770, #16676, #50461, #954, #35664, #20554, #10565 ),
 .UNSPECIFIED., .F., .F. ) 
 B_SPLINE_CURVE_WITH_KNOTS ( ( 3, 2, 2, 2, 3 ),
 ( 0.7482142857142857206, 0.7488095238095238138, 0.7500000000000000000, 0.7511904761904761862, 0.7517857142857142794 ),
 .UNSPECIFIED. ) 
 CURVE ( )  GEOMETRIC_REPRESENTATION_ITEM ( )  RATIONAL_B_SPLINE_CURVE ( ( 0.9330127018922194093, 0.9330127018922194093, 1.000000000000000000, 0.8660254037844387076, 1.000000000000000000, 0.8660254037844387076, 1.000000000000000000, 0.9330127018922194093, 0.9330127018922194093 ) ) 
 REPRESENTATION_ITEM ( '' )  );
#55458=CARTESIAN_POINT ( 'NONE',  ( 9.457646018065525792E-16, -13.31249999863440259, 5.148502694627439702 ) ) ;
#55466=ORIENTED_EDGE ( 'NONE', *, *, #48143, .T. ) ;
#55470=CARTESIAN_POINT ( 'NONE',  ( 1.975475456537005874E-15, -58.75000000000000000, 5.000000000000000000 ) ) ;
#55479=EDGE_LOOP ( 'NONE', ( #3341, #42805, #58523, #28888 ) ) ;
#55482=CARTESIAN_POINT ( 'NONE',  ( 4.458734125000001214, 13.10416666803226171, 2.574251347313718519 ) ) ;
#55485=CARTESIAN_POINT ( 'NONE',  ( 2.500000000000002220, -44.66666666666665719, 4.330127018922192761 ) ) ;
#55487=VERTEX_POINT ( 'NONE', #45745 ) ;
#55488=CARTESIAN_POINT ( 'NONE',  ( -4.458734124999999437, -63.39583333196772941, -2.574251347313719407 ) ) ;
#55490=CARTESIAN_POINT ( 'NONE',  ( 4.458734124999998549, 15.27083333469893134, -2.574251347313721627 ) ) ;
#55491=CARTESIAN_POINT ( 'NONE',  ( -4.999999999999998224, -62.91666666666665719, 2.886751345948131764 ) ) ;
#55494=EDGE_CURVE ( 'NONE', #39571, #2897, #46658, .T. ) ;
#55495=CARTESIAN_POINT ( 'NONE',  ( -4.458734124999998549, -56.47916666530107221, 2.574251347313722516 ) ) ;
#55496=CARTESIAN_POINT ( 'NONE',  ( 5.000000000000000888, -12.45833333060214976, 2.886751345948126879 ) ) ;
#55497=CARTESIAN_POINT ( 'NONE',  ( 2.499999999999998668, -25.20833333060214443, -4.330127018922193649 ) ) ;
#55499=LINE ( 'NONE', #11414, #56166 ) ;
#55500=EDGE_CURVE ( 'NONE', #20861, #9561, #7222, .T. ) ;
#55501=CARTESIAN_POINT ( 'NONE',  ( 2.229367062500001939, -15.22916666530107399, 3.861377020970579999 ) ) ;
#55503=( BOUNDED_CURVE ( )  B_SPLINE_CURVE ( 2, ( #60799, #36341, #25094, #44702, #39877, #54692, #10614, #1001, #35387 ),
 .UNSPECIFIED., .F., .F. ) 
 B_SPLINE_CURVE_WITH_KNOTS ( ( 3, 2, 2, 2, 3 ),
 ( 0.3410714285714285809, 0.3416666666666666741, 0.3428571428571428603, 0.3440476190476190466, 0.3446428571428571397 ),
 .UNSPECIFIED. ) 
 CURVE ( )  GEOMETRIC_REPRESENTATION_ITEM ( )  RATIONAL_B_SPLINE_CURVE ( ( 0.9330127018922194093, 0.9330127018922194093, 1.000000000000000000, 0.8660254037844387076, 1.000000000000000000, 0.8660254037844387076, 1.000000000000000000, 0.9330127018922194093, 0.9330127018922194093 ) ) 
 REPRESENTATION_ITEM ( '' )  );
#55505=CARTESIAN_POINT ( 'NONE',  ( 9.457646018065525792E-16, -102.0624999986344079, 5.148502694627439702 ) ) ;
#55508=CARTESIAN_POINT ( 'NONE',  ( 9.457646018065525792E-16, -104.3124999986344221, 5.148502694627439702 ) ) ;
#55509=CARTESIAN_POINT ( 'NONE',  ( -2.229367062500000163, -28.47916666530107221, -3.861377020970580443 ) ) ;
#55510=CARTESIAN_POINT ( 'NONE',  ( -3.535250795749689387E-16, -63.12499999726880873, -5.773502691896257311 ) ) ;
#55511=EDGE_CURVE ( 'NONE', #45629, #11153, #47474, .T. ) ;
#55514=CARTESIAN_POINT ( 'NONE',  ( -4.458734124999997661, -21.22916666530107221, 2.574251347313722516 ) ) ;
#55515=ADVANCED_FACE ( 'NONE', ( #27853 ), #22733, .T. ) ;
#55516=CARTESIAN_POINT ( 'NONE',  ( 2.229367062500001939, -62.22916666530106511, 3.861377020970579999 ) ) ;
#55517=CARTESIAN_POINT ( 'NONE',  ( 0.000000000000000000, -120.0000000000000000, 5.000000000000000000 ) ) ;
#55519=CARTESIAN_POINT ( 'NONE',  ( 6.123233995736766282E-16, -120.0000000000000000, -5.000000000000000000 ) ) ;
#55521=CARTESIAN_POINT ( 'NONE',  ( -2.500000000000000444, -12.16666666666666607, -4.330127018922193649 ) ) ;
#55522=EDGE_CURVE ( 'NONE', #22293, #42943, #35954, .T. ) ;
#55527=CYLINDRICAL_SURFACE ( 'NONE', #16072, 5.000000000000000000 ) ;
#55533=CARTESIAN_POINT ( 'NONE',  ( 1.975475456537005874E-15, -53.62499999726880162, 5.000000000000000000 ) ) ;
#55537=CARTESIAN_POINT ( 'NONE',  ( -2.499999999999996447, -81.83333333333332860, 4.330127018922195425 ) ) ;
#55539=ORIENTED_EDGE ( 'NONE', *, *, #22, .T. ) ;
#55540=ORIENTED_EDGE ( 'NONE', *, *, #2076, .F. ) ;
#55541=CARTESIAN_POINT ( 'NONE',  ( 1.339745962155611592, 26.29465819873852084, 5.000000000000000888 ) ) ;
#55545=ORIENTED_EDGE ( 'NONE', *, *, #13014, .T. ) ;
#55547=ORIENTED_EDGE ( 'NONE', *, *, #12282, .F. ) ;
#55555=CARTESIAN_POINT ( 'NONE',  ( 1.975475456537005874E-15, -83.74999999999998579, 5.000000000000000000 ) ) ;
#55556=VERTEX_POINT ( 'NONE', #56832 ) ;
#55557=CARTESIAN_POINT ( 'NONE',  ( -4.458734124999999437, -78.39583333196772230, -2.574251347313719407 ) ) ;
#55558=CARTESIAN_POINT ( 'NONE',  ( -2.229367062500000163, -108.7291666653010651, -3.861377020970580443 ) ) ;
#55565=CARTESIAN_POINT ( 'NONE',  ( -4.458734124999999437, -45.31249999863440081, 0.000000000000000000 ) ) ;
#55567=CYLINDRICAL_SURFACE ( 'NONE', #58947, 5.000000000000000000 ) ;
#55568=CARTESIAN_POINT ( 'NONE',  ( 4.458734124999999437, -49.81249999863440792, -5.460374474430324690E-16 ) ) ;
#55572=CARTESIAN_POINT ( 'NONE',  ( -3.152548672688508926E-16, -17.56249999863440792, -5.148502694627439702 ) ) ;
#55573=CARTESIAN_POINT ( 'NONE',  ( 2.499999999999998668, -101.3333333333333286, -4.330127018922193649 ) ) ;
#55575=CARTESIAN_POINT ( 'NONE',  ( 2.229367062499998831, -36.89583333196773651, -3.861377020970580887 ) ) ;
#55576=CARTESIAN_POINT ( 'NONE',  ( 2.500000000000002220, 0.4583333360645182042, 4.330127018922192761 ) ) ;
#55579=CARTESIAN_POINT ( 'NONE',  ( 2.499999999999998668, 24.66666666666666785, -4.330127018922193649 ) ) ;
#55580=CARTESIAN_POINT ( 'NONE',  ( 5.000000000000000888, -30.45833333060214443, 2.886751345948126879 ) ) ;
#55581=CARTESIAN_POINT ( 'NONE',  ( 9.457646018065525792E-16, -2.312499998634407028, 5.148502694627439702 ) ) ;
#55584=CARTESIAN_POINT ( 'NONE',  ( -2.229367062499996610, -88.14583333196773651, 3.861377020970582219 ) ) ;
#55586=CARTESIAN_POINT ( 'NONE',  ( -4.458734124999999437, -86.56249999863439371, 0.000000000000000000 ) ) ;
#55589=( BOUNDED_CURVE ( )  B_SPLINE_CURVE ( 2, ( #28884, #38847, #4443, #47564, #63309, #9585, #29191, #48817, #19551 ),
 .UNSPECIFIED., .F., .F. ) 
 B_SPLINE_CURVE_WITH_KNOTS ( ( 3, 2, 2, 2, 3 ),
 ( 0.3375000000000000222, 0.3380952380952381153, 0.3392857142857143016, 0.3404761904761904878, 0.3410714285714285809 ),
 .UNSPECIFIED. ) 
 CURVE ( )  GEOMETRIC_REPRESENTATION_ITEM ( )  RATIONAL_B_SPLINE_CURVE ( ( 0.9330127018922194093, 0.9330127018922194093, 1.000000000000000000, 0.8660254037844387076, 1.000000000000000000, 0.8660254037844387076, 1.000000000000000000, 0.9330127018922194093, 0.9330127018922194093 ) ) 
 REPRESENTATION_ITEM ( '' )  );
#55591=CARTESIAN_POINT ( 'NONE',  ( -4.458734124999997661, -5.229166665301072214, 2.574251347313722516 ) ) ;
#55592=CARTESIAN_POINT ( 'NONE',  ( -2.229367062500000163, 24.27083333469892779, -3.861377020970580443 ) ) ;
#55593=CARTESIAN_POINT ( 'NONE',  ( 2.229367062499998831, -47.89583333196774362, -3.861377020970580887 ) ) ;
#55599=EDGE_LOOP ( 'NONE', ( #7815, #49734, #47673 ) ) ;
#55603=CARTESIAN_POINT ( 'NONE',  ( -4.458734124999999437, -75.39583333196773651, -2.574251347313719407 ) ) ;
#55604=CARTESIAN_POINT ( 'NONE',  ( -5.000000000000000000, -108.9583333306021586, -2.886751345948128211 ) ) ;
#55606=ADVANCED_FACE ( 'NONE', ( #61655 ), #37512, .T. ) ;
#55607=CARTESIAN_POINT ( 'NONE',  ( -2.499999999999996447, -57.70833333060214443, 4.330127018922195425 ) ) ;
#55610=CARTESIAN_POINT ( 'NONE',  ( 5.000000000000000888, -65.58333333333332860, 2.886751345948126879 ) ) ;
#55615=CARTESIAN_POINT ( 'NONE',  ( 1.339745962155615144, -52.58034179853029144, 4.999999999999999112 ) ) ;
#55625=CARTESIAN_POINT ( 'NONE',  ( -1.339745962155610925, 11.33034180399266511, 5.000000000000000000 ) ) ;
#55627=ORIENTED_EDGE ( 'NONE', *, *, #753, .T. ) ;
#55630=CARTESIAN_POINT ( 'NONE',  ( -4.458734124999999437, -46.64583333196774362, -2.574251347313719407 ) ) ;
#55631=CARTESIAN_POINT ( 'NONE',  ( -2.499999999999996447, -95.83333333333332860, 4.330127018922195425 ) ) ;
#55638=DIRECTION ( 'NONE',  ( -0.000000000000000000, 1.000000000000000000, -0.000000000000000000 ) ) ;
#55640=CARTESIAN_POINT ( 'NONE',  ( -3.152548672688508926E-16, -95.81249999863440792, -5.148502694627439702 ) ) ;
#55641=CARTESIAN_POINT ( 'NONE',  ( -5.000000000000000000, -107.0833333333333428, -2.886751345948128211 ) ) ;
#55643=ORIENTED_EDGE ( 'NONE', *, *, #55132, .T. ) ;
#55647=CARTESIAN_POINT ( 'NONE',  ( 0.000000000000000000, -120.0000000000000000, 5.000000000000000000 ) ) ;
#55648=ORIENTED_EDGE ( 'NONE', *, *, #4109, .T. ) ;
#55649=CARTESIAN_POINT ( 'NONE',  ( 9.457646018065525792E-16, -0.06249999863440491854, 5.148502694627439702 ) ) ;
#55650=ADVANCED_FACE ( 'NONE', ( #16948 ), #7625, .T. ) ;
#55651=CARTESIAN_POINT ( 'NONE',  ( -3.152548672688508926E-16, -23.81249999863440792, -5.148502694627439702 ) ) ;
#55652=CARTESIAN_POINT ( 'NONE',  ( 5.000000000000000888, -72.58333333333332860, 2.886751345948126879 ) ) ;
#55654=CARTESIAN_POINT ( 'NONE',  ( 1.339745962155615144, 23.41965820146970501, 4.999999999999999112 ) ) ;
#55656=CARTESIAN_POINT ( 'NONE',  ( -4.458734124999999437, 13.35416666803225993, -2.574251347313719407 ) ) ;
#55659=CARTESIAN_POINT ( 'NONE',  ( 5.000000000000000000, -57.37499999726880162, -6.123233995736766282E-16 ) ) ;
#55660=CARTESIAN_POINT ( 'NONE',  ( -2.499999999999996447, -87.83333333333332860, 4.330127018922195425 ) ) ;
#55661=CARTESIAN_POINT ( 'NONE',  ( -4.458734124999999437, -21.39583333196774007, -2.574251347313719407 ) ) ;
#55662=AXIS2_PLACEMENT_3D ( 'NONE', #33883, #3373, #9433 ) ;
#55663=FACE_OUTER_BOUND ( 'NONE', #22163, .T. ) ;
#55666=CARTESIAN_POINT ( 'NONE',  ( 2.500000000000002220, -44.54166666393547303, 4.330127018922192761 ) ) ;
#55668=CARTESIAN_POINT ( 'NONE',  ( 9.457646018065525792E-16, 5.937500001365593860, 5.148502694627439702 ) ) ;
#55669=DIRECTION ( 'NONE',  ( -0.000000000000000000, 1.000000000000000000, -0.000000000000000000 ) ) ;
#55671=CARTESIAN_POINT ( 'NONE',  ( -4.458734124999998549, -66.22916666530107932, 2.574251347313722516 ) ) ;
#55673=CARTESIAN_POINT ( 'NONE',  ( -2.499999999999996447, -0.8333333333333317050, 4.330127018922195425 ) ) ;
#55675=CARTESIAN_POINT ( 'NONE',  ( -2.499999999999996447, 26.29166666939785202, 4.330127018922195425 ) ) ;
#55676=CARTESIAN_POINT ( 'NONE',  ( 2.229367062500001939, -59.97916666530106511, 3.861377020970579999 ) ) ;
#55677=CARTESIAN_POINT ( 'NONE',  ( -2.499999999999996447, -93.70833333060214443, 4.330127018922195425 ) ) ;
#55678=FACE_OUTER_BOUND ( 'NONE', #59536, .T. ) ;
#55682=CARTESIAN_POINT ( 'NONE',  ( -5.000000000000000000, -47.08333333333333570, -2.886751345948128211 ) ) ;
#55683=CARTESIAN_POINT ( 'NONE',  ( 2.500000000000002220, -13.66666666666666785, 4.330127018922192761 ) ) ;
#55684=CARTESIAN_POINT ( 'NONE',  ( 2.500000000000002220, -17.54166666393547658, 4.330127018922192761 ) ) ;
#55685=ORIENTED_EDGE ( 'NONE', *, *, #7948, .T. ) ;
#55686=CARTESIAN_POINT ( 'NONE',  ( -2.229367062500000163, -107.4791666653010651, -3.861377020970580443 ) ) ;
#55687=CARTESIAN_POINT ( 'NONE',  ( 4.458734125000001214, -4.145833331967740065, 2.574251347313718519 ) ) ;
#55688=( BOUNDED_CURVE ( )  B_SPLINE_CURVE ( 2, ( #28644, #18988, #42182, #18372, #38307, #42494, #52787, #52481, #47637 ),
 .UNSPECIFIED., .F., .F. ) 
 B_SPLINE_CURVE_WITH_KNOTS ( ( 3, 2, 2, 2, 3 ),
 ( 0.8910714285714286254, 0.8916666666666667185, 0.8928571428571429047, 0.8940476190476190910, 0.8946428571428571841 ),
 .UNSPECIFIED. ) 
 CURVE ( )  GEOMETRIC_REPRESENTATION_ITEM ( )  RATIONAL_B_SPLINE_CURVE ( ( 0.9330127018922194093, 0.9330127018922256266, 1.000000000000000000, 0.8660254037844387076, 1.000000000000000000, 0.8660254037844387076, 1.000000000000000000, 0.9330127018922194093, 0.9330127018922194093 ) ) 
 REPRESENTATION_ITEM ( '' )  );
#55689=CARTESIAN_POINT ( 'NONE',  ( 5.000000000000000000, -73.37499999726880162, -6.123233995736766282E-16 ) ) ;
#55695=VERTEX_POINT ( 'NONE', #12112 ) ;
#55701=CARTESIAN_POINT ( 'NONE',  ( -2.229367062500000163, -28.72916666530107221, -3.861377020970580443 ) ) ;
#55706=EDGE_CURVE ( 'NONE', #39750, #44922, #42512, .T. ) ;
#55710=ORIENTED_EDGE ( 'NONE', *, *, #51104, .T. ) ;
#55711=CARTESIAN_POINT ( 'NONE',  ( 4.458734124999999437, -81.06249999863440792, -5.460374474430324690E-16 ) ) ;
#55713=VERTEX_POINT ( 'NONE', #4664 ) ;
#55714=DIRECTION ( 'NONE',  ( 0.000000000000000000, 0.000000000000000000, 1.000000000000000000 ) ) ;
#55717=CARTESIAN_POINT ( 'NONE',  ( -4.458734124999999437, -10.64583333196773829, -2.574251347313719407 ) ) ;
#55718=ORIENTED_EDGE ( 'NONE', *, *, #14881, .T. ) ;
#55719=CARTESIAN_POINT ( 'NONE',  ( -2.500000000000000444, -10.04166666393547658, -4.330127018922193649 ) ) ;
#55722=CARTESIAN_POINT ( 'NONE',  ( 4.458734124999999437, -7.062499998634404363, -5.460374474430324690E-16 ) ) ;
#55726=CARTESIAN_POINT ( 'NONE',  ( -4.458734124999997661, -89.22916666530107932, 2.574251347313722516 ) ) ;
#55727=CARTESIAN_POINT ( 'NONE',  ( -6.972266317189433020E-16, -29.12499999726880873, -5.000000000000000000 ) ) ;
#55728=CARTESIAN_POINT ( 'NONE',  ( -4.458734124999999437, -4.312499998634401699, 0.000000000000000000 ) ) ;
#55730=CARTESIAN_POINT ( 'NONE',  ( 2.500000000000002220, -30.54166666393548013, 4.330127018922192761 ) ) ;
#55731=CARTESIAN_POINT ( 'NONE',  ( 4.330127018922154569, 45.00000000000000000, -7.499999999999971578 ) ) ;
#55732=CARTESIAN_POINT ( 'NONE',  ( 9.457646018065525792E-16, 21.93750000136559208, 5.148502694627439702 ) ) ;
#55733=CARTESIAN_POINT ( 'NONE',  ( -5.000000000000000000, 23.00000000000000000, 0.000000000000000000 ) ) ;
#55735=CARTESIAN_POINT ( 'NONE',  ( -2.229367062499996610, -53.14583333196773651, 3.861377020970582219 ) ) ;
#55736=CARTESIAN_POINT ( 'NONE',  ( -4.458734124999997661, -35.47916666530107221, 2.574251347313722516 ) ) ;
#55739=CARTESIAN_POINT ( 'NONE',  ( -5.000000000000000000, 14.91666666666666607, -2.886751345948128211 ) ) ;
#55741=DIRECTION ( 'NONE',  ( 0.000000000000000000, 0.000000000000000000, 1.000000000000000000 ) ) ;
#55742=CARTESIAN_POINT ( 'NONE',  ( -4.458734124999998549, -43.22916666530105800, 2.574251347313722516 ) ) ;
#55743=CARTESIAN_POINT ( 'NONE',  ( 5.000000000000000000, -78.37499999726881583, -6.123233995736766282E-16 ) ) ;
#55745=CARTESIAN_POINT ( 'NONE',  ( -6.972266317189433020E-16, -24.12499999726881228, -5.000000000000000000 ) ) ;
#55747=CARTESIAN_POINT ( 'NONE',  ( -4.458734124999997661, -83.47916666530106511, 2.574251347313722516 ) ) ;
#55750=CARTESIAN_POINT ( 'NONE',  ( -3.535250795749689387E-16, -25.25000000000000355, -5.773502691896257311 ) ) ;
#55752=VERTEX_POINT ( 'NONE', #23673 ) ;
#55755=CARTESIAN_POINT ( 'NONE',  ( -4.458734124999999437, -91.39583333196773651, -2.574251347313719407 ) ) ;
#55756=CARTESIAN_POINT ( 'NONE',  ( -2.229367062500000163, 13.27083333469892779, -3.861377020970580443 ) ) ;
#55757=CARTESIAN_POINT ( 'NONE',  ( -5.000000000000000000, 15.04166666939785202, -2.886751345948128211 ) ) ;
#55765=CARTESIAN_POINT ( 'NONE',  ( 5.000000000000000000, 15.62500000273118417, -6.123233995736766282E-16 ) ) ;
#55766=CARTESIAN_POINT ( 'NONE',  ( 1.339745962155641346, -1.294658198738521282, -4.999999999999983125 ) ) ;
#55767=CARTESIAN_POINT ( 'NONE',  ( 1.975475456537005874E-15, 18.37500000273118062, 5.000000000000000000 ) ) ;
#55770=FACE_OUTER_BOUND ( 'NONE', #13725, .T. ) ;
#55771=CARTESIAN_POINT ( 'NONE',  ( 4.458734125000001214, -12.14583333196774007, 2.574251347313718519 ) ) ;
#55781=ORIENTED_EDGE ( 'NONE', *, *, #8730, .F. ) ;
#55789=CARTESIAN_POINT ( 'NONE',  ( 0.000000000000000000, -120.0000000000000000, 5.000000000000000000 ) ) ;
#55793=CARTESIAN_POINT ( 'NONE',  ( 2.499999999999998668, 11.66666666666666607, -4.330127018922193649 ) ) ;
#55795=CARTESIAN_POINT ( 'NONE',  ( 4.458734125000001214, 12.10416666803226171, 2.574251347313718519 ) ) ;
#55800=ORIENTED_EDGE ( 'NONE', *, *, #61839, .T. ) ;
#55801=CARTESIAN_POINT ( 'NONE',  ( 4.458734124999999437, -72.81249999863439371, -5.460374474430324690E-16 ) ) ;
#55802=CARTESIAN_POINT ( 'NONE',  ( -5.000000000000000000, -49.87499999726881583, 0.000000000000000000 ) ) ;
#55803=CARTESIAN_POINT ( 'NONE',  ( -2.229367062499996610, 11.85416666803225993, 3.861377020970582219 ) ) ;
#55804=EDGE_CURVE ( 'NONE', #14586, #34023, #29334, .T. ) ;
#55805=CARTESIAN_POINT ( 'NONE',  ( 6.158835246850667461E-14, 7.875000002731183280, -4.999999999999999112 ) ) ;
#55806=FACE_OUTER_BOUND ( 'NONE', #42307, .T. ) ;
#55807=CARTESIAN_POINT ( 'NONE',  ( 2.229367062499998831, -53.89583333196773651, -3.861377020970580887 ) ) ;
#55808=CARTESIAN_POINT ( 'NONE',  ( 5.000000000000000888, -14.45833333060214976, 2.886751345948126879 ) ) ;
#55810=CARTESIAN_POINT ( 'NONE',  ( -6.972266317189433020E-16, -105.2500000000000000, -5.000000000000000000 ) ) ;
#55811=CARTESIAN_POINT ( 'NONE',  ( 4.458734124999999437, -21.06249999863440436, -5.460374474430324690E-16 ) ) ;
#55813=CARTESIAN_POINT ( 'NONE',  ( -1.339745962155613812, -61.20534180126147561, -5.000000000000000000 ) ) ;
#55814=CARTESIAN_POINT ( 'NONE',  ( -4.458734124999999437, -105.3124999986344221, 0.000000000000000000 ) ) ;
#55817=CARTESIAN_POINT ( 'NONE',  ( 4.458734124999999437, -105.0624999986344079, -5.460374474430324690E-16 ) ) ;
#55818=CARTESIAN_POINT ( 'NONE',  ( 4.458734125000001214, -26.89583333196774007, 2.574251347313718519 ) ) ;
#55819=CARTESIAN_POINT ( 'NONE',  ( -4.999999999999999112, -64.79166666393547303, 2.886751345948131764 ) ) ;
#55822=EDGE_CURVE ( 'NONE', #56685, #6898, #13771, .T. ) ;
#55823=CARTESIAN_POINT ( 'NONE',  ( 4.458734125000000326, -24.89583333196773651, 2.574251347313718519 ) ) ;
#55824=CARTESIAN_POINT ( 'NONE',  ( -2.229367062500000163, -66.72916666530106511, -3.861377020970580443 ) ) ;
#55825=CARTESIAN_POINT ( 'NONE',  ( -6.972266317189433020E-16, -32.12499999726880873, -5.000000000000000000 ) ) ;
#55827=CARTESIAN_POINT ( 'NONE',  ( 2.499999999999998668, -32.33333333333332860, -4.330127018922193649 ) ) ;
#55829=CARTESIAN_POINT ( 'NONE',  ( 1.060575238724906964E-15, -10.75000000000000178, 5.773502691896257311 ) ) ;
#55837=CARTESIAN_POINT ( 'NONE',  ( 6.158835246850666199E-14, -2.250000000000001776, -4.999999999999999112 ) ) ;
#55840=DIRECTION ( 'NONE',  ( -0.000000000000000000, 1.000000000000000000, -0.000000000000000000 ) ) ;
#55844=ORIENTED_EDGE ( 'NONE', *, *, #12199, .T. ) ;
#55847=DIRECTION ( 'NONE',  ( -0.000000000000000000, 1.000000000000000000, -0.000000000000000000 ) ) ;
#55851=VECTOR ( 'NONE', #2632, 1000.000000000000000 ) ;
#55854=ADVANCED_FACE ( 'NONE', ( #57465 ), #13384, .T. ) ;
#55860=( BOUNDED_CURVE ( )  B_SPLINE_CURVE ( 2, ( #3713, #23329, #32339, #42933, #46818, #2762, #7592, #38119, #57742 ),
 .UNSPECIFIED., .F., .F. ) 
 B_SPLINE_CURVE_WITH_KNOTS ( ( 3, 2, 2, 2, 3 ),
 ( 0.7839285714285714191, 0.7845238095238095122, 0.7857142857142856984, 0.7869047619047618847, 0.7874999999999999778 ),
 .UNSPECIFIED. ) 
 CURVE ( )  GEOMETRIC_REPRESENTATION_ITEM ( )  RATIONAL_B_SPLINE_CURVE ( ( 0.9330127018922194093, 0.9330127018922194093, 1.000000000000000000, 0.8660254037844387076, 1.000000000000000000, 0.8660254037844387076, 1.000000000000000000, 0.9330127018922194093, 0.9330127018922194093 ) ) 
 REPRESENTATION_ITEM ( '' )  );
#55861=CARTESIAN_POINT ( 'NONE',  ( 5.000000000000000888, -55.58333333333332860, 2.886751345948126879 ) ) ;
#55866=EDGE_CURVE ( 'NONE', #35606, #39571, #5133, .T. ) ;
#55867=ORIENTED_EDGE ( 'NONE', *, *, #46874, .T. ) ;
#55868=CARTESIAN_POINT ( 'NONE',  ( 2.229367062500001939, -75.97916666530106511, 3.861377020970579999 ) ) ;
#55869=EDGE_CURVE ( 'NONE', #2392, #54097, #20350, .T. ) ;
#55870=CARTESIAN_POINT ( 'NONE',  ( -3.152548672688508926E-16, 28.43750000136559208, -5.148502694627439702 ) ) ;
#55871=CARTESIAN_POINT ( 'NONE',  ( 1.975475456537005874E-15, -53.74999999999999289, 5.000000000000000000 ) ) ;
#55881=CARTESIAN_POINT ( 'NONE',  ( 4.458734124999999437, -51.81249999863440792, -5.460374474430324690E-16 ) ) ;
#55883=CARTESIAN_POINT ( 'NONE',  ( 4.458734124999998549, 28.27083333469892779, -2.574251347313721627 ) ) ;
#55884=CARTESIAN_POINT ( 'NONE',  ( -4.999999999999999112, -106.9166666666666572, 2.886751345948131764 ) ) ;
#55886=CARTESIAN_POINT ( 'NONE',  ( 9.457646018065525792E-16, -38.31249999863441502, 5.148502694627439702 ) ) ;
#55887=CARTESIAN_POINT ( 'NONE',  ( 5.000000000000000000, -1.291666663935479908, -2.886751345948129988 ) ) ;
#55891=CARTESIAN_POINT ( 'NONE',  ( 1.339745962155615144, 24.29465819873852084, 4.999999999999999112 ) ) ;
#55892=CARTESIAN_POINT ( 'NONE',  ( 2.229367062499998831, -97.64583333196773651, -3.861377020970580887 ) ) ;
#55893=CARTESIAN_POINT ( 'NONE',  ( 2.229367062499998831, -2.895833331967738289, -3.861377020970580887 ) ) ;
#55897=CARTESIAN_POINT ( 'NONE',  ( -2.229367062499996610, -87.14583333196773651, 3.861377020970582219 ) ) ;
#55898=FACE_OUTER_BOUND ( 'NONE', #61952, .T. ) ;
#55899=CARTESIAN_POINT ( 'NONE',  ( -4.458734124999998549, -88.47916666530107932, 2.574251347313722516 ) ) ;
#55902=AXIS2_PLACEMENT_3D ( 'NONE', #3590, #57932, #42808 ) ;
#55904=CARTESIAN_POINT ( 'NONE',  ( -2.229367062499996610, -5.145833331967740065, 3.861377020970582219 ) ) ;
#55905=CARTESIAN_POINT ( 'NONE',  ( 4.458734125000001214, 14.85416666803225993, 2.574251347313718519 ) ) ;
#55906=CARTESIAN_POINT ( 'NONE',  ( -2.229367062499996610, -46.39583333196774362, 3.861377020970582219 ) ) ;
#55913=CARTESIAN_POINT ( 'NONE',  ( -2.229367062499996610, -77.14583333196773651, 3.861377020970582219 ) ) ;
#55914=CARTESIAN_POINT ( 'NONE',  ( 4.458734124999999437, 28.93750000136559208, -5.460374474430324690E-16 ) ) ;
#55916=CARTESIAN_POINT ( 'NONE',  ( -1.339745962155610925, -93.79465819873851729, 5.000000000000000000 ) ) ;
#55917=LINE ( 'NONE', #7029, #10089 ) ;
#55919=CARTESIAN_POINT ( 'NONE',  ( -3.535250795749689387E-16, -65.25000000000000000, -5.773502691896257311 ) ) ;
#55920=CARTESIAN_POINT ( 'NONE',  ( -5.000000000000000000, -31.95833333060214443, -2.886751345948128211 ) ) ;
#55922=ORIENTED_EDGE ( 'NONE', *, *, #10976, .F. ) ;
#55929=ADVANCED_FACE ( 'NONE', ( #5311 ), #24929, .T. ) ;
#55932=EDGE_LOOP ( 'NONE', ( #40586, #39036, #6637, #1451 ) ) ;
#55933=CARTESIAN_POINT ( 'NONE',  ( 1.975475456537005874E-15, -91.74999999999998579, 5.000000000000000000 ) ) ;
#55936=ORIENTED_EDGE ( 'NONE', *, *, #35533, .T. ) ;
#55939=CARTESIAN_POINT ( 'NONE',  ( 9.457646018065525792E-16, -46.31249999863440792, 5.148502694627439702 ) ) ;
#55940=CARTESIAN_POINT ( 'NONE',  ( -2.500000000000000444, -96.16666666666665719, -4.330127018922193649 ) ) ;
#55950=CARTESIAN_POINT ( 'NONE',  ( 9.457646018065525792E-16, -95.31249999863440792, 5.148502694627439702 ) ) ;
#55957=ADVANCED_FACE ( 'NONE', ( #54838 ), #10768, .T. ) ;
#55958=CARTESIAN_POINT ( 'NONE',  ( 2.499999999999998668, -60.33333333333333570, -4.330127018922193649 ) ) ;
#55959=CARTESIAN_POINT ( 'NONE',  ( -4.458734124999998549, -2.229166665301068662, 2.574251347313722516 ) ) ;
#55960=( BOUNDED_CURVE ( )  B_SPLINE_CURVE ( 2, ( #36393, #60850, #31568, #51201, #7135, #52773, #14149, #32514, #33159 ),
 .UNSPECIFIED., .F., .F. ) 
 B_SPLINE_CURVE_WITH_KNOTS ( ( 3, 2, 2, 2, 3 ),
 ( 0.8017857142857143238, 0.8023809523809524169, 0.8035714285714286031, 0.8047619047619047894, 0.8053571428571428825 ),
 .UNSPECIFIED. ) 
 CURVE ( )  GEOMETRIC_REPRESENTATION_ITEM ( )  RATIONAL_B_SPLINE_CURVE ( ( 0.9330127018922194093, 0.9330127018922194093, 1.000000000000000000, 0.8660254037844387076, 1.000000000000000000, 0.8660254037844387076, 1.000000000000000000, 0.9330127018922194093, 0.9330127018922194093 ) ) 
 REPRESENTATION_ITEM ( '' )  );
#55961=CARTESIAN_POINT ( 'NONE',  ( -4.458734124999997661, -97.47916666530105090, 2.574251347313722516 ) ) ;
#55962=ADVANCED_FACE ( 'NONE', ( #49040 ), #34559, .T. ) ;
#55964=CARTESIAN_POINT ( 'NONE',  ( -4.458734124999999437, -24.56249999863440436, 0.000000000000000000 ) ) ;
#55970=CARTESIAN_POINT ( 'NONE',  ( 2.229367062499998831, 16.10416666803225993, -3.861377020970580887 ) ) ;
#55971=ORIENTED_EDGE ( 'NONE', *, *, #44976, .F. ) ;
#55973=CARTESIAN_POINT ( 'NONE',  ( -6.972266317189433020E-16, -57.12499999726879452, -5.000000000000000000 ) ) ;
#55974=CARTESIAN_POINT ( 'NONE',  ( -2.499999999999996447, -83.83333333333332860, 4.330127018922195425 ) ) ;
#55975=CARTESIAN_POINT ( 'NONE',  ( -4.458734124999998549, -19.22916666530106866, 2.574251347313722516 ) ) ;
#55979=CARTESIAN_POINT ( 'NONE',  ( -5.000000000000000000, -47.87499999726880873, 0.000000000000000000 ) ) ;
#55980=CARTESIAN_POINT ( 'NONE',  ( 1.339745962155612702, -41.16965819600732601, -5.000000000000000000 ) ) ;
#55981=CARTESIAN_POINT ( 'NONE',  ( -4.458734124999997661, 7.770833334698926009, 2.574251347313722516 ) ) ;
#55982=DIRECTION ( 'NONE',  ( 0.000000000000000000, 0.000000000000000000, 1.000000000000000000 ) ) ;
#55983=DIRECTION ( 'NONE',  ( 0.000000000000000000, 0.000000000000000000, 1.000000000000000000 ) ) ;
#55985=CARTESIAN_POINT ( 'NONE',  ( -2.229367062500000163, -65.47916666530106511, -3.861377020970580443 ) ) ;
#55987=CARTESIAN_POINT ( 'NONE',  ( -3.535250795749689387E-16, -0.2500000000000002220, -5.773502691896257311 ) ) ;
#55990=CARTESIAN_POINT ( 'NONE',  ( -3.152548672688508926E-16, -58.56249999863440081, -5.148502694627439702 ) ) ;
#55991=CARTESIAN_POINT ( 'NONE',  ( 2.500000000000002220, -93.54166666393547303, 4.330127018922192761 ) ) ;
#55992=AXIS2_PLACEMENT_3D ( 'NONE', #14458, #49512, #15102 ) ;
#55994=DIRECTION ( 'NONE',  ( -0.000000000000000000, 1.000000000000000000, -0.000000000000000000 ) ) ;
#55996=CARTESIAN_POINT ( 'NONE',  ( 1.975475456537005874E-15, -90.62499999726880162, 5.000000000000000000 ) ) ;
#55997=CARTESIAN_POINT ( 'NONE',  ( 2.499999999999998668, -49.33333333333332860, -4.330127018922193649 ) ) ;
#55998=CARTESIAN_POINT ( 'NONE',  ( 0.000000000000000000, -120.0000000000000000, 5.000000000000000000 ) ) ;
#56001=CARTESIAN_POINT ( 'NONE',  ( 9.457646018065525792E-16, -108.0624999986343937, 5.148502694627439702 ) ) ;
#56002=CARTESIAN_POINT ( 'NONE',  ( -4.458734124999998549, -0.4791666653010707710, 2.574251347313722516 ) ) ;
#56003=CARTESIAN_POINT ( 'NONE',  ( 2.500000000000002220, -73.54166666393548724, 4.330127018922192761 ) ) ;
#56010=CARTESIAN_POINT ( 'NONE',  ( -6.972266317189433020E-16, -17.12499999726881583, -5.000000000000000000 ) ) ;
#56013=( BOUNDED_CURVE ( )  B_SPLINE_CURVE ( 2, ( #55871, #41370, #1850, #7304, #60384, #27534, #51039, #12431, #31401 ),
 .UNSPECIFIED., .F., .F. ) 
 B_SPLINE_CURVE_WITH_KNOTS ( ( 3, 2, 2, 2, 3 ),
 ( 0.5982142857142856984, 0.5988095238095237915, 0.5999999999999999778, 0.6011904761904761640, 0.6017857142857142572 ),
 .UNSPECIFIED. ) 
 CURVE ( )  GEOMETRIC_REPRESENTATION_ITEM ( )  RATIONAL_B_SPLINE_CURVE ( ( 0.9330127018922194093, 0.9330127018922194093, 1.000000000000000000, 0.8660254037844387076, 1.000000000000000000, 0.8660254037844387076, 1.000000000000000000, 0.9330127018922194093, 0.9330127018922194093 ) ) 
 REPRESENTATION_ITEM ( '' )  );
#56017=CARTESIAN_POINT ( 'NONE',  ( 4.458734125000001214, -29.14583333196774362, 2.574251347313718519 ) ) ;
#56024=CARTESIAN_POINT ( 'NONE',  ( 1.975475456537005874E-15, -70.62499999726880162, 5.000000000000000000 ) ) ;
#56025=VERTEX_POINT ( 'NONE', #25563 ) ;
#56026=CARTESIAN_POINT ( 'NONE',  ( -4.458734124999999437, -80.56249999863440792, 0.000000000000000000 ) ) ;
#56027=CARTESIAN_POINT ( 'NONE',  ( 2.499999999999998668, 3.666666666666665186, -4.330127018922193649 ) ) ;
#56032=CARTESIAN_POINT ( 'NONE',  ( 4.458734125000001214, -7.145833331967734736, 2.574251347313718519 ) ) ;
#56033=ORIENTED_EDGE ( 'NONE', *, *, #17481, .F. ) ;
#56034=VECTOR ( 'NONE', #17027, 1000.000000000000000 ) ;
#56035=CARTESIAN_POINT ( 'NONE',  ( -2.499999999999996447, -84.83333333333332860, 4.330127018922195425 ) ) ;
#56038=CARTESIAN_POINT ( 'NONE',  ( 2.229367062499998831, -5.895833331967740953, -3.861377020970580887 ) ) ;
#56043=CARTESIAN_POINT ( 'NONE',  ( -6.972266317189433020E-16, -37.12499999726880873, -5.000000000000000000 ) ) ;
#56045=CARTESIAN_POINT ( 'NONE',  ( -4.458734124999997661, -85.22916666530107932, 2.574251347313722516 ) ) ;
#56046=FACE_OUTER_BOUND ( 'NONE', #26160, .T. ) ;
#56047=CARTESIAN_POINT ( 'NONE',  ( -4.458734124999999437, -2.395833331967737845, -2.574251347313719407 ) ) ;
#56049=CARTESIAN_POINT ( 'NONE',  ( -5.000000000000000000, -28.87499999726881228, 0.000000000000000000 ) ) ;
#56051=CARTESIAN_POINT ( 'NONE',  ( 9.457646018065525792E-16, 23.93750000136559564, 5.148502694627439702 ) ) ;
#56052=CARTESIAN_POINT ( 'NONE',  ( -2.499999999999996447, -94.83333333333332860, 4.330127018922195425 ) ) ;
#56054=CARTESIAN_POINT ( 'NONE',  ( 2.229367062499998831, -51.64583333196773651, -3.861377020970580887 ) ) ;
#56055=CARTESIAN_POINT ( 'NONE',  ( -4.458734124999999437, -38.56249999863440081, 0.000000000000000000 ) ) ;
#56057=( BOUNDED_CURVE ( )  B_SPLINE_CURVE ( 2, ( #29584, #29905, #5793, #59517, #15766, #35382, #19307, #54035, #38921 ),
 .UNSPECIFIED., .F., .F. ) 
 B_SPLINE_CURVE_WITH_KNOTS ( ( 3, 2, 2, 2, 3 ),
 ( 0.7339285714285714857, 0.7345238095238095788, 0.7357142857142857650, 0.7369047619047619513, 0.7375000000000000444 ),
 .UNSPECIFIED. ) 
 CURVE ( )  GEOMETRIC_REPRESENTATION_ITEM ( )  RATIONAL_B_SPLINE_CURVE ( ( 0.9330127018922194093, 0.9330127018922256266, 1.000000000000000000, 0.8660254037844387076, 1.000000000000000000, 0.8660254037844387076, 1.000000000000000000, 0.9330127018922194093, 0.9330127018922194093 ) ) 
 REPRESENTATION_ITEM ( '' )  );
#56058=CARTESIAN_POINT ( 'NONE',  ( -6.972266317189433020E-16, -18.25000000000000000, -5.000000000000000000 ) ) ;
#56059=CARTESIAN_POINT ( 'NONE',  ( -5.000000000000000000, 16.00000000000000000, 0.000000000000000000 ) ) ;
#56062=CARTESIAN_POINT ( 'NONE',  ( -2.229367062499996610, -45.14583333196774362, 3.861377020970582219 ) ) ;
#56063=CARTESIAN_POINT ( 'NONE',  ( 5.000000000000000888, -78.45833333060214443, 2.886751345948126879 ) ) ;
#56067=CARTESIAN_POINT ( 'NONE',  ( 9.457646018065525792E-16, -85.31249999863439371, 5.148502694627439702 ) ) ;
#56070=CARTESIAN_POINT ( 'NONE',  ( -3.535250795749689387E-16, -33.25000000000000000, -5.773502691896257311 ) ) ;
#56074=CARTESIAN_POINT ( 'NONE',  ( -4.458734124999999437, -89.31249999863440792, 0.000000000000000000 ) ) ;
#56075=CARTESIAN_POINT ( 'NONE',  ( 4.458734124999999437, 12.93750000136559208, -5.460374474430324690E-16 ) ) ;
#56076=CARTESIAN_POINT ( 'NONE',  ( -3.535250795749689387E-16, 15.87500000273118417, -5.773502691896257311 ) ) ;
#56077=CARTESIAN_POINT ( 'NONE',  ( -1.336351044127974539E-14, 25.24999999999999645, 5.000000000000000000 ) ) ;
#56082=CARTESIAN_POINT ( 'NONE',  ( 5.000000000000000000, 15.70833333606451809, -2.886751345948130876 ) ) ;
#56084=CARTESIAN_POINT ( 'NONE',  ( -2.499999999999996447, 18.29166666939785202, 4.330127018922195425 ) ) ;
#56088=CARTESIAN_POINT ( 'NONE',  ( -4.458734124999999437, -12.64583333196774007, -2.574251347313719407 ) ) ;
#56089=CARTESIAN_POINT ( 'NONE',  ( -2.500000000000000444, -58.16666666666665719, -4.330127018922193649 ) ) ;
#56096=VERTEX_POINT ( 'NONE', #1462 ) ;
#56098=ORIENTED_EDGE ( 'NONE', *, *, #56171, .T. ) ;
#56099=CARTESIAN_POINT ( 'NONE',  ( 4.458734124999998549, -61.97916666530106511, -2.574251347313721627 ) ) ;
#56101=CARTESIAN_POINT ( 'NONE',  ( 2.499999999999998668, -8.333333333333332149, -4.330127018922193649 ) ) ;
#56103=ORIENTED_EDGE ( 'NONE', *, *, #28594, .F. ) ;
#56110=CARTESIAN_POINT ( 'NONE',  ( -3.152548672688508926E-16, 8.437500001365595637, -5.148502694627439702 ) ) ;
#56113=CARTESIAN_POINT ( 'NONE',  ( 5.000000000000000000, -78.29166666393547303, -2.886751345948130876 ) ) ;
#56116=CARTESIAN_POINT ( 'NONE',  ( -2.229367062500000163, -70.47916666530107932, -3.861377020970580443 ) ) ;
#56118=CARTESIAN_POINT ( 'NONE',  ( 9.457646018065525792E-16, 14.93750000136559564, 5.148502694627439702 ) ) ;
#56119=AXIS2_PLACEMENT_3D ( 'NONE', #50129, #1905, #49808 ) ;
#56121=FACE_OUTER_BOUND ( 'NONE', #20307, .T. ) ;
#56122=DIRECTION ( 'NONE',  ( 0.000000000000000000, 0.000000000000000000, 1.000000000000000000 ) ) ;
#56123=CARTESIAN_POINT ( 'NONE',  ( 2.229367062500001939, -57.22916666530107932, 3.861377020970579999 ) ) ;
#56124=CARTESIAN_POINT ( 'NONE',  ( 5.000000000000000000, -14.37499999726881228, -6.123233995736766282E-16 ) ) ;
#56125=CYLINDRICAL_SURFACE ( 'NONE', #50151, 5.000000000000000000 ) ;
#56126=CARTESIAN_POINT ( 'NONE',  ( -1.339745962155613812, -45.08034179853028434, -5.000000000000000000 ) ) ;
#56128=CARTESIAN_POINT ( 'NONE',  ( -3.152548672688508926E-16, -19.81249999863440081, -5.148502694627439702 ) ) ;
#56129=ORIENTED_EDGE ( 'NONE', *, *, #43284, .T. ) ;
#56131=CARTESIAN_POINT ( 'NONE',  ( -2.500000000000000444, 29.83333333333333215, -4.330127018922193649 ) ) ;
#56135=CARTESIAN_POINT ( 'NONE',  ( 9.457646018065525792E-16, -102.3124999986344221, 5.148502694627439702 ) ) ;
#56137=CARTESIAN_POINT ( 'NONE',  ( 2.229367062499998831, -26.64583333196774007, -3.861377020970580887 ) ) ;
#56138=CARTESIAN_POINT ( 'NONE',  ( -5.000000000000000000, -63.95833333060213732, -2.886751345948128211 ) ) ;
#56142=CARTESIAN_POINT ( 'NONE',  ( 2.229367062500001939, -22.97916666530107221, 3.861377020970579999 ) ) ;
#56143=CARTESIAN_POINT ( 'NONE',  ( -3.152548672688508926E-16, -71.81249999863439371, -5.148502694627439702 ) ) ;
#56147=CARTESIAN_POINT ( 'NONE',  ( -2.500000000000000444, -17.16666666666666430, -4.330127018922193649 ) ) ;
#56152=CARTESIAN_POINT ( 'NONE',  ( 6.123233995736766282E-16, -120.0000000000000000, -5.000000000000000000 ) ) ;
#56154=CARTESIAN_POINT ( 'NONE',  ( 6.123233995736766282E-16, -120.0000000000000000, -5.000000000000000000 ) ) ;
#56156=( BOUNDED_CURVE ( )  B_SPLINE_CURVE ( 2, ( #40254, #39920, #11294, #40567, #21275, #59568, #50546, #59895, #15815 ),
 .UNSPECIFIED., .F., .F. ) 
 B_SPLINE_CURVE_WITH_KNOTS ( ( 3, 2, 2, 2, 3 ),
 ( 0.9375000000000000000, 0.9380952380952380931, 0.9392857142857142794, 0.9404761904761904656, 0.9410714285714285587 ),
 .UNSPECIFIED. ) 
 CURVE ( )  GEOMETRIC_REPRESENTATION_ITEM ( )  RATIONAL_B_SPLINE_CURVE ( ( 0.9330127018922194093, 0.9330127018922194093, 1.000000000000000000, 0.8660254037844387076, 1.000000000000000000, 0.8660254037844387076, 1.000000000000000000, 0.9330127018922194093, 0.9330127018922194093 ) ) 
 REPRESENTATION_ITEM ( '' )  );
#56157=EDGE_CURVE ( 'NONE', #51535, #51665, #16240, .T. ) ;
#56164=ORIENTED_EDGE ( 'NONE', *, *, #38743, .T. ) ;
#56166=VECTOR ( 'NONE', #31033, 1000.000000000000000 ) ;
#56170=VECTOR ( 'NONE', #62578, 1000.000000000000000 ) ;
#56171=EDGE_CURVE ( 'NONE', #29860, #33989, #44961, .T. ) ;
#56173=VERTEX_POINT ( 'NONE', #22660 ) ;
#56178=LINE ( 'NONE', #61325, #37480 ) ;
#56179=EDGE_LOOP ( 'NONE', ( #62674, #54690, #36543, #10576 ) ) ;
#56182=EDGE_LOOP ( 'NONE', ( #19120, #49115, #26535, #21540 ) ) ;
#56183=EDGE_CURVE ( 'NONE', #7429, #59301, #49076, .T. ) ;
#56184=CARTESIAN_POINT ( 'NONE',  ( 9.457646018065525792E-16, -77.06249999863440792, 5.148502694627439702 ) ) ;
#56185=CARTESIAN_POINT ( 'NONE',  ( 2.229367062499998831, 25.35416666803225993, -3.861377020970580887 ) ) ;
#56187=ORIENTED_EDGE ( 'NONE', *, *, #11497, .F. ) ;
#56192=DIRECTION ( 'NONE',  ( 0.000000000000000000, -0.000000000000000000, 1.000000000000000000 ) ) ;
#56195=CARTESIAN_POINT ( 'NONE',  ( -4.458734124999999437, -57.31249999863440081, 0.000000000000000000 ) ) ;
#56197=CARTESIAN_POINT ( 'NONE',  ( 2.229367062499998831, 26.35416666803225993, -3.861377020970580887 ) ) ;
#56198=CARTESIAN_POINT ( 'NONE',  ( -5.000000000000000000, -106.9999999999999858, 0.000000000000000000 ) ) ;
#56200=CARTESIAN_POINT ( 'NONE',  ( 4.458734124999999437, -39.06249999863440081, -5.460374474430324690E-16 ) ) ;
#56201=CARTESIAN_POINT ( 'NONE',  ( 5.000000000000000000, -1.374999997268814500, -6.123233995736766282E-16 ) ) ;
#56205=CARTESIAN_POINT ( 'NONE',  ( 9.457646018065525792E-16, -105.0624999986344079, 5.148502694627439702 ) ) ;
#56206=CARTESIAN_POINT ( 'NONE',  ( 2.229367062499998831, -5.895833331967740953, -3.861377020970580887 ) ) ;
#56207=( BOUNDED_CURVE ( )  B_SPLINE_CURVE ( 2, ( #39567, #30559, #55018, #20928, #60491, #20285, #30887, #40532, #60174 ),
 .UNSPECIFIED., .F., .F. ) 
 B_SPLINE_CURVE_WITH_KNOTS ( ( 3, 2, 2, 2, 3 ),
 ( 0.4660714285714285809, 0.4666666666666666741, 0.4678571428571428603, 0.4690476190476190466, 0.4696428571428571397 ),
 .UNSPECIFIED. ) 
 CURVE ( )  GEOMETRIC_REPRESENTATION_ITEM ( )  RATIONAL_B_SPLINE_CURVE ( ( 0.9330127018922194093, 0.9330127018922194093, 1.000000000000000000, 0.8660254037844387076, 1.000000000000000000, 0.8660254037844387076, 1.000000000000000000, 0.9330127018922194093, 0.9330127018922194093 ) ) 
 REPRESENTATION_ITEM ( '' )  );
#56209=AXIS2_PLACEMENT_3D ( 'NONE', #11001, #20673, #55403 ) ;
#56211=CARTESIAN_POINT ( 'NONE',  ( -1.339745962155613812, -36.08034179853029144, -5.000000000000000000 ) ) ;
#56212=CARTESIAN_POINT ( 'NONE',  ( 2.229367062500001939, -94.97916666530106511, 3.861377020970579999 ) ) ;
#56214=CARTESIAN_POINT ( 'NONE',  ( 9.457646018065525792E-16, -89.31249999863440792, 5.148502694627439702 ) ) ;
#56221=VECTOR ( 'NONE', #41967, 1000.000000000000000 ) ;
#56222=CARTESIAN_POINT ( 'NONE',  ( -4.458734124999999437, -9.395833331967736513, -2.574251347313719407 ) ) ;
#56223=CARTESIAN_POINT ( 'NONE',  ( -2.229367062500000163, 16.27083333469892779, -3.861377020970580443 ) ) ;
#56224=CARTESIAN_POINT ( 'NONE',  ( -4.458734124999997661, -52.47916666530107221, 2.574251347313722516 ) ) ;
#56225=CARTESIAN_POINT ( 'NONE',  ( -1.339745962155599601, 16.91965820146970501, -5.000000000000007994 ) ) ;
#56228=CARTESIAN_POINT ( 'NONE',  ( 5.000000000000000888, -106.4583333306021586, 2.886751345948126879 ) ) ;
#56229=ORIENTED_EDGE ( 'NONE', *, *, #51725, .T. ) ;
#56232=CARTESIAN_POINT ( 'NONE',  ( -4.458734124999998549, -81.22916666530106511, 2.574251347313722516 ) ) ;
#56233=CARTESIAN_POINT ( 'NONE',  ( -4.999999999999999112, -109.7916666639354730, 2.886751345948131764 ) ) ;
#56240=CARTESIAN_POINT ( 'NONE',  ( 2.500000000000002220, -64.66666666666665719, 4.330127018922192761 ) ) ;
#56241=CARTESIAN_POINT ( 'NONE',  ( 5.000000000000000888, -63.45833333060215153, 2.886751345948126879 ) ) ;
#56245=( BOUNDED_CURVE ( )  B_SPLINE_CURVE ( 2, ( #15958, #1190, #31705, #11756, #31374, #1825, #36528, #21426, #40392 ),
 .UNSPECIFIED., .F., .F. ) 
 B_SPLINE_CURVE_WITH_KNOTS ( ( 3, 2, 2, 2, 3 ),
 ( 0.8874999999999999556, 0.8880952380952380487, 0.8892857142857142350, 0.8904761904761904212, 0.8910714285714286254 ),
 .UNSPECIFIED. ) 
 CURVE ( )  GEOMETRIC_REPRESENTATION_ITEM ( )  RATIONAL_B_SPLINE_CURVE ( ( 0.9330127018922194093, 0.9330127018922194093, 1.000000000000000000, 0.8660254037844387076, 1.000000000000000000, 0.8660254037844387076, 1.000000000000000000, 0.9330127018922130810, 0.9330127018922194093 ) ) 
 REPRESENTATION_ITEM ( '' )  );
#56246=CARTESIAN_POINT ( 'NONE',  ( -1.975475456537005874E-15, 28.25000000000000000, 5.000000000000000000 ) ) ;
#56247=LINE ( 'NONE', #16681, #36925 ) ;
#56259=CARTESIAN_POINT ( 'NONE',  ( 9.457646018065525792E-16, -51.31249999863440792, 5.148502694627439702 ) ) ;
#56265=EDGE_CURVE ( 'NONE', #26190, #56652, #60197, .T. ) ;
#56270=CARTESIAN_POINT ( 'NONE',  ( -4.458734124999999437, -99.64583333196773651, -2.574251347313719407 ) ) ;
#56271=CARTESIAN_POINT ( 'NONE',  ( -6.972266317189433020E-16, -21.12499999726881228, -5.000000000000000000 ) ) ;
#56272=EDGE_LOOP ( 'NONE', ( #62125, #31936, #25314, #17431 ) ) ;
#56275=CARTESIAN_POINT ( 'NONE',  ( 1.975475456537005874E-15, -60.75000000000000000, 5.000000000000000000 ) ) ;
#56276=CARTESIAN_POINT ( 'NONE',  ( -4.458734124999999437, -3.312499998634407916, 0.000000000000000000 ) ) ;
#56277=CARTESIAN_POINT ( 'NONE',  ( 9.457646018065525792E-16, -95.31249999863440792, 5.148502694627439702 ) ) ;
#56279=CARTESIAN_POINT ( 'NONE',  ( 2.229367062500001939, -25.22916666530106866, 3.861377020970579999 ) ) ;
#56283=CARTESIAN_POINT ( 'NONE',  ( 2.500000000000002220, -72.66666666666667140, 4.330127018922192761 ) ) ;
#56286=CARTESIAN_POINT ( 'NONE',  ( 9.457646018065525792E-16, 10.68750000136559386, 5.148502694627439702 ) ) ;
#56288=LINE ( 'NONE', #62379, #13047 ) ;
#56289=CARTESIAN_POINT ( 'NONE',  ( 5.000000000000000000, -87.50000000000000000, -6.123233995736766282E-16 ) ) ;
#56290=CARTESIAN_POINT ( 'NONE',  ( 4.458734124999999437, -23.81249999863440436, -5.460374474430324690E-16 ) ) ;
#56294=EDGE_CURVE ( 'NONE', #16469, #12275, #24857, .T. ) ;
#56296=CARTESIAN_POINT ( 'NONE',  ( 2.499999999999998668, -47.20833333060214443, -4.330127018922193649 ) ) ;
#56297=CARTESIAN_POINT ( 'NONE',  ( 6.158835246850667461E-14, -2.124999997268816276, -4.999999999999999112 ) ) ;
#56298=CARTESIAN_POINT ( 'NONE',  ( 9.457646018065525792E-16, 7.937500001365596525, 5.148502694627439702 ) ) ;
#56299=FACE_OUTER_BOUND ( 'NONE', #50349, .T. ) ;
#56303=CARTESIAN_POINT ( 'NONE',  ( 2.229367062500001939, -64.97916666530106511, 3.861377020970579999 ) ) ;
#56306=VECTOR ( 'NONE', #50983, 1000.000000000000000 ) ;
#56307=CARTESIAN_POINT ( 'NONE',  ( -2.500000000000000444, -0.1666666666666656582, -4.330127018922193649 ) ) ;
#56309=CARTESIAN_POINT ( 'NONE',  ( -3.152548672688508926E-16, -62.56249999863440792, -5.148502694627439702 ) ) ;
#56310=CARTESIAN_POINT ( 'NONE',  ( -2.500000000000000444, -93.04166666393547303, -4.330127018922193649 ) ) ;
#56313=EDGE_CURVE ( 'NONE', #18131, #45003, #53224, .T. ) ;
#56314=CARTESIAN_POINT ( 'NONE',  ( -5.000000000000000000, -80.00000000000000000, 0.000000000000000000 ) ) ;
#56315=CARTESIAN_POINT ( 'NONE',  ( 5.000000000000000888, -56.58333333333333570, 2.886751345948126879 ) ) ;
#56317=EDGE_CURVE ( 'NONE', #456, #11867, #25233, .T. ) ;
#56318=CARTESIAN_POINT ( 'NONE',  ( 6.123233995736766282E-16, -114.9999999999999858, -5.000000000000000000 ) ) ;
#56320=CARTESIAN_POINT ( 'NONE',  ( -2.499999999999996447, -48.83333333333332860, 4.330127018922195425 ) ) ;
#56321=CARTESIAN_POINT ( 'NONE',  ( -6.972266317189433020E-16, -72.12499999726878741, -5.000000000000000000 ) ) ;
#56324=CARTESIAN_POINT ( 'NONE',  ( -4.458734124999999437, -106.3958333319677507, -2.574251347313719407 ) ) ;
#56325=CARTESIAN_POINT ( 'NONE',  ( 4.458734124999998549, -2.979166665301069994, -2.574251347313721627 ) ) ;
#56329=EDGE_CURVE ( 'NONE', #40984, #143, #48696, .T. ) ;
#56331=VECTOR ( 'NONE', #12276, 1000.000000000000000 ) ;
#56332=LINE ( 'NONE', #62098, #25718 ) ;
#56342=CARTESIAN_POINT ( 'NONE',  ( -3.152548672688508926E-16, -36.81249999863440792, -5.148502694627439702 ) ) ;
#56352=CARTESIAN_POINT ( 'NONE',  ( -4.458734124999999437, -78.56249999863440792, 0.000000000000000000 ) ) ;
#56353=CARTESIAN_POINT ( 'NONE',  ( 1.339745962155612702, 3.705341801261478718, -5.000000000000000000 ) ) ;
#56355=CARTESIAN_POINT ( 'NONE',  ( -5.000000000000000000, -14.87499999726881228, 0.000000000000000000 ) ) ;
#56356=VECTOR ( 'NONE', #5069, 1000.000000000000000 ) ;
#56359=CARTESIAN_POINT ( 'NONE',  ( 2.229367062499998831, -9.895833331967738289, -3.861377020970580887 ) ) ;
#56360=ORIENTED_EDGE ( 'NONE', *, *, #35745, .F. ) ;
#56362=CARTESIAN_POINT ( 'NONE',  ( 5.000000000000000000, 17.50000000000000000, -6.123233995736766282E-16 ) ) ;
#56363=CARTESIAN_POINT ( 'NONE',  ( 2.229367062500001939, -6.229166665301072214, 3.861377020970579999 ) ) ;
#56367=CARTESIAN_POINT ( 'NONE',  ( -3.152548672688508926E-16, 29.18750000136559208, -5.148502694627439702 ) ) ;
#56369=CARTESIAN_POINT ( 'NONE',  ( 9.457646018065525792E-16, -86.06249999863439371, 5.148502694627439702 ) ) ;
#56370=CARTESIAN_POINT ( 'NONE',  ( -5.000000000000000000, -67.99999999999998579, 0.000000000000000000 ) ) ;
#56371=CARTESIAN_POINT ( 'NONE',  ( 4.458734125000001214, -0.8958333319677401763, 2.574251347313718519 ) ) ;
#56374=CARTESIAN_POINT ( 'NONE',  ( 5.000000000000000000, -32.29166666393548724, -2.886751345948129988 ) ) ;
#56375=DIRECTION ( 'NONE',  ( -1.000000000000000000, 0.000000000000000000, 0.000000000000000000 ) ) ;
#56376=CARTESIAN_POINT ( 'NONE',  ( -2.229367062500000163, 22.52083333469892423, -3.861377020970580443 ) ) ;
#56377=CARTESIAN_POINT ( 'NONE',  ( -2.500000000000000444, -21.04166666393548013, -4.330127018922193649 ) ) ;
#56379=CARTESIAN_POINT ( 'NONE',  ( 9.457646018065525792E-16, -50.06249999863440792, 5.148502694627439702 ) ) ;
#56380=CARTESIAN_POINT ( 'NONE',  ( -3.152548672688508926E-16, -37.81249999863440792, -5.148502694627439702 ) ) ;
#56383=CARTESIAN_POINT ( 'NONE',  ( -3.535250795749689387E-16, 13.75000000000000000, -5.773502691896257311 ) ) ;
#56385=CARTESIAN_POINT ( 'NONE',  ( 1.975475456537005874E-15, -70.62499999726880162, 5.000000000000000000 ) ) ;
#56386=CARTESIAN_POINT ( 'NONE',  ( 4.458734124999999437, -42.81249999863440081, -5.460374474430324690E-16 ) ) ;
#56387=CARTESIAN_POINT ( 'NONE',  ( -2.500000000000000444, -81.04166666393547303, -4.330127018922193649 ) ) ;
#56390=CARTESIAN_POINT ( 'NONE',  ( -2.500000000000000444, -64.04166666393547303, -4.330127018922193649 ) ) ;
#56391=CARTESIAN_POINT ( 'NONE',  ( -4.458734124999999437, -87.64583333196773651, -2.574251347313719407 ) ) ;
#56394=CARTESIAN_POINT ( 'NONE',  ( -5.000000000000000000, -33.08333333333332149, -2.886751345948128211 ) ) ;
#56396=VERTEX_POINT ( 'NONE', #38071 ) ;
#56400=CARTESIAN_POINT ( 'NONE',  ( 4.458734124999999437, -89.81249999863440792, -5.460374474430324690E-16 ) ) ;
#56401=CARTESIAN_POINT ( 'NONE',  ( 2.229367062499998831, 16.10416666803225993, -3.861377020970580887 ) ) ;
#56403=CARTESIAN_POINT ( 'NONE',  ( 2.499999999999998668, 13.79166666939785202, -4.330127018922193649 ) ) ;
#56404=CARTESIAN_POINT ( 'NONE',  ( -1.339745962155613812, -29.08034179853029144, -5.000000000000000000 ) ) ;
#56409=CARTESIAN_POINT ( 'NONE',  ( -6.972266317189433020E-16, -52.25000000000000711, -5.000000000000000000 ) ) ;
#56416=CARTESIAN_POINT ( 'NONE',  ( 4.458734125000001214, -14.14583333196774184, 2.574251347313718519 ) ) ;
#56425=CARTESIAN_POINT ( 'NONE',  ( 1.339745962155615144, -85.58034179853028434, 4.999999999999999112 ) ) ;
#56427=( BOUNDED_CURVE ( )  B_SPLINE_CURVE ( 2, ( #6549, #40321, #1428, #30984, #15567, #5589, #60595, #50930, #21027 ),
 .UNSPECIFIED., .F., .F. ) 
 B_SPLINE_CURVE_WITH_KNOTS ( ( 3, 2, 2, 2, 3 ),
 ( 0.6410714285714286254, 0.6416666666666667185, 0.6428571428571429047, 0.6440476190476190910, 0.6446428571428571841 ),
 .UNSPECIFIED. ) 
 CURVE ( )  GEOMETRIC_REPRESENTATION_ITEM ( )  RATIONAL_B_SPLINE_CURVE ( ( 0.9330127018922194093, 0.9330127018922256266, 1.000000000000000000, 0.8660254037844387076, 1.000000000000000000, 0.8660254037844387076, 1.000000000000000000, 0.9330127018922194093, 0.9330127018922194093 ) ) 
 REPRESENTATION_ITEM ( '' )  );
#56428=CARTESIAN_POINT ( 'NONE',  ( 2.229367062499998831, -61.89583333196774362, -3.861377020970580887 ) ) ;
#56431=ORIENTED_EDGE ( 'NONE', *, *, #40450, .T. ) ;
#56434=CARTESIAN_POINT ( 'NONE',  ( -6.972266317189433020E-16, -85.25000000000000000, -5.000000000000000000 ) ) ;
#56436=EDGE_LOOP ( 'NONE', ( #3357, #20343, #31246, #39696 ) ) ;
#56437=CARTESIAN_POINT ( 'NONE',  ( 1.975475456537005874E-15, -109.6249999972688158, 5.000000000000000000 ) ) ;
#56438=CARTESIAN_POINT ( 'NONE',  ( 4.458734125000001214, 9.104166668032261711, 2.574251347313718519 ) ) ;
#56444=ORIENTED_EDGE ( 'NONE', *, *, #62832, .F. ) ;
#56445=CARTESIAN_POINT ( 'NONE',  ( 4.458734125000000326, -68.89583333196773651, 2.574251347313718519 ) ) ;
#56446=DIRECTION ( 'NONE',  ( -0.000000000000000000, 1.000000000000000000, -0.000000000000000000 ) ) ;
#56447=CARTESIAN_POINT ( 'NONE',  ( -4.458734124999999437, 13.60416666803226349, -2.574251347313719407 ) ) ;
#56449=DIRECTION ( 'NONE',  ( -0.000000000000000000, 1.000000000000000000, -0.000000000000000000 ) ) ;
#56450=CARTESIAN_POINT ( 'NONE',  ( -4.458734124999998549, -53.47916666530106511, 2.574251347313722516 ) ) ;
#56451=CARTESIAN_POINT ( 'NONE',  ( -3.535250795749689387E-16, -12.12499999726881761, -5.773502691896257311 ) ) ;
#56452=FACE_OUTER_BOUND ( 'NONE', #58502, .T. ) ;
#56455=CARTESIAN_POINT ( 'NONE',  ( 2.229367062499998831, -33.64583333196772941, -3.861377020970580887 ) ) ;
#56456=CARTESIAN_POINT ( 'NONE',  ( 2.229367062500001939, -22.22916666530107221, 3.861377020970579999 ) ) ;
#56457=ORIENTED_EDGE ( 'NONE', *, *, #8306, .F. ) ;
#56459=CARTESIAN_POINT ( 'NONE',  ( -4.999999999999999112, 29.08333333333333215, 2.886751345948131764 ) ) ;
#56462=CARTESIAN_POINT ( 'NONE',  ( 4.458734125000001214, -102.1458333319677365, 2.574251347313718519 ) ) ;
#56463=CARTESIAN_POINT ( 'NONE',  ( -2.229367062500000163, -27.47916666530107221, -3.861377020970580443 ) ) ;
#56464=CARTESIAN_POINT ( 'NONE',  ( -2.500000000000000444, -63.04166666393547303, -4.330127018922193649 ) ) ;
#56467=CARTESIAN_POINT ( 'NONE',  ( -4.458734124999999437, -30.31249999863440436, 0.000000000000000000 ) ) ;
#56468=CARTESIAN_POINT ( 'NONE',  ( -4.458734124999999437, -68.56249999863439371, 0.000000000000000000 ) ) ;
#56471=CARTESIAN_POINT ( 'NONE',  ( -1.339745962155613812, -33.20534180126147561, -5.000000000000000000 ) ) ;
#56473=CARTESIAN_POINT ( 'NONE',  ( -2.500000000000000444, -14.16666666666666785, -4.330127018922193649 ) ) ;
#56476=CARTESIAN_POINT ( 'NONE',  ( -6.031010364368858512E-14, 3.249999999999997335, 5.000000000000000000 ) ) ;
#56479=CARTESIAN_POINT ( 'NONE',  ( 1.975475456537005874E-15, -81.62499999726881583, 5.000000000000000000 ) ) ;
#56481=CARTESIAN_POINT ( 'NONE',  ( 5.000000000000000000, -76.37499999726880162, -6.123233995736766282E-16 ) ) ;
#56496=ORIENTED_EDGE ( 'NONE', *, *, #11489, .F. ) ;
#56498=ORIENTED_EDGE ( 'NONE', *, *, #57098, .T. ) ;
#56505=CARTESIAN_POINT ( 'NONE',  ( -2.500000000000000444, 20.83333333333333215, -4.330127018922193649 ) ) ;
#56507=CARTESIAN_POINT ( 'NONE',  ( -3.152548672688508926E-16, -76.56249999863440792, -5.148502694627439702 ) ) ;
#56508=CARTESIAN_POINT ( 'NONE',  ( -4.458734124999999437, 26.68750000136559564, 0.000000000000000000 ) ) ;
#56509=LINE ( 'NONE', #11783, #948 ) ;
#56510=ORIENTED_EDGE ( 'NONE', *, *, #55822, .F. ) ;
#56511=CYLINDRICAL_SURFACE ( 'NONE', #34596, 5.000000000000000000 ) ;
#56515=CARTESIAN_POINT ( 'NONE',  ( 1.339745962155612702, -74.16965819600731891, -5.000000000000000000 ) ) ;
#56516=CARTESIAN_POINT ( 'NONE',  ( -4.769696007084728073, -114.9999999999999858, 1.499999999999999556 ) ) ;
#56518=CARTESIAN_POINT ( 'NONE',  ( 2.229367062500001939, -54.97916666530107221, 3.861377020970579999 ) ) ;
#56521=( BOUNDED_CURVE ( )  B_SPLINE_CURVE ( 2, ( #33759, #37972, #28614, #53063, #44029, #48230, #62734, #39523, #19275 ),
 .UNSPECIFIED., .F., .F. ) 
 B_SPLINE_CURVE_WITH_KNOTS ( ( 3, 2, 2, 2, 3 ),
 ( 0.5303571428571428603, 0.5309523809523809534, 0.5321428571428571397, 0.5333333333333333259, 0.5339285714285714191 ),
 .UNSPECIFIED. ) 
 CURVE ( )  GEOMETRIC_REPRESENTATION_ITEM ( )  RATIONAL_B_SPLINE_CURVE ( ( 0.9330127018922194093, 0.9330127018922194093, 1.000000000000000000, 0.8660254037844387076, 1.000000000000000000, 0.8660254037844387076, 1.000000000000000000, 0.9330127018922194093, 0.9330127018922194093 ) ) 
 REPRESENTATION_ITEM ( '' )  );
#56522=CARTESIAN_POINT ( 'NONE',  ( -5.000000000000000000, -104.0833333333333428, -2.886751345948128211 ) ) ;
#56524=CARTESIAN_POINT ( 'NONE',  ( 4.458734124999999437, -41.06249999863440081, -5.460374474430324690E-16 ) ) ;
#56525=CARTESIAN_POINT ( 'NONE',  ( -4.999999999999999112, -0.7916666639354794643, 2.886751345948131764 ) ) ;
#56526=CARTESIAN_POINT ( 'NONE',  ( -6.972266317189433020E-16, -95.12499999726880162, -5.000000000000000000 ) ) ;
#56529=CARTESIAN_POINT ( 'NONE',  ( 2.500000000000002220, 24.33333333333333215, 4.330127018922192761 ) ) ;
#56530=CARTESIAN_POINT ( 'NONE',  ( 2.229367062499998831, -101.6458333319677365, -3.861377020970580887 ) ) ;
#56531=CARTESIAN_POINT ( 'NONE',  ( 9.457646018065525792E-16, -8.312499998634406140, 5.148502694627439702 ) ) ;
#56534=CARTESIAN_POINT ( 'NONE',  ( 4.458734124999999437, -92.81249999863440792, -5.460374474430324690E-16 ) ) ;
#56536=CARTESIAN_POINT ( 'NONE',  ( -3.152548672688508926E-16, -86.81249999863439371, -5.148502694627439702 ) ) ;
#56539=CARTESIAN_POINT ( 'NONE',  ( 6.123233995736766282E-16, -120.0000000000000000, -5.000000000000000000 ) ) ;
#56541=( BOUNDED_CURVE ( )  B_SPLINE_CURVE ( 2, ( #61225, #37713, #56716, #47055, #51260, #46732, #12634, #57034, #52519 ),
 .UNSPECIFIED., .F., .F. ) 
 B_SPLINE_CURVE_WITH_KNOTS ( ( 3, 2, 2, 2, 3 ),
 ( 0.6410714285714286254, 0.6416666666666667185, 0.6428571428571429047, 0.6440476190476190910, 0.6446428571428571841 ),
 .UNSPECIFIED. ) 
 CURVE ( )  GEOMETRIC_REPRESENTATION_ITEM ( )  RATIONAL_B_SPLINE_CURVE ( ( 0.9330127018922194093, 0.9330127018922256266, 1.000000000000000000, 0.8660254037844387076, 1.000000000000000000, 0.8660254037844387076, 1.000000000000000000, 0.9330127018922194093, 0.9330127018922194093 ) ) 
 REPRESENTATION_ITEM ( '' )  );
#56542=CARTESIAN_POINT ( 'NONE',  ( 2.229367062500001939, -8.979166665301075767, 3.861377020970579999 ) ) ;
#56543=CARTESIAN_POINT ( 'NONE',  ( 4.458734125000001214, 18.85416666803226349, 2.574251347313718519 ) ) ;
#56544=CARTESIAN_POINT ( 'NONE',  ( -4.458734124999999437, -54.56249999863440081, 0.000000000000000000 ) ) ;
#56545=CARTESIAN_POINT ( 'NONE',  ( -2.500000000000000444, 16.95833333606451987, -4.330127018922193649 ) ) ;
#56548=ORIENTED_EDGE ( 'NONE', *, *, #16412, .F. ) ;
#56552=CARTESIAN_POINT ( 'NONE',  ( 4.458734124999999437, -80.81249999863440792, -5.460374474430324690E-16 ) ) ;
#56553=CARTESIAN_POINT ( 'NONE',  ( 4.458734124999999437, 23.93750000136559564, -5.460374474430324690E-16 ) ) ;
#56556=DIRECTION ( 'NONE',  ( 0.000000000000000000, 0.000000000000000000, 1.000000000000000000 ) ) ;
#56558=CARTESIAN_POINT ( 'NONE',  ( 1.060575238724906964E-15, -64.75000000000000000, 5.773502691896257311 ) ) ;
#56561=ORIENTED_EDGE ( 'NONE', *, *, #59400, .T. ) ;
#56562=CARTESIAN_POINT ( 'NONE',  ( -2.499999999999996447, -61.70833333060214443, 4.330127018922195425 ) ) ;
#56571=CARTESIAN_POINT ( 'NONE',  ( 1.339745962155615144, -28.70534180126147561, 4.999999999999999112 ) ) ;
#56577=CARTESIAN_POINT ( 'NONE',  ( -3.152548672688508926E-16, -51.81249999863440792, -5.148502694627439702 ) ) ;
#56589=CARTESIAN_POINT ( 'NONE',  ( -4.458734124999999437, -97.64583333196772230, -2.574251347313719407 ) ) ;
#56595=ADVANCED_FACE ( 'NONE', ( #29664 ), #40282, .T. ) ;
#56597=CARTESIAN_POINT ( 'NONE',  ( -4.458734124999999437, -8.312499998634406140, 0.000000000000000000 ) ) ;
#56598=CARTESIAN_POINT ( 'NONE',  ( 4.458734124999998549, -97.97916666530105090, -2.574251347313721627 ) ) ;
#56600=CARTESIAN_POINT ( 'NONE',  ( -2.229367062499996610, -24.39583333196773651, 3.861377020970582219 ) ) ;
#56601=EDGE_CURVE ( 'NONE', #38122, #38750, #26937, .T. ) ;
#56602=CARTESIAN_POINT ( 'NONE',  ( 1.339745962155615144, -46.70534180126147561, 4.999999999999999112 ) ) ;
#56608=CARTESIAN_POINT ( 'NONE',  ( -2.229367062500000163, 10.27083333469892779, -3.861377020970580443 ) ) ;
#56610=CARTESIAN_POINT ( 'NONE',  ( -4.999999999999998224, -52.79166666393548013, 2.886751345948131764 ) ) ;
#56611=CARTESIAN_POINT ( 'NONE',  ( 1.339745962155615144, -61.70534180126146850, 4.999999999999999112 ) ) ;
#56612=CARTESIAN_POINT ( 'NONE',  ( 1.060575238724906964E-15, -91.75000000000000000, 5.773502691896257311 ) ) ;
#56613=CARTESIAN_POINT ( 'NONE',  ( -4.458734124999999437, -23.39583333196773296, -2.574251347313719407 ) ) ;
#56615=CARTESIAN_POINT ( 'NONE',  ( -4.458734124999998549, -68.47916666530106511, 2.574251347313722516 ) ) ;
#56616=CARTESIAN_POINT ( 'NONE',  ( 6.123233995736766282E-16, -120.0000000000000000, -5.000000000000000000 ) ) ;
#56619=CARTESIAN_POINT ( 'NONE',  ( -4.999999999999999112, -51.79166666393548013, 2.886751345948131764 ) ) ;
#56620=CARTESIAN_POINT ( 'NONE',  ( 5.000000000000000000, -24.50000000000000000, -6.123233995736766282E-16 ) ) ;
#56621=CARTESIAN_POINT ( 'NONE',  ( 4.458734125000000326, 8.104166668032261711, 2.574251347313718519 ) ) ;
#56622=CARTESIAN_POINT ( 'NONE',  ( -6.972266317189433020E-16, -89.24999999999998579, -5.000000000000000000 ) ) ;
#56623=CARTESIAN_POINT ( 'NONE',  ( 0.000000000000000000, -120.0000000000000000, 0.000000000000000000 ) ) ;
#56625=CARTESIAN_POINT ( 'NONE',  ( 4.458734125000001214, -73.89583333196773651, 2.574251347313718519 ) ) ;
#56627=( BOUNDED_CURVE ( )  B_SPLINE_CURVE ( 2, ( #62499, #18417, #12642, #51266, #57670, #3012, #32257, #51887, #7828 ),
 .UNSPECIFIED., .F., .F. ) 
 B_SPLINE_CURVE_WITH_KNOTS ( ( 3, 2, 2, 2, 3 ),
 ( 0.4946428571428571619, 0.4952380952380952550, 0.4964285714285714413, 0.4976190476190476275, 0.4982142857142857206 ),
 .UNSPECIFIED. ) 
 CURVE ( )  GEOMETRIC_REPRESENTATION_ITEM ( )  RATIONAL_B_SPLINE_CURVE ( ( 0.9330127018922194093, 0.9330127018922194093, 1.000000000000000000, 0.8660254037844387076, 1.000000000000000000, 0.8660254037844387076, 1.000000000000000000, 0.9330127018922194093, 0.9330127018922194093 ) ) 
 REPRESENTATION_ITEM ( '' )  );
#56628=CARTESIAN_POINT ( 'NONE',  ( 5.000000000000000888, -1.583333333333332593, 2.886751345948126879 ) ) ;
#56631=CARTESIAN_POINT ( 'NONE',  ( -2.229367062499996610, -66.14583333196773651, 3.861377020970582219 ) ) ;
#56632=CARTESIAN_POINT ( 'NONE',  ( 5.000000000000000000, -99.29166666393545881, -2.886751345948129988 ) ) ;
#56633=CARTESIAN_POINT ( 'NONE',  ( 0.000000000000000000, -120.0000000000000000, 5.000000000000000000 ) ) ;
#56638=CARTESIAN_POINT ( 'NONE',  ( -3.535250795749689387E-16, -47.25000000000000000, -5.773502691896257311 ) ) ;
#56639=CARTESIAN_POINT ( 'NONE',  ( -2.499999999999996447, 27.16666666666666430, 4.330127018922195425 ) ) ;
#56640=PLANE ( 'NONE',  #47923 ) ;
#56642=CARTESIAN_POINT ( 'NONE',  ( 1.339745962155612702, -94.29465819873851729, -5.000000000000000000 ) ) ;
#56643=CARTESIAN_POINT ( 'NONE',  ( -6.972266317189433020E-16, 11.74999999999999645, -5.000000000000000000 ) ) ;
#56652=VERTEX_POINT ( 'NONE', #51532 ) ;
#56655=CARTESIAN_POINT ( 'NONE',  ( -2.229367062499996610, -35.39583333196772941, 3.861377020970582219 ) ) ;
#56666=CARTESIAN_POINT ( 'NONE',  ( -3.152548672688508926E-16, -82.81249999863442213, -5.148502694627439702 ) ) ;
#56672=CARTESIAN_POINT ( 'NONE',  ( -4.458734124999997661, -36.22916666530106511, 2.574251347313722516 ) ) ;
#56673=CARTESIAN_POINT ( 'NONE',  ( -2.229367062499996610, -7.395833331967735624, 3.861377020970582219 ) ) ;
#56678=CARTESIAN_POINT ( 'NONE',  ( -4.458734124999999437, -6.645833331967741842, -2.574251347313719407 ) ) ;
#56684=CARTESIAN_POINT ( 'NONE',  ( -4.458734124999999437, 28.35416666803225993, -2.574251347313719407 ) ) ;
#56685=VERTEX_POINT ( 'NONE', #61507 ) ;
#56686=CARTESIAN_POINT ( 'NONE',  ( -4.458734124999999437, -87.39583333196773651, -2.574251347313719407 ) ) ;
#56688=CARTESIAN_POINT ( 'NONE',  ( -4.458734124999999437, -9.395833331967736513, -2.574251347313719407 ) ) ;
#56689=CARTESIAN_POINT ( 'NONE',  ( 0.000000000000000000, -120.0000000000000000, 5.000000000000000000 ) ) ;
#56690=DIRECTION ( 'NONE',  ( -0.000000000000000000, 1.000000000000000000, -0.000000000000000000 ) ) ;
#56692=CARTESIAN_POINT ( 'NONE',  ( -2.500000000000000444, -36.04166666393547303, -4.330127018922193649 ) ) ;
#56693=LINE ( 'NONE', #60878, #55042 ) ;
#56694=CARTESIAN_POINT ( 'NONE',  ( -4.458734124999997661, 26.77083333469892779, 2.574251347313722516 ) ) ;
#56695=CARTESIAN_POINT ( 'NONE',  ( -4.999999999999998224, -20.79166666393548013, 2.886751345948131764 ) ) ;
#56697=CARTESIAN_POINT ( 'NONE',  ( -4.458734124999998549, -58.22916666530105800, 2.574251347313722516 ) ) ;
#56700=CARTESIAN_POINT ( 'NONE',  ( -2.500000000000000444, 15.83333333333333037, -4.330127018922193649 ) ) ;
#56702=CARTESIAN_POINT ( 'NONE',  ( 2.229367062500001939, -48.97916666530107221, 3.861377020970579999 ) ) ;
#56703=CARTESIAN_POINT ( 'NONE',  ( 5.000000000000000000, -81.37499999726881583, -6.123233995736766282E-16 ) ) ;
#56706=CARTESIAN_POINT ( 'NONE',  ( 2.229367062500001939, -88.22916666530107932, 3.861377020970579999 ) ) ;
#56708=CARTESIAN_POINT ( 'NONE',  ( 5.000000000000000000, -33.50000000000000000, -6.123233995736766282E-16 ) ) ;
#56710=EDGE_LOOP ( 'NONE', ( #8376, #15440, #3458, #55388 ) ) ;
#56712=ORIENTED_EDGE ( 'NONE', *, *, #3219, .F. ) ;
#56713=CARTESIAN_POINT ( 'NONE',  ( 4.458734125000001214, -95.89583333196773651, 2.574251347313718519 ) ) ;
#56714=CARTESIAN_POINT ( 'NONE',  ( -2.229367062500000163, 15.27083333469892779, -3.861377020970580443 ) ) ;
#56715=CARTESIAN_POINT ( 'NONE',  ( -4.999999999999999112, 15.20833333606451987, 2.886751345948131764 ) ) ;
#56716=CARTESIAN_POINT ( 'NONE',  ( -2.499999999999996447, -59.83333333333333570, 4.330127018922195425 ) ) ;
#56719=( BOUNDED_CURVE ( )  B_SPLINE_CURVE ( 2, ( #9672, #1570, #24476, #9993, #29606, #46, #32718, #32078, #37542 ),
 .UNSPECIFIED., .F., .F. ) 
 B_SPLINE_CURVE_WITH_KNOTS ( ( 3, 2, 2, 2, 3 ),
 ( 0.9875000000000000444, 0.9880952380952381375, 0.9892857142857143238, 0.9904761904761905100, 0.9910714285714286031 ),
 .UNSPECIFIED. ) 
 CURVE ( )  GEOMETRIC_REPRESENTATION_ITEM ( )  RATIONAL_B_SPLINE_CURVE ( ( 0.9330127018922194093, 0.9330127018922194093, 1.000000000000000000, 0.8660254037844387076, 1.000000000000000000, 0.8660254037844387076, 1.000000000000000000, 0.9330127018922194093, 0.9330127018922194093 ) ) 
 REPRESENTATION_ITEM ( '' )  );
#56721=CARTESIAN_POINT ( 'NONE',  ( 1.060575238724906964E-15, -81.75000000000000000, 5.773502691896257311 ) ) ;
#56723=FACE_OUTER_BOUND ( 'NONE', #11717, .T. ) ;
#56724=CARTESIAN_POINT ( 'NONE',  ( -1.339745962155613812, -26.08034179853029499, -5.000000000000000000 ) ) ;
#56725=CARTESIAN_POINT ( 'NONE',  ( 5.000000000000000000, -109.4999999999999858, -6.123233995736766282E-16 ) ) ;
#56729=CARTESIAN_POINT ( 'NONE',  ( 2.229367062499998831, -17.89583333196773651, -3.861377020970580887 ) ) ;
#56737=EDGE_CURVE ( 'NONE', #60194, #61583, #18288, .T. ) ;
#56739=CARTESIAN_POINT ( 'NONE',  ( 1.975475456537005874E-15, -46.74999999999999289, 5.000000000000000000 ) ) ;
#56741=CARTESIAN_POINT ( 'NONE',  ( 2.229367062499998831, -66.89583333196773651, -3.861377020970580887 ) ) ;
#56744=EDGE_LOOP ( 'NONE', ( #16233, #19169, #13026, #30846 ) ) ;
#56751=CARTESIAN_POINT ( 'NONE',  ( 9.457646018065525792E-16, 5.937500001365592972, 5.148502694627439702 ) ) ;
#56759=CARTESIAN_POINT ( 'NONE',  ( 9.457646018065525792E-16, -72.06249999863439371, 5.148502694627439702 ) ) ;
#56760=CARTESIAN_POINT ( 'NONE',  ( 5.000000000000000000, -10.37499999726881583, -6.123233995736766282E-16 ) ) ;
#56761=CARTESIAN_POINT ( 'NONE',  ( 4.458734125000001214, 8.104166668032261711, 2.574251347313718519 ) ) ;
#56764=CARTESIAN_POINT ( 'NONE',  ( 4.458734125000001214, -61.14583333196773651, 2.574251347313718519 ) ) ;
#56765=CARTESIAN_POINT ( 'NONE',  ( 2.499999999999998668, -14.20833333060214976, -4.330127018922193649 ) ) ;
#56768=CARTESIAN_POINT ( 'NONE',  ( 2.500000000000002220, -30.54166666393548013, 4.330127018922192761 ) ) ;
#56770=CARTESIAN_POINT ( 'NONE',  ( -4.999999999999998224, -83.79166666393545881, 2.886751345948131764 ) ) ;
#56771=CARTESIAN_POINT ( 'NONE',  ( 2.229367062499998831, -35.64583333196772941, -3.861377020970580887 ) ) ;
#56772=CARTESIAN_POINT ( 'NONE',  ( -4.458734124999999437, -21.64583333196774007, -2.574251347313719407 ) ) ;
#56773=( BOUNDED_CURVE ( )  B_SPLINE_CURVE ( 2, ( #3413, #7920, #47154, #32991, #32356, #3101, #23958, #4039, #28781 ),
 .UNSPECIFIED., .F., .F. ) 
 B_SPLINE_CURVE_WITH_KNOTS ( ( 3, 2, 2, 2, 3 ),
 ( 0.2982142857142857095, 0.2988095238095238027, 0.2999999999999999889, 0.3011904761904761751, 0.3017857142857142683 ),
 .UNSPECIFIED. ) 
 CURVE ( )  GEOMETRIC_REPRESENTATION_ITEM ( )  RATIONAL_B_SPLINE_CURVE ( ( 0.9330127018922194093, 0.9330127018922194093, 1.000000000000000000, 0.8660254037844387076, 1.000000000000000000, 0.8660254037844387076, 1.000000000000000000, 0.9330127018922194093, 0.9330127018922194093 ) ) 
 REPRESENTATION_ITEM ( '' )  );
#56776=CARTESIAN_POINT ( 'NONE',  ( -3.535250795749689387E-16, 28.74999999999999645, -5.773502691896257311 ) ) ;
#56779=CARTESIAN_POINT ( 'NONE',  ( -2.229367062499996610, -105.3958333319677365, 3.861377020970582219 ) ) ;
#56780=CARTESIAN_POINT ( 'NONE',  ( 4.458734124999998549, -33.72916666530106511, -2.574251347313721627 ) ) ;
#56781=CARTESIAN_POINT ( 'NONE',  ( 2.500000000000002220, -63.54166666393547303, 4.330127018922192761 ) ) ;
#56784=CARTESIAN_POINT ( 'NONE',  ( 2.229367062499998831, -29.64583333196773296, -3.861377020970580887 ) ) ;
#56785=CARTESIAN_POINT ( 'NONE',  ( -4.458734124999999437, -68.64583333196773651, -2.574251347313719407 ) ) ;
#56786=DIRECTION ( 'NONE',  ( -0.000000000000000000, 1.000000000000000000, -0.000000000000000000 ) ) ;
#56790=CARTESIAN_POINT ( 'NONE',  ( -5.000000000000000000, -18.08333333333333570, -2.886751345948128211 ) ) ;
#56792=EDGE_LOOP ( 'NONE', ( #48232, #60680, #680, #23990 ) ) ;
#56796=DIRECTION ( 'NONE',  ( 0.000000000000000000, 0.000000000000000000, 1.000000000000000000 ) ) ;
#56798=CARTESIAN_POINT ( 'NONE',  ( 2.499999999999998668, 25.66666666666666430, -4.330127018922193649 ) ) ;
#56800=CARTESIAN_POINT ( 'NONE',  ( -2.499999999999996447, -51.70833333060213732, 4.330127018922195425 ) ) ;
#56804=( BOUNDED_CURVE ( )  B_SPLINE_CURVE ( 2, ( #5275, #24253, #18786, #29063, #460, #9147, #24896, #19427, #38717 ),
 .UNSPECIFIED., .F., .F. ) 
 B_SPLINE_CURVE_WITH_KNOTS ( ( 3, 2, 2, 2, 3 ),
 ( 0.5517857142857143238, 0.5523809523809524169, 0.5535714285714286031, 0.5547619047619047894, 0.5553571428571428825 ),
 .UNSPECIFIED. ) 
 CURVE ( )  GEOMETRIC_REPRESENTATION_ITEM ( )  RATIONAL_B_SPLINE_CURVE ( ( 0.9330127018922194093, 0.9330127018922194093, 1.000000000000000000, 0.8660254037844387076, 1.000000000000000000, 0.8660254037844387076, 1.000000000000000000, 0.9330127018922194093, 0.9330127018922194093 ) ) 
 REPRESENTATION_ITEM ( '' )  );
#56814=ORIENTED_EDGE ( 'NONE', *, *, #14087, .T. ) ;
#56817=( BOUNDED_CURVE ( )  B_SPLINE_CURVE ( 2, ( #62284, #17888, #57148, #57461, #46846, #27849, #42327, #7621, #52314 ),
 .UNSPECIFIED., .F., .F. ) 
 B_SPLINE_CURVE_WITH_KNOTS ( ( 3, 2, 2, 2, 3 ),
 ( 0.1089285714285714302, 0.1095238095238095233, 0.1107142857142857095, 0.1119047619047619097, 0.1125000000000000028 ),
 .UNSPECIFIED. ) 
 CURVE ( )  GEOMETRIC_REPRESENTATION_ITEM ( )  RATIONAL_B_SPLINE_CURVE ( ( 0.9330127018922194093, 0.9330127018922194093, 1.000000000000000000, 0.8660254037844387076, 1.000000000000000000, 0.8660254037844387076, 1.000000000000000000, 0.9330127018922194093, 0.9330127018922194093 ) ) 
 REPRESENTATION_ITEM ( '' )  );
#56822=ORIENTED_EDGE ( 'NONE', *, *, #5436, .F. ) ;
#56823=CARTESIAN_POINT ( 'NONE',  ( -2.229367062500000163, -80.47916666530106511, -3.861377020970580443 ) ) ;
#56824=VECTOR ( 'NONE', #50359, 1000.000000000000000 ) ;
#56825=CARTESIAN_POINT ( 'NONE',  ( -4.458734124999999437, 24.60416666803225993, -2.574251347313719407 ) ) ;
#56827=ORIENTED_EDGE ( 'NONE', *, *, #2863, .F. ) ;
#56832=CARTESIAN_POINT ( 'NONE',  ( 1.975475456537005874E-15, -85.75000000000000000, 5.000000000000000000 ) ) ;
#56835=CARTESIAN_POINT ( 'NONE',  ( -4.458734124999999437, -52.31249999863440792, 0.000000000000000000 ) ) ;
#56838=CARTESIAN_POINT ( 'NONE',  ( -5.000000000000000000, -106.0833333333333286, -2.886751345948128211 ) ) ;
#56840=CARTESIAN_POINT ( 'NONE',  ( -3.152548672688508926E-16, -43.81249999863440081, -5.148502694627439702 ) ) ;
#56841=CARTESIAN_POINT ( 'NONE',  ( -3.535250795749689387E-16, -1.124999997268814056, -5.773502691896257311 ) ) ;
#56843=DIRECTION ( 'NONE',  ( -0.000000000000000000, 1.000000000000000000, -0.000000000000000000 ) ) ;
#56845=CARTESIAN_POINT ( 'NONE',  ( 4.458734124999999437, -101.8124999986344079, -5.460374474430324690E-16 ) ) ;
#56846=CARTESIAN_POINT ( 'NONE',  ( -4.458734124999997661, -6.479166665301072214, 2.574251347313722516 ) ) ;
#56848=CARTESIAN_POINT ( 'NONE',  ( -5.000000000000000000, -35.95833333060213732, -2.886751345948128211 ) ) ;
#56849=CARTESIAN_POINT ( 'NONE',  ( -4.458734124999999437, -91.39583333196773651, -2.574251347313719407 ) ) ;
#56851=CARTESIAN_POINT ( 'NONE',  ( 4.458734124999998549, -84.97916666530106511, -2.574251347313721627 ) ) ;
#56855=CARTESIAN_POINT ( 'NONE',  ( 4.458734124999999437, -13.81249999863440259, -5.460374474430324690E-16 ) ) ;
#56856=CARTESIAN_POINT ( 'NONE',  ( -4.458734124999999437, 16.43750000136559564, 0.000000000000000000 ) ) ;
#56857=CARTESIAN_POINT ( 'NONE',  ( -4.458734124999999437, -51.64583333196773651, -2.574251347313719407 ) ) ;
#56859=CARTESIAN_POINT ( 'NONE',  ( -2.500000000000000444, -106.1666666666666572, -4.330127018922193649 ) ) ;
#56861=CARTESIAN_POINT ( 'NONE',  ( -1.339745962155610925, -38.79465819873851729, 5.000000000000000000 ) ) ;
#56862=ORIENTED_EDGE ( 'NONE', *, *, #48453, .T. ) ;
#56865=CARTESIAN_POINT ( 'NONE',  ( 5.000000000000000000, -76.50000000000000000, -6.123233995736766282E-16 ) ) ;
#56866=CARTESIAN_POINT ( 'NONE',  ( -4.458734124999999437, -79.39583333196773651, -2.574251347313719407 ) ) ;
#56867=CARTESIAN_POINT ( 'NONE',  ( -3.152548672688508926E-16, 22.18750000136559564, -5.148502694627439702 ) ) ;
#56869=VECTOR ( 'NONE', #2957, 1000.000000000000000 ) ;
#56874=CARTESIAN_POINT ( 'NONE',  ( 2.499999999999998668, -65.33333333333332860, -4.330127018922193649 ) ) ;
#56875=CARTESIAN_POINT ( 'NONE',  ( -2.500000000000000444, 29.83333333333333215, -4.330127018922193649 ) ) ;
#56877=ORIENTED_EDGE ( 'NONE', *, *, #24758, .F. ) ;
#56883=CARTESIAN_POINT ( 'NONE',  ( 2.500000000000002220, -62.66666666666666430, 4.330127018922192761 ) ) ;
#56886=ORIENTED_EDGE ( 'NONE', *, *, #17311, .T. ) ;
#56889=ORIENTED_EDGE ( 'NONE', *, *, #29529, .T. ) ;
#56892=CARTESIAN_POINT ( 'NONE',  ( 4.458734124999998549, -50.97916666530107221, -2.574251347313721627 ) ) ;
#56894=CARTESIAN_POINT ( 'NONE',  ( -5.000000000000000000, -54.95833333060214443, -2.886751345948128211 ) ) ;
#56899=( BOUNDED_CURVE ( )  B_SPLINE_CURVE ( 2, ( #9461, #24581, #48694, #4635, #24259, #43862, #63509, #30991, #45150 ),
 .UNSPECIFIED., .F., .F. ) 
 B_SPLINE_CURVE_WITH_KNOTS ( ( 3, 2, 2, 2, 3 ),
 ( 0.8446428571428571397, 0.8452380952380952328, 0.8464285714285714191, 0.8476190476190476053, 0.8482142857142856984 ),
 .UNSPECIFIED. ) 
 CURVE ( )  GEOMETRIC_REPRESENTATION_ITEM ( )  RATIONAL_B_SPLINE_CURVE ( ( 0.9330127018922194093, 0.9330127018922194093, 1.000000000000000000, 0.8660254037844387076, 1.000000000000000000, 0.8660254037844387076, 1.000000000000000000, 0.9330127018922194093, 0.9330127018922194093 ) ) 
 REPRESENTATION_ITEM ( '' )  );
#56903=CARTESIAN_POINT ( 'NONE',  ( -4.458734124999999437, -100.5624999986344079, 0.000000000000000000 ) ) ;
#56905=VERTEX_POINT ( 'NONE', #21628 ) ;
#56909=CARTESIAN_POINT ( 'NONE',  ( -4.458734124999999437, -9.312499998634406140, 0.000000000000000000 ) ) ;
#56910=CARTESIAN_POINT ( 'NONE',  ( 2.229367062499998831, -94.89583333196773651, -3.861377020970580887 ) ) ;
#56911=( BOUNDED_CURVE ( )  B_SPLINE_CURVE ( 2, ( #958, #15085, #34699, #10261, #25372, #20558, #40161, #54962, #10892 ),
 .UNSPECIFIED., .F., .F. ) 
 B_SPLINE_CURVE_WITH_KNOTS ( ( 3, 2, 2, 2, 3 ),
 ( 0.9196428571428570953, 0.9202380952380951884, 0.9214285714285713746, 0.9226190476190476719, 0.9232142857142857650 ),
 .UNSPECIFIED. ) 
 CURVE ( )  GEOMETRIC_REPRESENTATION_ITEM ( )  RATIONAL_B_SPLINE_CURVE ( ( 0.9330127018922194093, 0.9330127018922194093, 1.000000000000000000, 0.8660254037844387076, 1.000000000000000000, 0.8660254037844387076, 1.000000000000000000, 0.9330127018922194093, 0.9330127018922194093 ) ) 
 REPRESENTATION_ITEM ( '' )  );
#56913=CARTESIAN_POINT ( 'NONE',  ( -4.458734124999999437, -22.56249999863440436, 0.000000000000000000 ) ) ;
#56918=CARTESIAN_POINT ( 'NONE',  ( 0.000000000000000000, -120.0000000000000000, 0.000000000000000000 ) ) ;
#56920=CARTESIAN_POINT ( 'NONE',  ( 4.458734124999999437, 8.937500001365592084, -5.460374474430324690E-16 ) ) ;
#56921=ORIENTED_EDGE ( 'NONE', *, *, #30283, .F. ) ;
#56923=CARTESIAN_POINT ( 'NONE',  ( 1.339745962155615144, -66.58034179853028434, 4.999999999999999112 ) ) ;
#56924=CARTESIAN_POINT ( 'NONE',  ( -5.000000000000000000, -89.08333333333334281, -2.886751345948128211 ) ) ;
#56925=CARTESIAN_POINT ( 'NONE',  ( 4.458734124999998549, -22.72916666530107221, -2.574251347313721627 ) ) ;
#56926=CARTESIAN_POINT ( 'NONE',  ( -5.000000000000000000, -76.87499999726880162, 0.000000000000000000 ) ) ;
#56927=CARTESIAN_POINT ( 'NONE',  ( -3.152548672688508926E-16, -70.81249999863440792, -5.148502694627439702 ) ) ;
#56931=CARTESIAN_POINT ( 'NONE',  ( 2.229367062499998831, 3.354166668032259935, -3.861377020970580887 ) ) ;
#56932=DIRECTION ( 'NONE',  ( -0.000000000000000000, 1.000000000000000000, -0.000000000000000000 ) ) ;
#56935=CARTESIAN_POINT ( 'NONE',  ( 2.229367062499998831, -73.64583333196773651, -3.861377020970580887 ) ) ;
#56937=CARTESIAN_POINT ( 'NONE',  ( -2.499999999999996447, -2.833333333333333481, 4.330127018922195425 ) ) ;
#56940=CARTESIAN_POINT ( 'NONE',  ( -4.458734124999999437, -62.39583333196774362, -2.574251347313719407 ) ) ;
#56941=CARTESIAN_POINT ( 'NONE',  ( 1.060575238724906964E-15, -98.62499999726883004, 5.773502691896257311 ) ) ;
#56942=EDGE_CURVE ( 'NONE', #48295, #42800, #33868, .T. ) ;
#56945=CARTESIAN_POINT ( 'NONE',  ( 4.458734125000000326, -105.1458333319677365, 2.574251347313718519 ) ) ;
#56947=CARTESIAN_POINT ( 'NONE',  ( 5.000000000000000000, -50.41666666666666430, -2.886751345948129988 ) ) ;
#56950=ORIENTED_EDGE ( 'NONE', *, *, #18815, .T. ) ;
#56951=CARTESIAN_POINT ( 'NONE',  ( 2.500000000000002220, -94.66666666666665719, 4.330127018922192761 ) ) ;
#56952=CARTESIAN_POINT ( 'NONE',  ( -1.339745962155610925, -99.66965819600733312, 5.000000000000000000 ) ) ;
#56956=VECTOR ( 'NONE', #32178, 1000.000000000000000 ) ;
#56961=CARTESIAN_POINT ( 'NONE',  ( 5.000000000000000888, -100.4583333306021444, 2.886751345948126879 ) ) ;
#56968=CARTESIAN_POINT ( 'NONE',  ( -4.458734124999999437, -37.64583333196773651, -2.574251347313719407 ) ) ;
#56969=DIRECTION ( 'NONE',  ( -0.000000000000000000, 1.000000000000000000, -0.000000000000000000 ) ) ;
#56976=EDGE_CURVE ( 'NONE', #26112, #52286, #55688, .T. ) ;
#56978=CARTESIAN_POINT ( 'NONE',  ( -2.229367062500000163, -83.72916666530106511, -3.861377020970580443 ) ) ;
#56980=ORIENTED_EDGE ( 'NONE', *, *, #22183, .F. ) ;
#56981=CARTESIAN_POINT ( 'NONE',  ( -1.339745962155610925, -94.66965819600731891, 5.000000000000000000 ) ) ;
#56984=CARTESIAN_POINT ( 'NONE',  ( -3.152548672688508926E-16, -39.56249999863440081, -5.148502694627439702 ) ) ;
#56985=CARTESIAN_POINT ( 'NONE',  ( 2.229367062500001939, -8.229166665301073991, 3.861377020970579999 ) ) ;
#56986=ORIENTED_EDGE ( 'NONE', *, *, #53403, .T. ) ;
#56988=CARTESIAN_POINT ( 'NONE',  ( -2.500000000000000444, -2.166666666666663854, -4.330127018922193649 ) ) ;
#56990=CARTESIAN_POINT ( 'NONE',  ( 4.458734124999999437, -6.062499998634403475, -5.460374474430324690E-16 ) ) ;
#56991=CYLINDRICAL_SURFACE ( 'NONE', #27105, 5.000000000000000000 ) ;
#56995=( BOUNDED_CURVE ( )  B_SPLINE_CURVE ( 2, ( #56437, #26518, #46134, #61257, #15911, #36807, #16236, #60307, #11079 ),
 .UNSPECIFIED., .F., .F. ) 
 B_SPLINE_CURVE_WITH_KNOTS ( ( 3, 2, 2, 2, 3 ),
 ( 0.9910714285714286031, 0.9916666666666666963, 0.9928571428571428825, 0.9940476190476190688, 0.9946428571428571619 ),
 .UNSPECIFIED. ) 
 CURVE ( )  GEOMETRIC_REPRESENTATION_ITEM ( )  RATIONAL_B_SPLINE_CURVE ( ( 0.9330127018922194093, 0.9330127018922194093, 1.000000000000000000, 0.8660254037844387076, 1.000000000000000000, 0.8660254037844387076, 1.000000000000000000, 0.9330127018922194093, 0.9330127018922194093 ) ) 
 REPRESENTATION_ITEM ( '' )  );
#56996=CARTESIAN_POINT ( 'NONE',  ( 4.458734124999999437, 25.93750000136559564, -5.460374474430324690E-16 ) ) ;
#56997=ORIENTED_EDGE ( 'NONE', *, *, #23885, .F. ) ;
#56998=CARTESIAN_POINT ( 'NONE',  ( 4.458734125000000326, -88.89583333196773651, 2.574251347313718519 ) ) ;
#57000=CARTESIAN_POINT ( 'NONE',  ( -4.458734124999999437, -11.31249999863440792, 0.000000000000000000 ) ) ;
#57001=CYLINDRICAL_SURFACE ( 'NONE', #32378, 5.000000000000000000 ) ;
#57005=CARTESIAN_POINT ( 'NONE',  ( 5.000000000000000000, -37.37499999726881583, -6.123233995736766282E-16 ) ) ;
#57007=CARTESIAN_POINT ( 'NONE',  ( 4.458734124999998549, 26.27083333469892423, -2.574251347313721627 ) ) ;
#57008=CARTESIAN_POINT ( 'NONE',  ( -5.000000000000000000, -95.00000000000000000, 0.000000000000000000 ) ) ;
#57010=CARTESIAN_POINT ( 'NONE',  ( -4.458734124999998549, -56.22916666530107221, 2.574251347313722516 ) ) ;
#57012=CYLINDRICAL_SURFACE ( 'NONE', #9301, 5.000000000000000000 ) ;
#57013=CARTESIAN_POINT ( 'NONE',  ( -5.000000000000000000, 17.00000000000000000, 0.000000000000000000 ) ) ;
#57016=CARTESIAN_POINT ( 'NONE',  ( 9.457646018065525792E-16, -50.06249999863440792, 5.148502694627439702 ) ) ;
#57017=CARTESIAN_POINT ( 'NONE',  ( 2.499999999999998668, -85.20833333060214443, -4.330127018922193649 ) ) ;
#57020=CARTESIAN_POINT ( 'NONE',  ( 5.000000000000000000, -65.29166666393547303, -2.886751345948130876 ) ) ;
#57021=ADVANCED_FACE ( 'NONE', ( #12908 ), #53407, .T. ) ;
#57022=CARTESIAN_POINT ( 'NONE',  ( 1.975475456537005874E-15, -89.62499999726880162, 5.000000000000000000 ) ) ;
#57023=EDGE_CURVE ( 'NONE', #32043, #34883, #38011, .T. ) ;
#57024=CARTESIAN_POINT ( 'NONE',  ( -2.229367062500000163, -84.72916666530107932, -3.861377020970580443 ) ) ;
#57026=CARTESIAN_POINT ( 'NONE',  ( -4.999999999999999112, -31.91666666666666430, 2.886751345948131764 ) ) ;
#57030=ORIENTED_EDGE ( 'NONE', *, *, #21310, .F. ) ;
#57031=CARTESIAN_POINT ( 'NONE',  ( -4.458734124999999437, -97.31249999863440792, 0.000000000000000000 ) ) ;
#57032=CARTESIAN_POINT ( 'NONE',  ( 4.458734125000001214, 7.854166668032260823, 2.574251347313718519 ) ) ;
#57033=CARTESIAN_POINT ( 'NONE',  ( -5.000000000000000000, 12.12500000273118772, 0.000000000000000000 ) ) ;
#57034=CARTESIAN_POINT ( 'NONE',  ( -1.339745962155613812, -60.20534180126147561, -5.000000000000000000 ) ) ;
#57039=CARTESIAN_POINT ( 'NONE',  ( 2.500000000000002220, -80.66666666666665719, 4.330127018922192761 ) ) ;
#57043=CARTESIAN_POINT ( 'NONE',  ( 6.123233995736766282E-16, -120.0000000000000000, -5.000000000000000000 ) ) ;
#57044=EDGE_CURVE ( 'NONE', #62422, #44925, #1034, .T. ) ;
#57047=CARTESIAN_POINT ( 'NONE',  ( 5.000000000000000000, -107.4999999999999858, -6.123233995736766282E-16 ) ) ;
#57048=DIRECTION ( 'NONE',  ( 0.000000000000000000, 0.000000000000000000, 1.000000000000000000 ) ) ;
#57049=CARTESIAN_POINT ( 'NONE',  ( 4.458734124999999437, -22.06249999863440436, -5.460374474430324690E-16 ) ) ;
#57050=CARTESIAN_POINT ( 'NONE',  ( -1.339745962155610925, -57.79465819873852439, 5.000000000000000000 ) ) ;
#57061=CARTESIAN_POINT ( 'NONE',  ( -3.152548672688508926E-16, -65.81249999863440792, -5.148502694627439702 ) ) ;
#57069=CARTESIAN_POINT ( 'NONE',  ( -6.972266317189433020E-16, -88.12499999726880162, -5.000000000000000000 ) ) ;
#57070=CARTESIAN_POINT ( 'NONE',  ( -3.152548672688508926E-16, 7.437500001365594748, -5.148502694627439702 ) ) ;
#57076=CARTESIAN_POINT ( 'NONE',  ( -4.458734124999999437, -68.31249999863439371, 0.000000000000000000 ) ) ;
#57078=CARTESIAN_POINT ( 'NONE',  ( 4.458734124999999437, 7.187500001365594748, -5.460374474430324690E-16 ) ) ;
#57080=CARTESIAN_POINT ( 'NONE',  ( 2.229367062499998831, -61.89583333196774362, -3.861377020970580887 ) ) ;
#57081=CARTESIAN_POINT ( 'NONE',  ( -5.000000000000000000, -18.95833333060214443, -2.886751345948128211 ) ) ;
#57082=CARTESIAN_POINT ( 'NONE',  ( -1.339745962155555858, -19.20534180126148271, -5.000000000000032863 ) ) ;
#57084=CARTESIAN_POINT ( 'NONE',  ( -6.972266317189433020E-16, -84.12499999726880162, -5.000000000000000000 ) ) ;
#57085=CARTESIAN_POINT ( 'NONE',  ( 4.458734124999998549, -39.72916666530107932, -2.574251347313721627 ) ) ;
#57086=CARTESIAN_POINT ( 'NONE',  ( 4.458734125000000326, -19.14583333196774007, 2.574251347313718519 ) ) ;
#57088=CARTESIAN_POINT ( 'NONE',  ( -6.972266317189433020E-16, -102.2499999999999858, -5.000000000000000000 ) ) ;
#57089=CARTESIAN_POINT ( 'NONE',  ( 4.458734124999998549, -109.7291666653010793, -2.574251347313721627 ) ) ;
#57091=VERTEX_POINT ( 'NONE', #5156 ) ;
#57092=CARTESIAN_POINT ( 'NONE',  ( -4.458734124999999437, -109.5624999986343937, 0.000000000000000000 ) ) ;
#57093=CARTESIAN_POINT ( 'NONE',  ( -4.458734124999999437, -34.39583333196772941, -2.574251347313719407 ) ) ;
#57094=CARTESIAN_POINT ( 'NONE',  ( -5.000000000000000000, -65.87499999726881583, 0.000000000000000000 ) ) ;
#57098=EDGE_CURVE ( 'NONE', #15518, #62343, #44571, .T. ) ;
#57100=CARTESIAN_POINT ( 'NONE',  ( -2.229367062499996610, -27.14583333196774007, 3.861377020970582219 ) ) ;
#57101=CARTESIAN_POINT ( 'NONE',  ( 4.458734125000000326, -67.14583333196773651, 2.574251347313718519 ) ) ;
#57105=CARTESIAN_POINT ( 'NONE',  ( 1.339745962155612702, -32.29465819873852439, -5.000000000000000000 ) ) ;
#57106=CARTESIAN_POINT ( 'NONE',  ( 5.000000000000000000, -5.291666663935480130, -2.886751345948130876 ) ) ;
#57107=CARTESIAN_POINT ( 'NONE',  ( -3.535250795749689387E-16, -14.25000000000000178, -5.773502691896257311 ) ) ;
#57110=CARTESIAN_POINT ( 'NONE',  ( 6.123233995736766282E-16, -120.0000000000000000, -5.000000000000000000 ) ) ;
#57113=CARTESIAN_POINT ( 'NONE',  ( -4.999999999999998224, -0.9166666666666664076, 2.886751345948131764 ) ) ;
#57115=EDGE_CURVE ( 'NONE', #14315, #59250, #40205, .T. ) ;
#57117=CARTESIAN_POINT ( 'NONE',  ( 2.499999999999998668, -76.20833333060214443, -4.330127018922193649 ) ) ;
#57121=CARTESIAN_POINT ( 'NONE',  ( 5.000000000000000888, -87.45833333060214443, 2.886751345948126879 ) ) ;
#57123=EDGE_CURVE ( 'NONE', #61001, #21194, #19940, .T. ) ;
#57125=CARTESIAN_POINT ( 'NONE',  ( 0.000000000000000000, -120.0000000000000000, 0.000000000000000000 ) ) ;
#57126=VERTEX_POINT ( 'NONE', #10297 ) ;
#57129=EDGE_CURVE ( 'NONE', #44174, #39750, #56057, .T. ) ;
#57131=EDGE_CURVE ( 'NONE', #59301, #34883, #25, .T. ) ;
#57135=ORIENTED_EDGE ( 'NONE', *, *, #32539, .F. ) ;
#57136=CARTESIAN_POINT ( 'NONE',  ( -2.499999999999996447, -102.7083333306021444, 4.330127018922195425 ) ) ;
#57140=CARTESIAN_POINT ( 'NONE',  ( 6.123233995736766282E-16, -120.0000000000000000, -5.000000000000000000 ) ) ;
#57141=AXIS2_PLACEMENT_3D ( 'NONE', #14722, #40442, #49777 ) ;
#57142=EDGE_LOOP ( 'NONE', ( #24348, #35271, #13329, #56886 ) ) ;
#57144=CARTESIAN_POINT ( 'NONE',  ( 4.458734124999999437, -81.81249999863440792, -5.460374474430324690E-16 ) ) ;
#57145=CARTESIAN_POINT ( 'NONE',  ( 4.458734125000001214, 25.10416666803225638, 2.574251347313718519 ) ) ;
#57146=DIRECTION ( 'NONE',  ( -0.000000000000000000, 1.000000000000000000, -0.000000000000000000 ) ) ;
#57148=CARTESIAN_POINT ( 'NONE',  ( 2.499999999999998668, 14.66666666666666607, -4.330127018922193649 ) ) ;
#57152=DIRECTION ( 'NONE',  ( 0.000000000000000000, 0.000000000000000000, 1.000000000000000000 ) ) ;
#57156=CARTESIAN_POINT ( 'NONE',  ( 9.457646018065525792E-16, -55.06249999863440081, 5.148502694627439702 ) ) ;
#57157=CARTESIAN_POINT ( 'NONE',  ( -6.972266317189433020E-16, 10.75000000000000000, -5.000000000000000000 ) ) ;
#57158=CARTESIAN_POINT ( 'NONE',  ( 4.458734124999998549, 22.27083333469893134, -2.574251347313721627 ) ) ;
#57159=CARTESIAN_POINT ( 'NONE',  ( -5.000000000000000000, -107.0833333333333428, -2.886751345948128211 ) ) ;
#57161=CARTESIAN_POINT ( 'NONE',  ( 2.229367062500001939, -45.22916666530106511, 3.861377020970579999 ) ) ;
#57162=CARTESIAN_POINT ( 'NONE',  ( -5.000000000000000000, -4.874999997268810503, 0.000000000000000000 ) ) ;
#57166=CARTESIAN_POINT ( 'NONE',  ( -2.229367062499996610, -104.1458333319677365, 3.861377020970582219 ) ) ;
#57167=CARTESIAN_POINT ( 'NONE',  ( -4.458734124999999437, -5.645833331967740953, -2.574251347313719407 ) ) ;
#57170=CARTESIAN_POINT ( 'NONE',  ( -4.458734124999999437, -95.39583333196772230, -2.574251347313719407 ) ) ;
#57172=CARTESIAN_POINT ( 'NONE',  ( -3.152548672688508926E-16, -89.81249999863439371, -5.148502694627439702 ) ) ;
#57176=CARTESIAN_POINT ( 'NONE',  ( -2.229367062499996610, -12.14583333196774007, 3.861377020970582219 ) ) ;
#57177=CARTESIAN_POINT ( 'NONE',  ( -4.458734124999999437, 12.43750000136559564, 0.000000000000000000 ) ) ;
#57178=CARTESIAN_POINT ( 'NONE',  ( 4.458734125000000326, -56.14583333196773651, 2.574251347313718519 ) ) ;
#57179=CARTESIAN_POINT ( 'NONE',  ( -5.000000000000000000, -69.08333333333332860, -2.886751345948128211 ) ) ;
#57186=DIRECTION ( 'NONE',  ( 0.000000000000000000, 0.000000000000000000, 1.000000000000000000 ) ) ;
#57187=CARTESIAN_POINT ( 'NONE',  ( -2.229367062500000163, -80.47916666530106511, -3.861377020970580443 ) ) ;
#57188=CARTESIAN_POINT ( 'NONE',  ( 9.457646018065525792E-16, 25.68750000136559208, 5.148502694627439702 ) ) ;
#57192=DIRECTION ( 'NONE',  ( -0.000000000000000000, 1.000000000000000000, -0.000000000000000000 ) ) ;
#57194=CARTESIAN_POINT ( 'NONE',  ( 2.499999999999998668, -69.33333333333332860, -4.330127018922193649 ) ) ;
#57195=CARTESIAN_POINT ( 'NONE',  ( -5.000000000000000000, 29.91666666666666430, -2.886751345948128211 ) ) ;
#57197=ORIENTED_EDGE ( 'NONE', *, *, #40512, .T. ) ;
#57200=( BOUNDED_CURVE ( )  B_SPLINE_CURVE ( 2, ( #5247, #39963, #24871, #53499, #4928, #10387, #19716, #54777, #29345 ),
 .UNSPECIFIED., .F., .F. ) 
 B_SPLINE_CURVE_WITH_KNOTS ( ( 3, 2, 2, 2, 3 ),
 ( 0.2303571428571428714, 0.2309523809523809645, 0.2321428571428571508, 0.2333333333333333370, 0.2339285714285714302 ),
 .UNSPECIFIED. ) 
 CURVE ( )  GEOMETRIC_REPRESENTATION_ITEM ( )  RATIONAL_B_SPLINE_CURVE ( ( 0.9330127018922194093, 0.9330127018922209636, 1.000000000000000000, 0.8660254037844387076, 1.000000000000000000, 0.8660254037844387076, 1.000000000000000000, 0.9330127018922194093, 0.9330127018922194093 ) ) 
 REPRESENTATION_ITEM ( '' )  );
#57204=EDGE_CURVE ( 'NONE', #15879, #23303, #9260, .T. ) ;
#57207=ORIENTED_EDGE ( 'NONE', *, *, #3657, .F. ) ;
#57213=CARTESIAN_POINT ( 'NONE',  ( -4.458734124999998549, -51.47916666530106511, 2.574251347313722516 ) ) ;
#57215=CARTESIAN_POINT ( 'NONE',  ( -1.339745962155610925, -54.66965819600732601, 5.000000000000000000 ) ) ;
#57223=CARTESIAN_POINT ( 'NONE',  ( -2.229367062499996610, -102.3958333319677365, 3.861377020970582219 ) ) ;
#57228=VECTOR ( 'NONE', #54468, 1000.000000000000000 ) ;
#57230=CARTESIAN_POINT ( 'NONE',  ( -4.458734124999999437, -5.312499998634402587, 0.000000000000000000 ) ) ;
#57232=CARTESIAN_POINT ( 'NONE',  ( -3.152548672688508926E-16, -96.81249999863440792, -5.148502694627439702 ) ) ;
#57234=CARTESIAN_POINT ( 'NONE',  ( 2.229367062500001939, -29.22916666530107221, 3.861377020970579999 ) ) ;
#57236=CARTESIAN_POINT ( 'NONE',  ( 1.975475456537005874E-15, -66.62499999726881583, 5.000000000000000000 ) ) ;
#57239=CARTESIAN_POINT ( 'NONE',  ( -2.499999999999996447, -15.83333333333333037, 4.330127018922195425 ) ) ;
#57240=DIRECTION ( 'NONE',  ( -0.000000000000000000, 1.000000000000000000, -0.000000000000000000 ) ) ;
#57242=CARTESIAN_POINT ( 'NONE',  ( -2.229367062500000163, 8.270833334698926009, -3.861377020970580443 ) ) ;
#57246=CARTESIAN_POINT ( 'NONE',  ( -2.500000000000000444, -93.16666666666665719, -4.330127018922193649 ) ) ;
#57247=CARTESIAN_POINT ( 'NONE',  ( 4.458734124999998549, -23.72916666530107221, -2.574251347313721627 ) ) ;
#57248=CARTESIAN_POINT ( 'NONE',  ( 1.975475456537005874E-15, -76.62499999726880162, 5.000000000000000000 ) ) ;
#57249=CARTESIAN_POINT ( 'NONE',  ( 2.229367062499998831, -76.89583333196773651, -3.861377020970580887 ) ) ;
#57251=CARTESIAN_POINT ( 'NONE',  ( 6.123233995736766282E-16, -120.0000000000000000, -5.000000000000000000 ) ) ;
#57253=CARTESIAN_POINT ( 'NONE',  ( 2.229367062500001939, 5.020833334698926897, 3.861377020970579999 ) ) ;
#57254=LINE ( 'NONE', #42431, #11938 ) ;
#57257=CARTESIAN_POINT ( 'NONE',  ( -4.458734124999999437, -73.31249999863439371, 0.000000000000000000 ) ) ;
#57259=CARTESIAN_POINT ( 'NONE',  ( 1.060575238724906964E-15, -7.749999999999999112, 5.773502691896257311 ) ) ;
#57262=CARTESIAN_POINT ( 'NONE',  ( 2.229367062500001939, -63.97916666530106511, 3.861377020970579999 ) ) ;
#57263=CARTESIAN_POINT ( 'NONE',  ( -5.000000000000000000, -97.95833333060214443, -2.886751345948128211 ) ) ;
#57266=FACE_OUTER_BOUND ( 'NONE', #54247, .T. ) ;
#57267=CARTESIAN_POINT ( 'NONE',  ( 2.229367062499998831, -104.8958333319677365, -3.861377020970580887 ) ) ;
#57269=CARTESIAN_POINT ( 'NONE',  ( -5.000000000000000000, -56.08333333333332860, -2.886751345948128211 ) ) ;
#57271=CARTESIAN_POINT ( 'NONE',  ( -5.000000000000000000, 15.91666666666666430, -2.886751345948128211 ) ) ;
#57272=EDGE_LOOP ( 'NONE', ( #62514, #43092, #43687, #2086 ) ) ;
#57277=AXIS2_PLACEMENT_3D ( 'NONE', #35638, #11184, #60413 ) ;
#57281=CARTESIAN_POINT ( 'NONE',  ( 7.204675194429079505E-15, 27.74999999999999645, -5.000000000000000000 ) ) ;
#57291=CARTESIAN_POINT ( 'NONE',  ( -4.458734124999998549, -38.47916666530107221, 2.574251347313722516 ) ) ;
#57299=CARTESIAN_POINT ( 'NONE',  ( 5.000000000000000888, -26.58333333333333215, 2.886751345948126879 ) ) ;
#57300=CARTESIAN_POINT ( 'NONE',  ( -4.458734124999999437, -85.56249999863439371, 0.000000000000000000 ) ) ;
#57301=CARTESIAN_POINT ( 'NONE',  ( 5.000000000000000888, 3.416666666666665186, 2.886751345948126879 ) ) ;
#57302=VERTEX_POINT ( 'NONE', #11879 ) ;
#57304=CARTESIAN_POINT ( 'NONE',  ( -2.499999999999996447, -104.8333333333333286, 4.330127018922195425 ) ) ;
#57308=ORIENTED_EDGE ( 'NONE', *, *, #24062, .T. ) ;
#57311=CARTESIAN_POINT ( 'NONE',  ( 9.457646018065525792E-16, -12.31249999863440259, 5.148502694627439702 ) ) ;
#57315=CARTESIAN_POINT ( 'NONE',  ( -3.152548672688508926E-16, 28.18750000136558853, -5.148502694627439702 ) ) ;
#57317=CARTESIAN_POINT ( 'NONE',  ( 4.458734125000000326, -89.89583333196773651, 2.574251347313718519 ) ) ;
#57318=CARTESIAN_POINT ( 'NONE',  ( -5.000000000000000000, -97.08333333333332860, -2.886751345948128211 ) ) ;
#57319=CARTESIAN_POINT ( 'NONE',  ( 1.975475456537005874E-15, -62.74999999999998579, 5.000000000000000000 ) ) ;
#57320=CARTESIAN_POINT ( 'NONE',  ( 2.229367062499998831, -7.645833331967735624, -3.861377020970580887 ) ) ;
#57324=EDGE_CURVE ( 'NONE', #59413, #56396, #50817, .T. ) ;
#57325=LINE ( 'NONE', #40680, #23283 ) ;
#57326=CARTESIAN_POINT ( 'NONE',  ( -3.535250795749689387E-16, -37.12499999726881583, -5.773502691896257311 ) ) ;
#57327=CARTESIAN_POINT ( 'NONE',  ( 2.500000000000002220, -29.66666666666666785, 4.330127018922192761 ) ) ;
#57328=CARTESIAN_POINT ( 'NONE',  ( -2.229367062499996610, 18.85416666803225993, 3.861377020970582219 ) ) ;
#57330=CARTESIAN_POINT ( 'NONE',  ( -2.229367062500000163, -58.47916666530106511, -3.861377020970580443 ) ) ;
#57332=CARTESIAN_POINT ( 'NONE',  ( 0.000000000000000000, -120.0000000000000000, 0.000000000000000000 ) ) ;
#57333=CARTESIAN_POINT ( 'NONE',  ( -4.999999999999999112, 10.08333333333333393, 2.886751345948131764 ) ) ;
#57336=CARTESIAN_POINT ( 'NONE',  ( -4.458734124999999437, -46.39583333196774362, -2.574251347313719407 ) ) ;
#57337=CARTESIAN_POINT ( 'NONE',  ( -2.500000000000000444, -83.04166666393547303, -4.330127018922193649 ) ) ;
#57339=CARTESIAN_POINT ( 'NONE',  ( 1.975475456537005874E-15, -65.62499999726881583, 5.000000000000000000 ) ) ;
#57341=CARTESIAN_POINT ( 'NONE',  ( -4.458734124999997661, -91.47916666530106511, 2.574251347313722516 ) ) ;
#57343=CARTESIAN_POINT ( 'NONE',  ( 5.000000000000000888, -31.58333333333333215, 2.886751345948126879 ) ) ;
#57344=ORIENTED_EDGE ( 'NONE', *, *, #7133, .T. ) ;
#57347=CARTESIAN_POINT ( 'NONE',  ( 4.458734125000001214, -94.89583333196773651, 2.574251347313718519 ) ) ;
#57348=CARTESIAN_POINT ( 'NONE',  ( -4.458734124999999437, 8.437500001365595637, 0.000000000000000000 ) ) ;
#57349=CARTESIAN_POINT ( 'NONE',  ( -2.500000000000000444, 12.95833333606451809, -4.330127018922193649 ) ) ;
#57350=( BOUNDED_CURVE ( )  B_SPLINE_CURVE ( 2, ( #46801, #40695, #7262, #60340, #46170, #16268, #26875, #2748, #35887 ),
 .UNSPECIFIED., .F., .F. ) 
 B_SPLINE_CURVE_WITH_KNOTS ( ( 3, 2, 2, 2, 3 ),
 ( 0.4910714285714285476, 0.4916666666666666408, 0.4928571428571428825, 0.4940476190476190688, 0.4946428571428571619 ),
 .UNSPECIFIED. ) 
 CURVE ( )  GEOMETRIC_REPRESENTATION_ITEM ( )  RATIONAL_B_SPLINE_CURVE ( ( 0.9330127018922194093, 0.9330127018922194093, 1.000000000000000000, 0.8660254037844387076, 1.000000000000000000, 0.8660254037844387076, 1.000000000000000000, 0.9330127018922194093, 0.9330127018922194093 ) ) 
 REPRESENTATION_ITEM ( '' )  );
#57351=CARTESIAN_POINT ( 'NONE',  ( -6.972266317189433020E-16, -29.12499999726880873, -5.000000000000000000 ) ) ;
#57354=CARTESIAN_POINT ( 'NONE',  ( 5.000000000000000888, -78.58333333333334281, 2.886751345948126879 ) ) ;
#57360=CARTESIAN_POINT ( 'NONE',  ( -2.229367062499996610, -20.39583333196774007, 3.861377020970582219 ) ) ;
#57369=VERTEX_POINT ( 'NONE', #31498 ) ;
#57372=CARTESIAN_POINT ( 'NONE',  ( -2.229367062499996610, -68.39583333196773651, 3.861377020970582219 ) ) ;
#57374=CARTESIAN_POINT ( 'NONE',  ( -6.972266317189433020E-16, -6.124999997268813168, -5.000000000000000000 ) ) ;
#57384=CARTESIAN_POINT ( 'NONE',  ( -2.229367062500000163, 1.520833334698927564, -3.861377020970580443 ) ) ;
#57389=VERTEX_POINT ( 'NONE', #16082 ) ;
#57390=CARTESIAN_POINT ( 'NONE',  ( 2.229367062500001939, -74.97916666530106511, 3.861377020970579999 ) ) ;
#57393=CARTESIAN_POINT ( 'NONE',  ( -3.152548672688508926E-16, 6.437500001365592972, -5.148502694627439702 ) ) ;
#57395=CARTESIAN_POINT ( 'NONE',  ( -4.458734124999999437, -62.56249999863440792, 0.000000000000000000 ) ) ;
#57396=CARTESIAN_POINT ( 'NONE',  ( 5.000000000000000000, -19.29166666393548013, -2.886751345948129988 ) ) ;
#57397=EDGE_CURVE ( 'NONE', #5237, #456, #57746, .T. ) ;
#57399=CARTESIAN_POINT ( 'NONE',  ( 1.339745962155615144, -28.58034179853029144, 4.999999999999999112 ) ) ;
#57401=CARTESIAN_POINT ( 'NONE',  ( -2.500000000000000444, -84.04166666393547303, -4.330127018922193649 ) ) ;
#57403=CARTESIAN_POINT ( 'NONE',  ( -2.229367062499996610, -39.14583333196773651, 3.861377020970582219 ) ) ;
#57404=CARTESIAN_POINT ( 'NONE',  ( 4.458734124999998549, -26.97916666530107221, -2.574251347313721627 ) ) ;
#57405=VECTOR ( 'NONE', #42057, 1000.000000000000000 ) ;
#57407=CARTESIAN_POINT ( 'NONE',  ( -4.458734124999998549, -108.2291666653010651, 2.574251347313722516 ) ) ;
#57409=EDGE_LOOP ( 'NONE', ( #50157, #28090, #38372, #41363 ) ) ;
#57410=CARTESIAN_POINT ( 'NONE',  ( 4.458734125000001214, -106.1458333319677365, 2.574251347313718519 ) ) ;
#57411=CARTESIAN_POINT ( 'NONE',  ( -3.152548672688508926E-16, -34.56249999863440792, -5.148502694627439702 ) ) ;
#57412=CARTESIAN_POINT ( 'NONE',  ( -5.000000000000000000, -69.95833333060214443, -2.886751345948128211 ) ) ;
#57415=CARTESIAN_POINT ( 'NONE',  ( 4.458734125000000326, -28.89583333196774007, 2.574251347313718519 ) ) ;
#57416=CARTESIAN_POINT ( 'NONE',  ( -2.229367062499996610, -71.39583333196773651, 3.861377020970582219 ) ) ;
#57420=CARTESIAN_POINT ( 'NONE',  ( 2.499999999999998668, 22.79166666939785202, -4.330127018922193649 ) ) ;
#57421=CARTESIAN_POINT ( 'NONE',  ( 5.000000000000000888, -18.58333333333333215, 2.886751345948126879 ) ) ;
#57423=VERTEX_POINT ( 'NONE', #43052 ) ;
#57426=CARTESIAN_POINT ( 'NONE',  ( -5.000000000000000000, 29.04166666939784847, -2.886751345948128211 ) ) ;
#57427=CARTESIAN_POINT ( 'NONE',  ( 1.975475456537005874E-15, -0.7499999999999996669, 5.000000000000000000 ) ) ;
#57435=ORIENTED_EDGE ( 'NONE', *, *, #26376, .T. ) ;
#57437=ORIENTED_EDGE ( 'NONE', *, *, #60578, .F. ) ;
#57442=VERTEX_POINT ( 'NONE', #18917 ) ;
#57444=EDGE_LOOP ( 'NONE', ( #34644, #31620, #52515, #17717 ) ) ;
#57448=CARTESIAN_POINT ( 'NONE',  ( 0.000000000000000000, -120.0000000000000000, 0.000000000000000000 ) ) ;
#57450=AXIS2_PLACEMENT_3D ( 'NONE', #34810, #5539, #21289 ) ;
#57452=ORIENTED_EDGE ( 'NONE', *, *, #12202, .F. ) ;
#57454=EDGE_CURVE ( 'NONE', #61001, #23800, #20736, .T. ) ;
#57455=EDGE_CURVE ( 'NONE', #5237, #26195, #13479, .T. ) ;
#57456=CARTESIAN_POINT ( 'NONE',  ( -4.458734124999998549, -80.22916666530106511, 2.574251347313722516 ) ) ;
#57457=CARTESIAN_POINT ( 'NONE',  ( 2.229367062500001939, 23.02083333469892423, 3.861377020970579999 ) ) ;
#57458=CARTESIAN_POINT ( 'NONE',  ( 1.975475456537005874E-15, 11.24999999999999822, 5.000000000000000000 ) ) ;
#57459=EDGE_CURVE ( 'NONE', #59581, #5972, #61889, .T. ) ;
#57460=ORIENTED_EDGE ( 'NONE', *, *, #7152, .T. ) ;
#57461=CARTESIAN_POINT ( 'NONE',  ( 5.000000000000000000, 14.58333333333333215, -2.886751345948130876 ) ) ;
#57465=FACE_OUTER_BOUND ( 'NONE', #50661, .T. ) ;
#57466=CARTESIAN_POINT ( 'NONE',  ( 0.000000000000000000, -120.0000000000000000, 0.000000000000000000 ) ) ;
#57468=CARTESIAN_POINT ( 'NONE',  ( -4.458734124999999437, -56.39583333196773651, -2.574251347313719407 ) ) ;
#57469=DIRECTION ( 'NONE',  ( -0.000000000000000000, 1.000000000000000000, -0.000000000000000000 ) ) ;
#57470=CARTESIAN_POINT ( 'NONE',  ( 2.229367062499998831, 21.35416666803226349, -3.861377020970580887 ) ) ;
#57475=CARTESIAN_POINT ( 'NONE',  ( 2.229367062500001939, -43.22916666530107932, 3.861377020970579999 ) ) ;
#57476=CARTESIAN_POINT ( 'NONE',  ( 2.499999999999998668, -6.208333330602149758, -4.330127018922193649 ) ) ;
#57479=FACE_OUTER_BOUND ( 'NONE', #4917, .T. ) ;
#57481=CARTESIAN_POINT ( 'NONE',  ( -3.152548672688508926E-16, -103.5624999986344079, -5.148502694627439702 ) ) ;
#57482=CARTESIAN_POINT ( 'NONE',  ( 2.229367062500001939, -5.229166665301071326, 3.861377020970579999 ) ) ;
#57483=ORIENTED_EDGE ( 'NONE', *, *, #26107, .T. ) ;
#57485=CARTESIAN_POINT ( 'NONE',  ( -4.458734124999999437, -92.31249999863440792, 0.000000000000000000 ) ) ;
#57486=ADVANCED_FACE ( 'NONE', ( #61747 ), #37289, .T. ) ;
#57488=CARTESIAN_POINT ( 'NONE',  ( 9.457646018065525792E-16, -91.31249999863440792, 5.148502694627439702 ) ) ;
#57491=CARTESIAN_POINT ( 'NONE',  ( -3.152548672688508926E-16, -14.56249999863440259, -5.148502694627439702 ) ) ;
#57492=CARTESIAN_POINT ( 'NONE',  ( 4.458734124999998549, 12.02083333469892601, -2.574251347313721627 ) ) ;
#57493=CARTESIAN_POINT ( 'NONE',  ( -4.458734124999997661, -51.47916666530107932, 2.574251347313722516 ) ) ;
#57495=CARTESIAN_POINT ( 'NONE',  ( -6.972266317189433020E-16, -106.2500000000000000, -5.000000000000000000 ) ) ;
#57497=CARTESIAN_POINT ( 'NONE',  ( -6.972266317189433020E-16, -106.1249999972688016, -5.000000000000000000 ) ) ;
#57501=UNCERTAINTY_MEASURE_WITH_UNIT (LENGTH_MEASURE( 1.000000000000000082E-05 ), #53783, 'distance_accuracy_value', 'NONE');
#57505=CARTESIAN_POINT ( 'NONE',  ( -4.458734124999999437, -80.31249999863440792, 0.000000000000000000 ) ) ;
#57506=CARTESIAN_POINT ( 'NONE',  ( 2.229367062500001939, 23.77083333469892779, 3.861377020970579999 ) ) ;
#57508=CARTESIAN_POINT ( 'NONE',  ( -2.500000000000000444, 6.833333333333333925, -4.330127018922193649 ) ) ;
#57509=DIRECTION ( 'NONE',  ( -0.000000000000000000, 1.000000000000000000, -0.000000000000000000 ) ) ;
#57511=CARTESIAN_POINT ( 'NONE',  ( -2.499999999999996447, -67.83333333333332860, 4.330127018922195425 ) ) ;
#57514=CARTESIAN_POINT ( 'NONE',  ( -1.339745962155610925, -61.66965819600733312, 5.000000000000000000 ) ) ;
#57515=CARTESIAN_POINT ( 'NONE',  ( 5.000000000000000000, -40.41666666666667140, -2.886751345948130876 ) ) ;
#57521=ORIENTED_EDGE ( 'NONE', *, *, #9495, .T. ) ;
#57523=ORIENTED_EDGE ( 'NONE', *, *, #5455, .F. ) ;
#57526=CARTESIAN_POINT ( 'NONE',  ( 4.458734125000001214, -54.14583333196773651, 2.574251347313718519 ) ) ;
#57527=( BOUNDED_CURVE ( )  B_SPLINE_CURVE ( 2, ( #61702, #57195, #56875, #22141, #17631 ),
 .UNSPECIFIED., .F., .F. ) 
 B_SPLINE_CURVE_WITH_KNOTS ( ( 3, 2, 3 ),
 ( 0.000000000000000000, 0.001190476190476190584, 0.001785714285714286092 ),
 .UNSPECIFIED. ) 
 CURVE ( )  GEOMETRIC_REPRESENTATION_ITEM ( )  RATIONAL_B_SPLINE_CURVE ( ( 1.000000000000000000, 0.8660254037844387076, 1.000000000000000000, 0.9330127018922192983, 0.9330127018922194093 ) ) 
 REPRESENTATION_ITEM ( '' )  );
#57529=CARTESIAN_POINT ( 'NONE',  ( -4.999999999999998224, -54.79166666393548013, 2.886751345948131764 ) ) ;
#57530=EDGE_LOOP ( 'NONE', ( #50880, #11421, #5366, #19277 ) ) ;
#57534=VERTEX_POINT ( 'NONE', #52088 ) ;
#57535=ADVANCED_FACE ( 'NONE', ( #8026 ), #42416, .T. ) ;
#57537=CARTESIAN_POINT ( 'NONE',  ( -4.458734124999999437, -97.56249999863440792, 0.000000000000000000 ) ) ;
#57542=CARTESIAN_POINT ( 'NONE',  ( -6.972266317189433020E-16, -83.24999999999998579, -5.000000000000000000 ) ) ;
#57543=CARTESIAN_POINT ( 'NONE',  ( -4.458734124999998549, -7.229166665301073103, 2.574251347313722516 ) ) ;
#57544=CARTESIAN_POINT ( 'NONE',  ( -2.229367062499996610, -103.3958333319677365, 3.861377020970582219 ) ) ;
#57546=CARTESIAN_POINT ( 'NONE',  ( 4.458734124999999437, -26.06249999863440792, -5.460374474430324690E-16 ) ) ;
#57547=CARTESIAN_POINT ( 'NONE',  ( 1.975475456537005874E-15, -55.62499999726880873, 5.000000000000000000 ) ) ;
#57553=CARTESIAN_POINT ( 'NONE',  ( -1.339745962155610925, -33.79465819873851729, 5.000000000000000000 ) ) ;
#57555=CARTESIAN_POINT ( 'NONE',  ( 4.458734124999999437, 11.93750000136559564, -5.460374474430324690E-16 ) ) ;
#57558=EDGE_CURVE ( 'NONE', #28144, #4881, #20524, .T. ) ;
#57560=CARTESIAN_POINT ( 'NONE',  ( -3.535250795749689387E-16, -92.25000000000001421, -5.773502691896257311 ) ) ;
#57561=CARTESIAN_POINT ( 'NONE',  ( -3.152548672688508926E-16, -22.56249999863440081, -5.148502694627439702 ) ) ;
#57563=CARTESIAN_POINT ( 'NONE',  ( -2.229367062499996610, -74.39583333196773651, 3.861377020970582219 ) ) ;
#57565=CARTESIAN_POINT ( 'NONE',  ( 2.500000000000002220, -79.54166666393547303, 4.330127018922192761 ) ) ;
#57568=CARTESIAN_POINT ( 'NONE',  ( 2.229367062500001939, 4.020833334698926009, 3.861377020970579999 ) ) ;
#57569=CARTESIAN_POINT ( 'NONE',  ( 9.457646018065525792E-16, 26.68750000136559564, 5.148502694627439702 ) ) ;
#57570=CARTESIAN_POINT ( 'NONE',  ( 2.229367062499998831, -38.89583333196773651, -3.861377020970580887 ) ) ;
#57572=CARTESIAN_POINT ( 'NONE',  ( 4.458734125000001214, -71.89583333196773651, 2.574251347313718519 ) ) ;
#57574=( BOUNDED_CURVE ( )  B_SPLINE_CURVE ( 2, ( #51010, #7901, #56798, #26563, #46182, #27506, #3082, #21747, #42299 ),
 .UNSPECIFIED., .F., .F. ) 
 B_SPLINE_CURVE_WITH_KNOTS ( ( 3, 2, 2, 2, 3 ),
 ( 0.03035714285714285685, 0.03095238095238095344, 0.03214285714285713969, 0.03333333333333333287, 0.03392857142857143293 ),
 .UNSPECIFIED. ) 
 CURVE ( )  GEOMETRIC_REPRESENTATION_ITEM ( )  RATIONAL_B_SPLINE_CURVE ( ( 0.9330127018922194093, 0.9330127018922194093, 1.000000000000000000, 0.8660254037844387076, 1.000000000000000000, 0.8660254037844387076, 1.000000000000000000, 0.9330127018922189652, 0.9330127018922194093 ) ) 
 REPRESENTATION_ITEM ( '' )  );
#57575=CARTESIAN_POINT ( 'NONE',  ( 5.000000000000000000, -8.500000000000000000, -6.123233995736766282E-16 ) ) ;
#57578=CARTESIAN_POINT ( 'NONE',  ( 2.229367062499998831, -64.64583333196773651, -3.861377020970580887 ) ) ;
#57579=CARTESIAN_POINT ( 'NONE',  ( -5.000000000000000000, -98.95833333060213022, -2.886751345948128211 ) ) ;
#57582=LINE ( 'NONE', #9293, #22564 ) ;
#57583=CARTESIAN_POINT ( 'NONE',  ( 2.229367062499998831, -103.8958333319677365, -3.861377020970580887 ) ) ;
#57585=CARTESIAN_POINT ( 'NONE',  ( -3.535250795749689387E-16, -55.24999999999998579, -5.773502691896257311 ) ) ;
#57594=CARTESIAN_POINT ( 'NONE',  ( -5.000000000000000000, -4.874999997268810503, 0.000000000000000000 ) ) ;
#57604=CARTESIAN_POINT ( 'NONE',  ( -2.229367062500000163, -37.72916666530107221, -3.861377020970580443 ) ) ;
#57613=CARTESIAN_POINT ( 'NONE',  ( -2.229367062499996610, -86.39583333196773651, 3.861377020970582219 ) ) ;
#57615=ORIENTED_EDGE ( 'NONE', *, *, #47661, .F. ) ;
#57621=CARTESIAN_POINT ( 'NONE',  ( -6.972266317189433020E-16, -14.24999999999999822, -5.000000000000000000 ) ) ;
#57622=CARTESIAN_POINT ( 'NONE',  ( -4.458734124999998549, -13.47916666530107221, 2.574251347313722516 ) ) ;
#57623=CARTESIAN_POINT ( 'NONE',  ( 1.339745962155612702, -105.1696581960073331, -5.000000000000000000 ) ) ;
#57627=CARTESIAN_POINT ( 'NONE',  ( -4.458734124999999437, 26.43750000136559564, 0.000000000000000000 ) ) ;
#57629=CARTESIAN_POINT ( 'NONE',  ( 4.458734124999998549, -90.72916666530106511, -2.574251347313721627 ) ) ;
#57631=CARTESIAN_POINT ( 'NONE',  ( 1.975475456537005874E-15, 7.375000002731186832, 5.000000000000000000 ) ) ;
#57632=CARTESIAN_POINT ( 'NONE',  ( -2.229367062500000163, -9.479166665301068662, -3.861377020970580443 ) ) ;
#57635=DIRECTION ( 'NONE',  ( -0.000000000000000000, 1.000000000000000000, -0.000000000000000000 ) ) ;
#57637=CARTESIAN_POINT ( 'NONE',  ( -3.535250795749689387E-16, -38.12499999726881583, -5.773502691896257311 ) ) ;
#57639=CARTESIAN_POINT ( 'NONE',  ( -4.458734124999999437, 17.68750000136559208, 0.000000000000000000 ) ) ;
#57640=CARTESIAN_POINT ( 'NONE',  ( -2.500000000000000444, -95.16666666666667140, -4.330127018922193649 ) ) ;
#57642=CARTESIAN_POINT ( 'NONE',  ( -4.458734124999999437, -56.39583333196773651, -2.574251347313719407 ) ) ;
#57644=DIRECTION ( 'NONE',  ( 0.000000000000000000, 0.000000000000000000, 1.000000000000000000 ) ) ;
#57645=CARTESIAN_POINT ( 'NONE',  ( 5.000000000000000888, 9.416666666666666075, 2.886751345948126879 ) ) ;
#57648=CARTESIAN_POINT ( 'NONE',  ( 2.229367062500001939, -49.97916666530107221, 3.861377020970579999 ) ) ;
#57649=CARTESIAN_POINT ( 'NONE',  ( 2.500000000000002220, -86.54166666393547303, 4.330127018922192761 ) ) ;
#57651=( BOUNDED_CURVE ( )  B_SPLINE_CURVE ( 2, ( #17, #653, #19618, #40509, #58855, #19933, #15445, #30214, #49525 ),
 .UNSPECIFIED., .F., .F. ) 
 B_SPLINE_CURVE_WITH_KNOTS ( ( 3, 2, 2, 2, 3 ),
 ( 0.4874999999999999889, 0.4880952380952380820, 0.4892857142857142683, 0.4904761904761904545, 0.4910714285714285476 ),
 .UNSPECIFIED. ) 
 CURVE ( )  GEOMETRIC_REPRESENTATION_ITEM ( )  RATIONAL_B_SPLINE_CURVE ( ( 0.9330127018922194093, 0.9330127018922194093, 1.000000000000000000, 0.8660254037844387076, 1.000000000000000000, 0.8660254037844387076, 1.000000000000000000, 0.9330127018922194093, 0.9330127018922194093 ) ) 
 REPRESENTATION_ITEM ( '' )  );
#57653=DIRECTION ( 'NONE',  ( -0.000000000000000000, 1.000000000000000000, -0.000000000000000000 ) ) ;
#57654=CARTESIAN_POINT ( 'NONE',  ( 2.229367062499998831, -91.89583333196773651, -3.861377020970580887 ) ) ;
#57656=CARTESIAN_POINT ( 'NONE',  ( 1.060575238724906964E-15, -39.75000000000000000, 5.773502691896257311 ) ) ;
#57657=CARTESIAN_POINT ( 'NONE',  ( 1.975475456537005874E-15, 24.24999999999999645, 5.000000000000000000 ) ) ;
#57661=CARTESIAN_POINT ( 'NONE',  ( -4.458734124999999437, -94.31249999863440792, 0.000000000000000000 ) ) ;
#57662=CARTESIAN_POINT ( 'NONE',  ( -2.229367062500000163, 10.27083333469892779, -3.861377020970580443 ) ) ;
#57663=CARTESIAN_POINT ( 'NONE',  ( -2.500000000000000444, 10.95833333606451632, -4.330127018922193649 ) ) ;
#57670=CARTESIAN_POINT ( 'NONE',  ( 5.000000000000000000, -40.37499999726880162, -6.123233995736766282E-16 ) ) ;
#57675=CARTESIAN_POINT ( 'NONE',  ( -3.152548672688508926E-16, -17.81249999863440792, -5.148502694627439702 ) ) ;
#57684=VERTEX_POINT ( 'NONE', #30147 ) ;
#57687=CARTESIAN_POINT ( 'NONE',  ( -2.229367062500000163, -67.72916666530106511, -3.861377020970580443 ) ) ;
#57689=VERTEX_POINT ( 'NONE', #53336 ) ;
#57692=CARTESIAN_POINT ( 'NONE',  ( 4.458734124999998549, 4.020833334698926009, -2.574251347313721627 ) ) ;
#57694=CARTESIAN_POINT ( 'NONE',  ( -2.500000000000000444, 1.958333336064519647, -4.330127018922193649 ) ) ;
#57695=CARTESIAN_POINT ( 'NONE',  ( 2.229367062500001939, 3.020833334698928674, 3.861377020970579999 ) ) ;
#57701=EDGE_LOOP ( 'NONE', ( #22000, #41116, #28153, #21341 ) ) ;
#57702=CARTESIAN_POINT ( 'NONE',  ( -2.229367062499996610, -77.14583333196773651, 3.861377020970582219 ) ) ;
#57704=CARTESIAN_POINT ( 'NONE',  ( -4.458734124999998549, 5.770833334698927786, 2.574251347313722516 ) ) ;
#57705=CARTESIAN_POINT ( 'NONE',  ( -5.000000000000000000, -41.99999999999999289, 0.000000000000000000 ) ) ;
#57706=CARTESIAN_POINT ( 'NONE',  ( -4.458734124999999437, -61.64583333196773651, -2.574251347313719407 ) ) ;
#57707=CARTESIAN_POINT ( 'NONE',  ( -4.999999999999999112, -21.79166666393547658, 2.886751345948131764 ) ) ;
#57708=CARTESIAN_POINT ( 'NONE',  ( 5.000000000000000000, -96.37499999726881583, -6.123233995736766282E-16 ) ) ;
#57709=CARTESIAN_POINT ( 'NONE',  ( 0.000000000000000000, -120.0000000000000000, 0.000000000000000000 ) ) ;
#57713=CARTESIAN_POINT ( 'NONE',  ( -4.458734124999998549, -39.22916666530107221, 2.574251347313722516 ) ) ;
#57714=CARTESIAN_POINT ( 'NONE',  ( 4.458734124999999437, -29.06249999863440436, -5.460374474430324690E-16 ) ) ;
#57715=DIRECTION ( 'NONE',  ( -0.000000000000000000, 1.000000000000000000, -0.000000000000000000 ) ) ;
#57716=CARTESIAN_POINT ( 'NONE',  ( 2.500000000000002220, 26.33333333333333215, 4.330127018922192761 ) ) ;
#57719=CARTESIAN_POINT ( 'NONE',  ( -1.339745962155610925, -49.79465819873851729, 5.000000000000000000 ) ) ;
#57720=CARTESIAN_POINT ( 'NONE',  ( -3.152548672688508926E-16, -31.56249999863440436, -5.148502694627439702 ) ) ;
#57721=CARTESIAN_POINT ( 'NONE',  ( -2.499999999999996447, -70.70833333060214443, 4.330127018922195425 ) ) ;
#57724=CARTESIAN_POINT ( 'NONE',  ( -2.229367062500000163, -27.47916666530107221, -3.861377020970580443 ) ) ;
#57725=CARTESIAN_POINT ( 'NONE',  ( 2.229367062500001939, -73.22916666530107932, 3.861377020970579999 ) ) ;
#57728=CARTESIAN_POINT ( 'NONE',  ( 1.975475456537005874E-15, -23.62499999726880873, 5.000000000000000000 ) ) ;
#57730=CARTESIAN_POINT ( 'NONE',  ( -2.500000000000000444, -21.16666666666666785, -4.330127018922193649 ) ) ;
#57733=CARTESIAN_POINT ( 'NONE',  ( -6.972266317189433020E-16, -79.12499999726881583, -5.000000000000000000 ) ) ;
#57735=CARTESIAN_POINT ( 'NONE',  ( 5.000000000000000000, 25.70833333606452342, -2.886751345948129988 ) ) ;
#57736=CYLINDRICAL_SURFACE ( 'NONE', #26820, 5.000000000000000000 ) ;
#57739=CARTESIAN_POINT ( 'NONE',  ( 0.000000000000000000, -120.0000000000000000, 5.000000000000000000 ) ) ;
#57742=CARTESIAN_POINT ( 'NONE',  ( -6.972266317189433020E-16, -81.12499999726881583, -5.000000000000000000 ) ) ;
#57744=DIRECTION ( 'NONE',  ( -0.000000000000000000, 1.000000000000000000, -0.000000000000000000 ) ) ;
#57745=ORIENTED_EDGE ( 'NONE', *, *, #8289, .F. ) ;
#57746=( BOUNDED_CURVE ( )  B_SPLINE_CURVE ( 2, ( #1951, #60795, #7714, #23126, #32456, #47869, #18615, #28570, #32135 ),
 .UNSPECIFIED., .F., .F. ) 
 B_SPLINE_CURVE_WITH_KNOTS ( ( 3, 2, 2, 2, 3 ),
 ( 0.09107142857142856707, 0.09166666666666666019, 0.09285714285714286031, 0.09404761904761904656, 0.09464285714285713969 ),
 .UNSPECIFIED. ) 
 CURVE ( )  GEOMETRIC_REPRESENTATION_ITEM ( )  RATIONAL_B_SPLINE_CURVE ( ( 0.9330127018922194093, 0.9330127018922194093, 1.000000000000000000, 0.8660254037844387076, 1.000000000000000000, 0.8660254037844387076, 1.000000000000000000, 0.9330127018922194093, 0.9330127018922194093 ) ) 
 REPRESENTATION_ITEM ( '' )  );
#57747=CARTESIAN_POINT ( 'NONE',  ( 5.000000000000000000, 10.62500000273118594, -6.123233995736766282E-16 ) ) ;
#57750=ADVANCED_FACE ( 'NONE', ( #54286 ), #63310, .T. ) ;
#57752=ORIENTED_EDGE ( 'NONE', *, *, #54312, .F. ) ;
#57756=CARTESIAN_POINT ( 'NONE',  ( -1.339745962155613812, -96.20534180126146850, -5.000000000000000000 ) ) ;
#57757=CARTESIAN_POINT ( 'NONE',  ( 2.499999999999998668, -53.33333333333332860, -4.330127018922193649 ) ) ;
#57765=CARTESIAN_POINT ( 'NONE',  ( 9.457646018065525792E-16, -83.06249999863439371, 5.148502694627439702 ) ) ;
#57766=CARTESIAN_POINT ( 'NONE',  ( 2.229367062500001939, 18.02083333469892779, 3.861377020970579999 ) ) ;
#57767=CARTESIAN_POINT ( 'NONE',  ( -6.972266317189433020E-16, -12.12499999726881406, -5.000000000000000000 ) ) ;
#57772=CARTESIAN_POINT ( 'NONE',  ( 5.000000000000000000, -88.50000000000000000, -6.123233995736766282E-16 ) ) ;
#57774=CARTESIAN_POINT ( 'NONE',  ( -6.972266317189433020E-16, 4.749999999999999112, -5.000000000000000000 ) ) ;
#57775=CARTESIAN_POINT ( 'NONE',  ( -2.229367062499996610, -61.14583333196774362, 3.861377020970582219 ) ) ;
#57777=CARTESIAN_POINT ( 'NONE',  ( 2.229367062499998831, 24.35416666803225993, -3.861377020970580887 ) ) ;
#57778=CARTESIAN_POINT ( 'NONE',  ( -4.999999999999999112, -109.9166666666666572, 2.886751345948131764 ) ) ;
#57780=CARTESIAN_POINT ( 'NONE',  ( 4.458734125000001214, -45.14583333196774362, 2.574251347313718519 ) ) ;
#57782=CARTESIAN_POINT ( 'NONE',  ( 2.500000000000002220, -4.541666663935479242, 4.330127018922192761 ) ) ;
#57783=CARTESIAN_POINT ( 'NONE',  ( -4.330127018922101279, 30.00000000000000000, 7.500000000000002665 ) ) ;
#57786=CARTESIAN_POINT ( 'NONE',  ( 2.229367062499998831, -105.6458333319677365, -3.861377020970580887 ) ) ;
#57787=CARTESIAN_POINT ( 'NONE',  ( 4.458734124999999437, -9.062499998634406140, -5.460374474430324690E-16 ) ) ;
#57788=ORIENTED_EDGE ( 'NONE', *, *, #18939, .T. ) ;
#57790=CARTESIAN_POINT ( 'NONE',  ( 4.458734125000001214, -97.89583333196773651, 2.574251347313718519 ) ) ;
#57792=CARTESIAN_POINT ( 'NONE',  ( -4.458734124999999437, -89.64583333196773651, -2.574251347313719407 ) ) ;
#57793=CARTESIAN_POINT ( 'NONE',  ( -5.000000000000000000, -53.95833333060214443, -2.886751345948128211 ) ) ;
#57796=CARTESIAN_POINT ( 'NONE',  ( -4.458734124999999437, -15.31249999863440436, 0.000000000000000000 ) ) ;
#57797=CARTESIAN_POINT ( 'NONE',  ( -2.229367062499996610, 12.60416666803226171, 3.861377020970582219 ) ) ;
#57798=CARTESIAN_POINT ( 'NONE',  ( 2.229367062500001939, -59.22916666530106511, 3.861377020970579999 ) ) ;
#57800=CARTESIAN_POINT ( 'NONE',  ( -2.499999999999996447, -36.83333333333332860, 4.330127018922195425 ) ) ;
#57802=CYLINDRICAL_SURFACE ( 'NONE', #22694, 5.000000000000000000 ) ;
#57806=CARTESIAN_POINT ( 'NONE',  ( 5.000000000000000888, -68.58333333333332860, 2.886751345948126879 ) ) ;
#57807=CARTESIAN_POINT ( 'NONE',  ( -2.499999999999996447, -66.70833333060214443, 4.330127018922195425 ) ) ;
#57808=CARTESIAN_POINT ( 'NONE',  ( -3.152548672688508926E-16, -83.56249999863440792, -5.148502694627439702 ) ) ;
#57809=CARTESIAN_POINT ( 'NONE',  ( 4.458734124999998549, 24.02083333469892423, -2.574251347313721627 ) ) ;
#57812=EDGE_CURVE ( 'NONE', #57126, #19298, #12089, .T. ) ;
#57813=ADVANCED_FACE ( 'NONE', ( #7871 ), #61273, .T. ) ;
#57814=CARTESIAN_POINT ( 'NONE',  ( -2.499999999999996447, 7.166666666666665186, 4.330127018922195425 ) ) ;
#57817=CARTESIAN_POINT ( 'NONE',  ( -4.999999999999999112, -70.91666666666667140, 2.886751345948131764 ) ) ;
#57820=CARTESIAN_POINT ( 'NONE',  ( 0.000000000000000000, -120.0000000000000000, 0.000000000000000000 ) ) ;
#57825=EDGE_CURVE ( 'NONE', #26615, #15325, #7247, .T. ) ;
#57826=( BOUNDED_CURVE ( )  B_SPLINE_CURVE ( 2, ( #329, #16069, #44047, #19615, #649, #19928, #35369, #39227, #44688 ),
 .UNSPECIFIED., .F., .F. ) 
 B_SPLINE_CURVE_WITH_KNOTS ( ( 3, 2, 2, 2, 3 ),
 ( 0.3446428571428571397, 0.3452380952380952328, 0.3464285714285714191, 0.3476190476190476053, 0.3482142857142856984 ),
 .UNSPECIFIED. ) 
 CURVE ( )  GEOMETRIC_REPRESENTATION_ITEM ( )  RATIONAL_B_SPLINE_CURVE ( ( 0.9330127018922194093, 0.9330127018922194093, 1.000000000000000000, 0.8660254037844387076, 1.000000000000000000, 0.8660254037844387076, 1.000000000000000000, 0.9330127018922194093, 0.9330127018922194093 ) ) 
 REPRESENTATION_ITEM ( '' )  );
#57829=ORIENTED_EDGE ( 'NONE', *, *, #7928, .F. ) ;
#57833=ORIENTED_EDGE ( 'NONE', *, *, #52798, .T. ) ;
#57836=CARTESIAN_POINT ( 'NONE',  ( -4.458734124999999437, -54.64583333196774362, -2.574251347313719407 ) ) ;
#57839=VERTEX_POINT ( 'NONE', #17526 ) ;
#57847=CARTESIAN_POINT ( 'NONE',  ( 9.457646018065525792E-16, -106.3124999986343795, 5.148502694627439702 ) ) ;
#57848=CARTESIAN_POINT ( 'NONE',  ( -1.230605004983934782E-13, -26.62499999726881583, 5.000000000000000000 ) ) ;
#57849=ORIENTED_EDGE ( 'NONE', *, *, #33680, .F. ) ;
#57853=CARTESIAN_POINT ( 'NONE',  ( 4.458734124999999437, -7.812499998634405252, -5.460374474430324690E-16 ) ) ;
#57854=CARTESIAN_POINT ( 'NONE',  ( -4.458734124999997661, -103.4791666653010651, 2.574251347313722516 ) ) ;
#57856=CARTESIAN_POINT ( 'NONE',  ( 4.458734124999998549, -25.97916666530106866, -2.574251347313721627 ) ) ;
#57860=CARTESIAN_POINT ( 'NONE',  ( 5.000000000000000000, -21.29166666393548013, -2.886751345948130876 ) ) ;
#57862=CARTESIAN_POINT ( 'NONE',  ( -2.229367062499996610, 5.604166668032261711, 3.861377020970582219 ) ) ;
#57863=ORIENTED_EDGE ( 'NONE', *, *, #9170, .F. ) ;
#57864=DIRECTION ( 'NONE',  ( -0.000000000000000000, 1.000000000000000000, -0.000000000000000000 ) ) ;
#57866=CARTESIAN_POINT ( 'NONE',  ( -4.999999999999999112, -92.91666666666665719, 2.886751345948131764 ) ) ;
#57867=CARTESIAN_POINT ( 'NONE',  ( -3.152548672688508926E-16, -30.56249999863440436, -5.148502694627439702 ) ) ;
#57869=CARTESIAN_POINT ( 'NONE',  ( 2.229367062499998831, -75.89583333196773651, -3.861377020970580887 ) ) ;
#57873=CARTESIAN_POINT ( 'NONE',  ( 9.457646018065525792E-16, 3.937500001365595192, 5.148502694627439702 ) ) ;
#57874=CARTESIAN_POINT ( 'NONE',  ( 4.458734124999999437, 25.93750000136559564, -5.460374474430324690E-16 ) ) ;
#57875=CARTESIAN_POINT ( 'NONE',  ( 9.457646018065525792E-16, -40.31249999863440081, 5.148502694627439702 ) ) ;
#57880=CARTESIAN_POINT ( 'NONE',  ( -4.458734124999998549, -70.22916666530107932, 2.574251347313722516 ) ) ;
#57881=CARTESIAN_POINT ( 'NONE',  ( -4.999999999999999112, -97.79166666393545881, 2.886751345948131764 ) ) ;
#57883=EDGE_CURVE ( 'NONE', #45091, #44922, #8188, .T. ) ;
#57884=CARTESIAN_POINT ( 'NONE',  ( 2.500000000000002220, 9.458333336064519870, 4.330127018922192761 ) ) ;
#57885=CARTESIAN_POINT ( 'NONE',  ( 4.458734125000000326, -107.1458333319677365, 2.574251347313718519 ) ) ;
#57887=CARTESIAN_POINT ( 'NONE',  ( 2.500000000000002220, -55.66666666666667140, 4.330127018922192761 ) ) ;
#57897=EDGE_CURVE ( 'NONE', #45293, #47799, #3366, .T. ) ;
#57908=EDGE_CURVE ( 'NONE', #20484, #40086, #31673, .T. ) ;
#57910=CARTESIAN_POINT ( 'NONE',  ( -3.152548672688508926E-16, -40.81249999863440081, -5.148502694627439702 ) ) ;
#57918=VECTOR ( 'NONE', #6747, 1000.000000000000000 ) ;
#57919=ADVANCED_FACE ( 'NONE', ( #8807 ), #24224, .T. ) ;
#57920=DIRECTION ( 'NONE',  ( -0.000000000000000000, 1.000000000000000000, -0.000000000000000000 ) ) ;
#57922=CARTESIAN_POINT ( 'NONE',  ( -2.229367062499996610, -84.39583333196773651, 3.861377020970582219 ) ) ;
#57923=CARTESIAN_POINT ( 'NONE',  ( 5.000000000000000000, -34.29166666393547303, -2.886751345948130876 ) ) ;
#57924=VERTEX_POINT ( 'NONE', #4926 ) ;
#57929=ORIENTED_EDGE ( 'NONE', *, *, #11857, .T. ) ;
#57930=CARTESIAN_POINT ( 'NONE',  ( 1.975475456537005874E-15, -78.74999999999998579, 5.000000000000000000 ) ) ;
#57931=CARTESIAN_POINT ( 'NONE',  ( 4.458734124999998549, -9.979166665301068662, -2.574251347313721627 ) ) ;
#57932=DIRECTION ( 'NONE',  ( -0.000000000000000000, 1.000000000000000000, -0.000000000000000000 ) ) ;
#57934=CARTESIAN_POINT ( 'NONE',  ( -5.000000000000000000, -11.87499999726881761, 0.000000000000000000 ) ) ;
#57937=CARTESIAN_POINT ( 'NONE',  ( -2.229367062499996610, 22.60416666803225993, 3.861377020970582219 ) ) ;
#57938=ORIENTED_EDGE ( 'NONE', *, *, #29400, .F. ) ;
#57939=CARTESIAN_POINT ( 'NONE',  ( -4.458734124999999437, -89.39583333196773651, -2.574251347313719407 ) ) ;
#57940=CARTESIAN_POINT ( 'NONE',  ( 5.000000000000000000, -47.50000000000000000, -6.123233995736766282E-16 ) ) ;
#57942=CARTESIAN_POINT ( 'NONE',  ( 9.457646018065525792E-16, -10.06249999863440792, 5.148502694627439702 ) ) ;
#57943=CARTESIAN_POINT ( 'NONE',  ( 1.975475456537005874E-15, -2.624999997268813168, 5.000000000000000000 ) ) ;
#57944=LINE ( 'NONE', #47957, #2727 ) ;
#57946=CARTESIAN_POINT ( 'NONE',  ( 2.500000000000002220, -34.54166666393547303, 4.330127018922192761 ) ) ;
#57948=CARTESIAN_POINT ( 'NONE',  ( -3.152548672688508926E-16, 19.43750000136559208, -5.148502694627439702 ) ) ;
#57951=CARTESIAN_POINT ( 'NONE',  ( -4.458734124999999437, -55.39583333196773651, -2.574251347313719407 ) ) ;
#57954=CARTESIAN_POINT ( 'NONE',  ( -2.499999999999996447, 10.16666666666666785, 4.330127018922195425 ) ) ;
#57956=CARTESIAN_POINT ( 'NONE',  ( 1.339745962155612702, -69.29465819873850307, -5.000000000000000000 ) ) ;
#57957=CARTESIAN_POINT ( 'NONE',  ( 4.458734124999999437, -46.81249999863440792, -5.460374474430324690E-16 ) ) ;
#57958=CARTESIAN_POINT ( 'NONE',  ( 5.000000000000000888, -83.45833333060213022, 2.886751345948126879 ) ) ;
#57960=DIRECTION ( 'NONE',  ( -0.000000000000000000, 1.000000000000000000, -0.000000000000000000 ) ) ;
#57962=CARTESIAN_POINT ( 'NONE',  ( 4.458734125000000326, -92.14583333196773651, 2.574251347313718519 ) ) ;
#57964=CARTESIAN_POINT ( 'NONE',  ( 2.500000000000002220, -38.66666666666667140, 4.330127018922192761 ) ) ;
#57967=CARTESIAN_POINT ( 'NONE',  ( -2.229367062500000163, -97.47916666530105090, -3.861377020970580443 ) ) ;
#57968=CARTESIAN_POINT ( 'NONE',  ( 4.458734124999999437, 10.93750000136559386, -5.460374474430324690E-16 ) ) ;
#57969=CARTESIAN_POINT ( 'NONE',  ( 5.000000000000000000, 11.70833333606451809, -2.886751345948129988 ) ) ;
#57976=CARTESIAN_POINT ( 'NONE',  ( 1.339745962155612702, 19.70534180126147561, -5.000000000000000000 ) ) ;
#57977=CARTESIAN_POINT ( 'NONE',  ( 1.339745962155615144, -19.70534180126147561, 4.999999999999999112 ) ) ;
#57979=CARTESIAN_POINT ( 'NONE',  ( -1.336351044127974539E-14, 24.37500000273118417, 5.000000000000000000 ) ) ;
#57980=CARTESIAN_POINT ( 'NONE',  ( 4.458734124999998549, -21.97916666530107221, -2.574251347313721627 ) ) ;
#57990=ORIENTED_EDGE ( 'NONE', *, *, #20223, .F. ) ;
#57991=CARTESIAN_POINT ( 'NONE',  ( 4.458734125000001214, -68.14583333196773651, 2.574251347313718519 ) ) ;
#57992=CARTESIAN_POINT ( 'NONE',  ( -6.972266317189433020E-16, -82.12499999726881583, -5.000000000000000000 ) ) ;
#57993=DIRECTION ( 'NONE',  ( 0.000000000000000000, 0.000000000000000000, 1.000000000000000000 ) ) ;
#57997=CARTESIAN_POINT ( 'NONE',  ( 4.458734124999999437, 3.937500001365595192, -5.460374474430324690E-16 ) ) ;
#58006=CARTESIAN_POINT ( 'NONE',  ( -4.458734124999999437, -74.31249999863440792, 0.000000000000000000 ) ) ;
#58008=CARTESIAN_POINT ( 'NONE',  ( -3.152548672688508926E-16, 9.437500001365593860, -5.148502694627439702 ) ) ;
#58011=CARTESIAN_POINT ( 'NONE',  ( 4.458734124999999437, -60.06249999863440081, -5.460374474430324690E-16 ) ) ;
#58012=CARTESIAN_POINT ( 'NONE',  ( -2.500000000000000444, -19.04166666393547658, -4.330127018922193649 ) ) ;
#58014=DIRECTION ( 'NONE',  ( -0.000000000000000000, 1.000000000000000000, -0.000000000000000000 ) ) ;
#58015=CARTESIAN_POINT ( 'NONE',  ( -1.339745962155610925, -58.79465819873852439, 5.000000000000000000 ) ) ;
#58016=CARTESIAN_POINT ( 'NONE',  ( -4.458734124999999437, -41.39583333196773651, -2.574251347313719407 ) ) ;
#58017=CARTESIAN_POINT ( 'NONE',  ( 2.229367062500001939, -29.22916666530107221, 3.861377020970579999 ) ) ;
#58019=CARTESIAN_POINT ( 'NONE',  ( -5.000000000000000000, 24.00000000000000000, 0.000000000000000000 ) ) ;
#58021=CARTESIAN_POINT ( 'NONE',  ( 2.229367062499998831, -106.8958333319677365, -3.861377020970580887 ) ) ;
#58022=CARTESIAN_POINT ( 'NONE',  ( -3.152548672688508926E-16, -32.56249999863440792, -5.148502694627439702 ) ) ;
#58023=CARTESIAN_POINT ( 'NONE',  ( 2.499999999999998668, -67.20833333060214443, -4.330127018922193649 ) ) ;
#58026=CARTESIAN_POINT ( 'NONE',  ( -2.229367062499996610, -77.39583333196773651, 3.861377020970582219 ) ) ;
#58029=CYLINDRICAL_SURFACE ( 'NONE', #60575, 5.000000000000000000 ) ;
#58030=CARTESIAN_POINT ( 'NONE',  ( -2.499999999999996447, -19.83333333333333570, 4.330127018922195425 ) ) ;
#58034=CARTESIAN_POINT ( 'NONE',  ( 2.500000000000002220, -16.54166666393548368, 4.330127018922192761 ) ) ;
#58036=CARTESIAN_POINT ( 'NONE',  ( -2.500000000000000444, 26.95833333606451632, -4.330127018922193649 ) ) ;
#58037=CARTESIAN_POINT ( 'NONE',  ( 5.000000000000000000, 4.625000002731187720, -6.123233995736766282E-16 ) ) ;
#58043=CARTESIAN_POINT ( 'NONE',  ( -4.999999999999998224, -76.91666666666667140, 2.886751345948131764 ) ) ;
#58046=ORIENTED_EDGE ( 'NONE', *, *, #5012, .T. ) ;
#58047=CARTESIAN_POINT ( 'NONE',  ( 5.000000000000000000, -97.29166666393547303, -2.886751345948130876 ) ) ;
#58051=ORIENTED_EDGE ( 'NONE', *, *, #62887, .F. ) ;
#58053=ORIENTED_EDGE ( 'NONE', *, *, #26206, .F. ) ;
#58056=CARTESIAN_POINT ( 'NONE',  ( 1.975475456537005874E-15, -102.6249999972688158, 5.000000000000000000 ) ) ;
#58058=VERTEX_POINT ( 'NONE', #63476 ) ;
#58059=CARTESIAN_POINT ( 'NONE',  ( -5.000000000000000000, -38.95833333060214443, -2.886751345948128211 ) ) ;
#58064=CARTESIAN_POINT ( 'NONE',  ( 9.457646018065525792E-16, -80.06249999863439371, 5.148502694627439702 ) ) ;
#58065=CARTESIAN_POINT ( 'NONE',  ( -4.458734124999999437, 21.68750000136559208, 0.000000000000000000 ) ) ;
#58066=CARTESIAN_POINT ( 'NONE',  ( -2.500000000000000444, -18.04166666393547658, -4.330127018922193649 ) ) ;
#58070=CARTESIAN_POINT ( 'NONE',  ( 1.339745962155615144, -74.58034179853031276, 4.999999999999999112 ) ) ;
#58073=CARTESIAN_POINT ( 'NONE',  ( 2.229367062499998831, -57.64583333196773651, -3.861377020970580887 ) ) ;
#58074=CARTESIAN_POINT ( 'NONE',  ( 1.339745962155615144, 10.29465819873852084, 4.999999999999999112 ) ) ;
#58075=CARTESIAN_POINT ( 'NONE',  ( -2.229367062500000163, 24.52083333469892779, -3.861377020970580443 ) ) ;
#58076=ADVANCED_FACE ( 'NONE', ( #43206 ), #48660, .T. ) ;
#58080=CARTESIAN_POINT ( 'NONE',  ( -4.458734124999999437, -43.64583333196774362, -2.574251347313719407 ) ) ;
#58081=CARTESIAN_POINT ( 'NONE',  ( -5.000000000000000000, -2.874999997268815832, 0.000000000000000000 ) ) ;
#58084=CARTESIAN_POINT ( 'NONE',  ( 2.229367062499998831, -106.6458333319677365, -3.861377020970580887 ) ) ;
#58085=CARTESIAN_POINT ( 'NONE',  ( 2.229367062499998831, -10.89583333196773829, -3.861377020970580887 ) ) ;
#58088=CARTESIAN_POINT ( 'NONE',  ( 4.458734124999999437, -100.8124999986344079, -5.460374474430324690E-16 ) ) ;
#58090=CARTESIAN_POINT ( 'NONE',  ( 2.229367062500001939, -92.22916666530106511, 3.861377020970579999 ) ) ;
#58091=CARTESIAN_POINT ( 'NONE',  ( 1.060575238724906964E-15, -54.62499999726880873, 5.773502691896257311 ) ) ;
#58094=ADVANCED_FACE ( 'NONE', ( #4601 ), #28423, .T. ) ;
#58096=CARTESIAN_POINT ( 'NONE',  ( -2.229367062500000163, -10.47916666530106866, -3.861377020970580443 ) ) ;
#58097=CARTESIAN_POINT ( 'NONE',  ( -2.229367062499996610, 11.60416666803225993, 3.861377020970582219 ) ) ;
#58098=ADVANCED_FACE ( 'NONE', ( #4298 ), #38691, .T. ) ;
#58099=CARTESIAN_POINT ( 'NONE',  ( 4.458734125000000326, -60.14583333196774362, 2.574251347313718519 ) ) ;
#58100=CARTESIAN_POINT ( 'NONE',  ( -1.339745962155613812, -69.20534180126148271, -5.000000000000000000 ) ) ;
#58102=CARTESIAN_POINT ( 'NONE',  ( 1.975475456537005874E-15, -106.6249999972687874, 5.000000000000000000 ) ) ;
#58103=ORIENTED_EDGE ( 'NONE', *, *, #23608, .T. ) ;
#58108=CARTESIAN_POINT ( 'NONE',  ( -2.499999999999996447, -24.83333333333333215, 4.330127018922195425 ) ) ;
#58109=CARTESIAN_POINT ( 'NONE',  ( 2.229367062499998831, -83.64583333196773651, -3.861377020970580887 ) ) ;
#58110=CARTESIAN_POINT ( 'NONE',  ( -3.152548672688508926E-16, 17.18750000136559919, -5.148502694627439702 ) ) ;
#58115=CARTESIAN_POINT ( 'NONE',  ( 1.060575238724906964E-15, -71.75000000000000000, 5.773502691896257311 ) ) ;
#58118=CARTESIAN_POINT ( 'NONE',  ( 5.000000000000000888, -79.58333333333332860, 2.886751345948126879 ) ) ;
#58119=ORIENTED_EDGE ( 'NONE', *, *, #32997, .T. ) ;
#58121=CARTESIAN_POINT ( 'NONE',  ( 1.975475456537005874E-15, -70.75000000000000000, 5.000000000000000000 ) ) ;
#58125=EDGE_CURVE ( 'NONE', #62202, #57126, #40443, .T. ) ;
#58127=ORIENTED_EDGE ( 'NONE', *, *, #49085, .F. ) ;
#58133=CARTESIAN_POINT ( 'NONE',  ( -4.458734124999998549, -58.47916666530106511, 2.574251347313722516 ) ) ;
#58136=EDGE_LOOP ( 'NONE', ( #43735, #923, #35749, #52540 ) ) ;
#58143=CARTESIAN_POINT ( 'NONE',  ( -2.229367062500000163, -103.7291666653010651, -3.861377020970580443 ) ) ;
#58148=CARTESIAN_POINT ( 'NONE',  ( -4.458734124999997661, -40.22916666530107932, 2.574251347313722516 ) ) ;
#58149=DIRECTION ( 'NONE',  ( -0.000000000000000000, 1.000000000000000000, -0.000000000000000000 ) ) ;
#58151=CARTESIAN_POINT ( 'NONE',  ( 2.229367062500001939, -13.97916666530107221, 3.861377020970579999 ) ) ;
#58152=CARTESIAN_POINT ( 'NONE',  ( 2.229367062499998831, -100.8958333319677365, -3.861377020970580887 ) ) ;
#58154=CARTESIAN_POINT ( 'NONE',  ( -3.152548672688508926E-16, -26.81249999863440436, -5.148502694627439702 ) ) ;
#58158=CARTESIAN_POINT ( 'NONE',  ( -4.999999999999998224, -90.91666666666665719, 2.886751345948131764 ) ) ;
#58161=CARTESIAN_POINT ( 'NONE',  ( -2.229367062500000163, 3.270833334698929118, -3.861377020970580443 ) ) ;
#58163=MECHANICAL_DESIGN_GEOMETRIC_PRESENTATION_REPRESENTATION('',(#36743),#53023);
#58166=CARTESIAN_POINT ( 'NONE',  ( -2.500000000000000444, -95.16666666666667140, -4.330127018922193649 ) ) ;
#58167=CARTESIAN_POINT ( 'NONE',  ( 9.457646018065525792E-16, -30.06249999863440081, 5.148502694627439702 ) ) ;
#58168=CARTESIAN_POINT ( 'NONE',  ( 0.000000000000000000, -120.0000000000000000, 5.000000000000000000 ) ) ;
#58169=CARTESIAN_POINT ( 'NONE',  ( -2.229367062499996610, -77.39583333196773651, 3.861377020970582219 ) ) ;
#58175=CARTESIAN_POINT ( 'NONE',  ( 9.457646018065525792E-16, 1.937500001365593416, 5.148502694627439702 ) ) ;
#58176=CARTESIAN_POINT ( 'NONE',  ( 4.458734124999998549, 29.02083333469893134, -2.574251347313721627 ) ) ;
#58177=EDGE_CURVE ( 'NONE', #4805, #11153, #63553, .T. ) ;
#58178=CARTESIAN_POINT ( 'NONE',  ( -4.458734124999999437, -41.64583333196773651, -2.574251347313719407 ) ) ;
#58179=CARTESIAN_POINT ( 'NONE',  ( -5.000000000000000000, -3.874999997268816720, 0.000000000000000000 ) ) ;
#58181=EDGE_CURVE ( 'NONE', #47937, #26829, #17159, .T. ) ;
#58184=CARTESIAN_POINT ( 'NONE',  ( -2.229367062500000163, -69.47916666530107932, -3.861377020970580443 ) ) ;
#58185=CARTESIAN_POINT ( 'NONE',  ( -3.535250795749689387E-16, -103.1249999972688300, -5.773502691896257311 ) ) ;
#58186=( BOUNDED_CURVE ( )  B_SPLINE_CURVE ( 2, ( #13152, #61743, #3511, #36650, #17968, #2565, #32772, #27937, #41782 ),
 .UNSPECIFIED., .F., .F. ) 
 B_SPLINE_CURVE_WITH_KNOTS ( ( 3, 2, 2, 2, 3 ),
 ( 0.6910714285714285587, 0.6916666666666666519, 0.6928571428571428381, 0.6940476190476190244, 0.6946428571428571175 ),
 .UNSPECIFIED. ) 
 CURVE ( )  GEOMETRIC_REPRESENTATION_ITEM ( )  RATIONAL_B_SPLINE_CURVE ( ( 0.9330127018922194093, 0.9330127018922194093, 1.000000000000000000, 0.8660254037844387076, 1.000000000000000000, 0.8660254037844387076, 1.000000000000000000, 0.9330127018922194093, 0.9330127018922194093 ) ) 
 REPRESENTATION_ITEM ( '' )  );
#58188=CARTESIAN_POINT ( 'NONE',  ( 4.458734125000000326, -108.1458333319677365, 2.574251347313718519 ) ) ;
#58190=CARTESIAN_POINT ( 'NONE',  ( 1.060575238724906964E-15, -51.75000000000000711, 5.773502691896257311 ) ) ;
#58193=ORIENTED_EDGE ( 'NONE', *, *, #49558, .T. ) ;
#58195=CARTESIAN_POINT ( 'NONE',  ( 5.000000000000000888, -27.45833333060214798, 2.886751345948126879 ) ) ;
#58198=EDGE_CURVE ( 'NONE', #51032, #33480, #50016, .T. ) ;
#58205=CARTESIAN_POINT ( 'NONE',  ( 2.500000000000002220, -98.66666666666665719, 4.330127018922192761 ) ) ;
#58207=ORIENTED_EDGE ( 'NONE', *, *, #31958, .T. ) ;
#58211=CARTESIAN_POINT ( 'NONE',  ( 4.458734124999998549, -41.97916666530107932, -2.574251347313721627 ) ) ;
#58212=CARTESIAN_POINT ( 'NONE',  ( 0.000000000000000000, -120.0000000000000000, 0.000000000000000000 ) ) ;
#58216=VECTOR ( 'NONE', #57744, 1000.000000000000000 ) ;
#58218=AXIS2_PLACEMENT_3D ( 'NONE', #51393, #42354, #32070 ) ;
#58220=CARTESIAN_POINT ( 'NONE',  ( -5.000000000000000000, -24.95833333060214443, -2.886751345948128211 ) ) ;
#58222=CARTESIAN_POINT ( 'NONE',  ( -2.229367062499996610, -91.39583333196773651, 3.861377020970582219 ) ) ;
#58223=CARTESIAN_POINT ( 'NONE',  ( 5.000000000000000888, -34.45833333060213732, 2.886751345948126879 ) ) ;
#58224=VERTEX_POINT ( 'NONE', #34834 ) ;
#58225=CARTESIAN_POINT ( 'NONE',  ( -6.972266317189433020E-16, -33.12499999726880873, -5.000000000000000000 ) ) ;
#58227=CARTESIAN_POINT ( 'NONE',  ( 1.339745962155615144, -43.70534180126147561, 4.999999999999999112 ) ) ;
#58228=ORIENTED_EDGE ( 'NONE', *, *, #50321, .F. ) ;
#58230=EDGE_CURVE ( 'NONE', #54554, #56173, #26558, .T. ) ;
#58232=CARTESIAN_POINT ( 'NONE',  ( 2.229367062499998831, -13.89583333196774184, -3.861377020970580887 ) ) ;
#58238=CARTESIAN_POINT ( 'NONE',  ( -2.229367062500000163, 19.27083333469892779, -3.861377020970580443 ) ) ;
#58239=ORIENTED_EDGE ( 'NONE', *, *, #27108, .T. ) ;
#58240=CARTESIAN_POINT ( 'NONE',  ( -3.152548672688508926E-16, -92.56249999863439371, -5.148502694627439702 ) ) ;
#58241=CARTESIAN_POINT ( 'NONE',  ( -1.339745962155613812, -34.08034179853029144, -5.000000000000000000 ) ) ;
#58242=DIRECTION ( 'NONE',  ( -0.000000000000000000, 1.000000000000000000, -0.000000000000000000 ) ) ;
#58243=CARTESIAN_POINT ( 'NONE',  ( -2.229367062499996610, -15.14583333196773474, 3.861377020970582219 ) ) ;
#58244=EDGE_CURVE ( 'NONE', #62968, #20764, #48330, .T. ) ;
#58245=FACE_OUTER_BOUND ( 'NONE', #14383, .T. ) ;
#58246=EDGE_CURVE ( 'NONE', #29631, #9470, #53262, .T. ) ;
#58249=CARTESIAN_POINT ( 'NONE',  ( -2.500000000000000444, -39.04166666393548013, -4.330127018922193649 ) ) ;
#58250=CARTESIAN_POINT ( 'NONE',  ( 2.499999999999998668, -29.33333333333332860, -4.330127018922193649 ) ) ;
#58251=CARTESIAN_POINT ( 'NONE',  ( -4.458734124999997661, 17.77083333469892779, 2.574251347313722516 ) ) ;
#58253=EDGE_CURVE ( 'NONE', #56396, #54905, #54534, .T. ) ;
#58254=ORIENTED_EDGE ( 'NONE', *, *, #30207, .F. ) ;
#58257=CARTESIAN_POINT ( 'NONE',  ( -4.458734124999999437, -64.31249999863440792, 0.000000000000000000 ) ) ;
#58260=DIRECTION ( 'NONE',  ( -0.000000000000000000, 1.000000000000000000, -0.000000000000000000 ) ) ;
#58261=CARTESIAN_POINT ( 'NONE',  ( 1.060575238724906964E-15, 10.24999999999999822, 5.773502691896257311 ) ) ;
#58266=CARTESIAN_POINT ( 'NONE',  ( -4.458734124999999437, -55.39583333196773651, -2.574251347313719407 ) ) ;
#58267=CARTESIAN_POINT ( 'NONE',  ( 5.000000000000000000, -83.37499999726881583, -6.123233995736766282E-16 ) ) ;
#58268=VECTOR ( 'NONE', #47878, 1000.000000000000000 ) ;
#58271=CARTESIAN_POINT ( 'NONE',  ( 0.000000000000000000, -120.0000000000000000, 0.000000000000000000 ) ) ;
#58272=CARTESIAN_POINT ( 'NONE',  ( -6.972266317189433020E-16, -105.1249999972687874, -5.000000000000000000 ) ) ;
#58274=CARTESIAN_POINT ( 'NONE',  ( -4.458734124999999437, -89.56249999863440792, 0.000000000000000000 ) ) ;
#58276=CARTESIAN_POINT ( 'NONE',  ( -2.500000000000000444, -37.16666666666666430, -4.330127018922193649 ) ) ;
#58279=EDGE_LOOP ( 'NONE', ( #35266, #53725, #49329, #44990 ) ) ;
#58280=CARTESIAN_POINT ( 'NONE',  ( -2.229367062500000163, -101.4791666653010651, -3.861377020970580443 ) ) ;
#58281=CARTESIAN_POINT ( 'NONE',  ( -2.229367062500000163, 9.270833334698927786, -3.861377020970580443 ) ) ;
#58282=CARTESIAN_POINT ( 'NONE',  ( 1.060575238724906964E-15, 12.37500000273118417, 5.773502691896257311 ) ) ;
#58286=CARTESIAN_POINT ( 'NONE',  ( -6.972266317189433020E-16, -32.24999999999999289, -5.000000000000000000 ) ) ;
#58295=CARTESIAN_POINT ( 'NONE',  ( 2.229367062499998831, -26.89583333196774007, -3.861377020970580887 ) ) ;
#58304=ORIENTED_EDGE ( 'NONE', *, *, #10239, .T. ) ;
#58305=CARTESIAN_POINT ( 'NONE',  ( -4.458734124999999437, -70.56249999863439371, 0.000000000000000000 ) ) ;
#58313=CARTESIAN_POINT ( 'NONE',  ( 4.458734124999999437, -1.062499998634405696, -5.460374474430324690E-16 ) ) ;
#58314=VERTEX_POINT ( 'NONE', #25255 ) ;
#58315=DIRECTION ( 'NONE',  ( -0.000000000000000000, 1.000000000000000000, -0.000000000000000000 ) ) ;
#58318=CARTESIAN_POINT ( 'NONE',  ( 5.000000000000000000, 16.58333333333333215, -2.886751345948130876 ) ) ;
#58320=EDGE_LOOP ( 'NONE', ( #25581, #46807, #13401, #61149 ) ) ;
#58321=CARTESIAN_POINT ( 'NONE',  ( -4.458734124999999437, -73.39583333196772230, -2.574251347313719407 ) ) ;
#58323=CARTESIAN_POINT ( 'NONE',  ( 4.458734124999999437, 4.187500001365595637, -5.460374474430324690E-16 ) ) ;
#58325=CARTESIAN_POINT ( 'NONE',  ( 4.458734124999999437, -68.06249999863440792, -5.460374474430324690E-16 ) ) ;
#58326=CARTESIAN_POINT ( 'NONE',  ( 5.000000000000000000, -25.29166666393547658, -2.886751345948129988 ) ) ;
#58331=EDGE_CURVE ( 'NONE', #30770, #21697, #37633, .T. ) ;
#58332=CARTESIAN_POINT ( 'NONE',  ( -3.152548672688508926E-16, -42.56249999863440792, -5.148502694627439702 ) ) ;
#58333=CARTESIAN_POINT ( 'NONE',  ( -2.229367062499996610, -24.39583333196773651, 3.861377020970582219 ) ) ;
#58336=CARTESIAN_POINT ( 'NONE',  ( 5.000000000000000000, 24.50000000000000000, -6.123233995736766282E-16 ) ) ;
#58338=CARTESIAN_POINT ( 'NONE',  ( -2.499999999999996447, -49.83333333333332860, 4.330127018922195425 ) ) ;
#58339=CARTESIAN_POINT ( 'NONE',  ( 4.458734124999999437, -35.81249999863440792, -5.460374474430324690E-16 ) ) ;
#58340=CARTESIAN_POINT ( 'NONE',  ( 5.000000000000000000, -66.37499999726881583, -6.123233995736766282E-16 ) ) ;
#58344=CARTESIAN_POINT ( 'NONE',  ( -2.229367062500000163, -74.72916666530106511, -3.861377020970580443 ) ) ;
#58347=CARTESIAN_POINT ( 'NONE',  ( 1.975475456537005874E-15, -27.62499999726881228, 5.000000000000000000 ) ) ;
#58349=CARTESIAN_POINT ( 'NONE',  ( -2.500000000000000444, -22.16666666666666785, -4.330127018922193649 ) ) ;
#58351=ORIENTED_EDGE ( 'NONE', *, *, #58951, .F. ) ;
#58355=VECTOR ( 'NONE', #50643, 1000.000000000000000 ) ;
#58356=CARTESIAN_POINT ( 'NONE',  ( 5.000000000000000000, 28.70833333606451987, -2.886751345948129988 ) ) ;
#58366=CARTESIAN_POINT ( 'NONE',  ( 9.457646018065525792E-16, -19.06249999863440792, 5.148502694627439702 ) ) ;
#58369=AXIS2_PLACEMENT_3D ( 'NONE', #47486, #56843, #7949 ) ;
#58374=FACE_OUTER_BOUND ( 'NONE', #24025, .T. ) ;
#58375=CARTESIAN_POINT ( 'NONE',  ( -5.000000000000000000, -3.083333333333333925, -2.886751345948128211 ) ) ;
#58383=ORIENTED_EDGE ( 'NONE', *, *, #55429, .T. ) ;
#58384=( BOUNDED_CURVE ( )  B_SPLINE_CURVE ( 2, ( #46637, #31840, #27019, #2583, #56620, #17052, #21564, #50829, #12536 ),
 .UNSPECIFIED., .F., .F. ) 
 B_SPLINE_CURVE_WITH_KNOTS ( ( 3, 2, 2, 2, 3 ),
 ( 0.3875000000000000111, 0.3880952380952381042, 0.3892857142857142905, 0.3904761904761904767, 0.3910714285714285698 ),
 .UNSPECIFIED. ) 
 CURVE ( )  GEOMETRIC_REPRESENTATION_ITEM ( )  RATIONAL_B_SPLINE_CURVE ( ( 0.9330127018922194093, 0.9330127018922194093, 1.000000000000000000, 0.8660254037844387076, 1.000000000000000000, 0.8660254037844387076, 1.000000000000000000, 0.9330127018922194093, 0.9330127018922194093 ) ) 
 REPRESENTATION_ITEM ( '' )  );
#58386=LINE ( 'NONE', #49035, #20339 ) ;
#58387=CARTESIAN_POINT ( 'NONE',  ( 4.458734124999999437, 21.18750000136559208, -5.460374474430324690E-16 ) ) ;
#58394=CARTESIAN_POINT ( 'NONE',  ( -4.458734124999999437, -59.31249999863440081, 0.000000000000000000 ) ) ;
#58396=CARTESIAN_POINT ( 'NONE',  ( 4.458734124999999437, 21.18750000136559208, -5.460374474430324690E-16 ) ) ;
#58397=AXIS2_PLACEMENT_3D ( 'NONE', #58212, #43101, #62431 ) ;
#58398=CARTESIAN_POINT ( 'NONE',  ( 5.000000000000000888, -102.4583333306021586, 2.886751345948126879 ) ) ;
#58400=CARTESIAN_POINT ( 'NONE',  ( 4.458734125000001214, -50.14583333196773651, 2.574251347313718519 ) ) ;
#58401=CARTESIAN_POINT ( 'NONE',  ( 2.500000000000002220, -3.541666663935478354, 4.330127018922192761 ) ) ;
#58403=DIRECTION ( 'NONE',  ( 0.000000000000000000, 0.000000000000000000, 1.000000000000000000 ) ) ;
#58405=CARTESIAN_POINT ( 'NONE',  ( 9.457646018065525792E-16, -108.0624999986343937, 5.148502694627439702 ) ) ;
#58406=CARTESIAN_POINT ( 'NONE',  ( 9.457646018065525792E-16, -13.31249999863440259, 5.148502694627439702 ) ) ;
#58409=CARTESIAN_POINT ( 'NONE',  ( 2.229367062499998831, -100.6458333319677365, -3.861377020970580887 ) ) ;
#58411=CARTESIAN_POINT ( 'NONE',  ( 4.458734124999999437, -90.06249999863440792, -5.460374474430324690E-16 ) ) ;
#58413=CARTESIAN_POINT ( 'NONE',  ( 5.000000000000000000, -50.37499999726881583, -6.123233995736766282E-16 ) ) ;
#58414=CARTESIAN_POINT ( 'NONE',  ( -2.500000000000000444, -37.04166666393548013, -4.330127018922193649 ) ) ;
#58418=CARTESIAN_POINT ( 'NONE',  ( 4.458734124999998549, -18.72916666530106866, -2.574251347313721627 ) ) ;
#58419=CARTESIAN_POINT ( 'NONE',  ( -3.152548672688508926E-16, 12.18750000136559564, -5.148502694627439702 ) ) ;
#58420=CARTESIAN_POINT ( 'NONE',  ( 2.229367062499998831, -57.89583333196773651, -3.861377020970580887 ) ) ;
#58427=CARTESIAN_POINT ( 'NONE',  ( -1.339745962155610925, -37.79465819873851729, 5.000000000000000000 ) ) ;
#58429=CARTESIAN_POINT ( 'NONE',  ( -3.152548672688508926E-16, -85.56249999863439371, -5.148502694627439702 ) ) ;
#58430=CARTESIAN_POINT ( 'NONE',  ( -4.458734124999999437, 20.43750000136559208, 0.000000000000000000 ) ) ;
#58432=CARTESIAN_POINT ( 'NONE',  ( -1.339745962155610925, -88.66965819600733312, 5.000000000000000000 ) ) ;
#58435=CARTESIAN_POINT ( 'NONE',  ( 2.500000000000002220, -69.66666666666667140, 4.330127018922192761 ) ) ;
#58436=( BOUNDED_CURVE ( )  B_SPLINE_CURVE ( 2, ( #15984, #5384, #35609, #25955, #15352, #54592, #20178, #1528, #21132 ),
 .UNSPECIFIED., .F., .F. ) 
 B_SPLINE_CURVE_WITH_KNOTS ( ( 3, 2, 2, 2, 3 ),
 ( 0.06607142857142857262, 0.06666666666666666574, 0.06785714285714285199, 0.06904761904761905211, 0.06964285714285714524 ),
 .UNSPECIFIED. ) 
 CURVE ( )  GEOMETRIC_REPRESENTATION_ITEM ( )  RATIONAL_B_SPLINE_CURVE ( ( 0.9330127018922194093, 0.9330127018922194093, 1.000000000000000000, 0.8660254037844387076, 1.000000000000000000, 0.8660254037844387076, 1.000000000000000000, 0.9330127018922194093, 0.9330127018922194093 ) ) 
 REPRESENTATION_ITEM ( '' )  );
#58439=CARTESIAN_POINT ( 'NONE',  ( 1.339745962155612702, -79.29465819873851729, -5.000000000000000000 ) ) ;
#58440=VERTEX_POINT ( 'NONE', #55810 ) ;
#58456=LINE ( 'NONE', #53626, #10414 ) ;
#58457=CARTESIAN_POINT ( 'NONE',  ( 4.458734124999998549, -57.97916666530107221, -2.574251347313721627 ) ) ;
#58459=CARTESIAN_POINT ( 'NONE',  ( 5.000000000000000000, 3.708333336064517649, -2.886751345948130876 ) ) ;
#58465=CARTESIAN_POINT ( 'NONE',  ( 2.229367062499998831, -106.8958333319677365, -3.861377020970580887 ) ) ;
#58467=ORIENTED_EDGE ( 'NONE', *, *, #18156, .T. ) ;
#58470=CARTESIAN_POINT ( 'NONE',  ( 2.229367062499998831, -40.64583333196773651, -3.861377020970580887 ) ) ;
#58473=CARTESIAN_POINT ( 'NONE',  ( -2.229367062499996610, -12.14583333196774007, 3.861377020970582219 ) ) ;
#58474=CARTESIAN_POINT ( 'NONE',  ( 4.458734124999999437, -101.0624999986344079, -5.460374474430324690E-16 ) ) ;
#58475=ORIENTED_EDGE ( 'NONE', *, *, #29547, .F. ) ;
#58477=CARTESIAN_POINT ( 'NONE',  ( 2.229367062499998831, -28.89583333196774007, -3.861377020970580887 ) ) ;
#58482=DIRECTION ( 'NONE',  ( -0.000000000000000000, 1.000000000000000000, -0.000000000000000000 ) ) ;
#58485=CARTESIAN_POINT ( 'NONE',  ( -2.229367062499996610, 6.604166668032259935, 3.861377020970582219 ) ) ;
#58489=CARTESIAN_POINT ( 'NONE',  ( -3.535250795749689387E-16, -98.25000000000000000, -5.773502691896257311 ) ) ;
#58490=CARTESIAN_POINT ( 'NONE',  ( -4.458734124999999437, -32.31249999863440792, 0.000000000000000000 ) ) ;
#58492=CARTESIAN_POINT ( 'NONE',  ( 2.229367062500001939, -74.22916666530106511, 3.861377020970579999 ) ) ;
#58497=CARTESIAN_POINT ( 'NONE',  ( 2.229367062499998831, 0.3541666680322609340, -3.861377020970580887 ) ) ;
#58498=CARTESIAN_POINT ( 'NONE',  ( -3.152548672688508926E-16, 25.18750000136558853, -5.148502694627439702 ) ) ;
#58499=CARTESIAN_POINT ( 'NONE',  ( 2.229367062500001939, -44.22916666530106511, 3.861377020970579999 ) ) ;
#58502=EDGE_LOOP ( 'NONE', ( #55547, #63450, #53231, #4946 ) ) ;
#58504=CARTESIAN_POINT ( 'NONE',  ( 9.457646018065525792E-16, -72.06249999863439371, 5.148502694627439702 ) ) ;
#58505=CARTESIAN_POINT ( 'NONE',  ( 1.060575238724906964E-15, -103.6249999972688158, 5.773502691896257311 ) ) ;
#58507=CARTESIAN_POINT ( 'NONE',  ( -5.000000000000000000, -64.00000000000000000, 0.000000000000000000 ) ) ;
#58508=CARTESIAN_POINT ( 'NONE',  ( -4.458734124999999437, -110.5624999986343937, 0.000000000000000000 ) ) ;
#58510=CARTESIAN_POINT ( 'NONE',  ( 2.499999999999998668, -52.33333333333332860, -4.330127018922193649 ) ) ;
#58511=CARTESIAN_POINT ( 'NONE',  ( 1.975475456537005874E-15, -65.74999999999998579, 5.000000000000000000 ) ) ;
#58514=CARTESIAN_POINT ( 'NONE',  ( -5.000000000000000000, -27.08333333333333215, -2.886751345948128211 ) ) ;
#58523=ORIENTED_EDGE ( 'NONE', *, *, #62536, .T. ) ;
#58531=CARTESIAN_POINT ( 'NONE',  ( -4.458734124999999437, -39.64583333196774362, -2.574251347313719407 ) ) ;
#58532=CARTESIAN_POINT ( 'NONE',  ( 1.975475456537005874E-15, -10.75000000000000000, 5.000000000000000000 ) ) ;
#58534=EDGE_CURVE ( 'NONE', #44207, #8918, #35231, .T. ) ;
#58540=CARTESIAN_POINT ( 'NONE',  ( -6.972266317189433020E-16, -89.24999999999998579, -5.000000000000000000 ) ) ;
#58543=CARTESIAN_POINT ( 'NONE',  ( -2.229367062499996610, -87.39583333196773651, 3.861377020970582219 ) ) ;
#58546=CARTESIAN_POINT ( 'NONE',  ( -1.975475456537005874E-15, 27.37500000273118417, 5.000000000000000000 ) ) ;
#58547=DIRECTION ( 'NONE',  ( -0.000000000000000000, 1.000000000000000000, -0.000000000000000000 ) ) ;
#58549=LINE ( 'NONE', #34091, #51723 ) ;
#58550=ORIENTED_EDGE ( 'NONE', *, *, #62179, .F. ) ;
#58553=CARTESIAN_POINT ( 'NONE',  ( -2.229367062499996610, -13.39583333196774007, 3.861377020970582219 ) ) ;
#58554=CARTESIAN_POINT ( 'NONE',  ( 5.000000000000000888, -105.4583333306021444, 2.886751345948126879 ) ) ;
#58556=CARTESIAN_POINT ( 'NONE',  ( -1.339745962155610925, 4.330341803992665106, 5.000000000000000000 ) ) ;
#58558=CARTESIAN_POINT ( 'NONE',  ( -4.458734124999997661, 21.52083333469893134, 2.574251347313722516 ) ) ;
#58560=CARTESIAN_POINT ( 'NONE',  ( 4.458734124999998549, -93.72916666530105090, -2.574251347313721627 ) ) ;
#58563=CARTESIAN_POINT ( 'NONE',  ( 4.458734125000001214, -15.89583333196773651, 2.574251347313718519 ) ) ;
#58565=FACE_OUTER_BOUND ( 'NONE', #31580, .T. ) ;
#58568=EDGE_CURVE ( 'NONE', #49961, #47640, #18142, .T. ) ;
#58569=CARTESIAN_POINT ( 'NONE',  ( 2.499999999999998668, -41.20833333060214443, -4.330127018922193649 ) ) ;
#58571=CARTESIAN_POINT ( 'NONE',  ( 4.458734125000000326, 18.10416666803225993, 2.574251347313718519 ) ) ;
#58575=CARTESIAN_POINT ( 'NONE',  ( -2.229367062499996610, -62.14583333196774362, 3.861377020970582219 ) ) ;
#58578=CARTESIAN_POINT ( 'NONE',  ( 5.000000000000000888, 8.416666666666666075, 2.886751345948126879 ) ) ;
#58580=CARTESIAN_POINT ( 'NONE',  ( -2.500000000000000444, -99.04166666393545881, -4.330127018922193649 ) ) ;
#58581=AXIS2_PLACEMENT_3D ( 'NONE', #7435, #32173, #7748 ) ;
#58582=CARTESIAN_POINT ( 'NONE',  ( 4.458734124999998549, -54.72916666530107932, -2.574251347313721627 ) ) ;
#58583=CARTESIAN_POINT ( 'NONE',  ( -2.500000000000000444, -91.04166666393547303, -4.330127018922193649 ) ) ;
#58584=CARTESIAN_POINT ( 'NONE',  ( -6.972266317189433020E-16, 21.75000000000000000, -5.000000000000000000 ) ) ;
#58586=CARTESIAN_POINT ( 'NONE',  ( 1.339745962155611592, 25.41965820146970501, 5.000000000000000888 ) ) ;
#58587=DIRECTION ( 'NONE',  ( -0.000000000000000000, 1.000000000000000000, -0.000000000000000000 ) ) ;
#58589=CARTESIAN_POINT ( 'NONE',  ( 2.500000000000002220, -39.66666666666667140, 4.330127018922192761 ) ) ;
#58590=CARTESIAN_POINT ( 'NONE',  ( 5.000000000000000888, -98.45833333060213022, 2.886751345948126879 ) ) ;
#58591=CARTESIAN_POINT ( 'NONE',  ( 1.975475456537005874E-15, 15.37500000273118417, 5.000000000000000000 ) ) ;
#58593=CARTESIAN_POINT ( 'NONE',  ( 4.458734124999998549, -101.7291666653010793, -2.574251347313721627 ) ) ;
#58594=CARTESIAN_POINT ( 'NONE',  ( 9.457646018065525792E-16, 4.687500001365596525, 5.148502694627439702 ) ) ;
#58600=EDGE_CURVE ( 'NONE', #26022, #55695, #6463, .T. ) ;
#58606=CARTESIAN_POINT ( 'NONE',  ( -5.000000000000000000, 24.91666666666666785, -2.886751345948128211 ) ) ;
#58608=CARTESIAN_POINT ( 'NONE',  ( 2.229367062500001939, -23.22916666530107221, 3.861377020970579999 ) ) ;
#58609=DIRECTION ( 'NONE',  ( -0.000000000000000000, 1.000000000000000000, -0.000000000000000000 ) ) ;
#58617=ORIENTED_EDGE ( 'NONE', *, *, #19949, .F. ) ;
#58619=EDGE_CURVE ( 'NONE', #17564, #35972, #39303, .T. ) ;
#58621=CARTESIAN_POINT ( 'NONE',  ( 2.229367062500001939, -75.22916666530106511, 3.861377020970579999 ) ) ;
#58622=CARTESIAN_POINT ( 'NONE',  ( -5.000000000000000000, 28.99999999999999645, 0.000000000000000000 ) ) ;
#58623=VERTEX_POINT ( 'NONE', #46156 ) ;
#58624=VECTOR ( 'NONE', #14569, 1000.000000000000000 ) ;
#58625=CARTESIAN_POINT ( 'NONE',  ( 1.975475456537005874E-15, -106.6249999972687874, 5.000000000000000000 ) ) ;
#58627=CARTESIAN_POINT ( 'NONE',  ( 9.457646018065525792E-16, 3.687500001365594748, 5.148502694627439702 ) ) ;
#58630=CARTESIAN_POINT ( 'NONE',  ( -1.339745962155613368, 28.91965820146970501, -5.000000000000000000 ) ) ;
#58637=CARTESIAN_POINT ( 'NONE',  ( -4.458734124999999437, -76.39583333196773651, -2.574251347313719407 ) ) ;
#58639=CARTESIAN_POINT ( 'NONE',  ( -4.458734124999998549, 3.770833334698929562, 2.574251347313722516 ) ) ;
#58640=CARTESIAN_POINT ( 'NONE',  ( -2.499999999999996447, -42.70833333060214443, 4.330127018922195425 ) ) ;
#58641=CARTESIAN_POINT ( 'NONE',  ( 2.229367062499998831, -65.89583333196773651, -3.861377020970580887 ) ) ;
#58642=CARTESIAN_POINT ( 'NONE',  ( -4.999999999999999112, -22.79166666393548013, 2.886751345948131764 ) ) ;
#58644=CARTESIAN_POINT ( 'NONE',  ( 1.339745962155615144, -44.58034179853027723, 4.999999999999999112 ) ) ;
#58646=CARTESIAN_POINT ( 'NONE',  ( -2.229367062499996610, -46.14583333196774362, 3.861377020970582219 ) ) ;
#58647=CARTESIAN_POINT ( 'NONE',  ( -3.152548672688508926E-16, -24.81249999863440436, -5.148502694627439702 ) ) ;
#58649=CARTESIAN_POINT ( 'NONE',  ( -2.500000000000000444, 25.83333333333333215, -4.330127018922193649 ) ) ;
#58651=CARTESIAN_POINT ( 'NONE',  ( -5.000000000000000000, -50.08333333333332860, -2.886751345948128211 ) ) ;
#58652=CARTESIAN_POINT ( 'NONE',  ( 4.458734124999999437, -39.81249999863440081, -5.460374474430324690E-16 ) ) ;
#58653=CARTESIAN_POINT ( 'NONE',  ( -5.000000000000000000, -72.95833333060214443, -2.886751345948128211 ) ) ;
#58656=CARTESIAN_POINT ( 'NONE',  ( -4.458734124999997661, -74.47916666530106511, 2.574251347313722516 ) ) ;
#58661=CARTESIAN_POINT ( 'NONE',  ( -5.000000000000000000, -24.00000000000000000, 0.000000000000000000 ) ) ;
#58667=CARTESIAN_POINT ( 'NONE',  ( 2.499999999999998668, 28.79166666939784847, -4.330127018922193649 ) ) ;
#58674=CARTESIAN_POINT ( 'NONE',  ( 1.975475456537005874E-15, 0.2500000000000001665, 5.000000000000000000 ) ) ;
#58676=CARTESIAN_POINT ( 'NONE',  ( -1.339745962155613812, 4.794658198738519950, -5.000000000000000000 ) ) ;
#58677=CARTESIAN_POINT ( 'NONE',  ( 4.458734124999998549, -22.72916666530107221, -2.574251347313721627 ) ) ;
#58685=DIRECTION ( 'NONE',  ( -0.000000000000000000, 1.000000000000000000, -0.000000000000000000 ) ) ;
#58688=EDGE_CURVE ( 'NONE', #46066, #2855, #22672, .T. ) ;
#58691=CARTESIAN_POINT ( 'NONE',  ( 2.500000000000002220, -23.54166666393548368, 4.330127018922192761 ) ) ;
#58697=CARTESIAN_POINT ( 'NONE',  ( -2.229367062499996610, 19.85416666803225993, 3.861377020970582219 ) ) ;
#58698=DIRECTION ( 'NONE',  ( 0.000000000000000000, 0.000000000000000000, 1.000000000000000000 ) ) ;
#58703=CARTESIAN_POINT ( 'NONE',  ( 5.000000000000000000, -100.4166666666666572, -2.886751345948130876 ) ) ;
#58705=CARTESIAN_POINT ( 'NONE',  ( 4.458734124999998549, -59.72916666530106511, -2.574251347313721627 ) ) ;
#58708=CARTESIAN_POINT ( 'NONE',  ( -2.229367062499996610, 15.85416666803226171, 3.861377020970582219 ) ) ;
#58710=CARTESIAN_POINT ( 'NONE',  ( 2.229367062499998831, -49.89583333196772941, -3.861377020970580887 ) ) ;
#58711=CARTESIAN_POINT ( 'NONE',  ( 5.000000000000000888, -9.458333330602144429, 2.886751345948126879 ) ) ;
#58712=CARTESIAN_POINT ( 'NONE',  ( -5.000000000000000000, -93.00000000000000000, 0.000000000000000000 ) ) ;
#58714=DIRECTION ( 'NONE',  ( 0.000000000000000000, 0.000000000000000000, 1.000000000000000000 ) ) ;
#58715=CARTESIAN_POINT ( 'NONE',  ( -2.229367062500000163, -109.4791666653010651, -3.861377020970580443 ) ) ;
#58716=CARTESIAN_POINT ( 'NONE',  ( 9.457646018065525792E-16, -12.31249999863440259, 5.148502694627439702 ) ) ;
#58717=VERTEX_POINT ( 'NONE', #31989 ) ;
#58719=CARTESIAN_POINT ( 'NONE',  ( -4.458734124999998549, -96.22916666530106511, 2.574251347313722516 ) ) ;
#58721=CARTESIAN_POINT ( 'NONE',  ( -2.229367062500000163, -97.72916666530105090, -3.861377020970580443 ) ) ;
#58723=CARTESIAN_POINT ( 'NONE',  ( 5.000000000000000000, -50.29166666393548013, -2.886751345948129988 ) ) ;
#58727=CARTESIAN_POINT ( 'NONE',  ( 4.458734124999999437, -20.81249999863440081, -5.460374474430324690E-16 ) ) ;
#58728=CARTESIAN_POINT ( 'NONE',  ( 4.458734125000001214, 4.854166668032262599, 2.574251347313718519 ) ) ;
#58729=CARTESIAN_POINT ( 'NONE',  ( 4.458734125000000326, -57.14583333196773651, 2.574251347313718519 ) ) ;
#58734=CARTESIAN_POINT ( 'NONE',  ( 1.060575238724906964E-15, -8.750000000000000000, 5.773502691896257311 ) ) ;
#58740=CARTESIAN_POINT ( 'NONE',  ( 4.458734125000001214, -83.89583333196773651, 2.574251347313718519 ) ) ;
#58741=CARTESIAN_POINT ( 'NONE',  ( -4.458734124999999437, 18.35416666803225993, -2.574251347313719407 ) ) ;
#58743=CARTESIAN_POINT ( 'NONE',  ( 2.499999999999998668, -0.3333333333333348136, -4.330127018922193649 ) ) ;
#58746=CARTESIAN_POINT ( 'NONE',  ( -5.000000000000000000, -75.08333333333332860, -2.886751345948128211 ) ) ;
#58748=VERTEX_POINT ( 'NONE', #7557 ) ;
#58750=ORIENTED_EDGE ( 'NONE', *, *, #16773, .F. ) ;
#58761=ORIENTED_EDGE ( 'NONE', *, *, #18161, .F. ) ;
#58763=CARTESIAN_POINT ( 'NONE',  ( 1.975475456537005874E-15, -103.7500000000000000, 5.000000000000000000 ) ) ;
#58764=CARTESIAN_POINT ( 'NONE',  ( -4.458734124999999437, -58.64583333196774362, -2.574251347313719407 ) ) ;
#58766=CARTESIAN_POINT ( 'NONE',  ( 1.339745962155586056, 3.419658201469704562, 5.000000000000015987 ) ) ;
#58767=VERTEX_POINT ( 'NONE', #2732 ) ;
#58773=CARTESIAN_POINT ( 'NONE',  ( -2.229367062500000163, -107.7291666653010651, -3.861377020970580443 ) ) ;
#58774=VERTEX_POINT ( 'NONE', #19073 ) ;
#58777=CARTESIAN_POINT ( 'NONE',  ( -2.229367062499996610, -40.14583333196773651, 3.861377020970582219 ) ) ;
#58781=CARTESIAN_POINT ( 'NONE',  ( -4.458734124999999437, -10.31249999863440792, 0.000000000000000000 ) ) ;
#58782=CARTESIAN_POINT ( 'NONE',  ( -4.458734124999997661, -99.47916666530105090, 2.574251347313722516 ) ) ;
#58785=CARTESIAN_POINT ( 'NONE',  ( 4.458734125000001214, -36.14583333196773651, 2.574251347313718519 ) ) ;
#58786=CARTESIAN_POINT ( 'NONE',  ( 2.500000000000002220, 7.458333336064517205, 4.330127018922192761 ) ) ;
#58787=CARTESIAN_POINT ( 'NONE',  ( -5.000000000000000000, 11.91666666666666607, -2.886751345948128211 ) ) ;
#58793=CARTESIAN_POINT ( 'NONE',  ( -4.458734124999999437, 5.354166668032261711, -2.574251347313719407 ) ) ;
#58794=ORIENTED_EDGE ( 'NONE', *, *, #4010, .F. ) ;
#58795=DIRECTION ( 'NONE',  ( -0.000000000000000000, 1.000000000000000000, -0.000000000000000000 ) ) ;
#58796=CARTESIAN_POINT ( 'NONE',  ( 5.000000000000000000, -94.41666666666665719, -2.886751345948129988 ) ) ;
#58797=CARTESIAN_POINT ( 'NONE',  ( -4.458734124999998549, -28.22916666530106866, 2.574251347313722516 ) ) ;
#58798=CARTESIAN_POINT ( 'NONE',  ( -2.499999999999996447, -22.70833333060214443, 4.330127018922195425 ) ) ;
#58799=CARTESIAN_POINT ( 'NONE',  ( -2.229367062500000163, -79.72916666530106511, -3.861377020970580443 ) ) ;
#58803=CARTESIAN_POINT ( 'NONE',  ( 4.458734124999998549, -1.729166665301068440, -2.574251347313721627 ) ) ;
#58804=CARTESIAN_POINT ( 'NONE',  ( 9.457646018065525792E-16, 24.68750000136559208, 5.148502694627439702 ) ) ;
#58805=CARTESIAN_POINT ( 'NONE',  ( 4.458734124999999437, -42.06249999863440081, -5.460374474430324690E-16 ) ) ;
#58806=( BOUNDED_CURVE ( )  B_SPLINE_CURVE ( 2, ( #25869, #36474, #35206, #31005, #55144, #5615, #35845, #50311, #16222 ),
 .UNSPECIFIED., .F., .F. ) 
 B_SPLINE_CURVE_WITH_KNOTS ( ( 3, 2, 2, 2, 3 ),
 ( 0.3660714285714285476, 0.3666666666666666408, 0.3678571428571428825, 0.3690476190476190688, 0.3696428571428571619 ),
 .UNSPECIFIED. ) 
 CURVE ( )  GEOMETRIC_REPRESENTATION_ITEM ( )  RATIONAL_B_SPLINE_CURVE ( ( 0.9330127018922194093, 0.9330127018922194093, 1.000000000000000000, 0.8660254037844387076, 1.000000000000000000, 0.8660254037844387076, 1.000000000000000000, 0.9330127018922194093, 0.9330127018922194093 ) ) 
 REPRESENTATION_ITEM ( '' )  );
#58807=CARTESIAN_POINT ( 'NONE',  ( -1.339745962155610925, -45.66965819600733312, 5.000000000000000000 ) ) ;
#58811=( BOUNDED_CURVE ( )  B_SPLINE_CURVE ( 2, ( #17465, #31611, #51247, #47044, #32239, #51868, #7811, #18078, #18400 ),
 .UNSPECIFIED., .F., .F. ) 
 B_SPLINE_CURVE_WITH_KNOTS ( ( 3, 2, 2, 2, 3 ),
 ( 0.4732142857142856984, 0.4738095238095237915, 0.4749999999999999778, 0.4761904761904761640, 0.4767857142857143127 ),
 .UNSPECIFIED. ) 
 CURVE ( )  GEOMETRIC_REPRESENTATION_ITEM ( )  RATIONAL_B_SPLINE_CURVE ( ( 0.9330127018922194093, 0.9330127018922194093, 1.000000000000000000, 0.8660254037844387076, 1.000000000000000000, 0.8660254037844387076, 1.000000000000000000, 0.9330127018922163007, 0.9330127018922194093 ) ) 
 REPRESENTATION_ITEM ( '' )  );
#58812=CARTESIAN_POINT ( 'NONE',  ( 9.457646018065525792E-16, -67.06249999863440792, 5.148502694627439702 ) ) ;
#58813=CARTESIAN_POINT ( 'NONE',  ( 5.000000000000000888, -106.4583333306021586, 2.886751345948126879 ) ) ;
#58815=CARTESIAN_POINT ( 'NONE',  ( 6.158835246850667461E-14, 9.749999999999996447, -4.999999999999999112 ) ) ;
#58816=PLANE ( 'NONE',  #13177 ) ;
#58818=CARTESIAN_POINT ( 'NONE',  ( 5.000000000000000000, -60.50000000000000000, -6.123233995736766282E-16 ) ) ;
#58819=DIRECTION ( 'NONE',  ( 0.000000000000000000, 0.000000000000000000, 1.000000000000000000 ) ) ;
#58823=CARTESIAN_POINT ( 'NONE',  ( 3.044556291839386294E-14, 12.75000000000000000, -5.000000000000000000 ) ) ;
#58830=VERTEX_POINT ( 'NONE', #62850 ) ;
#58831=CARTESIAN_POINT ( 'NONE',  ( 0.000000000000000000, -120.0000000000000000, 5.000000000000000000 ) ) ;
#58834=ORIENTED_EDGE ( 'NONE', *, *, #13111, .T. ) ;
#58835=( BOUNDED_CURVE ( )  B_SPLINE_CURVE ( 2, ( #26408, #35423, #60833, #15807, #51184, #7116, #49887, #46346, #59561 ),
 .UNSPECIFIED., .F., .F. ) 
 B_SPLINE_CURVE_WITH_KNOTS ( ( 3, 2, 2, 2, 3 ),
 ( 0.3982142857142857428, 0.3988095238095238360, 0.4000000000000000222, 0.4011904761904762085, 0.4017857142857143016 ),
 .UNSPECIFIED. ) 
 CURVE ( )  GEOMETRIC_REPRESENTATION_ITEM ( )  RATIONAL_B_SPLINE_CURVE ( ( 0.9330127018922194093, 0.9330127018922225179, 1.000000000000000000, 0.8660254037844387076, 1.000000000000000000, 0.8660254037844387076, 1.000000000000000000, 0.9330127018922194093, 0.9330127018922194093 ) ) 
 REPRESENTATION_ITEM ( '' )  );
#58839=CARTESIAN_POINT ( 'NONE',  ( 4.458734125000001214, -42.14583333196773651, 2.574251347313718519 ) ) ;
#58840=CARTESIAN_POINT ( 'NONE',  ( 1.975475456537005874E-15, -39.75000000000000000, 5.000000000000000000 ) ) ;
#58848=CARTESIAN_POINT ( 'NONE',  ( 2.229367062500001939, -88.22916666530107932, 3.861377020970579999 ) ) ;
#58851=DIRECTION ( 'NONE',  ( 0.000000000000000000, -1.000000000000000000, 0.000000000000000000 ) ) ;
#58854=( BOUNDED_CURVE ( )  B_SPLINE_CURVE ( 2, ( #50533, #44733, #693, #35416, #26084, #39906, #30906, #15486, #54723 ),
 .UNSPECIFIED., .F., .F. ) 
 B_SPLINE_CURVE_WITH_KNOTS ( ( 3, 2, 2, 2, 3 ),
 ( 0.2517857142857142794, 0.2523809523809523725, 0.2535714285714285587, 0.2547619047619047450, 0.2553571428571428381 ),
 .UNSPECIFIED. ) 
 CURVE ( )  GEOMETRIC_REPRESENTATION_ITEM ( )  RATIONAL_B_SPLINE_CURVE ( ( 0.9330127018922194093, 0.9330127018922194093, 1.000000000000000000, 0.8660254037844387076, 1.000000000000000000, 0.8660254037844387076, 1.000000000000000000, 0.9330127018922194093, 0.9330127018922194093 ) ) 
 REPRESENTATION_ITEM ( '' )  );
#58855=CARTESIAN_POINT ( 'NONE',  ( 5.000000000000000000, -38.49999999999999289, -6.123233995736766282E-16 ) ) ;
#58856=ORIENTED_EDGE ( 'NONE', *, *, #61532, .T. ) ;
#58857=CARTESIAN_POINT ( 'NONE',  ( -4.458734124999999437, 0.6041666680322611560, -2.574251347313719407 ) ) ;
#58859=CARTESIAN_POINT ( 'NONE',  ( 4.458734124999998549, -15.97916666530107221, -2.574251347313721627 ) ) ;
#58862=CARTESIAN_POINT ( 'NONE',  ( 0.000000000000000000, -120.0000000000000000, 5.000000000000000000 ) ) ;
#58864=CARTESIAN_POINT ( 'NONE',  ( 4.458734125000000326, 18.85416666803225993, 2.574251347313718519 ) ) ;
#58866=CARTESIAN_POINT ( 'NONE',  ( -2.229367062499996610, -96.14583333196773651, 3.861377020970582219 ) ) ;
#58868=CYLINDRICAL_SURFACE ( 'NONE', #21627, 5.000000000000000000 ) ;
#58869=CARTESIAN_POINT ( 'NONE',  ( -4.458734124999999437, -13.39583333196774184, -2.574251347313719407 ) ) ;
#58870=EDGE_CURVE ( 'NONE', #57924, #50850, #38694, .T. ) ;
#58874=CARTESIAN_POINT ( 'NONE',  ( 5.000000000000000888, -41.45833333060213732, 2.886751345948126879 ) ) ;
#58875=CARTESIAN_POINT ( 'NONE',  ( 4.458734124999999437, 16.18750000136559564, -5.460374474430324690E-16 ) ) ;
#58879=CARTESIAN_POINT ( 'NONE',  ( 4.458734124999998549, -60.72916666530106511, -2.574251347313721627 ) ) ;
#58883=CARTESIAN_POINT ( 'NONE',  ( 5.000000000000000000, 5.500000000000001776, -6.123233995736766282E-16 ) ) ;
#58885=CYLINDRICAL_SURFACE ( 'NONE', #10965, 5.000000000000000000 ) ;
#58886=CARTESIAN_POINT ( 'NONE',  ( -4.458734124999998549, -52.22916666530106511, 2.574251347313722516 ) ) ;
#58887=CARTESIAN_POINT ( 'NONE',  ( -4.999999999999999112, -87.79166666393550145, 2.886751345948131764 ) ) ;
#58888=CARTESIAN_POINT ( 'NONE',  ( -4.458734124999999437, -34.39583333196772941, -2.574251347313719407 ) ) ;
#58889=CARTESIAN_POINT ( 'NONE',  ( 1.339745962155615144, -14.58034179853029322, 4.999999999999999112 ) ) ;
#58893=EDGE_CURVE ( 'NONE', #28617, #41864, #32752, .T. ) ;
#58895=CARTESIAN_POINT ( 'NONE',  ( 5.000000000000000000, -40.41666666666667140, -2.886751345948129988 ) ) ;
#58896=CARTESIAN_POINT ( 'NONE',  ( -1.339745962155610925, -19.66965819600733667, 5.000000000000000000 ) ) ;
#58897=CARTESIAN_POINT ( 'NONE',  ( 1.975475456537005874E-15, -22.74999999999999645, 5.000000000000000000 ) ) ;
#58899=CARTESIAN_POINT ( 'NONE',  ( -4.458734124999999437, -103.3124999986344079, 0.000000000000000000 ) ) ;
#58900=CARTESIAN_POINT ( 'NONE',  ( -4.458734124999999437, 5.354166668032262599, -2.574251347313719407 ) ) ;
#58909=ORIENTED_EDGE ( 'NONE', *, *, #8583, .T. ) ;
#58912=CARTESIAN_POINT ( 'NONE',  ( 5.000000000000000000, -20.49999999999999645, -6.123233995736766282E-16 ) ) ;
#58915=CARTESIAN_POINT ( 'NONE',  ( 2.229367062499998831, -24.89583333196773651, -3.861377020970580887 ) ) ;
#58927=CARTESIAN_POINT ( 'NONE',  ( 4.458734124999999437, -71.06249999863439371, -5.460374474430324690E-16 ) ) ;
#58928=CARTESIAN_POINT ( 'NONE',  ( 3.253724281355068545E-15, 28.75000000000000000, -5.000000000000000000 ) ) ;
#58932=CARTESIAN_POINT ( 'NONE',  ( 1.339745962155615144, -31.58034179853029499, 4.999999999999999112 ) ) ;
#58934=CARTESIAN_POINT ( 'NONE',  ( -4.458734124999999437, 1.354166668032261933, -2.574251347313719407 ) ) ;
#58937=FACE_OUTER_BOUND ( 'NONE', #28574, .T. ) ;
#58942=EDGE_LOOP ( 'NONE', ( #24104, #49675, #34960, #13200 ) ) ;
#58943=CARTESIAN_POINT ( 'NONE',  ( 9.457646018065525792E-16, -82.06249999863440792, 5.148502694627439702 ) ) ;
#58945=CARTESIAN_POINT ( 'NONE',  ( 4.458734124999999437, 0.1875000013655953035, -5.460374474430324690E-16 ) ) ;
#58947=AXIS2_PLACEMENT_3D ( 'NONE', #22096, #1858, #35617 ) ;
#58949=CARTESIAN_POINT ( 'NONE',  ( -5.000000000000000000, -83.08333333333332860, -2.886751345948128211 ) ) ;
#58950=CARTESIAN_POINT ( 'NONE',  ( 6.123233995736766282E-16, -120.0000000000000000, -5.000000000000000000 ) ) ;
#58951=EDGE_CURVE ( 'NONE', #53159, #8589, #50410, .T. ) ;
#58952=CARTESIAN_POINT ( 'NONE',  ( -4.458734124999999437, -63.56249999863440792, 0.000000000000000000 ) ) ;
#58953=CARTESIAN_POINT ( 'NONE',  ( 5.000000000000000000, -24.29166666393548368, -2.886751345948129988 ) ) ;
#58955=CARTESIAN_POINT ( 'NONE',  ( 4.458734124999998549, 29.27083333469893134, -2.574251347313721627 ) ) ;
#58958=CARTESIAN_POINT ( 'NONE',  ( -4.458734124999999437, -48.39583333196772941, -2.574251347313719407 ) ) ;
#58960=CARTESIAN_POINT ( 'NONE',  ( 9.457646018065525792E-16, -31.31249999863440436, 5.148502694627439702 ) ) ;
#58963=CARTESIAN_POINT ( 'NONE',  ( -2.500000000000000444, 24.83333333333333215, -4.330127018922193649 ) ) ;
#58965=LINE ( 'NONE', #15549, #57228 ) ;
#58966=CARTESIAN_POINT ( 'NONE',  ( -3.152548672688508926E-16, -36.56249999863441502, -5.148502694627439702 ) ) ;
#58967=CARTESIAN_POINT ( 'NONE',  ( -5.000000000000000000, -74.95833333060214443, -2.886751345948128211 ) ) ;
#58970=LINE ( 'NONE', #11032, #61410 ) ;
#58971=EDGE_CURVE ( 'NONE', #21496, #36016, #44208, .T. ) ;
#58972=CARTESIAN_POINT ( 'NONE',  ( 4.458734125000000326, -75.14583333196775072, 2.574251347313718519 ) ) ;
#58976=CARTESIAN_POINT ( 'NONE',  ( -6.972266317189433020E-16, -65.24999999999998579, -5.000000000000000000 ) ) ;
#58977=CARTESIAN_POINT ( 'NONE',  ( 5.000000000000000000, -22.50000000000000000, -6.123233995736766282E-16 ) ) ;
#58979=ORIENTED_EDGE ( 'NONE', *, *, #55522, .T. ) ;
#58981=VERTEX_POINT ( 'NONE', #24923 ) ;
#58983=CARTESIAN_POINT ( 'NONE',  ( -4.999999999999999112, 22.20833333606451987, 2.886751345948131764 ) ) ;
#58989=CARTESIAN_POINT ( 'NONE',  ( 2.493747252781420335E-13, -77.25000000000001421, -5.000000000000000000 ) ) ;
#58993=CARTESIAN_POINT ( 'NONE',  ( 4.458734125000001214, -18.89583333196773651, 2.574251347313718519 ) ) ;
#58994=LINE ( 'NONE', #14923, #28595 ) ;
#59004=CARTESIAN_POINT ( 'NONE',  ( -2.500000000000000444, -68.04166666393547303, -4.330127018922193649 ) ) ;
#59006=ORIENTED_EDGE ( 'NONE', *, *, #60235, .F. ) ;
#59007=( BOUNDED_CURVE ( )  B_SPLINE_CURVE ( 2, ( #26458, #46076, #39962, #59610, #11019, #15541, #35161, #54776, #10708 ),
 .UNSPECIFIED., .F., .F. ) 
 B_SPLINE_CURVE_WITH_KNOTS ( ( 3, 2, 2, 2, 3 ),
 ( 0.9946428571428571619, 0.9952380952380952550, 0.9964285714285714413, 0.9976190476190476275, 0.9982142857142857206 ),
 .UNSPECIFIED. ) 
 CURVE ( )  GEOMETRIC_REPRESENTATION_ITEM ( )  RATIONAL_B_SPLINE_CURVE ( ( 0.9330127018922194093, 0.9330127018922194093, 1.000000000000000000, 0.8660254037844387076, 1.000000000000000000, 0.8660254037844387076, 1.000000000000000000, 0.9330127018922194093, 0.9330127018922194093 ) ) 
 REPRESENTATION_ITEM ( '' )  );
#59011=ORIENTED_EDGE ( 'NONE', *, *, #12202, .T. ) ;
#59013=CARTESIAN_POINT ( 'NONE',  ( -3.152548672688508926E-16, 17.43750000136559564, -5.148502694627439702 ) ) ;
#59021=CARTESIAN_POINT ( 'NONE',  ( 4.458734125000000326, -60.89583333196774362, 2.574251347313718519 ) ) ;
#59023=CARTESIAN_POINT ( 'NONE',  ( -4.458734124999999437, 18.60416666803225993, -2.574251347313719407 ) ) ;
#59024=DIRECTION ( 'NONE',  ( 0.000000000000000000, 0.000000000000000000, 1.000000000000000000 ) ) ;
#59025=EDGE_CURVE ( 'NONE', #49354, #1660, #58386, .T. ) ;
#59027=CARTESIAN_POINT ( 'NONE',  ( -4.458734124999998549, -51.47916666530106511, 2.574251347313722516 ) ) ;
#59028=CARTESIAN_POINT ( 'NONE',  ( 5.000000000000000000, -8.374999997268814056, -6.123233995736766282E-16 ) ) ;
#59031=CYLINDRICAL_SURFACE ( 'NONE', #42787, 5.000000000000000000 ) ;
#59033=CARTESIAN_POINT ( 'NONE',  ( 2.229367062500001939, -108.9791666653010651, 3.861377020970579999 ) ) ;
#59035=CARTESIAN_POINT ( 'NONE',  ( 9.457646018065525792E-16, -14.31249999863440614, 5.148502694627439702 ) ) ;
#59036=ORIENTED_EDGE ( 'NONE', *, *, #3135, .F. ) ;
#59038=CARTESIAN_POINT ( 'NONE',  ( -3.152548672688508926E-16, -97.56249999863440792, -5.148502694627439702 ) ) ;
#59040=CARTESIAN_POINT ( 'NONE',  ( -2.229367062500000163, -99.72916666530106511, -3.861377020970580443 ) ) ;
#59042=CARTESIAN_POINT ( 'NONE',  ( -4.999999999999999112, -54.79166666393547303, 2.886751345948131764 ) ) ;
#59043=EDGE_CURVE ( 'NONE', #60943, #19776, #25238, .T. ) ;
#59044=LINE ( 'NONE', #52645, #63373 ) ;
#59045=EDGE_CURVE ( 'NONE', #62028, #6651, #20420, .T. ) ;
#59049=CARTESIAN_POINT ( 'NONE',  ( 4.458734125000000326, -18.89583333196774362, 2.574251347313718519 ) ) ;
#59050=CARTESIAN_POINT ( 'NONE',  ( -4.458734124999999437, 7.354166668032259935, -2.574251347313719407 ) ) ;
#59051=CARTESIAN_POINT ( 'NONE',  ( 4.458734124999998549, -57.97916666530107932, -2.574251347313721627 ) ) ;
#59052=LINE ( 'NONE', #11111, #44910 ) ;
#59056=CARTESIAN_POINT ( 'NONE',  ( 1.060575238724906964E-15, -5.749999999999998224, 5.773502691896257311 ) ) ;
#59058=EDGE_LOOP ( 'NONE', ( #56129, #50463, #9966, #51935 ) ) ;
#59060=CARTESIAN_POINT ( 'NONE',  ( 1.339745962155619807, 21.83034180399265978, -4.999999999999996447 ) ) ;
#59065=CARTESIAN_POINT ( 'NONE',  ( -2.229367062499996610, -85.14583333196773651, 3.861377020970582219 ) ) ;
#59066=CARTESIAN_POINT ( 'NONE',  ( -3.152548672688508926E-16, 19.18750000136559208, -5.148502694627439702 ) ) ;
#59068=CARTESIAN_POINT ( 'NONE',  ( -6.972266317189433020E-16, -93.24999999999998579, -5.000000000000000000 ) ) ;
#59072=CARTESIAN_POINT ( 'NONE',  ( 5.000000000000000000, -73.50000000000000000, -6.123233995736766282E-16 ) ) ;
#59075=LINE ( 'NONE', #34613, #41775 ) ;
#59086=ORIENTED_EDGE ( 'NONE', *, *, #48459, .F. ) ;
#59089=CARTESIAN_POINT ( 'NONE',  ( -3.152548672688508926E-16, -55.81249999863440081, -5.148502694627439702 ) ) ;
#59096=ORIENTED_EDGE ( 'NONE', *, *, #27600, .F. ) ;
#59099=CARTESIAN_POINT ( 'NONE',  ( -3.152548672688508926E-16, -105.8124999986344079, -5.148502694627439702 ) ) ;
#59101=ORIENTED_EDGE ( 'NONE', *, *, #47645, .F. ) ;
#59105=CARTESIAN_POINT ( 'NONE',  ( 9.457646018065525792E-16, -45.06249999863440081, 5.148502694627439702 ) ) ;
#59108=CYLINDRICAL_SURFACE ( 'NONE', #52208, 5.000000000000000000 ) ;
#59109=CARTESIAN_POINT ( 'NONE',  ( 4.458734125000001214, -12.89583333196774184, 2.574251347313718519 ) ) ;
#59110=CARTESIAN_POINT ( 'NONE',  ( -5.000000000000000000, -102.0833333333333286, -2.886751345948128211 ) ) ;
#59111=VERTEX_POINT ( 'NONE', #26844 ) ;
#59113=CARTESIAN_POINT ( 'NONE',  ( -4.458734124999999437, -34.64583333196773651, -2.574251347313719407 ) ) ;
#59114=CARTESIAN_POINT ( 'NONE',  ( 5.000000000000000888, 7.541666669397851130, 2.886751345948126879 ) ) ;
#59115=CARTESIAN_POINT ( 'NONE',  ( 1.339745962155615144, -50.70534180126148271, 4.999999999999999112 ) ) ;
#59120=DIRECTION ( 'NONE',  ( 0.000000000000000000, 0.000000000000000000, 1.000000000000000000 ) ) ;
#59121=CARTESIAN_POINT ( 'NONE',  ( -3.152548672688508926E-16, 5.187500001365592972, -5.148502694627439702 ) ) ;
#59123=CARTESIAN_POINT ( 'NONE',  ( 1.339745962155627135, 16.83034180399266688, -4.999999999999991118 ) ) ;
#59125=CARTESIAN_POINT ( 'NONE',  ( 1.060575238724906964E-15, -96.75000000000001421, 5.773502691896257311 ) ) ;
#59126=CARTESIAN_POINT ( 'NONE',  ( -4.458734124999998549, -30.22916666530106866, 2.574251347313722516 ) ) ;
#59127=DIRECTION ( 'NONE',  ( 0.000000000000000000, 0.000000000000000000, 1.000000000000000000 ) ) ;
#59128=CARTESIAN_POINT ( 'NONE',  ( -4.458734124999999437, -79.64583333196772230, -2.574251347313719407 ) ) ;
#59130=CARTESIAN_POINT ( 'NONE',  ( 0.000000000000000000, -120.0000000000000000, 5.000000000000000000 ) ) ;
#59132=CARTESIAN_POINT ( 'NONE',  ( -4.458734124999999437, -2.395833331967737845, -2.574251347313719407 ) ) ;
#59133=CARTESIAN_POINT ( 'NONE',  ( 4.458734124999999437, 20.93750000136559208, -5.460374474430324690E-16 ) ) ;
#59134=CARTESIAN_POINT ( 'NONE',  ( -2.229367062499996610, -40.39583333196773651, 3.861377020970582219 ) ) ;
#59137=ORIENTED_EDGE ( 'NONE', *, *, #34729, .F. ) ;
#59139=CARTESIAN_POINT ( 'NONE',  ( 2.229367062499998831, -67.64583333196773651, -3.861377020970580887 ) ) ;
#59140=CARTESIAN_POINT ( 'NONE',  ( 2.500000000000002220, -106.5416666639354730, 4.330127018922192761 ) ) ;
#59141=( BOUNDED_CURVE ( )  B_SPLINE_CURVE ( 2, ( #41311, #41947, #7246, #22981, #12687, #7555, #61272, #2416, #13319 ),
 .UNSPECIFIED., .F., .F. ) 
 B_SPLINE_CURVE_WITH_KNOTS ( ( 3, 2, 2, 2, 3 ),
 ( 0.9267857142857143238, 0.9273809523809524169, 0.9285714285714286031, 0.9297619047619047894, 0.9303571428571428825 ),
 .UNSPECIFIED. ) 
 CURVE ( )  GEOMETRIC_REPRESENTATION_ITEM ( )  RATIONAL_B_SPLINE_CURVE ( ( 0.9330127018922194093, 0.9330127018922194093, 1.000000000000000000, 0.8660254037844387076, 1.000000000000000000, 0.8660254037844387076, 1.000000000000000000, 0.9330127018922194093, 0.9330127018922194093 ) ) 
 REPRESENTATION_ITEM ( '' )  );
#59143=EDGE_CURVE ( 'NONE', #23270, #16611, #41378, .T. ) ;
#59144=CARTESIAN_POINT ( 'NONE',  ( 5.000000000000000000, -58.29166666393548013, -2.886751345948130876 ) ) ;
#59145=CARTESIAN_POINT ( 'NONE',  ( 1.975475456537005874E-15, -14.74999999999999822, 5.000000000000000000 ) ) ;
#59147=CARTESIAN_POINT ( 'NONE',  ( -2.499999999999996447, -58.83333333333333570, 4.330127018922195425 ) ) ;
#59148=CARTESIAN_POINT ( 'NONE',  ( -6.972266317189433020E-16, -66.24999999999998579, -5.000000000000000000 ) ) ;
#59150=EDGE_LOOP ( 'NONE', ( #56496, #15311, #39281, #40760 ) ) ;
#59160=CARTESIAN_POINT ( 'NONE',  ( 1.339745962155612702, -35.16965819600734022, -5.000000000000000000 ) ) ;
#59161=CARTESIAN_POINT ( 'NONE',  ( 0.000000000000000000, -120.0000000000000000, 5.000000000000000000 ) ) ;
#59163=ORIENTED_EDGE ( 'NONE', *, *, #2887, .F. ) ;
#59167=CARTESIAN_POINT ( 'NONE',  ( 2.229367062500001939, -41.22916666530107932, 3.861377020970579999 ) ) ;
#59168=CARTESIAN_POINT ( 'NONE',  ( -1.339745962155613812, -16.08034179853029499, -5.000000000000000000 ) ) ;
#59174=CARTESIAN_POINT ( 'NONE',  ( 5.000000000000000000, -89.41666666666665719, -2.886751345948130876 ) ) ;
#59176=CARTESIAN_POINT ( 'NONE',  ( -2.229367062499996610, -89.39583333196773651, 3.861377020970582219 ) ) ;
#59178=ORIENTED_EDGE ( 'NONE', *, *, #12586, .T. ) ;
#59179=CARTESIAN_POINT ( 'NONE',  ( 1.975475456537005874E-15, -31.75000000000000000, 5.000000000000000000 ) ) ;
#59183=CARTESIAN_POINT ( 'NONE',  ( 5.000000000000000000, -82.29166666393547303, -2.886751345948130876 ) ) ;
#59185=VECTOR ( 'NONE', #25049, 1000.000000000000000 ) ;
#59186=CARTESIAN_POINT ( 'NONE',  ( -2.229367062499996610, 4.854166668032261711, 3.861377020970582219 ) ) ;
#59188=CARTESIAN_POINT ( 'NONE',  ( -6.972266317189433020E-16, -1.124999997268814278, -5.000000000000000000 ) ) ;
#59189=CARTESIAN_POINT ( 'NONE',  ( -3.152548672688508926E-16, -18.81249999863440792, -5.148502694627439702 ) ) ;
#59193=CARTESIAN_POINT ( 'NONE',  ( 1.339745962155615144, -55.58034179853028434, 4.999999999999999112 ) ) ;
#59196=CARTESIAN_POINT ( 'NONE',  ( -4.458734124999997661, 20.52083333469892423, 2.574251347313722516 ) ) ;
#59197=ORIENTED_EDGE ( 'NONE', *, *, #15034, .T. ) ;
#59198=CARTESIAN_POINT ( 'NONE',  ( 9.457646018065525792E-16, -97.06249999863439371, 5.148502694627439702 ) ) ;
#59201=CARTESIAN_POINT ( 'NONE',  ( -4.458734124999998549, -13.22916666530107221, 2.574251347313722516 ) ) ;
#59205=CARTESIAN_POINT ( 'NONE',  ( -5.000000000000000000, -40.87499999726880162, 0.000000000000000000 ) ) ;
#59206=CARTESIAN_POINT ( 'NONE',  ( -3.152548672688508926E-16, 13.43750000136559386, -5.148502694627439702 ) ) ;
#59208=FACE_OUTER_BOUND ( 'NONE', #44610, .T. ) ;
#59210=CARTESIAN_POINT ( 'NONE',  ( -4.458734124999999437, -59.39583333196773651, -2.574251347313719407 ) ) ;
#59211=ORIENTED_EDGE ( 'NONE', *, *, #43621, .F. ) ;
#59213=CARTESIAN_POINT ( 'NONE',  ( -4.999999999999999112, 7.083333333333333037, 2.886751345948131764 ) ) ;
#59215=CARTESIAN_POINT ( 'NONE',  ( 2.229367062500001939, -54.97916666530107221, 3.861377020970579999 ) ) ;
#59216=CARTESIAN_POINT ( 'NONE',  ( 5.000000000000000000, -91.37499999726880162, -6.123233995736766282E-16 ) ) ;
#59217=CARTESIAN_POINT ( 'NONE',  ( -4.458734124999997661, -35.22916666530107221, 2.574251347313722516 ) ) ;
#59218=CARTESIAN_POINT ( 'NONE',  ( 0.000000000000000000, -120.0000000000000000, 0.000000000000000000 ) ) ;
#59219=FACE_OUTER_BOUND ( 'NONE', #30373, .T. ) ;
#59222=CARTESIAN_POINT ( 'NONE',  ( 5.000000000000000888, -44.58333333333333570, 2.886751345948126879 ) ) ;
#59226=CARTESIAN_POINT ( 'NONE',  ( 9.457646018065525792E-16, -100.0624999986344221, 5.148502694627439702 ) ) ;
#59227=CARTESIAN_POINT ( 'NONE',  ( -4.458734124999998549, 1.520833334698927342, 2.574251347313722516 ) ) ;
#59236=ORIENTED_EDGE ( 'NONE', *, *, #33494, .F. ) ;
#59240=CARTESIAN_POINT ( 'NONE',  ( 2.229367062500001939, -25.22916666530106866, 3.861377020970579999 ) ) ;
#59243=( BOUNDED_CURVE ( )  B_SPLINE_CURVE ( 2, ( #14212, #4886, #53459, #62503, #9389, #28692, #48311, #13600, #13280 ),
 .UNSPECIFIED., .F., .F. ) 
 B_SPLINE_CURVE_WITH_KNOTS ( ( 3, 2, 2, 2, 3 ),
 ( 0.8482142857142856984, 0.8488095238095237915, 0.8499999999999999778, 0.8511904761904761640, 0.8517857142857142572 ),
 .UNSPECIFIED. ) 
 CURVE ( )  GEOMETRIC_REPRESENTATION_ITEM ( )  RATIONAL_B_SPLINE_CURVE ( ( 0.9330127018922194093, 0.9330127018922194093, 1.000000000000000000, 0.8660254037844387076, 1.000000000000000000, 0.8660254037844387076, 1.000000000000000000, 0.9330127018922194093, 0.9330127018922194093 ) ) 
 REPRESENTATION_ITEM ( '' )  );
#59250=VERTEX_POINT ( 'NONE', #20742 ) ;
#59251=CYLINDRICAL_SURFACE ( 'NONE', #2283, 5.000000000000000000 ) ;
#59253=CARTESIAN_POINT ( 'NONE',  ( -4.458734124999999437, -73.64583333196773651, -2.574251347313719407 ) ) ;
#59254=CYLINDRICAL_SURFACE ( 'NONE', #57450, 5.000000000000000000 ) ;
#59256=EDGE_LOOP ( 'NONE', ( #1205, #12710, #25806, #63555 ) ) ;
#59257=CARTESIAN_POINT ( 'NONE',  ( 2.500000000000002220, 12.33333333333333215, 4.330127018922192761 ) ) ;
#59258=CARTESIAN_POINT ( 'NONE',  ( 2.499999999999998668, -31.20833333060214443, -4.330127018922193649 ) ) ;
#59260=CARTESIAN_POINT ( 'NONE',  ( -2.229367062499996610, -5.395833331967740953, 3.861377020970582219 ) ) ;
#59269=EDGE_LOOP ( 'NONE', ( #46611, #53317, #15584, #29793 ) ) ;
#59270=CARTESIAN_POINT ( 'NONE',  ( 4.458734124999998549, -82.72916666530106511, -2.574251347313721627 ) ) ;
#59271=CARTESIAN_POINT ( 'NONE',  ( 4.458734124999998549, 2.270833334698928230, -2.574251347313721627 ) ) ;
#59273=CARTESIAN_POINT ( 'NONE',  ( 5.000000000000000000, -85.49999999999998579, -6.123233995736766282E-16 ) ) ;
#59275=CARTESIAN_POINT ( 'NONE',  ( 9.457646018065525792E-16, -64.31249999863440792, 5.148502694627439702 ) ) ;
#59276=CARTESIAN_POINT ( 'NONE',  ( -4.999999999999999112, -27.79166666393547658, 2.886751345948131764 ) ) ;
#59278=CARTESIAN_POINT ( 'NONE',  ( -4.458734124999999437, 28.68750000136559208, 0.000000000000000000 ) ) ;
#59279=LINE ( 'NONE', #48354, #18232 ) ;
#59280=FACE_OUTER_BOUND ( 'NONE', #41152, .T. ) ;
#59281=CARTESIAN_POINT ( 'NONE',  ( -4.458734124999998549, -48.22916666530106511, 2.574251347313722516 ) ) ;
#59282=CARTESIAN_POINT ( 'NONE',  ( 9.457646018065525792E-16, -32.31249999863440792, 5.148502694627439702 ) ) ;
#59285=CARTESIAN_POINT ( 'NONE',  ( 5.000000000000000000, 21.50000000000000000, -6.123233995736766282E-16 ) ) ;
#59287=CARTESIAN_POINT ( 'NONE',  ( 1.339745962155615144, -54.58034179853029144, 4.999999999999999112 ) ) ;
#59288=CARTESIAN_POINT ( 'NONE',  ( 2.229367062499998831, -36.64583333196773651, -3.861377020970580887 ) ) ;
#59289=CARTESIAN_POINT ( 'NONE',  ( 2.500000000000002220, -75.54166666393547303, 4.330127018922192761 ) ) ;
#59293=CARTESIAN_POINT ( 'NONE',  ( 4.458734125000000326, -79.14583333196773651, 2.574251347313718519 ) ) ;
#59297=CARTESIAN_POINT ( 'NONE',  ( -3.535250795749689387E-16, -27.24999999999999645, -5.773502691896257311 ) ) ;
#59301=VERTEX_POINT ( 'NONE', #7229 ) ;
#59303=CARTESIAN_POINT ( 'NONE',  ( 5.000000000000000888, 20.54166666939784847, 2.886751345948126879 ) ) ;
#59309=CARTESIAN_POINT ( 'NONE',  ( -2.500000000000000444, -77.16666666666665719, -4.330127018922193649 ) ) ;
#59311=CYLINDRICAL_SURFACE ( 'NONE', #700, 5.000000000000000000 ) ;
#59313=CARTESIAN_POINT ( 'NONE',  ( -4.458734124999999437, -23.31249999863440436, 0.000000000000000000 ) ) ;
#59314=VECTOR ( 'NONE', #55333, 1000.000000000000000 ) ;
#59315=CARTESIAN_POINT ( 'NONE',  ( -1.339745962155610925, -77.66965819600730470, 5.000000000000000000 ) ) ;
#59326=CARTESIAN_POINT ( 'NONE',  ( 2.499999999999998668, -87.33333333333332860, -4.330127018922193649 ) ) ;
#59327=CARTESIAN_POINT ( 'NONE',  ( -6.972266317189433020E-16, -29.25000000000000000, -5.000000000000000000 ) ) ;
#59329=ORIENTED_EDGE ( 'NONE', *, *, #5455, .T. ) ;
#59331=CYLINDRICAL_SURFACE ( 'NONE', #28281, 5.000000000000000000 ) ;
#59333=CYLINDRICAL_SURFACE ( 'NONE', #14907, 5.000000000000000000 ) ;
#59337=CARTESIAN_POINT ( 'NONE',  ( 5.000000000000000000, -103.3749999972688158, -6.123233995736766282E-16 ) ) ;
#59339=CARTESIAN_POINT ( 'NONE',  ( 2.229367062499998831, 11.35416666803225993, -3.861377020970580887 ) ) ;
#59340=ORIENTED_EDGE ( 'NONE', *, *, #23243, .T. ) ;
#59343=CARTESIAN_POINT ( 'NONE',  ( 2.500000000000002220, 12.45833333606451809, 4.330127018922192761 ) ) ;
#59344=CARTESIAN_POINT ( 'NONE',  ( 5.000000000000000888, -39.58333333333333570, 2.886751345948126879 ) ) ;
#59345=CARTESIAN_POINT ( 'NONE',  ( -1.339745962155610925, -102.7946581987385031, 5.000000000000000000 ) ) ;
#59346=CARTESIAN_POINT ( 'NONE',  ( -3.152548672688508926E-16, -67.56249999863440792, -5.148502694627439702 ) ) ;
#59348=CARTESIAN_POINT ( 'NONE',  ( 4.458734124999998549, 18.27083333469893134, -2.574251347313721627 ) ) ;
#59350=CARTESIAN_POINT ( 'NONE',  ( 4.458734124999999437, -49.06249999863440792, -5.460374474430324690E-16 ) ) ;
#59351=CARTESIAN_POINT ( 'NONE',  ( -3.535250795749689387E-16, -7.124999997268813168, -5.773502691896257311 ) ) ;
#59353=CARTESIAN_POINT ( 'NONE',  ( -2.499999999999996447, -73.83333333333332860, 4.330127018922195425 ) ) ;
#59355=CARTESIAN_POINT ( 'NONE',  ( -2.229367062500000163, -17.72916666530106866, -3.861377020970580443 ) ) ;
#59356=VERTEX_POINT ( 'NONE', #45816 ) ;
#59358=CARTESIAN_POINT ( 'NONE',  ( -4.458734124999998549, -102.2291666653010651, 2.574251347313722516 ) ) ;
#59360=CARTESIAN_POINT ( 'NONE',  ( 4.458734125000001214, -97.14583333196773651, 2.574251347313718519 ) ) ;
#59361=EDGE_CURVE ( 'NONE', #57689, #43948, #56995, .T. ) ;
#59362=AXIS2_PLACEMENT_3D ( 'NONE', #29391, #49673, #5616 ) ;
#59364=CARTESIAN_POINT ( 'NONE',  ( -2.499999999999996447, -56.70833333060214443, 4.330127018922195425 ) ) ;
#59365=CARTESIAN_POINT ( 'NONE',  ( -6.972266317189433020E-16, -62.12499999726880162, -5.000000000000000000 ) ) ;
#59368=CARTESIAN_POINT ( 'NONE',  ( -4.458734124999997661, -18.22916666530106866, 2.574251347313722516 ) ) ;
#59369=CARTESIAN_POINT ( 'NONE',  ( -2.229367062499996610, 8.604166668032261711, 3.861377020970582219 ) ) ;
#59370=CARTESIAN_POINT ( 'NONE',  ( 4.458734124999999437, -62.06249999863440792, -5.460374474430324690E-16 ) ) ;
#59375=CARTESIAN_POINT ( 'NONE',  ( -3.535250795749689387E-16, -4.249999999999996447, -5.773502691896257311 ) ) ;
#59377=ORIENTED_EDGE ( 'NONE', *, *, #62536, .F. ) ;
#59380=CARTESIAN_POINT ( 'NONE',  ( 1.975475456537005874E-15, -91.62499999726877320, 5.000000000000000000 ) ) ;
#59382=CARTESIAN_POINT ( 'NONE',  ( 4.458734124999998549, -89.72916666530106511, -2.574251347313721627 ) ) ;
#59383=CARTESIAN_POINT ( 'NONE',  ( 4.458734124999998549, 17.02083333469892423, -2.574251347313721627 ) ) ;
#59384=AXIS2_PLACEMENT_3D ( 'NONE', #35770, #45095, #55714 ) ;
#59386=CARTESIAN_POINT ( 'NONE',  ( -1.339745962155613812, -89.08034179853027013, -5.000000000000000000 ) ) ;
#59387=CARTESIAN_POINT ( 'NONE',  ( 0.000000000000000000, -120.0000000000000000, 0.000000000000000000 ) ) ;
#59388=DIRECTION ( 'NONE',  ( -0.8660254037844414832, 0.000000000000000000, -0.4999999999999951705 ) ) ;
#59390=CARTESIAN_POINT ( 'NONE',  ( -3.535250795749689387E-16, -75.25000000000001421, -5.773502691896257311 ) ) ;
#59392=EDGE_LOOP ( 'NONE', ( #47609, #27944, #46534, #40827 ) ) ;
#59394=EDGE_LOOP ( 'NONE', ( #50100, #20153, #46049, #25444 ) ) ;
#59395=( BOUNDED_CURVE ( )  B_SPLINE_CURVE ( 2, ( #26068, #25104, #10941, #44714, #677, #60492, #1011, #60175, #20286 ),
 .UNSPECIFIED., .F., .F. ) 
 B_SPLINE_CURVE_WITH_KNOTS ( ( 3, 2, 2, 2, 3 ),
 ( 0.5482142857142857650, 0.5488095238095238582, 0.5500000000000000444, 0.5511904761904762307, 0.5517857142857143238 ),
 .UNSPECIFIED. ) 
 CURVE ( )  GEOMETRIC_REPRESENTATION_ITEM ( )  RATIONAL_B_SPLINE_CURVE ( ( 0.9330127018922194093, 0.9330127018922194093, 1.000000000000000000, 0.8660254037844387076, 1.000000000000000000, 0.8660254037844387076, 1.000000000000000000, 0.9330127018922194093, 0.9330127018922194093 ) ) 
 REPRESENTATION_ITEM ( '' )  );
#59400=EDGE_CURVE ( 'NONE', #60943, #10189, #31014, .T. ) ;
#59401=ORIENTED_EDGE ( 'NONE', *, *, #12282, .T. ) ;
#59406=ADVANCED_FACE ( 'NONE', ( #3037 ), #28091, .T. ) ;
#59409=CARTESIAN_POINT ( 'NONE',  ( 9.457646018065525792E-16, -61.31249999863440792, 5.148502694627439702 ) ) ;
#59413=VERTEX_POINT ( 'NONE', #62525 ) ;
#59415=VECTOR ( 'NONE', #55847, 1000.000000000000000 ) ;
#59417=CYLINDRICAL_SURFACE ( 'NONE', #39150, 5.000000000000000000 ) ;
#59418=ADVANCED_FACE ( 'NONE', ( #8792 ), #41935, .T. ) ;
#59422=CARTESIAN_POINT ( 'NONE',  ( -3.152548672688508926E-16, -108.8124999986343937, -5.148502694627439702 ) ) ;
#59428=CARTESIAN_POINT ( 'NONE',  ( 2.229367062499998831, -46.64583333196774362, -3.861377020970580887 ) ) ;
#59430=( BOUNDED_CURVE ( )  B_SPLINE_CURVE ( 2, ( #10694, #33012, #4363, #23981, #38759, #58398, #33947, #53568, #38154 ),
 .UNSPECIFIED., .F., .F. ) 
 B_SPLINE_CURVE_WITH_KNOTS ( ( 3, 2, 2, 2, 3 ),
 ( 0.9375000000000000000, 0.9380952380952380931, 0.9392857142857142794, 0.9404761904761904656, 0.9410714285714285587 ),
 .UNSPECIFIED. ) 
 CURVE ( )  GEOMETRIC_REPRESENTATION_ITEM ( )  RATIONAL_B_SPLINE_CURVE ( ( 0.9330127018922194093, 0.9330127018922194093, 1.000000000000000000, 0.8660254037844387076, 1.000000000000000000, 0.8660254037844387076, 1.000000000000000000, 0.9330127018922194093, 0.9330127018922194093 ) ) 
 REPRESENTATION_ITEM ( '' )  );
#59431=EDGE_CURVE ( 'NONE', #50402, #58314, #45896, .T. ) ;
#59433=CARTESIAN_POINT ( 'NONE',  ( -3.152548672688508926E-16, -48.56249999863440792, -5.148502694627439702 ) ) ;
#59435=CARTESIAN_POINT ( 'NONE',  ( -4.458734124999999437, -13.39583333196774184, -2.574251347313719407 ) ) ;
#59436=CARTESIAN_POINT ( 'NONE',  ( -5.000000000000000000, -101.0000000000000000, 0.000000000000000000 ) ) ;
#59438=CARTESIAN_POINT ( 'NONE',  ( 2.229367062500001939, -32.22916666530106511, 3.861377020970579999 ) ) ;
#59439=CARTESIAN_POINT ( 'NONE',  ( -2.500000000000000444, 7.958333336064518093, -4.330127018922193649 ) ) ;
#59443=LINE ( 'NONE', #14720, #32236 ) ;
#59445=CARTESIAN_POINT ( 'NONE',  ( -4.458734124999999437, 1.437500001365592972, 0.000000000000000000 ) ) ;
#59447=CARTESIAN_POINT ( 'NONE',  ( 5.000000000000000888, -57.58333333333332860, 2.886751345948126879 ) ) ;
#59448=CARTESIAN_POINT ( 'NONE',  ( -2.499999999999996447, -96.83333333333332860, 4.330127018922195425 ) ) ;
#59449=CARTESIAN_POINT ( 'NONE',  ( -2.229367062499996610, -35.14583333196772941, 3.861377020970582219 ) ) ;
#59450=CARTESIAN_POINT ( 'NONE',  ( -6.972266317189433020E-16, -23.12499999726880873, -5.000000000000000000 ) ) ;
#59451=CARTESIAN_POINT ( 'NONE',  ( 2.229367062500001939, -79.22916666530106511, 3.861377020970579999 ) ) ;
#59455=CARTESIAN_POINT ( 'NONE',  ( -4.458734124999997661, -1.229166665301071548, 2.574251347313722516 ) ) ;
#59456=CARTESIAN_POINT ( 'NONE',  ( 2.229367062499998831, 23.10416666803225993, -3.861377020970580887 ) ) ;
#59457=CARTESIAN_POINT ( 'NONE',  ( -4.458734124999999437, -43.56249999863440081, 0.000000000000000000 ) ) ;
#59458=CARTESIAN_POINT ( 'NONE',  ( -6.972266317189433020E-16, -15.25000000000000000, -5.000000000000000000 ) ) ;
#59463=CARTESIAN_POINT ( 'NONE',  ( -3.152548672688508926E-16, -72.56249999863439371, -5.148502694627439702 ) ) ;
#59464=CARTESIAN_POINT ( 'NONE',  ( 1.060575238724906964E-15, -105.6249999972688158, 5.773502691896257311 ) ) ;
#59465=AXIS2_PLACEMENT_3D ( 'NONE', #49351, #4038, #46126 ) ;
#59467=CARTESIAN_POINT ( 'NONE',  ( -5.000000000000000000, -65.00000000000000000, 0.000000000000000000 ) ) ;
#59470=CARTESIAN_POINT ( 'NONE',  ( 2.499999999999998668, -61.33333333333333570, -4.330127018922193649 ) ) ;
#59471=CARTESIAN_POINT ( 'NONE',  ( 1.975475456537005874E-15, -90.62499999726880162, 5.000000000000000000 ) ) ;
#59473=ORIENTED_EDGE ( 'NONE', *, *, #48459, .T. ) ;
#59474=CARTESIAN_POINT ( 'NONE',  ( -1.339745962155613812, -27.20534180126147916, -5.000000000000000000 ) ) ;
#59475=CARTESIAN_POINT ( 'NONE',  ( 1.339745962155615144, -67.70534180126149693, 4.999999999999999112 ) ) ;
#59480=EDGE_CURVE ( 'NONE', #2897, #28777, #61135, .T. ) ;
#59483=ORIENTED_EDGE ( 'NONE', *, *, #53972, .T. ) ;
#59484=CARTESIAN_POINT ( 'NONE',  ( -5.000000000000000000, -24.08333333333333215, -2.886751345948128211 ) ) ;
#59485=CARTESIAN_POINT ( 'NONE',  ( 1.339745962155613146, 27.41965820146970145, 5.000000000000000888 ) ) ;
#59491=CARTESIAN_POINT ( 'NONE',  ( -3.152548672688508926E-16, -47.81249999863440792, -5.148502694627439702 ) ) ;
#59500=CARTESIAN_POINT ( 'NONE',  ( 4.458734124999998549, -87.97916666530107932, -2.574251347313721627 ) ) ;
#59503=EDGE_CURVE ( 'NONE', #52308, #26333, #39676, .T. ) ;
#59504=CARTESIAN_POINT ( 'NONE',  ( -2.499999999999996447, -31.83333333333333215, 4.330127018922195425 ) ) ;
#59507=VECTOR ( 'NONE', #41492, 1000.000000000000000 ) ;
#59511=( BOUNDED_CURVE ( )  B_SPLINE_CURVE ( 2, ( #13629, #61585, #7549, #62216, #38381, #31982, #62841, #42262, #22976 ),
 .UNSPECIFIED., .F., .F. ) 
 B_SPLINE_CURVE_WITH_KNOTS ( ( 3, 2, 2, 2, 3 ),
 ( 0.1017857142857142849, 0.1023809523809523780, 0.1035714285714285782, 0.1047619047619047644, 0.1053571428571428575 ),
 .UNSPECIFIED. ) 
 CURVE ( )  GEOMETRIC_REPRESENTATION_ITEM ( )  RATIONAL_B_SPLINE_CURVE ( ( 0.9330127018922194093, 0.9330127018922194093, 1.000000000000000000, 0.8660254037844387076, 1.000000000000000000, 0.8660254037844387076, 1.000000000000000000, 0.9330127018922194093, 0.9330127018922194093 ) ) 
 REPRESENTATION_ITEM ( '' )  );
#59512=CARTESIAN_POINT ( 'NONE',  ( 4.458734124999998549, 5.270833334698926897, -2.574251347313721627 ) ) ;
#59515=CARTESIAN_POINT ( 'NONE',  ( -4.458734124999999437, -17.56249999863440792, 0.000000000000000000 ) ) ;
#59517=CARTESIAN_POINT ( 'NONE',  ( -4.999999999999998224, -73.79166666393547303, 2.886751345948131764 ) ) ;
#59519=CARTESIAN_POINT ( 'NONE',  ( 4.458734124999998549, 13.02083333469892779, -2.574251347313721627 ) ) ;
#59521=CARTESIAN_POINT ( 'NONE',  ( -4.458734124999999437, -97.39583333196773651, -2.574251347313719407 ) ) ;
#59523=CARTESIAN_POINT ( 'NONE',  ( 1.339745962155615144, -57.58034179853029144, 4.999999999999999112 ) ) ;
#59524=CARTESIAN_POINT ( 'NONE',  ( -4.458734124999998549, -16.22916666530107577, 2.574251347313722516 ) ) ;
#59526=CARTESIAN_POINT ( 'NONE',  ( -2.499999999999996447, -72.83333333333332860, 4.330127018922195425 ) ) ;
#59529=CARTESIAN_POINT ( 'NONE',  ( 1.060575238724906964E-15, -43.62499999726880873, 5.773502691896257311 ) ) ;
#59531=CARTESIAN_POINT ( 'NONE',  ( 2.229367062500001939, 15.02083333469892779, 3.861377020970579999 ) ) ;
#59532=CARTESIAN_POINT ( 'NONE',  ( 0.000000000000000000, 30.00000000000000000, 0.000000000000000000 ) ) ;
#59535=CARTESIAN_POINT ( 'NONE',  ( 2.229367062499998831, -61.64583333196774362, -3.861377020970580887 ) ) ;
#59536=EDGE_LOOP ( 'NONE', ( #15648, #19151, #48965, #24279 ) ) ;
#59538=CARTESIAN_POINT ( 'NONE',  ( -5.000000000000000000, 5.916666666666666963, -2.886751345948128211 ) ) ;
#59541=CARTESIAN_POINT ( 'NONE',  ( -2.229367062499996610, -56.14583333196773651, 3.861377020970582219 ) ) ;
#59542=CARTESIAN_POINT ( 'NONE',  ( -4.999999999999999112, -88.79166666393547303, 2.886751345948131764 ) ) ;
#59543=CARTESIAN_POINT ( 'NONE',  ( 9.457646018065525792E-16, -32.06249999863440792, 5.148502694627439702 ) ) ;
#59547=CARTESIAN_POINT ( 'NONE',  ( 1.975475456537005874E-15, -48.74999999999999289, 5.000000000000000000 ) ) ;
#59549=CARTESIAN_POINT ( 'NONE',  ( -5.000000000000000000, -44.00000000000000000, 0.000000000000000000 ) ) ;
#59553=CARTESIAN_POINT ( 'NONE',  ( 2.229367062499998831, -102.6458333319677365, -3.861377020970580887 ) ) ;
#59554=CARTESIAN_POINT ( 'NONE',  ( 4.458734124999998549, 5.020833334698926897, -2.574251347313721627 ) ) ;
#59556=LINE ( 'NONE', #29945, #15521 ) ;
#59561=CARTESIAN_POINT ( 'NONE',  ( -6.972266317189433020E-16, -26.25000000000000000, -5.000000000000000000 ) ) ;
#59565=CARTESIAN_POINT ( 'NONE',  ( 2.500000000000002220, -33.66666666666666430, 4.330127018922192761 ) ) ;
#59568=CARTESIAN_POINT ( 'NONE',  ( 5.000000000000000888, -101.5833333333333286, 2.886751345948126879 ) ) ;
#59571=CARTESIAN_POINT ( 'NONE',  ( -2.229367062500000163, -22.72916666530107221, -3.861377020970580443 ) ) ;
#59579=ORIENTED_EDGE ( 'NONE', *, *, #9884, .T. ) ;
#59581=VERTEX_POINT ( 'NONE', #57069 ) ;
#59582=CARTESIAN_POINT ( 'NONE',  ( -3.152548672688508926E-16, -71.81249999863439371, -5.148502694627439702 ) ) ;
#59589=CARTESIAN_POINT ( 'NONE',  ( -2.229367062499996610, -6.395833331967741842, 3.861377020970582219 ) ) ;
#59590=EDGE_LOOP ( 'NONE', ( #27039, #24319, #44880, #37221 ) ) ;
#59592=CARTESIAN_POINT ( 'NONE',  ( -6.972266317189433020E-16, -45.24999999999999289, -5.000000000000000000 ) ) ;
#59595=CARTESIAN_POINT ( 'NONE',  ( 1.339745962155615144, -47.58034179853029144, 4.999999999999999112 ) ) ;
#59599=CARTESIAN_POINT ( 'NONE',  ( 4.458734125000000326, -80.89583333196773651, 2.574251347313718519 ) ) ;
#59600=CYLINDRICAL_SURFACE ( 'NONE', #13091, 5.000000000000000000 ) ;
#59601=CARTESIAN_POINT ( 'NONE',  ( -4.458734124999999437, 4.604166668032261711, -2.574251347313719407 ) ) ;
#59603=CARTESIAN_POINT ( 'NONE',  ( 0.000000000000000000, -120.0000000000000000, 0.000000000000000000 ) ) ;
#59604=CARTESIAN_POINT ( 'NONE',  ( -4.999999999999999112, -84.91666666666667140, 2.886751345948131764 ) ) ;
#59606=CARTESIAN_POINT ( 'NONE',  ( -4.458734124999999437, -67.64583333196773651, -2.574251347313719407 ) ) ;
#59607=CARTESIAN_POINT ( 'NONE',  ( 2.500000000000002220, -26.54166666393547658, 4.330127018922192761 ) ) ;
#59609=CARTESIAN_POINT ( 'NONE',  ( -4.999999999999998224, -40.91666666666667140, 2.886751345948131764 ) ) ;
#59610=CARTESIAN_POINT ( 'NONE',  ( 5.000000000000000000, -110.2916666639354730, -2.886751345948130876 ) ) ;
#59611=CARTESIAN_POINT ( 'NONE',  ( 4.458734125000001214, -46.89583333196773651, 2.574251347313718519 ) ) ;
#59612=CARTESIAN_POINT ( 'NONE',  ( -3.152548672688508926E-16, -32.81249999863440792, -5.148502694627439702 ) ) ;
#59615=CARTESIAN_POINT ( 'NONE',  ( 2.500000000000002220, 21.33333333333333215, 4.330127018922192761 ) ) ;
#59618=EDGE_CURVE ( 'NONE', #45305, #37025, #13029, .T. ) ;
#59619=CARTESIAN_POINT ( 'NONE',  ( 4.458734125000001214, -38.89583333196773651, 2.574251347313718519 ) ) ;
#59620=CARTESIAN_POINT ( 'NONE',  ( -3.535250795749689387E-16, -74.12499999726880162, -5.773502691896257311 ) ) ;
#59624=CARTESIAN_POINT ( 'NONE',  ( -4.458734124999999437, -80.64583333196773651, -2.574251347313719407 ) ) ;
#59627=CARTESIAN_POINT ( 'NONE',  ( -4.999999999999999112, -27.91666666666666430, 2.886751345948131764 ) ) ;
#59629=ORIENTED_EDGE ( 'NONE', *, *, #50683, .F. ) ;
#59633=CARTESIAN_POINT ( 'NONE',  ( 1.060575238724906964E-15, 19.37500000273118772, 5.773502691896257311 ) ) ;
#59634=( BOUNDED_CURVE ( )  B_SPLINE_CURVE ( 2, ( #35634, #59123, #20201, #11502, #5726, #44633, #39803, #35314, #924 ),
 .UNSPECIFIED., .F., .F. ) 
 B_SPLINE_CURVE_WITH_KNOTS ( ( 3, 2, 2, 2, 3 ),
 ( 0.08750000000000000833, 0.08809523809523810145, 0.08928571428571428770, 0.09047619047619047394, 0.09107142857142856707 ),
 .UNSPECIFIED. ) 
 CURVE ( )  GEOMETRIC_REPRESENTATION_ITEM ( )  RATIONAL_B_SPLINE_CURVE ( ( 0.9330127018922192983, 0.9330127018922200755, 1.000000000000000000, 0.8660254037844387076, 1.000000000000000000, 0.8660254037844387076, 1.000000000000000000, 0.9330127018922194093, 0.9330127018922194093 ) ) 
 REPRESENTATION_ITEM ( '' )  );
#59642=CARTESIAN_POINT ( 'NONE',  ( 1.975475456537005874E-15, -74.62499999726880162, 5.000000000000000000 ) ) ;
#59643=CARTESIAN_POINT ( 'NONE',  ( -6.972266317189433020E-16, -74.25000000000000000, -5.000000000000000000 ) ) ;
#59646=CARTESIAN_POINT ( 'NONE',  ( 4.458734124999999437, -22.81249999863440436, -5.460374474430324690E-16 ) ) ;
#59647=CARTESIAN_POINT ( 'NONE',  ( 6.123233995736766282E-16, -120.0000000000000000, -5.000000000000000000 ) ) ;
#59657=CARTESIAN_POINT ( 'NONE',  ( -1.339745962155610925, -28.79465819873852084, 5.000000000000000000 ) ) ;
#59665=CARTESIAN_POINT ( 'NONE',  ( -6.972266317189433020E-16, -103.1249999972688158, -5.000000000000000000 ) ) ;
#59666=CARTESIAN_POINT ( 'NONE',  ( -2.229367062500000163, 15.52083333469892779, -3.861377020970580443 ) ) ;
#59669=DIRECTION ( 'NONE',  ( -0.000000000000000000, 1.000000000000000000, -0.000000000000000000 ) ) ;
#59670=CARTESIAN_POINT ( 'NONE',  ( 5.000000000000000000, -25.50000000000000355, -6.123233995736766282E-16 ) ) ;
#59671=LINE ( 'NONE', #15602, #15806 ) ;
#59672=CARTESIAN_POINT ( 'NONE',  ( -2.229367062499996610, -67.14583333196773651, 3.861377020970582219 ) ) ;
#59674=CARTESIAN_POINT ( 'NONE',  ( -4.458734124999999437, 16.60416666803225993, -2.574251347313719407 ) ) ;
#59676=CARTESIAN_POINT ( 'NONE',  ( -4.458734124999998549, -48.47916666530106511, 2.574251347313722516 ) ) ;
#59677=CARTESIAN_POINT ( 'NONE',  ( -2.500000000000000444, -7.041666663935481907, -4.330127018922193649 ) ) ;
#59678=CARTESIAN_POINT ( 'NONE',  ( 5.000000000000000000, -25.37499999726881583, -6.123233995736766282E-16 ) ) ;
#59682=CARTESIAN_POINT ( 'NONE',  ( 2.229367062500001939, -18.22916666530106866, 3.861377020970579999 ) ) ;
#59685=CARTESIAN_POINT ( 'NONE',  ( -3.152548672688508926E-16, -104.5624999986343937, -5.148502694627439702 ) ) ;
#59688=CARTESIAN_POINT ( 'NONE',  ( 2.229367062499998831, -95.89583333196773651, -3.861377020970580887 ) ) ;
#59689=AXIS2_PLACEMENT_3D ( 'NONE', #7584, #18170, #42613 ) ;
#59691=LINE ( 'NONE', #512, #25346 ) ;
#59692=CARTESIAN_POINT ( 'NONE',  ( 5.000000000000000000, -58.29166666393548724, -2.886751345948129988 ) ) ;
#59693=CARTESIAN_POINT ( 'NONE',  ( 2.500000000000002220, -62.54166666393547303, 4.330127018922192761 ) ) ;
#59696=CARTESIAN_POINT ( 'NONE',  ( -2.229367062499996610, -16.14583333196773651, 3.861377020970582219 ) ) ;
#59697=CARTESIAN_POINT ( 'NONE',  ( -2.229367062499996610, 5.604166668032261711, 3.861377020970582219 ) ) ;
#59698=CARTESIAN_POINT ( 'NONE',  ( -3.152548672688508926E-16, -61.81249999863440081, -5.148502694627439702 ) ) ;
#59702=CARTESIAN_POINT ( 'NONE',  ( 5.000000000000000888, -9.583333333333333925, 2.886751345948126879 ) ) ;
#59706=DIRECTION ( 'NONE',  ( 0.000000000000000000, 0.000000000000000000, 1.000000000000000000 ) ) ;
#59707=DIRECTION ( 'NONE',  ( -0.000000000000000000, 1.000000000000000000, -0.000000000000000000 ) ) ;
#59712=CYLINDRICAL_SURFACE ( 'NONE', #31864, 5.000000000000000000 ) ;
#59713=ADVANCED_FACE ( 'NONE', ( #4910 ), #54107, .T. ) ;
#59717=CARTESIAN_POINT ( 'NONE',  ( 2.499999999999998668, -77.33333333333334281, -4.330127018922193649 ) ) ;
#59719=EDGE_LOOP ( 'NONE', ( #212, #52682, #41217, #49034 ) ) ;
#59720=CARTESIAN_POINT ( 'NONE',  ( 1.339745962155615144, -80.58034179853028434, 4.999999999999999112 ) ) ;
#59722=CARTESIAN_POINT ( 'NONE',  ( 0.000000000000000000, -120.0000000000000000, 5.000000000000000000 ) ) ;
#59726=ORIENTED_EDGE ( 'NONE', *, *, #1696, .T. ) ;
#59729=ORIENTED_EDGE ( 'NONE', *, *, #56317, .T. ) ;
#59732=CARTESIAN_POINT ( 'NONE',  ( 4.458734124999999437, -62.06249999863440792, -5.460374474430324690E-16 ) ) ;
#59735=EDGE_LOOP ( 'NONE', ( #41660, #5699, #9251, #25542 ) ) ;
#59739=DIRECTION ( 'NONE',  ( 0.000000000000000000, 0.000000000000000000, 1.000000000000000000 ) ) ;
#59744=CARTESIAN_POINT ( 'NONE',  ( -2.229367062499996610, 28.85416666803226349, 3.861377020970582219 ) ) ;
#59746=ORIENTED_EDGE ( 'NONE', *, *, #38485, .F. ) ;
#59750=CARTESIAN_POINT ( 'NONE',  ( -4.458734124999997661, -43.22916666530106511, 2.574251347313722516 ) ) ;
#59752=CARTESIAN_POINT ( 'NONE',  ( 6.123233995736766282E-16, -120.0000000000000000, -5.000000000000000000 ) ) ;
#59753=CARTESIAN_POINT ( 'NONE',  ( -2.229367062499996610, -51.14583333196772941, 3.861377020970582219 ) ) ;
#59755=CARTESIAN_POINT ( 'NONE',  ( -4.458734124999998549, -17.22916666530106866, 2.574251347313722516 ) ) ;
#59756=CARTESIAN_POINT ( 'NONE',  ( -2.500000000000000444, -103.1666666666666572, -4.330127018922193649 ) ) ;
#59758=CARTESIAN_POINT ( 'NONE',  ( 4.458734124999999437, -31.06249999863440436, -5.460374474430324690E-16 ) ) ;
#59759=CARTESIAN_POINT ( 'NONE',  ( -5.000000000000000000, 7.125000002731185944, 0.000000000000000000 ) ) ;
#59760=DIRECTION ( 'NONE',  ( 0.000000000000000000, -0.000000000000000000, 1.000000000000000000 ) ) ;
#59763=FACE_OUTER_BOUND ( 'NONE', #39371, .T. ) ;
#59766=CARTESIAN_POINT ( 'NONE',  ( 4.458734124999998549, 2.020833334698927786, -2.574251347313721627 ) ) ;
#59768=CARTESIAN_POINT ( 'NONE',  ( 5.000000000000000888, -30.58333333333333215, 2.886751345948126879 ) ) ;
#59770=CARTESIAN_POINT ( 'NONE',  ( -4.458734124999998549, -87.22916666530107932, 2.574251347313722516 ) ) ;
#59771=CARTESIAN_POINT ( 'NONE',  ( -2.229367062499996610, -37.14583333196773651, 3.861377020970582219 ) ) ;
#59772=CARTESIAN_POINT ( 'NONE',  ( 2.499999999999998668, -9.333333333333332149, -4.330127018922193649 ) ) ;
#59773=CARTESIAN_POINT ( 'NONE',  ( 4.458734124999999437, -80.06249999863440792, -5.460374474430324690E-16 ) ) ;
#59774=EDGE_CURVE ( 'NONE', #55214, #16469, #10369, .T. ) ;
#59776=DIRECTION ( 'NONE',  ( 0.000000000000000000, 0.000000000000000000, 1.000000000000000000 ) ) ;
#59778=ADVANCED_FACE ( 'NONE', ( #58937 ), #29021, .T. ) ;
#59780=CARTESIAN_POINT ( 'NONE',  ( 4.458734125000000326, -1.895833331967737623, 2.574251347313718519 ) ) ;
#59781=CARTESIAN_POINT ( 'NONE',  ( -2.229367062500000163, 22.27083333469892423, -3.861377020970580443 ) ) ;
#59782=CARTESIAN_POINT ( 'NONE',  ( -2.229367062500000163, -46.72916666530106511, -3.861377020970580443 ) ) ;
#59783=CARTESIAN_POINT ( 'NONE',  ( 1.975475456537005874E-15, -45.62499999726880873, 5.000000000000000000 ) ) ;
#59786=ORIENTED_EDGE ( 'NONE', *, *, #59861, .T. ) ;
#59788=( BOUNDED_CURVE ( )  B_SPLINE_CURVE ( 2, ( #3143, #4082, #24004, #29127, #62633, #57179, #22764, #58100, #18555 ),
 .UNSPECIFIED., .F., .F. ) 
 B_SPLINE_CURVE_WITH_KNOTS ( ( 3, 2, 2, 2, 3 ),
 ( 0.7053571428571429047, 0.7059523809523809978, 0.7071428571428571841, 0.7083333333333333703, 0.7089285714285714635 ),
 .UNSPECIFIED. ) 
 CURVE ( )  GEOMETRIC_REPRESENTATION_ITEM ( )  RATIONAL_B_SPLINE_CURVE ( ( 0.9330127018922194093, 0.9330127018922194093, 1.000000000000000000, 0.8660254037844387076, 1.000000000000000000, 0.8660254037844387076, 1.000000000000000000, 0.9330127018922194093, 0.9330127018922194093 ) ) 
 REPRESENTATION_ITEM ( '' )  );
#59790=CARTESIAN_POINT ( 'NONE',  ( 4.458734124999998549, -74.72916666530106511, -2.574251347313721627 ) ) ;
#59791=CARTESIAN_POINT ( 'NONE',  ( 5.000000000000000000, -110.3749999972688016, -6.123233995736766282E-16 ) ) ;
#59792=ADVANCED_FACE ( 'NONE', ( #44773 ), #63147, .T. ) ;
#59794=CYLINDRICAL_SURFACE ( 'NONE', #28682, 5.000000000000000000 ) ;
#59795=ADVANCED_FACE ( 'NONE', ( #43816 ), #63463, .T. ) ;
#59798=CARTESIAN_POINT ( 'NONE',  ( 5.000000000000000888, -59.58333333333334281, 2.886751345948126879 ) ) ;
#59799=CARTESIAN_POINT ( 'NONE',  ( -1.339745962155610925, -74.79465819873854571, 5.000000000000000000 ) ) ;
#59818=CARTESIAN_POINT ( 'NONE',  ( -4.458734124999998549, -46.47916666530107221, 2.574251347313722516 ) ) ;
#59828=CARTESIAN_POINT ( 'NONE',  ( 4.458734124999999437, -92.06249999863440792, -5.460374474430324690E-16 ) ) ;
#59834=CARTESIAN_POINT ( 'NONE',  ( 2.500000000000002220, -82.54166666393547303, 4.330127018922192761 ) ) ;
#59836=CARTESIAN_POINT ( 'NONE',  ( 4.458734124999999437, -1.812499998634406584, -5.460374474430324690E-16 ) ) ;
#59837=CARTESIAN_POINT ( 'NONE',  ( 1.339745962155615144, 6.294658198738519062, 4.999999999999999112 ) ) ;
#59838=CARTESIAN_POINT ( 'NONE',  ( 2.229367062500001939, -18.22916666530106866, 3.861377020970579999 ) ) ;
#59839=CARTESIAN_POINT ( 'NONE',  ( -6.972266317189433020E-16, -101.2499999999999858, -5.000000000000000000 ) ) ;
#59843=CARTESIAN_POINT ( 'NONE',  ( 4.458734124999998549, 16.02083333469892779, -2.574251347313721627 ) ) ;
#59846=CARTESIAN_POINT ( 'NONE',  ( 1.975475456537005874E-15, -20.74999999999999645, 5.000000000000000000 ) ) ;
#59847=CARTESIAN_POINT ( 'NONE',  ( -4.458734124999998549, -21.22916666530107221, 2.574251347313722516 ) ) ;
#59852=CARTESIAN_POINT ( 'NONE',  ( -2.499999999999996447, -45.70833333060214443, 4.330127018922195425 ) ) ;
#59854=CARTESIAN_POINT ( 'NONE',  ( 4.458734124999998549, 16.27083333469892779, -2.574251347313721627 ) ) ;
#59855=LINE ( 'NONE', #1641, #43784 ) ;
#59858=CARTESIAN_POINT ( 'NONE',  ( -4.458734124999998549, -67.22916666530106511, 2.574251347313722516 ) ) ;
#59861=EDGE_CURVE ( 'NONE', #47452, #1619, #19584, .T. ) ;
#59862=CARTESIAN_POINT ( 'NONE',  ( 1.060575238724906964E-15, 5.250000000000000888, 5.773502691896257311 ) ) ;
#59865=CARTESIAN_POINT ( 'NONE',  ( -2.229367062500000163, -56.47916666530107221, -3.861377020970580443 ) ) ;
#59866=CARTESIAN_POINT ( 'NONE',  ( 5.000000000000000000, -90.29166666393547303, -2.886751345948129988 ) ) ;
#59867=CARTESIAN_POINT ( 'NONE',  ( -2.229367062499996610, -33.14583333196772941, 3.861377020970582219 ) ) ;
#59869=EDGE_CURVE ( 'NONE', #29404, #15518, #55401, .T. ) ;
#59870=DIRECTION ( 'NONE',  ( -0.000000000000000000, 1.000000000000000000, -0.000000000000000000 ) ) ;
#59871=DIRECTION ( 'NONE',  ( -0.000000000000000000, 1.000000000000000000, -0.000000000000000000 ) ) ;
#59875=CARTESIAN_POINT ( 'NONE',  ( 2.500000000000002220, -41.66666666666667140, 4.330127018922192761 ) ) ;
#59876=CARTESIAN_POINT ( 'NONE',  ( 1.975475456537005874E-15, -1.749999999999999334, 5.000000000000000000 ) ) ;
#59878=CARTESIAN_POINT ( 'NONE',  ( -6.972266317189433020E-16, -86.12499999726880162, -5.000000000000000000 ) ) ;
#59880=CARTESIAN_POINT ( 'NONE',  ( 2.229367062500001939, -108.9791666653010651, 3.861377020970579999 ) ) ;
#59881=CARTESIAN_POINT ( 'NONE',  ( -4.458734124999999437, 1.354166668032261933, -2.574251347313719407 ) ) ;
#59882=CARTESIAN_POINT ( 'NONE',  ( -2.499999999999996447, -96.70833333060213022, 4.330127018922195425 ) ) ;
#59883=EDGE_CURVE ( 'NONE', #45003, #57302, #21680, .T. ) ;
#59890=VERTEX_POINT ( 'NONE', #49917 ) ;
#59892=CARTESIAN_POINT ( 'NONE',  ( 2.500000000000002220, -22.54166666393548013, 4.330127018922192761 ) ) ;
#59894=ORIENTED_EDGE ( 'NONE', *, *, #49609, .T. ) ;
#59895=CARTESIAN_POINT ( 'NONE',  ( 1.339745962155615144, -101.7053418012614827, 4.999999999999999112 ) ) ;
#59897=CARTESIAN_POINT ( 'NONE',  ( 4.458734124999998549, -27.97916666530107577, -2.574251347313721627 ) ) ;
#59898=CARTESIAN_POINT ( 'NONE',  ( 6.123233995736766282E-16, -120.0000000000000000, -5.000000000000000000 ) ) ;
#59905=ORIENTED_EDGE ( 'NONE', *, *, #29741, .F. ) ;
#59907=ORIENTED_EDGE ( 'NONE', *, *, #38995, .F. ) ;
#59908=CARTESIAN_POINT ( 'NONE',  ( -4.458734124999998549, -79.47916666530106511, 2.574251347313722516 ) ) ;
#59912=CARTESIAN_POINT ( 'NONE',  ( -5.000000000000000000, 8.000000000000000000, 0.000000000000000000 ) ) ;
#59914=CARTESIAN_POINT ( 'NONE',  ( 9.457646018065525792E-16, -2.312499998634407028, 5.148502694627439702 ) ) ;
#59916=( BOUNDED_CURVE ( )  B_SPLINE_CURVE ( 2, ( #24079, #4761, #44312, #47875, #4150, #39170, #23768, #53025, #43368 ),
 .UNSPECIFIED., .F., .F. ) 
 B_SPLINE_CURVE_WITH_KNOTS ( ( 3, 2, 2, 2, 3 ),
 ( 0.09107142857142856707, 0.09166666666666666019, 0.09285714285714286031, 0.09404761904761904656, 0.09464285714285713969 ),
 .UNSPECIFIED. ) 
 CURVE ( )  GEOMETRIC_REPRESENTATION_ITEM ( )  RATIONAL_B_SPLINE_CURVE ( ( 0.9330127018922194093, 0.9330127018922194093, 1.000000000000000000, 0.8660254037844387076, 1.000000000000000000, 0.8660254037844387076, 1.000000000000000000, 0.9330127018922194093, 0.9330127018922194093 ) ) 
 REPRESENTATION_ITEM ( '' )  );
#59917=CARTESIAN_POINT ( 'NONE',  ( -2.500000000000000444, -93.04166666393547303, -4.330127018922193649 ) ) ;
#59918=CARTESIAN_POINT ( 'NONE',  ( -6.972266317189433020E-16, -91.24999999999998579, -5.000000000000000000 ) ) ;
#59922=CARTESIAN_POINT ( 'NONE',  ( 2.229367062499998831, 29.10416666803225993, -3.861377020970580887 ) ) ;
#59924=CARTESIAN_POINT ( 'NONE',  ( -2.229367062499996610, -81.14583333196773651, 3.861377020970582219 ) ) ;
#59926=CARTESIAN_POINT ( 'NONE',  ( -4.458734124999999437, -5.395833331967740953, -2.574251347313719407 ) ) ;
#59929=CARTESIAN_POINT ( 'NONE',  ( 4.458734124999999437, -69.06249999863439371, -5.460374474430324690E-16 ) ) ;
#59930=CARTESIAN_POINT ( 'NONE',  ( 1.060575238724906964E-15, -31.62499999726880873, 5.773502691896257311 ) ) ;
#59931=CARTESIAN_POINT ( 'NONE',  ( -1.339745962155613812, -15.20534180126147916, -5.000000000000000000 ) ) ;
#59933=CARTESIAN_POINT ( 'NONE',  ( -5.000000000000000000, 22.91666666666666430, -2.886751345948128211 ) ) ;
#59935=CARTESIAN_POINT ( 'NONE',  ( -2.229367062500000163, -43.47916666530106511, -3.861377020970580443 ) ) ;
#59936=CARTESIAN_POINT ( 'NONE',  ( 2.229367062499998831, -32.89583333196773651, -3.861377020970580887 ) ) ;
#59939=CARTESIAN_POINT ( 'NONE',  ( 5.000000000000000888, 19.41666666666666075, 2.886751345948126879 ) ) ;
#59942=CARTESIAN_POINT ( 'NONE',  ( -3.152548672688508926E-16, -40.56249999863440081, -5.148502694627439702 ) ) ;
#59943=CARTESIAN_POINT ( 'NONE',  ( 5.000000000000000888, -71.45833333060214443, 2.886751345948126879 ) ) ;
#59946=LINE ( 'NONE', #15868, #33916 ) ;
#59947=CARTESIAN_POINT ( 'NONE',  ( -6.972266317189433020E-16, -37.25000000000000000, -5.000000000000000000 ) ) ;
#59948=CARTESIAN_POINT ( 'NONE',  ( 9.457646018065525792E-16, -78.31249999863440792, 5.148502694627439702 ) ) ;
#59952=CARTESIAN_POINT ( 'NONE',  ( 5.000000000000000000, -25.50000000000000355, -6.123233995736766282E-16 ) ) ;
#59956=ORIENTED_EDGE ( 'NONE', *, *, #18613, .T. ) ;
#59958=CARTESIAN_POINT ( 'NONE',  ( 1.060575238724906964E-15, 21.37500000273118417, 5.773502691896257311 ) ) ;
#59966=CARTESIAN_POINT ( 'NONE',  ( 0.000000000000000000, -120.0000000000000000, 0.000000000000000000 ) ) ;
#59967=CARTESIAN_POINT ( 'NONE',  ( 1.339745962155615144, -11.58034179853029499, 4.999999999999999112 ) ) ;
#59968=CARTESIAN_POINT ( 'NONE',  ( 1.339745962155612702, -74.29465819873853150, -5.000000000000000000 ) ) ;
#59970=( BOUNDED_CURVE ( )  B_SPLINE_CURVE ( 2, ( #54319, #28913, #38266, #24731, #23789, #38562, #24102, #39194, #28601 ),
 .UNSPECIFIED., .F., .F. ) 
 B_SPLINE_CURVE_WITH_KNOTS ( ( 3, 2, 2, 2, 3 ),
 ( 0.3696428571428571619, 0.3702380952380952550, 0.3714285714285714413, 0.3726190476190476275, 0.3732142857142857206 ),
 .UNSPECIFIED. ) 
 CURVE ( )  GEOMETRIC_REPRESENTATION_ITEM ( )  RATIONAL_B_SPLINE_CURVE ( ( 0.9330127018922194093, 0.9330127018922194093, 1.000000000000000000, 0.8660254037844387076, 1.000000000000000000, 0.8660254037844387076, 1.000000000000000000, 0.9330127018922194093, 0.9330127018922194093 ) ) 
 REPRESENTATION_ITEM ( '' )  );
#59971=CARTESIAN_POINT ( 'NONE',  ( -4.458734124999999437, -13.56249999863440259, 0.000000000000000000 ) ) ;
#59975=VERTEX_POINT ( 'NONE', #25479 ) ;
#59976=CARTESIAN_POINT ( 'NONE',  ( -5.000000000000000000, 25.12500000273118417, 0.000000000000000000 ) ) ;
#59980=CARTESIAN_POINT ( 'NONE',  ( -5.000000000000000000, -86.00000000000000000, 0.000000000000000000 ) ) ;
#59985=DIRECTION ( 'NONE',  ( -0.000000000000000000, 1.000000000000000000, -0.000000000000000000 ) ) ;
#59987=ORIENTED_EDGE ( 'NONE', *, *, #30367, .T. ) ;
#59989=CARTESIAN_POINT ( 'NONE',  ( -3.152548672688508926E-16, 16.43750000136559564, -5.148502694627439702 ) ) ;
#59993=CARTESIAN_POINT ( 'NONE',  ( 6.123233995736766282E-16, -120.0000000000000000, -5.000000000000000000 ) ) ;
#59994=CARTESIAN_POINT ( 'NONE',  ( 4.458734125000000326, -64.89583333196773651, 2.574251347313718519 ) ) ;
#59996=CARTESIAN_POINT ( 'NONE',  ( 4.458734124999999437, 12.18750000136559564, -5.460374474430324690E-16 ) ) ;
#59999=CARTESIAN_POINT ( 'NONE',  ( -4.458734124999999437, -53.64583333196772941, -2.574251347313719407 ) ) ;
#60000=CARTESIAN_POINT ( 'NONE',  ( -5.000000000000000000, -6.874999997268812280, 0.000000000000000000 ) ) ;
#60001=CARTESIAN_POINT ( 'NONE',  ( -6.972266317189433020E-16, -25.12499999726881228, -5.000000000000000000 ) ) ;
#60002=CARTESIAN_POINT ( 'NONE',  ( -6.972266317189433020E-16, -66.12499999726881583, -5.000000000000000000 ) ) ;
#60005=CARTESIAN_POINT ( 'NONE',  ( -2.229367062500000163, -18.72916666530106866, -3.861377020970580443 ) ) ;
#60009=CARTESIAN_POINT ( 'NONE',  ( -2.229367062499996610, -106.1458333319677365, 3.861377020970582219 ) ) ;
#60011=VERTEX_POINT ( 'NONE', #10999 ) ;
#60012=CARTESIAN_POINT ( 'NONE',  ( 4.458734125000001214, -98.14583333196773651, 2.574251347313718519 ) ) ;
#60013=CARTESIAN_POINT ( 'NONE',  ( 2.229367062499998831, -24.64583333196773651, -3.861377020970580887 ) ) ;
#60014=CARTESIAN_POINT ( 'NONE',  ( -2.500000000000000444, -59.04166666393546592, -4.330127018922193649 ) ) ;
#60015=DIRECTION ( 'NONE',  ( 0.000000000000000000, 0.000000000000000000, 1.000000000000000000 ) ) ;
#60018=CARTESIAN_POINT ( 'NONE',  ( 4.458734125000000326, -25.89583333196773651, 2.574251347313718519 ) ) ;
#60019=CARTESIAN_POINT ( 'NONE',  ( -3.152548672688508926E-16, 6.187500001365593860, -5.148502694627439702 ) ) ;
#60020=CARTESIAN_POINT ( 'NONE',  ( 2.229367062499998831, -62.89583333196774362, -3.861377020970580887 ) ) ;
#60021=DIRECTION ( 'NONE',  ( -0.000000000000000000, 1.000000000000000000, -0.000000000000000000 ) ) ;
#60023=CARTESIAN_POINT ( 'NONE',  ( 0.000000000000000000, -120.0000000000000000, 0.000000000000000000 ) ) ;
#60025=CARTESIAN_POINT ( 'NONE',  ( 2.499999999999998668, -11.33333333333333393, -4.330127018922193649 ) ) ;
#60027=EDGE_LOOP ( 'NONE', ( #16311, #54051, #63623, #28948 ) ) ;
#60034=CARTESIAN_POINT ( 'NONE',  ( -4.999999999999998224, 26.08333333333332860, 2.886751345948131764 ) ) ;
#60036=CARTESIAN_POINT ( 'NONE',  ( 5.000000000000000000, -75.50000000000000000, -6.123233995736766282E-16 ) ) ;
#60040=ORIENTED_EDGE ( 'NONE', *, *, #56976, .F. ) ;
#60041=DIRECTION ( 'NONE',  ( 0.000000000000000000, 0.000000000000000000, 1.000000000000000000 ) ) ;
#60050=CARTESIAN_POINT ( 'NONE',  ( 2.500000000000002220, -55.66666666666667140, 4.330127018922192761 ) ) ;
#60053=EDGE_CURVE ( 'NONE', #34132, #48396, #30622, .T. ) ;
#60058=CARTESIAN_POINT ( 'NONE',  ( -2.229367062500000163, -77.47916666530106511, -3.861377020970580443 ) ) ;
#60059=CARTESIAN_POINT ( 'NONE',  ( 2.229367062499998831, -109.8958333319677365, -3.861377020970580887 ) ) ;
#60061=VERTEX_POINT ( 'NONE', #12283 ) ;
#60062=DIRECTION ( 'NONE',  ( 0.000000000000000000, 0.000000000000000000, 1.000000000000000000 ) ) ;
#60066=CARTESIAN_POINT ( 'NONE',  ( 4.458734124999999437, -41.81249999863440081, -5.460374474430324690E-16 ) ) ;
#60069=CARTESIAN_POINT ( 'NONE',  ( 4.458734124999998549, -50.72916666530106511, -2.574251347313721627 ) ) ;
#60071=CARTESIAN_POINT ( 'NONE',  ( 5.000000000000000000, 2.625000002731185500, -6.123233995736766282E-16 ) ) ;
#60072=CARTESIAN_POINT ( 'NONE',  ( -4.458734124999999437, -18.31249999863440792, 0.000000000000000000 ) ) ;
#60073=CARTESIAN_POINT ( 'NONE',  ( -2.500000000000000444, -101.1666666666666572, -4.330127018922193649 ) ) ;
#60077=CARTESIAN_POINT ( 'NONE',  ( 4.458734124999998549, -35.97916666530107221, -2.574251347313721627 ) ) ;
#60079=CARTESIAN_POINT ( 'NONE',  ( 2.499999999999998668, 6.791666669397851130, -4.330127018922193649 ) ) ;
#60084=FACE_OUTER_BOUND ( 'NONE', #59256, .T. ) ;
#60085=CARTESIAN_POINT ( 'NONE',  ( -2.229367062500000163, 1.270833334698927342, -3.861377020970580443 ) ) ;
#60088=CARTESIAN_POINT ( 'NONE',  ( -6.972266317189433020E-16, -34.12499999726881583, -5.000000000000000000 ) ) ;
#60089=CARTESIAN_POINT ( 'NONE',  ( 4.458734125000001214, -87.89583333196773651, 2.574251347313718519 ) ) ;
#60090=CARTESIAN_POINT ( 'NONE',  ( -4.458734124999999437, -36.31249999863440792, 0.000000000000000000 ) ) ;
#60091=CARTESIAN_POINT ( 'NONE',  ( -5.926426369611017623E-15, 27.24999999999999645, 5.000000000000000000 ) ) ;
#60092=CARTESIAN_POINT ( 'NONE',  ( -2.229367062499996610, -80.39583333196773651, 3.861377020970582219 ) ) ;
#60094=CARTESIAN_POINT ( 'NONE',  ( -5.000000000000000000, -52.99999999999999289, 0.000000000000000000 ) ) ;
#60097=CARTESIAN_POINT ( 'NONE',  ( -2.229367062499996610, -9.145833331967736513, 3.861377020970582219 ) ) ;
#60098=CARTESIAN_POINT ( 'NONE',  ( 2.229367062499998831, 21.10416666803226349, -3.861377020970580887 ) ) ;
#60099=CARTESIAN_POINT ( 'NONE',  ( 4.458734125000000326, -49.14583333196772941, 2.574251347313718519 ) ) ;
#60103=CARTESIAN_POINT ( 'NONE',  ( 1.975475456537005874E-15, -97.74999999999998579, 5.000000000000000000 ) ) ;
#60104=ORIENTED_EDGE ( 'NONE', *, *, #61039, .F. ) ;
#60107=CARTESIAN_POINT ( 'NONE',  ( -4.458734124999998549, -72.22916666530107932, 2.574251347313722516 ) ) ;
#60108=CARTESIAN_POINT ( 'NONE',  ( -2.229367062499996610, 28.60416666803226349, 3.861377020970582219 ) ) ;
#60110=LINE ( 'NONE', #10884, #23565 ) ;
#60113=CARTESIAN_POINT ( 'NONE',  ( 5.000000000000000000, -58.41666666666665719, -2.886751345948129988 ) ) ;
#60117=CARTESIAN_POINT ( 'NONE',  ( -5.000000000000000000, -56.99999999999999289, 0.000000000000000000 ) ) ;
#60118=CARTESIAN_POINT ( 'NONE',  ( 5.000000000000000888, -52.45833333060213732, 2.886751345948126879 ) ) ;
#60123=VECTOR ( 'NONE', #23819, 1000.000000000000000 ) ;
#60126=ORIENTED_EDGE ( 'NONE', *, *, #1416, .F. ) ;
#60128=CARTESIAN_POINT ( 'NONE',  ( 2.499999999999998668, 27.79166666939785202, -4.330127018922193649 ) ) ;
#60130=ORIENTED_EDGE ( 'NONE', *, *, #43546, .T. ) ;
#60134=CARTESIAN_POINT ( 'NONE',  ( 4.458734124999999437, -49.06249999863440792, -5.460374474430324690E-16 ) ) ;
#60135=CARTESIAN_POINT ( 'NONE',  ( 1.339745962155615144, -23.70534180126148271, 4.999999999999999112 ) ) ;
#60139=ADVANCED_FACE ( 'NONE', ( #41856 ), #51836, .T. ) ;
#60142=CARTESIAN_POINT ( 'NONE',  ( 5.000000000000000888, 22.41666666666666785, 2.886751345948126879 ) ) ;
#60144=CARTESIAN_POINT ( 'NONE',  ( -2.229367062500000163, -96.72916666530105090, -3.861377020970580443 ) ) ;
#60151=EDGE_CURVE ( 'NONE', #59975, #5237, #61509, .T. ) ;
#60152=CARTESIAN_POINT ( 'NONE',  ( 0.000000000000000000, -120.0000000000000000, 5.000000000000000000 ) ) ;
#60153=ORIENTED_EDGE ( 'NONE', *, *, #13887, .T. ) ;
#60154=CARTESIAN_POINT ( 'NONE',  ( -3.152548672688508926E-16, -0.5624999986344053626, -5.148502694627439702 ) ) ;
#60156=CARTESIAN_POINT ( 'NONE',  ( 2.229367062499998831, -18.89583333196774007, -3.861377020970580887 ) ) ;
#60158=CARTESIAN_POINT ( 'NONE',  ( -2.500000000000000444, -101.0416666639354588, -4.330127018922193649 ) ) ;
#60160=ADVANCED_FACE ( 'NONE', ( #52155 ), #14398, .T. ) ;
#60163=CARTESIAN_POINT ( 'NONE',  ( -4.458734124999999437, 14.35416666803226171, -2.574251347313719407 ) ) ;
#60166=CARTESIAN_POINT ( 'NONE',  ( 2.500000000000002220, -71.54166666393547303, 4.330127018922192761 ) ) ;
#60167=CARTESIAN_POINT ( 'NONE',  ( -4.458734124999998549, -18.22916666530107221, 2.574251347313722516 ) ) ;
#60171=CARTESIAN_POINT ( 'NONE',  ( 2.500000000000002220, -48.54166666393547303, 4.330127018922192761 ) ) ;
#60173=CARTESIAN_POINT ( 'NONE',  ( 4.458734124999998549, 13.27083333469892779, -2.574251347313721627 ) ) ;
#60174=CARTESIAN_POINT ( 'NONE',  ( 1.975475456537005874E-15, -35.75000000000000711, 5.000000000000000000 ) ) ;
#60175=CARTESIAN_POINT ( 'NONE',  ( -1.339745962155613812, -48.08034179853029144, -5.000000000000000000 ) ) ;
#60177=CARTESIAN_POINT ( 'NONE',  ( 2.229367062499998831, -69.64583333196773651, -3.861377020970580887 ) ) ;
#60179=CARTESIAN_POINT ( 'NONE',  ( 1.060575238724906964E-15, 4.250000000000000000, 5.773502691896257311 ) ) ;
#60181=CARTESIAN_POINT ( 'NONE',  ( 1.975475456537005874E-15, -0.6249999972688137229, 5.000000000000000000 ) ) ;
#60182=CARTESIAN_POINT ( 'NONE',  ( -2.229367062499996610, -57.14583333196773651, 3.861377020970582219 ) ) ;
#60183=CARTESIAN_POINT ( 'NONE',  ( -3.535250795749689387E-16, -96.12499999726880162, -5.773502691896257311 ) ) ;
#60184=EDGE_CURVE ( 'NONE', #13829, #6026, #47014, .T. ) ;
#60185=CARTESIAN_POINT ( 'NONE',  ( -5.000000000000000000, -41.87499999726880873, 0.000000000000000000 ) ) ;
#60186=CARTESIAN_POINT ( 'NONE',  ( -6.972266317189433020E-16, -30.25000000000000000, -5.000000000000000000 ) ) ;
#60187=CARTESIAN_POINT ( 'NONE',  ( 2.500000000000002220, -56.66666666666667140, 4.330127018922192761 ) ) ;
#60189=CARTESIAN_POINT ( 'NONE',  ( 0.000000000000000000, -120.0000000000000000, 5.000000000000000000 ) ) ;
#60191=CARTESIAN_POINT ( 'NONE',  ( 5.000000000000000000, -44.41666666666665719, -2.886751345948129988 ) ) ;
#60193=CARTESIAN_POINT ( 'NONE',  ( -2.499999999999996447, -107.8333333333333428, 4.330127018922195425 ) ) ;
#60194=VERTEX_POINT ( 'NONE', #47329 ) ;
#60195=CARTESIAN_POINT ( 'NONE',  ( -4.458734124999998549, -109.2291666653010793, 2.574251347313722516 ) ) ;
#60196=CARTESIAN_POINT ( 'NONE',  ( 4.458734125000001214, -1.145833331967740509, 2.574251347313718519 ) ) ;
#60197=( BOUNDED_CURVE ( )  B_SPLINE_CURVE ( 2, ( #12363, #51298, #40989, #56113, #51918, #61899, #31019, #26848, #17817 ),
 .UNSPECIFIED., .F., .F. ) 
 B_SPLINE_CURVE_WITH_KNOTS ( ( 3, 2, 2, 2, 3 ),
 ( 0.7660714285714286254, 0.7666666666666667185, 0.7678571428571429047, 0.7690476190476190910, 0.7696428571428571841 ),
 .UNSPECIFIED. ) 
 CURVE ( )  GEOMETRIC_REPRESENTATION_ITEM ( )  RATIONAL_B_SPLINE_CURVE ( ( 0.9330127018922194093, 0.9330127018922256266, 1.000000000000000000, 0.8660254037844387076, 1.000000000000000000, 0.8660254037844387076, 1.000000000000000000, 0.9330127018922194093, 0.9330127018922194093 ) ) 
 REPRESENTATION_ITEM ( '' )  );
#60210=CARTESIAN_POINT ( 'NONE',  ( -2.229367062500000163, -32.72916666530106511, -3.861377020970580443 ) ) ;
#60217=EDGE_CURVE ( 'NONE', #7933, #51679, #258, .T. ) ;
#60219=EDGE_CURVE ( 'NONE', #1619, #52308, #4372, .T. ) ;
#60220=CARTESIAN_POINT ( 'NONE',  ( 1.339745962155615144, -20.58034179853029144, 4.999999999999999112 ) ) ;
#60222=CARTESIAN_POINT ( 'NONE',  ( 4.458734125000001214, -79.14583333196772230, 2.574251347313718519 ) ) ;
#60224=EDGE_CURVE ( 'NONE', #12070, #7250, #10946, .T. ) ;
#60226=CARTESIAN_POINT ( 'NONE',  ( -2.499999999999996447, -14.70833333060214976, 4.330127018922195425 ) ) ;
#60229=CARTESIAN_POINT ( 'NONE',  ( -2.229367062500000163, -4.729166665301071326, -3.861377020970580443 ) ) ;
#60231=EDGE_CURVE ( 'NONE', #5205, #46124, #24106, .T. ) ;
#60234=LINE ( 'NONE', #35456, #21263 ) ;
#60235=EDGE_CURVE ( 'NONE', #25203, #15879, #1230, .T. ) ;
#60242=CARTESIAN_POINT ( 'NONE',  ( 4.458734124999999437, -82.81249999863440792, -5.460374474430324690E-16 ) ) ;
#60244=CARTESIAN_POINT ( 'NONE',  ( 2.500000000000002220, -75.66666666666665719, 4.330127018922192761 ) ) ;
#60245=CARTESIAN_POINT ( 'NONE',  ( 9.457646018065525792E-16, -4.062499998634408804, 5.148502694627439702 ) ) ;
#60248=CARTESIAN_POINT ( 'NONE',  ( -4.458734124999999437, -71.56249999863439371, 0.000000000000000000 ) ) ;
#60249=CARTESIAN_POINT ( 'NONE',  ( -4.999999999999999112, -28.79166666393548013, 2.886751345948131764 ) ) ;
#60252=CARTESIAN_POINT ( 'NONE',  ( -4.999999999999998224, -55.91666666666667140, 2.886751345948131764 ) ) ;
#60254=CARTESIAN_POINT ( 'NONE',  ( -4.458734124999999437, -51.31249999863440792, 0.000000000000000000 ) ) ;
#60255=CARTESIAN_POINT ( 'NONE',  ( -2.229367062499996610, -32.39583333196773651, 3.861377020970582219 ) ) ;
#60259=CARTESIAN_POINT ( 'NONE',  ( 1.060575238724906964E-15, 22.24999999999999645, 5.773502691896257311 ) ) ;
#60261=CARTESIAN_POINT ( 'NONE',  ( 2.229367062499998831, -40.64583333196773651, -3.861377020970580887 ) ) ;
#60262=CARTESIAN_POINT ( 'NONE',  ( -5.000000000000000000, -78.95833333060213022, -2.886751345948128211 ) ) ;
#60263=AXIS2_PLACEMENT_3D ( 'NONE', #27332, #46963, #2908 ) ;
#60267=CARTESIAN_POINT ( 'NONE',  ( 4.458734125000000326, -78.14583333196775072, 2.574251347313718519 ) ) ;
#60270=CARTESIAN_POINT ( 'NONE',  ( -5.000000000000000000, -27.08333333333333215, -2.886751345948128211 ) ) ;
#60274=ORIENTED_EDGE ( 'NONE', *, *, #50161, .T. ) ;
#60275=CARTESIAN_POINT ( 'NONE',  ( 5.000000000000000000, 22.62500000273118772, -6.123233995736766282E-16 ) ) ;
#60280=CARTESIAN_POINT ( 'NONE',  ( 6.123233995736766282E-16, -120.0000000000000000, -5.000000000000000000 ) ) ;
#60282=CARTESIAN_POINT ( 'NONE',  ( 4.648177544792955347E-16, 28.87500000273118417, -5.000000000000000000 ) ) ;
#60286=CARTESIAN_POINT ( 'NONE',  ( 4.458734124999998549, -15.97916666530107221, -2.574251347313721627 ) ) ;
#60294=DIRECTION ( 'NONE',  ( 0.000000000000000000, 0.000000000000000000, 1.000000000000000000 ) ) ;
#60295=VERTEX_POINT ( 'NONE', #24690 ) ;
#60297=CARTESIAN_POINT ( 'NONE',  ( 2.500000000000002220, -58.66666666666665719, 4.330127018922192761 ) ) ;
#60300=CARTESIAN_POINT ( 'NONE',  ( -6.972266317189433020E-16, -8.124999997268814056, -5.000000000000000000 ) ) ;
#60305=VERTEX_POINT ( 'NONE', #55247 ) ;
#60307=CARTESIAN_POINT ( 'NONE',  ( -1.339745962155613812, -110.0803417985302843, -5.000000000000000000 ) ) ;
#60308=CARTESIAN_POINT ( 'NONE',  ( -4.458734124999999437, 13.68750000136559386, 0.000000000000000000 ) ) ;
#60314=ORIENTED_EDGE ( 'NONE', *, *, #13018, .F. ) ;
#60315=ADVANCED_FACE ( 'NONE', ( #30790 ), #59108, .T. ) ;
#60316=CARTESIAN_POINT ( 'NONE',  ( 4.458734124999998549, -64.72916666530106511, -2.574251347313721627 ) ) ;
#60317=CARTESIAN_POINT ( 'NONE',  ( 6.123233995736766282E-16, -120.0000000000000000, -5.000000000000000000 ) ) ;
#60318=CARTESIAN_POINT ( 'NONE',  ( 4.458734124999998549, 11.27083333469892779, -2.574251347313721627 ) ) ;
#60319=CARTESIAN_POINT ( 'NONE',  ( -1.339745962155613812, -70.08034179853029855, -5.000000000000000000 ) ) ;
#60321=CARTESIAN_POINT ( 'NONE',  ( 4.458734124999998549, -52.97916666530107932, -2.574251347313721627 ) ) ;
#60322=CARTESIAN_POINT ( 'NONE',  ( 2.499999999999998668, -17.20833333060214443, -4.330127018922193649 ) ) ;
#60323=CARTESIAN_POINT ( 'NONE',  ( -2.500000000000000444, -109.1666666666666572, -4.330127018922193649 ) ) ;
#60325=CARTESIAN_POINT ( 'NONE',  ( 0.000000000000000000, -120.0000000000000000, 5.000000000000000000 ) ) ;
#60326=CARTESIAN_POINT ( 'NONE',  ( 5.000000000000000000, -64.37499999726881583, -6.123233995736766282E-16 ) ) ;
#60327=CARTESIAN_POINT ( 'NONE',  ( 2.229367062500001939, -16.22916666530107577, 3.861377020970579999 ) ) ;
#60328=ORIENTED_EDGE ( 'NONE', *, *, #10239, .F. ) ;
#60329=CARTESIAN_POINT ( 'NONE',  ( 0.000000000000000000, -120.0000000000000000, 0.000000000000000000 ) ) ;
#60330=CARTESIAN_POINT ( 'NONE',  ( 2.229367062500001939, -103.9791666653010651, 3.861377020970579999 ) ) ;
#60333=CARTESIAN_POINT ( 'NONE',  ( 4.458734124999998549, -101.9791666653010651, -2.574251347313721627 ) ) ;
#60334=CARTESIAN_POINT ( 'NONE',  ( 2.229367062500001939, -26.97916666530106866, 3.861377020970579999 ) ) ;
#60335=CARTESIAN_POINT ( 'NONE',  ( -3.535250795749689387E-16, -60.12499999726880162, -5.773502691896257311 ) ) ;
#60338=CARTESIAN_POINT ( 'NONE',  ( 4.458734124999999437, -22.81249999863440436, -5.460374474430324690E-16 ) ) ;
#60339=CARTESIAN_POINT ( 'NONE',  ( -2.229367062499996610, -62.39583333196774362, 3.861377020970582219 ) ) ;
#60340=CARTESIAN_POINT ( 'NONE',  ( -4.999999999999998224, -39.79166666393548013, 2.886751345948131764 ) ) ;
#60344=CARTESIAN_POINT ( 'NONE',  ( -2.499999999999996447, -10.83333333333333393, 4.330127018922195425 ) ) ;
#60348=( BOUNDED_CURVE ( )  B_SPLINE_CURVE ( 2, ( #12869, #41494, #56639, #8060, #23156, #51490, #46977, #12553, #13513 ),
 .UNSPECIFIED., .F., .F. ) 
 B_SPLINE_CURVE_WITH_KNOTS ( ( 3, 2, 2, 2, 3 ),
 ( 0.01964285714285714593, 0.02023809523809523905, 0.02142857142857142877, 0.02261904761904761849, 0.02321428571428571508 ),
 .UNSPECIFIED. ) 
 CURVE ( )  GEOMETRIC_REPRESENTATION_ITEM ( )  RATIONAL_B_SPLINE_CURVE ( ( 0.9330127018922194093, 0.9330127018922195203, 1.000000000000000000, 0.8660254037844387076, 1.000000000000000000, 0.8660254037844387076, 1.000000000000000000, 0.9330127018922191873, 0.9330127018922194093 ) ) 
 REPRESENTATION_ITEM ( '' )  );
#60349=AXIS2_PLACEMENT_3D ( 'NONE', #33005, #59669, #34898 ) ;
#60350=DIRECTION ( 'NONE',  ( -0.000000000000000000, 1.000000000000000000, -0.000000000000000000 ) ) ;
#60353=VECTOR ( 'NONE', #29196, 1000.000000000000000 ) ;
#60355=CARTESIAN_POINT ( 'NONE',  ( 1.339745962155612702, 1.830341803992665772, -5.000000000000000000 ) ) ;
#60360=CARTESIAN_POINT ( 'NONE',  ( 5.000000000000000888, -81.58333333333332860, 2.886751345948126879 ) ) ;
#60363=DIRECTION ( 'NONE',  ( -0.000000000000000000, 1.000000000000000000, -0.000000000000000000 ) ) ;
#60364=ORIENTED_EDGE ( 'NONE', *, *, #13796, .T. ) ;
#60365=CARTESIAN_POINT ( 'NONE',  ( 2.499999999999998668, -85.33333333333332860, -4.330127018922193649 ) ) ;
#60376=CARTESIAN_POINT ( 'NONE',  ( -8.660254037844341113, 30.00000000000000000, 6.047423072554883697E-14 ) ) ;
#60381=ORIENTED_EDGE ( 'NONE', *, *, #52040, .T. ) ;
#60382=CARTESIAN_POINT ( 'NONE',  ( 4.458734124999998549, -76.72916666530106511, -2.574251347313721627 ) ) ;
#60383=CARTESIAN_POINT ( 'NONE',  ( 9.457646018065525792E-16, -108.3124999986343937, 5.148502694627439702 ) ) ;
#60384=CARTESIAN_POINT ( 'NONE',  ( -5.000000000000000000, -53.99999999999999289, 0.000000000000000000 ) ) ;
#60390=CARTESIAN_POINT ( 'NONE',  ( 4.458734125000000326, -41.89583333196772941, 2.574251347313718519 ) ) ;
#60394=CARTESIAN_POINT ( 'NONE',  ( -4.458734124999999437, -47.39583333196774362, -2.574251347313719407 ) ) ;
#60396=CARTESIAN_POINT ( 'NONE',  ( 4.458734124999998549, 27.27083333469892423, -2.574251347313721627 ) ) ;
#60398=CARTESIAN_POINT ( 'NONE',  ( -2.229367062499996610, -17.14583333196773651, 3.861377020970582219 ) ) ;
#60399=CARTESIAN_POINT ( 'NONE',  ( 1.060575238724906964E-15, -98.75000000000000000, 5.773502691896257311 ) ) ;
#60401=CARTESIAN_POINT ( 'NONE',  ( -4.458734124999999437, -40.64583333196773651, -2.574251347313719407 ) ) ;
#60402=CARTESIAN_POINT ( 'NONE',  ( 5.000000000000000000, 0.7083333360645184262, -2.886751345948129988 ) ) ;
#60403=CARTESIAN_POINT ( 'NONE',  ( -5.000000000000000000, -6.958333330602150646, -2.886751345948128211 ) ) ;
#60406=CARTESIAN_POINT ( 'NONE',  ( 2.500000000000002220, -71.66666666666667140, 4.330127018922192761 ) ) ;
#60407=CARTESIAN_POINT ( 'NONE',  ( 4.458734125000000326, 1.854166668032262599, 2.574251347313718519 ) ) ;
#60409=CARTESIAN_POINT ( 'NONE',  ( 2.500000000000002220, 24.45833333606451987, 4.330127018922192761 ) ) ;
#60410=CARTESIAN_POINT ( 'NONE',  ( 1.339745962155615144, -57.70534180126147561, 4.999999999999999112 ) ) ;
#60411=CARTESIAN_POINT ( 'NONE',  ( -4.458734124999998549, -86.22916666530106511, 2.574251347313722516 ) ) ;
#60412=CARTESIAN_POINT ( 'NONE',  ( -4.458734124999999437, -37.31249999863440792, 0.000000000000000000 ) ) ;
#60413=DIRECTION ( 'NONE',  ( 0.000000000000000000, 0.000000000000000000, 1.000000000000000000 ) ) ;
#60414=CARTESIAN_POINT ( 'NONE',  ( 9.457646018065525792E-16, -85.31249999863439371, 5.148502694627439702 ) ) ;
#60418=CARTESIAN_POINT ( 'NONE',  ( -4.458734124999999437, -9.312499998634406140, 0.000000000000000000 ) ) ;
#60419=CARTESIAN_POINT ( 'NONE',  ( 4.458734124999999437, 22.93750000136559564, -5.460374474430324690E-16 ) ) ;
#60420=CARTESIAN_POINT ( 'NONE',  ( 2.229367062499998831, -46.89583333196774362, -3.861377020970580887 ) ) ;
#60421=CARTESIAN_POINT ( 'NONE',  ( -5.000000000000000000, 17.04166666939785202, -2.886751345948128211 ) ) ;
#60425=ORIENTED_EDGE ( 'NONE', *, *, #12576, .F. ) ;
#60428=CARTESIAN_POINT ( 'NONE',  ( -4.458734124999999437, -73.39583333196773651, -2.574251347313719407 ) ) ;
#60429=CARTESIAN_POINT ( 'NONE',  ( -2.229367062500000163, 27.27083333469892779, -3.861377020970580443 ) ) ;
#60435=CARTESIAN_POINT ( 'NONE',  ( 5.000000000000000000, -62.50000000000000000, -6.123233995736766282E-16 ) ) ;
#60439=CARTESIAN_POINT ( 'NONE',  ( -2.499999999999996447, -72.70833333060214443, 4.330127018922195425 ) ) ;
#60448=ORIENTED_EDGE ( 'NONE', *, *, #35378, .F. ) ;
#60450=CARTESIAN_POINT ( 'NONE',  ( 1.339745962155612702, -59.16965819600732601, -5.000000000000000000 ) ) ;
#60452=EDGE_LOOP ( 'NONE', ( #47697, #35040, #35121, #60520 ) ) ;
#60455=CARTESIAN_POINT ( 'NONE',  ( -4.458734124999999437, -48.56249999863440792, 0.000000000000000000 ) ) ;
#60456=CARTESIAN_POINT ( 'NONE',  ( -5.000000000000000000, 0.1250000027311869155, 0.000000000000000000 ) ) ;
#60461=VECTOR ( 'NONE', #46470, 1000.000000000000000 ) ;
#60463=CARTESIAN_POINT ( 'NONE',  ( -1.339745962155613812, -59.08034179853028434, -5.000000000000000000 ) ) ;
#60465=CARTESIAN_POINT ( 'NONE',  ( -4.458734124999999437, -94.56249999863440792, 0.000000000000000000 ) ) ;
#60467=ORIENTED_EDGE ( 'NONE', *, *, #51450, .F. ) ;
#60473=CARTESIAN_POINT ( 'NONE',  ( 4.458734124999998549, -4.729166665301071326, -2.574251347313721627 ) ) ;
#60474=( BOUNDED_CURVE ( )  B_SPLINE_CURVE ( 2, ( #21210, #17020, #22167, #7059, #40816, #31171, #50803, #60463, #1932 ),
 .UNSPECIFIED., .F., .F. ) 
 B_SPLINE_CURVE_WITH_KNOTS ( ( 3, 2, 2, 2, 3 ),
 ( 0.6267857142857142794, 0.6273809523809523725, 0.6285714285714285587, 0.6297619047619047450, 0.6303571428571428381 ),
 .UNSPECIFIED. ) 
 CURVE ( )  GEOMETRIC_REPRESENTATION_ITEM ( )  RATIONAL_B_SPLINE_CURVE ( ( 0.9330127018922194093, 0.9330127018922194093, 1.000000000000000000, 0.8660254037844387076, 1.000000000000000000, 0.8660254037844387076, 1.000000000000000000, 0.9330127018922194093, 0.9330127018922194093 ) ) 
 REPRESENTATION_ITEM ( '' )  );
#60475=CARTESIAN_POINT ( 'NONE',  ( -6.972266317189433020E-16, -106.2500000000000000, -5.000000000000000000 ) ) ;
#60476=CARTESIAN_POINT ( 'NONE',  ( 4.458734125000001214, -23.14583333196773651, 2.574251347313718519 ) ) ;
#60481=CARTESIAN_POINT ( 'NONE',  ( -2.229367062500000163, 14.27083333469892601, -3.861377020970580443 ) ) ;
#60482=EDGE_LOOP ( 'NONE', ( #26252, #45140, #7909, #48848 ) ) ;
#60483=DIRECTION ( 'NONE',  ( 0.000000000000000000, 0.000000000000000000, 1.000000000000000000 ) ) ;
#60484=CARTESIAN_POINT ( 'NONE',  ( 2.229367062500001939, -21.97916666530107221, 3.861377020970579999 ) ) ;
#60486=DIRECTION ( 'NONE',  ( -0.000000000000000000, 1.000000000000000000, -0.000000000000000000 ) ) ;
#60488=CARTESIAN_POINT ( 'NONE',  ( -3.535250795749689387E-16, -45.12499999726880162, -5.773502691896257311 ) ) ;
#60490=CARTESIAN_POINT ( 'NONE',  ( -2.229367062500000163, 6.520833334698928674, -3.861377020970580443 ) ) ;
#60491=CARTESIAN_POINT ( 'NONE',  ( 5.000000000000000000, -35.50000000000000711, -6.123233995736766282E-16 ) ) ;
#60492=CARTESIAN_POINT ( 'NONE',  ( -5.000000000000000000, -47.95833333060215153, -2.886751345948128211 ) ) ;
#60494=CARTESIAN_POINT ( 'NONE',  ( 4.458734124999998549, -69.72916666530107932, -2.574251347313721627 ) ) ;
#60496=CARTESIAN_POINT ( 'NONE',  ( 2.499999999999998668, 1.666666666666666963, -4.330127018922193649 ) ) ;
#60498=LINE ( 'NONE', #31210, #54114 ) ;
#60499=CARTESIAN_POINT ( 'NONE',  ( 2.229367062500001939, -58.97916666530106511, 3.861377020970579999 ) ) ;
#60500=CARTESIAN_POINT ( 'NONE',  ( 5.000000000000000888, -93.45833333060214443, 2.886751345948126879 ) ) ;
#60501=ADVANCED_FACE ( 'NONE', ( #46856 ), #43811, .T. ) ;
#60502=VECTOR ( 'NONE', #7264, 1000.000000000000000 ) ;
#60503=CARTESIAN_POINT ( 'NONE',  ( 0.000000000000000000, -120.0000000000000000, 0.000000000000000000 ) ) ;
#60504=LINE ( 'NONE', #56633, #21362 ) ;
#60507=CARTESIAN_POINT ( 'NONE',  ( -4.999999999999999112, -45.91666666666665719, 2.886751345948131764 ) ) ;
#60508=CARTESIAN_POINT ( 'NONE',  ( 2.499999999999998668, -13.33333333333333570, -4.330127018922193649 ) ) ;
#60509=CARTESIAN_POINT ( 'NONE',  ( -1.339745962155727277, -107.7946581987385173, 4.999999999999933387 ) ) ;
#60511=CARTESIAN_POINT ( 'NONE',  ( -4.458734124999999437, -109.3124999986343937, 0.000000000000000000 ) ) ;
#60512=CARTESIAN_POINT ( 'NONE',  ( 4.458734124999998549, -3.979166665301070438, -2.574251347313721627 ) ) ;
#60513=CARTESIAN_POINT ( 'NONE',  ( 5.000000000000000000, -73.29166666393548724, -2.886751345948130876 ) ) ;
#60517=EDGE_CURVE ( 'NONE', #46456, #28793, #31057, .T. ) ;
#60520=ORIENTED_EDGE ( 'NONE', *, *, #13712, .T. ) ;
#60521=CARTESIAN_POINT ( 'NONE',  ( 2.500000000000002220, -6.666666666666667851, 4.330127018922192761 ) ) ;
#60522=EDGE_CURVE ( 'NONE', #31783, #42322, #44188, .T. ) ;
#60526=CARTESIAN_POINT ( 'NONE',  ( -5.000000000000000000, -55.87499999726880162, 0.000000000000000000 ) ) ;
#60528=CARTESIAN_POINT ( 'NONE',  ( -3.152548672688508926E-16, -28.81249999863440436, -5.148502694627439702 ) ) ;
#60529=VECTOR ( 'NONE', #13027, 1000.000000000000000 ) ;
#60534=VECTOR ( 'NONE', #16391, 1000.000000000000000 ) ;
#60538=CARTESIAN_POINT ( 'NONE',  ( -1.339745962155613812, -94.08034179853028434, -5.000000000000000000 ) ) ;
#60540=CARTESIAN_POINT ( 'NONE',  ( -4.458734124999999437, -79.64583333196772230, -2.574251347313719407 ) ) ;
#60541=DIRECTION ( 'NONE',  ( -0.000000000000000000, 1.000000000000000000, -0.000000000000000000 ) ) ;
#60542=ORIENTED_EDGE ( 'NONE', *, *, #40149, .F. ) ;
#60546=CARTESIAN_POINT ( 'NONE',  ( -4.458734124999999437, -6.645833331967741842, -2.574251347313719407 ) ) ;
#60550=ORIENTED_EDGE ( 'NONE', *, *, #40533, .T. ) ;
#60558=CARTESIAN_POINT ( 'NONE',  ( 4.458734125000000326, -87.89583333196773651, 2.574251347313718519 ) ) ;
#60559=CARTESIAN_POINT ( 'NONE',  ( 5.000000000000000000, -29.29166666393548013, -2.886751345948130876 ) ) ;
#60560=CARTESIAN_POINT ( 'NONE',  ( -2.229367062500000163, -3.479166665301069994, -3.861377020970580443 ) ) ;
#60562=CARTESIAN_POINT ( 'NONE',  ( -2.500000000000000444, -31.04166666393548368, -4.330127018922193649 ) ) ;
#60563=CARTESIAN_POINT ( 'NONE',  ( 4.458734125000000326, 22.10416666803225993, 2.574251347313718519 ) ) ;
#60564=CARTESIAN_POINT ( 'NONE',  ( 1.975475456537005874E-15, -55.74999999999999289, 5.000000000000000000 ) ) ;
#60566=CARTESIAN_POINT ( 'NONE',  ( 4.458734124999998549, -50.72916666530107932, -2.574251347313721627 ) ) ;
#60567=CARTESIAN_POINT ( 'NONE',  ( 9.457646018065525792E-16, -36.31249999863440792, 5.148502694627439702 ) ) ;
#60570=( BOUNDED_CURVE ( )  B_SPLINE_CURVE ( 2, ( #39716, #29420, #59353, #44225, #49051, #5000, #191, #30068, #19790 ),
 .UNSPECIFIED., .F., .F. ) 
 B_SPLINE_CURVE_WITH_KNOTS ( ( 3, 2, 2, 2, 3 ),
 ( 0.7410714285714286031, 0.7416666666666666963, 0.7428571428571428825, 0.7440476190476190688, 0.7446428571428571619 ),
 .UNSPECIFIED. ) 
 CURVE ( )  GEOMETRIC_REPRESENTATION_ITEM ( )  RATIONAL_B_SPLINE_CURVE ( ( 0.9330127018922194093, 0.9330127018922194093, 1.000000000000000000, 0.8660254037844387076, 1.000000000000000000, 0.8660254037844387076, 1.000000000000000000, 0.9330127018922194093, 0.9330127018922194093 ) ) 
 REPRESENTATION_ITEM ( '' )  );
#60572=CARTESIAN_POINT ( 'NONE',  ( -2.500000000000000444, 18.83333333333333215, -4.330127018922193649 ) ) ;
#60575=AXIS2_PLACEMENT_3D ( 'NONE', #4619, #53205, #24244 ) ;
#60576=CARTESIAN_POINT ( 'NONE',  ( 2.229367062499998831, -41.64583333196773651, -3.861377020970580887 ) ) ;
#60577=CARTESIAN_POINT ( 'NONE',  ( -5.000000000000000000, -76.87499999726880162, 0.000000000000000000 ) ) ;
#60578=EDGE_CURVE ( 'NONE', #35769, #62971, #59430, .T. ) ;
#60582=CARTESIAN_POINT ( 'NONE',  ( 6.123233995736766282E-16, -120.0000000000000000, -5.000000000000000000 ) ) ;
#60584=CARTESIAN_POINT ( 'NONE',  ( 2.229367062500001939, -79.22916666530106511, 3.861377020970579999 ) ) ;
#60587=CARTESIAN_POINT ( 'NONE',  ( -5.000000000000000000, -29.08333333333332860, -2.886751345948128211 ) ) ;
#60592=CARTESIAN_POINT ( 'NONE',  ( 9.457646018065525792E-16, -89.06249999863439371, 5.148502694627439702 ) ) ;
#60593=CARTESIAN_POINT ( 'NONE',  ( -4.458734124999999437, 12.35416666803225993, -2.574251347313719407 ) ) ;
#60594=CARTESIAN_POINT ( 'NONE',  ( 5.000000000000000888, 15.54166666939785024, 2.886751345948126879 ) ) ;
#60595=CARTESIAN_POINT ( 'NONE',  ( -2.500000000000000444, -61.04166666393547303, -4.330127018922193649 ) ) ;
#60600=CARTESIAN_POINT ( 'NONE',  ( -6.972266317189433020E-16, -5.124999997268812280, -5.000000000000000000 ) ) ;
#60605=CARTESIAN_POINT ( 'NONE',  ( -6.972266317189433020E-16, -22.24999999999999645, -5.000000000000000000 ) ) ;
#60607=CARTESIAN_POINT ( 'NONE',  ( 2.499999999999998668, -74.33333333333332860, -4.330127018922193649 ) ) ;
#60609=CARTESIAN_POINT ( 'NONE',  ( -4.458734124999999437, -16.64583333196773651, -2.574251347313719407 ) ) ;
#60610=DIRECTION ( 'NONE',  ( -0.000000000000000000, 1.000000000000000000, -0.000000000000000000 ) ) ;
#60618=ORIENTED_EDGE ( 'NONE', *, *, #20787, .T. ) ;
#60619=CARTESIAN_POINT ( 'NONE',  ( -6.972266317189433020E-16, -4.249999999999997335, -5.000000000000000000 ) ) ;
#60620=CARTESIAN_POINT ( 'NONE',  ( 1.339745962155615144, -103.7053418012614827, 4.999999999999999112 ) ) ;
#60622=ORIENTED_EDGE ( 'NONE', *, *, #26451, .F. ) ;
#60626=CIRCLE ( 'NONE', #50319, 5.000000000000000000 ) ;
#60630=CARTESIAN_POINT ( 'NONE',  ( 4.458734124999998549, 16.27083333469892779, -2.574251347313721627 ) ) ;
#60633=CARTESIAN_POINT ( 'NONE',  ( 5.000000000000000000, -108.2916666639354730, -2.886751345948130876 ) ) ;
#60635=EDGE_LOOP ( 'NONE', ( #35848, #14131, #9002, #20567 ) ) ;
#60636=CARTESIAN_POINT ( 'NONE',  ( -4.458734124999999437, -65.39583333196773651, -2.574251347313719407 ) ) ;
#60638=CARTESIAN_POINT ( 'NONE',  ( 2.229367062499998831, 13.35416666803226171, -3.861377020970580887 ) ) ;
#60639=CARTESIAN_POINT ( 'NONE',  ( -6.972266317189433020E-16, -57.25000000000000000, -5.000000000000000000 ) ) ;
#60641=CARTESIAN_POINT ( 'NONE',  ( 9.457646018065525792E-16, -52.31249999863440792, 5.148502694627439702 ) ) ;
#60642=CARTESIAN_POINT ( 'NONE',  ( 5.000000000000000000, -13.37499999726881050, -6.123233995736766282E-16 ) ) ;
#60645=CARTESIAN_POINT ( 'NONE',  ( 2.229367062499998831, -19.89583333196774007, -3.861377020970580887 ) ) ;
#60646=VERTEX_POINT ( 'NONE', #56043 ) ;
#60648=CARTESIAN_POINT ( 'NONE',  ( 4.458734124999998549, -101.7291666653010793, -2.574251347313721627 ) ) ;
#60651=CARTESIAN_POINT ( 'NONE',  ( -4.458734124999999437, -104.5624999986344079, 0.000000000000000000 ) ) ;
#60652=CARTESIAN_POINT ( 'NONE',  ( -4.458734124999999437, -29.39583333196773296, -2.574251347313719407 ) ) ;
#60653=CARTESIAN_POINT ( 'NONE',  ( 5.000000000000000888, -64.45833333060213022, 2.886751345948126879 ) ) ;
#60658=CARTESIAN_POINT ( 'NONE',  ( -4.458734124999997661, -23.22916666530107221, 2.574251347313722516 ) ) ;
#60659=CARTESIAN_POINT ( 'NONE',  ( 4.458734124999999437, -66.06249999863440792, -5.460374474430324690E-16 ) ) ;
#60663=CARTESIAN_POINT ( 'NONE',  ( 5.000000000000000000, -9.500000000000001776, -6.123233995736766282E-16 ) ) ;
#60666=AXIS2_PLACEMENT_3D ( 'NONE', #32705, #37528, #52334 ) ;
#60672=DIRECTION ( 'NONE',  ( 0.000000000000000000, 0.000000000000000000, 1.000000000000000000 ) ) ;
#60679=ADVANCED_FACE ( 'NONE', ( #30304 ), #50894, .T. ) ;
#60680=ORIENTED_EDGE ( 'NONE', *, *, #18833, .F. ) ;
#60683=DIRECTION ( 'NONE',  ( -0.000000000000000000, 1.000000000000000000, -0.000000000000000000 ) ) ;
#60689=VERTEX_POINT ( 'NONE', #50574 ) ;
#60691=ORIENTED_EDGE ( 'NONE', *, *, #19949, .T. ) ;
#60695=ORIENTED_EDGE ( 'NONE', *, *, #53788, .T. ) ;
#60699=ORIENTED_EDGE ( 'NONE', *, *, #48201, .F. ) ;
#60700=CARTESIAN_POINT ( 'NONE',  ( 4.458734124999998549, -78.72916666530106511, -2.574251347313721627 ) ) ;
#60701=CARTESIAN_POINT ( 'NONE',  ( 4.458734124999998549, -107.9791666653010651, -2.574251347313721627 ) ) ;
#60706=VECTOR ( 'NONE', #50755, 1000.000000000000114 ) ;
#60709=CARTESIAN_POINT ( 'NONE',  ( 5.000000000000000000, 0.6250000027311873874, -6.123233995736766282E-16 ) ) ;
#60711=CARTESIAN_POINT ( 'NONE',  ( 9.457646018065525792E-16, -51.06249999863440792, 5.148502694627439702 ) ) ;
#60713=CARTESIAN_POINT ( 'NONE',  ( 2.499999999999998668, -105.3333333333333286, -4.330127018922193649 ) ) ;
#60715=CARTESIAN_POINT ( 'NONE',  ( 2.229367062500001939, -41.22916666530107932, 3.861377020970579999 ) ) ;
#60716=CARTESIAN_POINT ( 'NONE',  ( 2.499999999999998668, -1.208333330602148870, -4.330127018922193649 ) ) ;
#60720=CARTESIAN_POINT ( 'NONE',  ( 1.339745962155612702, -71.29465819873850307, -5.000000000000000000 ) ) ;
#60721=CARTESIAN_POINT ( 'NONE',  ( 4.458734125000000326, -95.89583333196773651, 2.574251347313718519 ) ) ;
#60722=CARTESIAN_POINT ( 'NONE',  ( -4.458734124999997661, -1.479166665301071992, 2.574251347313722516 ) ) ;
#60727=CARTESIAN_POINT ( 'NONE',  ( 4.458734124999998549, -87.72916666530107932, -2.574251347313721627 ) ) ;
#60728=CARTESIAN_POINT ( 'NONE',  ( 0.000000000000000000, -120.0000000000000000, 0.000000000000000000 ) ) ;
#60729=CARTESIAN_POINT ( 'NONE',  ( 9.457646018065525792E-16, -87.31249999863440792, 5.148502694627439702 ) ) ;
#60731=CARTESIAN_POINT ( 'NONE',  ( -6.031010364368858512E-14, 3.375000002731183280, 5.000000000000000000 ) ) ;
#60734=CARTESIAN_POINT ( 'NONE',  ( 4.458734125000000326, -6.895833331967734736, 2.574251347313718519 ) ) ;
#60735=CARTESIAN_POINT ( 'NONE',  ( 4.458734124999998549, 17.02083333469892423, -2.574251347313721627 ) ) ;
#60736=CARTESIAN_POINT ( 'NONE',  ( -4.458734124999999437, -48.64583333196773651, -2.574251347313719407 ) ) ;
#60744=CARTESIAN_POINT ( 'NONE',  ( 2.229367062499998831, -74.64583333196773651, -3.861377020970580887 ) ) ;
#60745=CARTESIAN_POINT ( 'NONE',  ( 1.060575238724906964E-15, -110.6249999972687874, 5.773502691896257311 ) ) ;
#60747=CARTESIAN_POINT ( 'NONE',  ( -1.339745962155610925, -57.66965819600732601, 5.000000000000000000 ) ) ;
#60750=CARTESIAN_POINT ( 'NONE',  ( -3.535250795749689387E-16, -66.25000000000000000, -5.773502691896257311 ) ) ;
#60751=DIRECTION ( 'NONE',  ( 0.000000000000000000, 0.000000000000000000, 1.000000000000000000 ) ) ;
#60754=FACE_OUTER_BOUND ( 'NONE', #63071, .T. ) ;
#60768=ORIENTED_EDGE ( 'NONE', *, *, #6440, .F. ) ;
#60771=CARTESIAN_POINT ( 'NONE',  ( 4.458734124999998549, -44.97916666530107221, -2.574251347313721627 ) ) ;
#60772=DIRECTION ( 'NONE',  ( -0.000000000000000000, 1.000000000000000000, -0.000000000000000000 ) ) ;
#60775=CARTESIAN_POINT ( 'NONE',  ( -5.000000000000000000, -21.87499999726881228, 0.000000000000000000 ) ) ;
#60782=CARTESIAN_POINT ( 'NONE',  ( 4.458734124999998549, -91.97916666530107932, -2.574251347313721627 ) ) ;
#60784=ORIENTED_EDGE ( 'NONE', *, *, #51104, .F. ) ;
#60788=CYLINDRICAL_SURFACE ( 'NONE', #4457, 5.000000000000000000 ) ;
#60789=CARTESIAN_POINT ( 'NONE',  ( 2.229367062500001939, -2.979166665301069550, 3.861377020970579999 ) ) ;
#60791=CARTESIAN_POINT ( 'NONE',  ( 9.457646018065525792E-16, -24.31249999863440792, 5.148502694627439702 ) ) ;
#60795=CARTESIAN_POINT ( 'NONE',  ( -1.339745962155610925, 17.20534180126147916, 5.000000000000000000 ) ) ;
#60797=CARTESIAN_POINT ( 'NONE',  ( 2.229367062499998831, 14.10416666803226171, -3.861377020970580887 ) ) ;
#60798=EDGE_LOOP ( 'NONE', ( #48957, #18267, #16542, #63357 ) ) ;
#60799=CARTESIAN_POINT ( 'NONE',  ( 1.975475456537005874E-15, -18.62499999726881228, 5.000000000000000000 ) ) ;
#60800=CARTESIAN_POINT ( 'NONE',  ( -5.000000000000000000, -84.99999999999998579, 0.000000000000000000 ) ) ;
#60801=CARTESIAN_POINT ( 'NONE',  ( 4.458734125000001214, -18.89583333196773651, 2.574251347313718519 ) ) ;
#60805=CARTESIAN_POINT ( 'NONE',  ( 5.000000000000000000, -44.29166666393546592, -2.886751345948129988 ) ) ;
#60807=CARTESIAN_POINT ( 'NONE',  ( -4.458734124999999437, 8.604166668032261711, -2.574251347313719407 ) ) ;
#60812=CARTESIAN_POINT ( 'NONE',  ( 4.458734125000001214, -64.89583333196773651, 2.574251347313718519 ) ) ;
#60815=CARTESIAN_POINT ( 'NONE',  ( 5.000000000000000000, -3.416666666666665186, -2.886751345948129988 ) ) ;
#60818=CARTESIAN_POINT ( 'NONE',  ( -2.229367062500000163, -58.47916666530106511, -3.861377020970580443 ) ) ;
#60819=CARTESIAN_POINT ( 'NONE',  ( 5.000000000000000000, -97.37499999726881583, -6.123233995736766282E-16 ) ) ;
#60820=DIRECTION ( 'NONE',  ( -0.000000000000000000, 1.000000000000000000, -0.000000000000000000 ) ) ;
#60824=CARTESIAN_POINT ( 'NONE',  ( -3.535250795749689387E-16, -50.25000000000000711, -5.773502691896257311 ) ) ;
#60825=CARTESIAN_POINT ( 'NONE',  ( -2.499999999999996447, 19.16666666666666430, 4.330127018922195425 ) ) ;
#60826=CARTESIAN_POINT ( 'NONE',  ( -2.480964764533239819E-13, -107.7500000000000000, 5.000000000000000000 ) ) ;
#60828=CARTESIAN_POINT ( 'NONE',  ( -4.458734124999998549, -104.2291666653010651, 2.574251347313722516 ) ) ;
#60829=CARTESIAN_POINT ( 'NONE',  ( 4.458734124999998549, -1.979166665301068662, -2.574251347313721627 ) ) ;
#60830=CARTESIAN_POINT ( 'NONE',  ( -1.339745962155613812, -100.0803417985302843, -5.000000000000000000 ) ) ;
#60833=CARTESIAN_POINT ( 'NONE',  ( -2.499999999999996447, -25.83333333333333215, 4.330127018922195425 ) ) ;
#60837=CARTESIAN_POINT ( 'NONE',  ( -4.999999999999998224, -16.79166666393548368, 2.886751345948131764 ) ) ;
#60839=ORIENTED_EDGE ( 'NONE', *, *, #9152, .T. ) ;
#60840=CARTESIAN_POINT ( 'NONE',  ( 0.000000000000000000, -120.0000000000000000, 5.000000000000000000 ) ) ;
#60842=CARTESIAN_POINT ( 'NONE',  ( 4.458734124999999437, -31.06249999863440436, -5.460374474430324690E-16 ) ) ;
#60843=CARTESIAN_POINT ( 'NONE',  ( -4.999999999999998224, -10.79166666393547835, 2.886751345948131764 ) ) ;
#60849=( BOUNDED_CURVE ( )  B_SPLINE_CURVE ( 2, ( #40583, #44451, #59258, #55395, #410, #15520, #49287, #58932, #30617 ),
 .UNSPECIFIED., .F., .F. ) 
 B_SPLINE_CURVE_WITH_KNOTS ( ( 3, 2, 2, 2, 3 ),
 ( 0.4303571428571428825, 0.4309523809523809756, 0.4321428571428571619, 0.4333333333333333481, 0.4339285714285714413 ),
 .UNSPECIFIED. ) 
 CURVE ( )  GEOMETRIC_REPRESENTATION_ITEM ( )  RATIONAL_B_SPLINE_CURVE ( ( 0.9330127018922194093, 0.9330127018922194093, 1.000000000000000000, 0.8660254037844387076, 1.000000000000000000, 0.8660254037844387076, 1.000000000000000000, 0.9330127018922194093, 0.9330127018922194093 ) ) 
 REPRESENTATION_ITEM ( '' )  );
#60850=CARTESIAN_POINT ( 'NONE',  ( 1.339745962155612702, -83.16965819600733312, -5.000000000000000000 ) ) ;
#60851=VERTEX_POINT ( 'NONE', #40284 ) ;
#60852=CARTESIAN_POINT ( 'NONE',  ( -2.229367062500000163, -77.72916666530106511, -3.861377020970580443 ) ) ;
#60855=DIRECTION ( 'NONE',  ( 0.000000000000000000, 0.000000000000000000, 1.000000000000000000 ) ) ;
#60858=EDGE_CURVE ( 'NONE', #45518, #43569, #26174, .T. ) ;
#60859=CARTESIAN_POINT ( 'NONE',  ( -2.229367062500000163, -11.72916666530107044, -3.861377020970580443 ) ) ;
#60860=ORIENTED_EDGE ( 'NONE', *, *, #7231, .T. ) ;
#60861=CARTESIAN_POINT ( 'NONE',  ( -2.499999999999996447, -9.708333330602146205, 4.330127018922195425 ) ) ;
#60864=CARTESIAN_POINT ( 'NONE',  ( -4.458734124999998549, -7.479166665301073991, 2.574251347313722516 ) ) ;
#60867=CARTESIAN_POINT ( 'NONE',  ( 5.000000000000000888, -64.58333333333332860, 2.886751345948126879 ) ) ;
#60869=DIRECTION ( 'NONE',  ( 0.000000000000000000, 0.000000000000000000, 1.000000000000000000 ) ) ;
#60871=CARTESIAN_POINT ( 'NONE',  ( -4.458734124999999437, -88.31249999863439371, 0.000000000000000000 ) ) ;
#60873=CARTESIAN_POINT ( 'NONE',  ( 2.229367062499998831, -1.645833331967737401, -3.861377020970580887 ) ) ;
#60876=CARTESIAN_POINT ( 'NONE',  ( 5.000000000000000888, -32.45833333060215153, 2.886751345948126879 ) ) ;
#60877=ADVANCED_FACE ( 'NONE', ( #1391 ), #36099, .T. ) ;
#60878=CARTESIAN_POINT ( 'NONE',  ( 6.123233995736766282E-16, -120.0000000000000000, -5.000000000000000000 ) ) ;
#60879=CARTESIAN_POINT ( 'NONE',  ( -2.229367062499996610, 23.85416666803225993, 3.861377020970582219 ) ) ;
#60881=CARTESIAN_POINT ( 'NONE',  ( 4.458734125000001214, -53.89583333196773651, 2.574251347313718519 ) ) ;
#60882=CARTESIAN_POINT ( 'NONE',  ( 4.458734125000000326, -35.14583333196772941, 2.574251347313718519 ) ) ;
#60884=CARTESIAN_POINT ( 'NONE',  ( -2.499999999999996447, -17.83333333333333215, 4.330127018922195425 ) ) ;
#60885=CARTESIAN_POINT ( 'NONE',  ( 2.499999999999998668, 16.66666666666666785, -4.330127018922193649 ) ) ;
#60888=CARTESIAN_POINT ( 'NONE',  ( 4.458734124999998549, -43.72916666530106511, -2.574251347313721627 ) ) ;
#60889=CARTESIAN_POINT ( 'NONE',  ( -3.535250795749689387E-16, -77.12499999726880162, -5.773502691896257311 ) ) ;
#60890=EDGE_CURVE ( 'NONE', #39916, #3550, #19962, .T. ) ;
#60894=CARTESIAN_POINT ( 'NONE',  ( -2.229367062499996610, -87.39583333196773651, 3.861377020970582219 ) ) ;
#60898=CARTESIAN_POINT ( 'NONE',  ( -2.499999999999996447, -32.83333333333332860, 4.330127018922195425 ) ) ;
#60902=VERTEX_POINT ( 'NONE', #615 ) ;
#60903=CARTESIAN_POINT ( 'NONE',  ( 4.458734124999998549, -92.72916666530107932, -2.574251347313721627 ) ) ;
#60904=CARTESIAN_POINT ( 'NONE',  ( 9.457646018065525792E-16, 11.68750000136559564, 5.148502694627439702 ) ) ;
#60905=( BOUNDED_CURVE ( )  B_SPLINE_CURVE ( 2, ( #34529, #48390, #14294, #34220, #43244, #54162, #33913, #9464, #4332 ),
 .UNSPECIFIED., .F., .F. ) 
 B_SPLINE_CURVE_WITH_KNOTS ( ( 3, 2, 2, 2, 3 ),
 ( 0.2089285714285714357, 0.2095238095238095288, 0.2107142857142857151, 0.2119047619047619013, 0.2124999999999999944 ),
 .UNSPECIFIED. ) 
 CURVE ( )  GEOMETRIC_REPRESENTATION_ITEM ( )  RATIONAL_B_SPLINE_CURVE ( ( 0.9330127018922194093, 0.9330127018922194093, 1.000000000000000000, 0.8660254037844387076, 1.000000000000000000, 0.8660254037844387076, 1.000000000000000000, 0.9330127018922194093, 0.9330127018922194093 ) ) 
 REPRESENTATION_ITEM ( '' )  );
#60906=CARTESIAN_POINT ( 'NONE',  ( 5.000000000000000000, 14.62500000273118594, -6.123233995736766282E-16 ) ) ;
#60914=CARTESIAN_POINT ( 'NONE',  ( -4.999999999999998224, -51.91666666666666430, 2.886751345948131764 ) ) ;
#60916=CARTESIAN_POINT ( 'NONE',  ( -6.972266317189433020E-16, -33.12499999726880873, -5.000000000000000000 ) ) ;
#60917=CARTESIAN_POINT ( 'NONE',  ( 2.499999999999998668, 28.79166666939784847, -4.330127018922193649 ) ) ;
#60919=CARTESIAN_POINT ( 'NONE',  ( 5.000000000000000888, -107.5833333333333428, 2.886751345948126879 ) ) ;
#60921=CARTESIAN_POINT ( 'NONE',  ( 4.458734124999998549, -11.97916666530107044, -2.574251347313721627 ) ) ;
#60922=CARTESIAN_POINT ( 'NONE',  ( 1.339745962155615144, -107.5803417985302985, 4.999999999999999112 ) ) ;
#60929=ORIENTED_EDGE ( 'NONE', *, *, #26376, .F. ) ;
#60931=ORIENTED_EDGE ( 'NONE', *, *, #50411, .T. ) ;
#60932=( BOUNDED_CURVE ( )  B_SPLINE_CURVE ( 2, ( #17623, #46891, #33042, #2834, #22452, #37240, #8285, #61692, #52657 ),
 .UNSPECIFIED., .F., .F. ) 
 B_SPLINE_CURVE_WITH_KNOTS ( ( 3, 2, 2, 2, 3 ),
 ( 0.01607142857142857331, 0.01666666666666666644, 0.01785714285714285615, 0.01904761904761904934, 0.01964285714285714593 ),
 .UNSPECIFIED. ) 
 CURVE ( )  GEOMETRIC_REPRESENTATION_ITEM ( )  RATIONAL_B_SPLINE_CURVE ( ( 0.9330127018922194093, 0.9330127018922195203, 1.000000000000000000, 0.8660254037844387076, 1.000000000000000000, 0.8660254037844387076, 1.000000000000000000, 0.9330127018922191873, 0.9330127018922194093 ) ) 
 REPRESENTATION_ITEM ( '' )  );
#60933=CARTESIAN_POINT ( 'NONE',  ( -3.152548672688508926E-16, -61.81249999863440081, -5.148502694627439702 ) ) ;
#60934=CARTESIAN_POINT ( 'NONE',  ( -4.999999999999998224, -27.91666666666666430, 2.886751345948131764 ) ) ;
#60935=CARTESIAN_POINT ( 'NONE',  ( 2.500000000000002220, -103.6666666666666572, 4.330127018922192761 ) ) ;
#60942=EDGE_CURVE ( 'NONE', #54724, #10579, #14746, .T. ) ;
#60943=VERTEX_POINT ( 'NONE', #296 ) ;
#60945=CARTESIAN_POINT ( 'NONE',  ( -2.229367062499996610, 10.85416666803225993, 3.861377020970582219 ) ) ;
#60948=CARTESIAN_POINT ( 'NONE',  ( -5.000000000000000000, -23.95833333060214443, -2.886751345948128211 ) ) ;
#60952=CARTESIAN_POINT ( 'NONE',  ( 4.458734124999999437, -71.81249999863439371, -5.460374474430324690E-16 ) ) ;
#60954=CARTESIAN_POINT ( 'NONE',  ( 2.229367062500001939, 10.02083333469892779, 3.861377020970579999 ) ) ;
#60956=CARTESIAN_POINT ( 'NONE',  ( 0.000000000000000000, -120.0000000000000000, 0.000000000000000000 ) ) ;
#60957=CARTESIAN_POINT ( 'NONE',  ( 9.457646018065525792E-16, -53.31249999863441502, 5.148502694627439702 ) ) ;
#60958=CARTESIAN_POINT ( 'NONE',  ( -5.000000000000000000, -15.95833333060214443, -2.886751345948128211 ) ) ;
#60959=ADVANCED_FACE ( 'NONE', ( #34055 ), #58816, .T. ) ;
#60963=CARTESIAN_POINT ( 'NONE',  ( 4.458734124999999437, -23.06249999863440436, -5.460374474430324690E-16 ) ) ;
#60965=CARTESIAN_POINT ( 'NONE',  ( 1.975475456537005874E-15, 6.249999999999998224, 5.000000000000000000 ) ) ;
#60966=CARTESIAN_POINT ( 'NONE',  ( -3.152548672688508926E-16, -106.5624999986343937, -5.148502694627439702 ) ) ;
#60968=ORIENTED_EDGE ( 'NONE', *, *, #14103, .F. ) ;
#60969=CARTESIAN_POINT ( 'NONE',  ( 4.458734124999999437, -102.0624999986344079, -5.460374474430324690E-16 ) ) ;
#60970=CARTESIAN_POINT ( 'NONE',  ( -4.458734124999998549, -26.22916666530106866, 2.574251347313722516 ) ) ;
#60971=CARTESIAN_POINT ( 'NONE',  ( 5.000000000000000000, -60.37499999726880873, -6.123233995736766282E-16 ) ) ;
#60974=CARTESIAN_POINT ( 'NONE',  ( -2.229367062499996610, -21.14583333196774007, 3.861377020970582219 ) ) ;
#60975=CARTESIAN_POINT ( 'NONE',  ( -4.458734124999997661, -67.47916666530106511, 2.574251347313722516 ) ) ;
#60978=CARTESIAN_POINT ( 'NONE',  ( 5.000000000000000888, -32.45833333060215153, 2.886751345948126879 ) ) ;
#60980=CARTESIAN_POINT ( 'NONE',  ( -2.500000000000000444, -11.16666666666666430, -4.330127018922193649 ) ) ;
#60984=CARTESIAN_POINT ( 'NONE',  ( -1.339745962155610925, -2.669658196007334450, 5.000000000000000000 ) ) ;
#60985=CARTESIAN_POINT ( 'NONE',  ( 1.339745962155612702, -92.29465819873853150, -5.000000000000000000 ) ) ;
#60987=EDGE_CURVE ( 'NONE', #2721, #34069, #20225, .T. ) ;
#60988=CARTESIAN_POINT ( 'NONE',  ( 1.975475456537005874E-15, -76.62499999726880162, 5.000000000000000000 ) ) ;
#60996=VERTEX_POINT ( 'NONE', #59145 ) ;
#60999=VECTOR ( 'NONE', #8634, 1000.000000000000000 ) ;
#61001=VERTEX_POINT ( 'NONE', #48843 ) ;
#61011=ORIENTED_EDGE ( 'NONE', *, *, #51725, .F. ) ;
#61014=CARTESIAN_POINT ( 'NONE',  ( 4.458734124999999437, -78.81249999863440792, -5.460374474430324690E-16 ) ) ;
#61015=CARTESIAN_POINT ( 'NONE',  ( -3.152548672688508926E-16, 25.43750000136559208, -5.148502694627439702 ) ) ;
#61016=EDGE_CURVE ( 'NONE', #15515, #62517, #9610, .T. ) ;
#61017=ORIENTED_EDGE ( 'NONE', *, *, #9495, .F. ) ;
#61018=CARTESIAN_POINT ( 'NONE',  ( -1.339745962155613812, 4.919658201469705006, -5.000000000000000000 ) ) ;
#61026=CARTESIAN_POINT ( 'NONE',  ( 9.457646018065525792E-16, -57.06249999863440081, 5.148502694627439702 ) ) ;
#61028=CARTESIAN_POINT ( 'NONE',  ( -2.229367062500000163, 27.52083333469892779, -3.861377020970580443 ) ) ;
#61029=ADVANCED_FACE ( 'NONE', ( #26006 ), #16032, .T. ) ;
#61032=CARTESIAN_POINT ( 'NONE',  ( 5.000000000000000000, -106.4999999999999858, -6.123233995736766282E-16 ) ) ;
#61034=CARTESIAN_POINT ( 'NONE',  ( -4.458734124999998549, -36.47916666530107221, 2.574251347313722516 ) ) ;
#61035=CARTESIAN_POINT ( 'NONE',  ( 5.000000000000000888, 0.5416666693978527958, 2.886751345948126879 ) ) ;
#61039=EDGE_CURVE ( 'NONE', #6898, #5972, #55917, .T. ) ;
#61040=CARTESIAN_POINT ( 'NONE',  ( 1.464175926609780648E-14, 24.74999999999999645, -5.000000000000000000 ) ) ;
#61041=CARTESIAN_POINT ( 'NONE',  ( 4.458734124999998549, -96.72916666530105090, -2.574251347313721627 ) ) ;
#61042=CARTESIAN_POINT ( 'NONE',  ( 9.457646018065525792E-16, -4.312499998634408804, 5.148502694627439702 ) ) ;
#61047=CARTESIAN_POINT ( 'NONE',  ( -4.458734124999999437, -93.39583333196773651, -2.574251347313719407 ) ) ;
#61050=CARTESIAN_POINT ( 'NONE',  ( 4.458734125000001214, -89.14583333196775072, 2.574251347313718519 ) ) ;
#61052=VECTOR ( 'NONE', #24688, 1000.000000000000000 ) ;
#61054=( BOUNDED_CURVE ( )  B_SPLINE_CURVE ( 2, ( #56246, #12167, #7359, #46906, #26968, #46587, #22468, #2530, #42065 ),
 .UNSPECIFIED., .F., .F. ) 
 B_SPLINE_CURVE_WITH_KNOTS ( ( 3, 2, 2, 2, 3 ),
 ( 0.01250000000000000069, 0.01309523809523809555, 0.01428571428571428527, 0.01547619047619047672, 0.01607142857142857331 ),
 .UNSPECIFIED. ) 
 CURVE ( )  GEOMETRIC_REPRESENTATION_ITEM ( )  RATIONAL_B_SPLINE_CURVE ( ( 0.9330127018922192983, 0.9330127018922194093, 1.000000000000000000, 0.8660254037844387076, 1.000000000000000000, 0.8660254037844387076, 1.000000000000000000, 0.9330127018922191873, 0.9330127018922194093 ) ) 
 REPRESENTATION_ITEM ( '' )  );
#61055=CARTESIAN_POINT ( 'NONE',  ( 2.229367062500001939, -5.979166665301072214, 3.861377020970579999 ) ) ;
#61056=CARTESIAN_POINT ( 'NONE',  ( -3.152548672688508926E-16, 15.18750000136559386, -5.148502694627439702 ) ) ;
#61057=CARTESIAN_POINT ( 'NONE',  ( -4.458734124999999437, -51.56249999863440792, 0.000000000000000000 ) ) ;
#61062=EDGE_LOOP ( 'NONE', ( #11066, #9759, #20442, #45167 ) ) ;
#61065=CARTESIAN_POINT ( 'NONE',  ( 4.458734124999998549, -79.72916666530107932, -2.574251347313721627 ) ) ;
#61066=CARTESIAN_POINT ( 'NONE',  ( -4.999999999999999112, -108.7916666639354730, 2.886751345948131764 ) ) ;
#61068=CARTESIAN_POINT ( 'NONE',  ( -1.339745962155613812, -94.20534180126146850, -5.000000000000000000 ) ) ;
#61071=CARTESIAN_POINT ( 'NONE',  ( -2.500000000000000444, -64.16666666666665719, -4.330127018922193649 ) ) ;
#61072=CARTESIAN_POINT ( 'NONE',  ( 2.499999999999998668, -63.20833333060215153, -4.330127018922193649 ) ) ;
#61084=CARTESIAN_POINT ( 'NONE',  ( 1.975475456537005874E-15, -28.74999999999999645, 5.000000000000000000 ) ) ;
#61089=CARTESIAN_POINT ( 'NONE',  ( -4.458734124999998549, -52.47916666530107221, 2.574251347313722516 ) ) ;
#61090=CARTESIAN_POINT ( 'NONE',  ( 1.975475456537005874E-15, 0.3750000027311862216, 5.000000000000000000 ) ) ;
#61092=CARTESIAN_POINT ( 'NONE',  ( -2.500000000000000444, -22.04166666393548013, -4.330127018922193649 ) ) ;
#61099=CARTESIAN_POINT ( 'NONE',  ( -4.458734124999999437, -96.56249999863440792, 0.000000000000000000 ) ) ;
#61104=( BOUNDED_CURVE ( )  B_SPLINE_CURVE ( 2, ( #41163, #13170, #2279, #37613, #22523, #52424, #21566, #32149, #42118 ),
 .UNSPECIFIED., .F., .F. ) 
 B_SPLINE_CURVE_WITH_KNOTS ( ( 3, 2, 2, 2, 3 ),
 ( 0.6553571428571428603, 0.6559523809523809534, 0.6571428571428571397, 0.6583333333333333259, 0.6589285714285714191 ),
 .UNSPECIFIED. ) 
 CURVE ( )  GEOMETRIC_REPRESENTATION_ITEM ( )  RATIONAL_B_SPLINE_CURVE ( ( 0.9330127018922194093, 0.9330127018922194093, 1.000000000000000000, 0.8660254037844387076, 1.000000000000000000, 0.8660254037844387076, 1.000000000000000000, 0.9330127018922194093, 0.9330127018922194093 ) ) 
 REPRESENTATION_ITEM ( '' )  );
#61106=CARTESIAN_POINT ( 'NONE',  ( -3.152548672688508926E-16, 0.4375000013655955255, -5.148502694627439702 ) ) ;
#61107=CARTESIAN_POINT ( 'NONE',  ( -4.458734124999999437, -94.56249999863440792, 0.000000000000000000 ) ) ;
#61109=CARTESIAN_POINT ( 'NONE',  ( 4.458734124999998549, -24.97916666530106511, -2.574251347313721627 ) ) ;
#61110=FACE_OUTER_BOUND ( 'NONE', #23187, .T. ) ;
#61117=CARTESIAN_POINT ( 'NONE',  ( -4.458734124999997661, 12.52083333469892601, 2.574251347313722516 ) ) ;
#61118=ORIENTED_EDGE ( 'NONE', *, *, #43702, .F. ) ;
#61119=CARTESIAN_POINT ( 'NONE',  ( 0.000000000000000000, -120.0000000000000000, 0.000000000000000000 ) ) ;
#61121=CARTESIAN_POINT ( 'NONE',  ( -4.999999999999999112, -85.91666666666667140, 2.886751345948131764 ) ) ;
#61122=CARTESIAN_POINT ( 'NONE',  ( 2.229367062499998831, -22.64583333196773651, -3.861377020970580887 ) ) ;
#61127=CARTESIAN_POINT ( 'NONE',  ( -3.535250795749689387E-16, -46.12499999726881583, -5.773502691896257311 ) ) ;
#61129=CARTESIAN_POINT ( 'NONE',  ( 9.457646018065525792E-16, 10.93750000136559208, 5.148502694627439702 ) ) ;
#61130=CARTESIAN_POINT ( 'NONE',  ( -6.972266317189433020E-16, -50.24999999999999289, -5.000000000000000000 ) ) ;
#61133=CARTESIAN_POINT ( 'NONE',  ( 4.458734125000001214, -66.89583333196773651, 2.574251347313718519 ) ) ;
#61135=( BOUNDED_CURVE ( )  B_SPLINE_CURVE ( 2, ( #32927, #33239, #42254, #7855, #38373, #52550, #42567, #12981, #2714 ),
 .UNSPECIFIED., .F., .F. ) 
 B_SPLINE_CURVE_WITH_KNOTS ( ( 3, 2, 2, 2, 3 ),
 ( 0.5374999999999999778, 0.5380952380952380709, 0.5392857142857142572, 0.5404761904761904434, 0.5410714285714285365 ),
 .UNSPECIFIED. ) 
 CURVE ( )  GEOMETRIC_REPRESENTATION_ITEM ( )  RATIONAL_B_SPLINE_CURVE ( ( 0.9330127018922194093, 0.9330127018922194093, 1.000000000000000000, 0.8660254037844387076, 1.000000000000000000, 0.8660254037844387076, 1.000000000000000000, 0.9330127018922194093, 0.9330127018922194093 ) ) 
 REPRESENTATION_ITEM ( '' )  );
#61136=CARTESIAN_POINT ( 'NONE',  ( 2.500000000000002220, -2.666666666666664298, 4.330127018922192761 ) ) ;
#61138=CARTESIAN_POINT ( 'NONE',  ( -1.339745962155610259, 25.91965820146970856, -5.000000000000002665 ) ) ;
#61139=CARTESIAN_POINT ( 'NONE',  ( 4.458734125000001214, -62.89583333196775072, 2.574251347313718519 ) ) ;
#61140=CARTESIAN_POINT ( 'NONE',  ( 5.000000000000000888, -94.45833333060213022, 2.886751345948126879 ) ) ;
#61141=CARTESIAN_POINT ( 'NONE',  ( -5.000000000000000000, -69.99999999999998579, 0.000000000000000000 ) ) ;
#61142=CARTESIAN_POINT ( 'NONE',  ( -5.000000000000000000, 30.00000000000000000, 0.000000000000000000 ) ) ;
#61146=CARTESIAN_POINT ( 'NONE',  ( 2.499999999999998668, -51.33333333333332860, -4.330127018922193649 ) ) ;
#61149=ORIENTED_EDGE ( 'NONE', *, *, #26834, .T. ) ;
#61150=CARTESIAN_POINT ( 'NONE',  ( 2.229367062499998831, -105.6458333319677365, -3.861377020970580887 ) ) ;
#61151=CARTESIAN_POINT ( 'NONE',  ( -2.229367062499996610, -3.395833331967738733, 3.861377020970582219 ) ) ;
#61155=CARTESIAN_POINT ( 'NONE',  ( 1.975475456537005874E-15, -30.62499999726881583, 5.000000000000000000 ) ) ;
#61159=CARTESIAN_POINT ( 'NONE',  ( 0.000000000000000000, -120.0000000000000000, 5.000000000000000000 ) ) ;
#61165=CARTESIAN_POINT ( 'NONE',  ( 2.229367062499998831, -29.89583333196773296, -3.861377020970580887 ) ) ;
#61166=CARTESIAN_POINT ( 'NONE',  ( 6.123233995736766282E-16, -120.0000000000000000, -5.000000000000000000 ) ) ;
#61174=CARTESIAN_POINT ( 'NONE',  ( 2.229367062499998831, -77.89583333196773651, -3.861377020970580887 ) ) ;
#61180=CARTESIAN_POINT ( 'NONE',  ( 4.458734124999998549, -9.979166665301068662, -2.574251347313721627 ) ) ;
#61184=CARTESIAN_POINT ( 'NONE',  ( 1.975475456537005874E-15, -1.749999999999999334, 5.000000000000000000 ) ) ;
#61185=CARTESIAN_POINT ( 'NONE',  ( -3.152548672688508926E-16, -8.812499998634406140, -5.148502694627439702 ) ) ;
#61190=CARTESIAN_POINT ( 'NONE',  ( 0.000000000000000000, -120.0000000000000000, 0.000000000000000000 ) ) ;
#61192=CARTESIAN_POINT ( 'NONE',  ( -3.152548672688508926E-16, -86.56249999863440792, -5.148502694627439702 ) ) ;
#61193=CARTESIAN_POINT ( 'NONE',  ( -5.000000000000000000, -78.00000000000000000, 0.000000000000000000 ) ) ;
#61194=CARTESIAN_POINT ( 'NONE',  ( 4.458734124999998549, -3.729166665301070438, -2.574251347313721627 ) ) ;
#61196=CARTESIAN_POINT ( 'NONE',  ( 5.000000000000000888, -31.45833333060214798, 2.886751345948126879 ) ) ;
#61198=CARTESIAN_POINT ( 'NONE',  ( -4.458734124999999437, 26.68750000136559564, 0.000000000000000000 ) ) ;
#61199=CARTESIAN_POINT ( 'NONE',  ( -6.972266317189433020E-16, -21.12499999726881228, -5.000000000000000000 ) ) ;
#61201=CARTESIAN_POINT ( 'NONE',  ( -4.458734124999999437, -49.31249999863440792, 0.000000000000000000 ) ) ;
#61202=CARTESIAN_POINT ( 'NONE',  ( -4.458734124999997661, -36.47916666530107221, 2.574251347313722516 ) ) ;
#61205=CARTESIAN_POINT ( 'NONE',  ( -2.499999999999996447, 14.16666666666666785, 4.330127018922195425 ) ) ;
#61208=CARTESIAN_POINT ( 'NONE',  ( -2.229367062500000163, -42.47916666530107932, -3.861377020970580443 ) ) ;
#61209=CARTESIAN_POINT ( 'NONE',  ( -2.499999999999996447, -76.70833333060214443, 4.330127018922195425 ) ) ;
#61213=CARTESIAN_POINT ( 'NONE',  ( 9.457646018065525792E-16, -86.31249999863439371, 5.148502694627439702 ) ) ;
#61215=CARTESIAN_POINT ( 'NONE',  ( 1.975475456537005874E-15, -95.75000000000000000, 5.000000000000000000 ) ) ;
#61216=CARTESIAN_POINT ( 'NONE',  ( -3.535250795749689387E-16, -30.24999999999999645, -5.773502691896257311 ) ) ;
#61222=CARTESIAN_POINT ( 'NONE',  ( 2.229367062499998831, -92.64583333196773651, -3.861377020970580887 ) ) ;
#61223=CARTESIAN_POINT ( 'NONE',  ( 4.458734124999999437, 14.93750000136559386, -5.460374474430324690E-16 ) ) ;
#61224=CARTESIAN_POINT ( 'NONE',  ( -5.000000000000000000, 14.04166666939785202, -2.886751345948128211 ) ) ;
#61225=CARTESIAN_POINT ( 'NONE',  ( -2.480964764533239819E-13, -59.75000000000000711, 5.000000000000000000 ) ) ;
#61229=( BOUNDED_CURVE ( )  B_SPLINE_CURVE ( 2, ( #13566, #3915, #58250, #28965, #48903, #9665, #57327, #8735, #43757 ),
 .UNSPECIFIED., .F., .F. ) 
 B_SPLINE_CURVE_WITH_KNOTS ( ( 3, 2, 2, 2, 3 ),
 ( 0.4232142857142857095, 0.4238095238095238027, 0.4249999999999999889, 0.4261904761904761751, 0.4267857142857142683 ),
 .UNSPECIFIED. ) 
 CURVE ( )  GEOMETRIC_REPRESENTATION_ITEM ( )  RATIONAL_B_SPLINE_CURVE ( ( 0.9330127018922194093, 0.9330127018922194093, 1.000000000000000000, 0.8660254037844387076, 1.000000000000000000, 0.8660254037844387076, 1.000000000000000000, 0.9330127018922194093, 0.9330127018922194093 ) ) 
 REPRESENTATION_ITEM ( '' )  );
#61236=DIRECTION ( 'NONE',  ( -0.000000000000000000, 1.000000000000000000, -0.000000000000000000 ) ) ;
#61237=CARTESIAN_POINT ( 'NONE',  ( -2.229367062499996610, -12.39583333196774007, 3.861377020970582219 ) ) ;
#61245=ORIENTED_EDGE ( 'NONE', *, *, #62997, .F. ) ;
#61248=CARTESIAN_POINT ( 'NONE',  ( 2.229367062500001939, -64.22916666530106511, 3.861377020970579999 ) ) ;
#61253=DIRECTION ( 'NONE',  ( -0.000000000000000000, 1.000000000000000000, -0.000000000000000000 ) ) ;
#61257=CARTESIAN_POINT ( 'NONE',  ( -4.999999999999998224, -109.7916666639354872, 2.886751345948131764 ) ) ;
#61258=CARTESIAN_POINT ( 'NONE',  ( 4.458734124999999437, 9.187500001365592084, -5.460374474430324690E-16 ) ) ;
#61262=DIRECTION ( 'NONE',  ( 0.000000000000000000, 0.000000000000000000, 1.000000000000000000 ) ) ;
#61263=AXIS2_PLACEMENT_3D ( 'NONE', #23093, #33061, #32741 ) ;
#61265=CARTESIAN_POINT ( 'NONE',  ( -2.229367062499996610, -71.14583333196773651, 3.861377020970582219 ) ) ;
#61266=DIRECTION ( 'NONE',  ( -0.000000000000000000, 1.000000000000000000, -0.000000000000000000 ) ) ;
#61267=CARTESIAN_POINT ( 'NONE',  ( -4.458734124999999437, 11.68750000136559564, 0.000000000000000000 ) ) ;
#61269=CARTESIAN_POINT ( 'NONE',  ( 1.975475456537005874E-15, -41.74999999999999289, 5.000000000000000000 ) ) ;
#61270=CARTESIAN_POINT ( 'NONE',  ( 4.458734124999998549, -56.97916666530107932, -2.574251347313721627 ) ) ;
#61271=CARTESIAN_POINT ( 'NONE',  ( 5.000000000000000000, -15.37499999726881228, -6.123233995736766282E-16 ) ) ;
#61272=CARTESIAN_POINT ( 'NONE',  ( -2.500000000000000444, -100.1666666666666572, -4.330127018922193649 ) ) ;
#61273=CYLINDRICAL_SURFACE ( 'NONE', #53212, 5.000000000000000000 ) ;
#61274=( BOUNDED_CURVE ( )  B_SPLINE_CURVE ( 2, ( #12020, #1766, #49672, #60934, #15588, #40010, #36162, #6261, #16539 ),
 .UNSPECIFIED., .F., .F. ) 
 B_SPLINE_CURVE_WITH_KNOTS ( ( 3, 2, 2, 2, 3 ),
 ( 0.4124999999999999778, 0.4130952380952380709, 0.4142857142857143127, 0.4154761904761904989, 0.4160714285714285920 ),
 .UNSPECIFIED. ) 
 CURVE ( )  GEOMETRIC_REPRESENTATION_ITEM ( )  RATIONAL_B_SPLINE_CURVE ( ( 0.9330127018922194093, 0.9330127018922194093, 1.000000000000000000, 0.8660254037844387076, 1.000000000000000000, 0.8660254037844387076, 1.000000000000000000, 0.9330127018922194093, 0.9330127018922194093 ) ) 
 REPRESENTATION_ITEM ( '' )  );
#61276=CARTESIAN_POINT ( 'NONE',  ( -2.229367062500000163, -19.72916666530107221, -3.861377020970580443 ) ) ;
#61277=( BOUNDED_CURVE ( )  B_SPLINE_CURVE ( 2, ( #1449, #45485, #21050, #21695, #11701, #50956, #60297, #40974, #55470 ),
 .UNSPECIFIED., .F., .F. ) 
 B_SPLINE_CURVE_WITH_KNOTS ( ( 3, 2, 2, 2, 3 ),
 ( 0.6303571428571428381, 0.6309523809523809312, 0.6321428571428571175, 0.6333333333333333037, 0.6339285714285713969 ),
 .UNSPECIFIED. ) 
 CURVE ( )  GEOMETRIC_REPRESENTATION_ITEM ( )  RATIONAL_B_SPLINE_CURVE ( ( 0.9330127018922194093, 0.9330127018922194093, 1.000000000000000000, 0.8660254037844387076, 1.000000000000000000, 0.8660254037844387076, 1.000000000000000000, 0.9330127018922194093, 0.9330127018922194093 ) ) 
 REPRESENTATION_ITEM ( '' )  );
#61279=CARTESIAN_POINT ( 'NONE',  ( -5.000000000000000000, -61.00000000000000000, 0.000000000000000000 ) ) ;
#61280=CARTESIAN_POINT ( 'NONE',  ( 2.229367062499998831, -106.6458333319677365, -3.861377020970580887 ) ) ;
#61283=CARTESIAN_POINT ( 'NONE',  ( 2.229367062499998831, -102.8958333319677365, -3.861377020970580887 ) ) ;
#61284=CARTESIAN_POINT ( 'NONE',  ( 4.458734124999999437, -25.81249999863440792, -5.460374474430324690E-16 ) ) ;
#61285=CARTESIAN_POINT ( 'NONE',  ( 1.060575238724906964E-15, -62.62499999726880873, 5.773502691896257311 ) ) ;
#61288=CARTESIAN_POINT ( 'NONE',  ( 9.457646018065525792E-16, -23.06249999863440792, 5.148502694627439702 ) ) ;
#61289=CARTESIAN_POINT ( 'NONE',  ( -4.458734124999999437, -70.56249999863439371, 0.000000000000000000 ) ) ;
#61294=CARTESIAN_POINT ( 'NONE',  ( 5.000000000000000000, -14.41666666666666963, -2.886751345948129988 ) ) ;
#61296=EDGE_LOOP ( 'NONE', ( #33622, #18451, #41658, #52454 ) ) ;
#61297=CYLINDRICAL_SURFACE ( 'NONE', #15328, 5.000000000000000000 ) ;
#61299=CARTESIAN_POINT ( 'NONE',  ( 1.339745962155612702, -84.16965819600731891, -5.000000000000000000 ) ) ;
#61301=EDGE_CURVE ( 'NONE', #58748, #44248, #37877, .T. ) ;
#61306=CARTESIAN_POINT ( 'NONE',  ( 1.975475456537005874E-15, -87.62499999726880162, 5.000000000000000000 ) ) ;
#61308=( BOUNDED_CURVE ( )  B_SPLINE_CURVE ( 2, ( #57427, #51960, #12401, #57113, #33282, #22378, #8215, #32331, #17554 ),
 .UNSPECIFIED., .F., .F. ) 
 B_SPLINE_CURVE_WITH_KNOTS ( ( 3, 2, 2, 2, 3 ),
 ( 0.2196428571428571397, 0.2202380952380952328, 0.2214285714285714191, 0.2226190476190476053, 0.2232142857142857262 ),
 .UNSPECIFIED. ) 
 CURVE ( )  GEOMETRIC_REPRESENTATION_ITEM ( )  RATIONAL_B_SPLINE_CURVE ( ( 0.9330127018922194093, 0.9330127018922194093, 1.000000000000000000, 0.8660254037844387076, 1.000000000000000000, 0.8660254037844387076, 1.000000000000000000, 0.9330127018922178550, 0.9330127018922194093 ) ) 
 REPRESENTATION_ITEM ( '' )  );
#61312=ORIENTED_EDGE ( 'NONE', *, *, #15706, .F. ) ;
#61318=ORIENTED_EDGE ( 'NONE', *, *, #52370, .T. ) ;
#61320=ADVANCED_FACE ( 'NONE', ( #32090 ), #33358, .T. ) ;
#61321=ORIENTED_EDGE ( 'NONE', *, *, #26460, .F. ) ;
#61325=CARTESIAN_POINT ( 'NONE',  ( 6.123233995736766282E-16, -120.0000000000000000, -5.000000000000000000 ) ) ;
#61329=CARTESIAN_POINT ( 'NONE',  ( -1.339745962155613812, 20.79465819873852084, -5.000000000000000000 ) ) ;
#61331=CARTESIAN_POINT ( 'NONE',  ( -4.458734124999999437, -75.39583333196773651, -2.574251347313719407 ) ) ;
#61332=CARTESIAN_POINT ( 'NONE',  ( -4.458734124999999437, 22.68750000136559564, 0.000000000000000000 ) ) ;
#61333=CARTESIAN_POINT ( 'NONE',  ( 5.000000000000000000, -18.41666666666666430, -2.886751345948130876 ) ) ;
#61335=CARTESIAN_POINT ( 'NONE',  ( 0.000000000000000000, -120.0000000000000000, 0.000000000000000000 ) ) ;
#61340=DIRECTION ( 'NONE',  ( -0.000000000000000000, 1.000000000000000000, -0.000000000000000000 ) ) ;
#61342=CARTESIAN_POINT ( 'NONE',  ( -4.458734124999999437, -53.31249999863439371, 0.000000000000000000 ) ) ;
#61344=CARTESIAN_POINT ( 'NONE',  ( 2.499999999999998668, -108.3333333333333428, -4.330127018922193649 ) ) ;
#61346=CARTESIAN_POINT ( 'NONE',  ( -3.152548672688508926E-16, -40.81249999863440081, -5.148502694627439702 ) ) ;
#61348=CARTESIAN_POINT ( 'NONE',  ( 5.000000000000000888, 1.541666669397853573, 2.886751345948126879 ) ) ;
#61353=CARTESIAN_POINT ( 'NONE',  ( 4.458734124999998549, -100.7291666653010651, -2.574251347313721627 ) ) ;
#61354=CARTESIAN_POINT ( 'NONE',  ( 4.458734125000000326, -8.145833331967736513, 2.574251347313718519 ) ) ;
#61355=ORIENTED_EDGE ( 'NONE', *, *, #601, .T. ) ;
#61356=VECTOR ( 'NONE', #19408, 1000.000000000000114 ) ;
#61357=CARTESIAN_POINT ( 'NONE',  ( -6.972266317189433020E-16, -36.12499999726880162, -5.000000000000000000 ) ) ;
#61358=CARTESIAN_POINT ( 'NONE',  ( 9.457646018065525792E-16, -94.06249999863439371, 5.148502694627439702 ) ) ;
#61359=CARTESIAN_POINT ( 'NONE',  ( 5.000000000000000000, 27.58333333333333215, -2.886751345948130876 ) ) ;
#61360=CARTESIAN_POINT ( 'NONE',  ( -3.152548672688508926E-16, -85.81249999863440792, -5.148502694627439702 ) ) ;
#61366=CARTESIAN_POINT ( 'NONE',  ( 2.229367062500001939, -9.979166665301068662, 3.861377020970579999 ) ) ;
#61367=CARTESIAN_POINT ( 'NONE',  ( -3.152548672688508926E-16, 18.18750000136559564, -5.148502694627439702 ) ) ;
#61368=CARTESIAN_POINT ( 'NONE',  ( -4.458734124999999437, -54.64583333196773651, -2.574251347313719407 ) ) ;
#61369=CARTESIAN_POINT ( 'NONE',  ( -5.000000000000000000, -105.9999999999999858, 0.000000000000000000 ) ) ;
#61376=CARTESIAN_POINT ( 'NONE',  ( -3.152548672688508926E-16, -81.56249999863440792, -5.148502694627439702 ) ) ;
#61377=CARTESIAN_POINT ( 'NONE',  ( 2.229367062500001939, 25.77083333469892779, 3.861377020970579999 ) ) ;
#61381=ADVANCED_FACE ( 'NONE', ( #23405 ), #62329, .T. ) ;
#61382=CARTESIAN_POINT ( 'NONE',  ( 0.000000000000000000, -120.0000000000000000, 0.000000000000000000 ) ) ;
#61385=CARTESIAN_POINT ( 'NONE',  ( -5.000000000000000000, -64.08333333333332860, -2.886751345948128211 ) ) ;
#61387=ORIENTED_EDGE ( 'NONE', *, *, #48439, .F. ) ;
#61388=FACE_OUTER_BOUND ( 'NONE', #20409, .T. ) ;
#61389=CARTESIAN_POINT ( 'NONE',  ( -6.972266317189433020E-16, -67.12499999726881583, -5.000000000000000000 ) ) ;
#61390=CARTESIAN_POINT ( 'NONE',  ( -2.500000000000000444, -72.16666666666667140, -4.330127018922193649 ) ) ;
#61404=CARTESIAN_POINT ( 'NONE',  ( 2.229367062500001939, -49.22916666530107221, 3.861377020970579999 ) ) ;
#61410=VECTOR ( 'NONE', #40309, 1000.000000000000000 ) ;
#61413=( BOUNDED_CURVE ( )  B_SPLINE_CURVE ( 2, ( #58674, #152, #49338, #34216, #10740, #30348, #467, #39674, #54810 ),
 .UNSPECIFIED., .F., .F. ) 
 B_SPLINE_CURVE_WITH_KNOTS ( ( 3, 2, 2, 2, 3 ),
 ( 0.2124999999999999944, 0.2130952380952380876, 0.2142857142857142738, 0.2154761904761904878, 0.2160714285714285809 ),
 .UNSPECIFIED. ) 
 CURVE ( )  GEOMETRIC_REPRESENTATION_ITEM ( )  RATIONAL_B_SPLINE_CURVE ( ( 0.9330127018922194093, 0.9330127018922194093, 1.000000000000000000, 0.8660254037844387076, 1.000000000000000000, 0.8660254037844387076, 1.000000000000000000, 0.9330127018922194093, 0.9330127018922194093 ) ) 
 REPRESENTATION_ITEM ( '' )  );
#61414=CARTESIAN_POINT ( 'NONE',  ( -4.999999999999998224, 1.083333333333331927, 2.886751345948131764 ) ) ;
#61416=CARTESIAN_POINT ( 'NONE',  ( 4.458734124999999437, -101.0624999986344079, -5.460374474430324690E-16 ) ) ;
#61417=CARTESIAN_POINT ( 'NONE',  ( 2.499999999999998668, -2.333333333333333037, -4.330127018922193649 ) ) ;
#61418=ORIENTED_EDGE ( 'NONE', *, *, #15730, .T. ) ;
#61422=CARTESIAN_POINT ( 'NONE',  ( 2.229367062499998831, -5.645833331967740953, -3.861377020970580887 ) ) ;
#61423=CARTESIAN_POINT ( 'NONE',  ( 4.458734124999999437, -94.06249999863440792, -5.460374474430324690E-16 ) ) ;
#61424=( BOUNDED_CURVE ( )  B_SPLINE_CURVE ( 2, ( #27984, #27045, #12877, #33140, #57594, #52448, #46663, #41826, #37638 ),
 .UNSPECIFIED., .F., .F. ) 
 B_SPLINE_CURVE_WITH_KNOTS ( ( 3, 2, 2, 2, 3 ),
 ( 0.2410714285714285754, 0.2416666666666666685, 0.2428571428571428548, 0.2440476190476190410, 0.2446428571428571341 ),
 .UNSPECIFIED. ) 
 CURVE ( )  GEOMETRIC_REPRESENTATION_ITEM ( )  RATIONAL_B_SPLINE_CURVE ( ( 0.9330127018922194093, 0.9330127018922194093, 1.000000000000000000, 0.8660254037844387076, 1.000000000000000000, 0.8660254037844387076, 1.000000000000000000, 0.9330127018922194093, 0.9330127018922194093 ) ) 
 REPRESENTATION_ITEM ( '' )  );
#61426=CARTESIAN_POINT ( 'NONE',  ( -2.229367062500000163, -20.72916666530107221, -3.861377020970580443 ) ) ;
#61432=CARTESIAN_POINT ( 'NONE',  ( -4.458734124999997661, 10.52083333469892779, 2.574251347313722516 ) ) ;
#61434=CYLINDRICAL_SURFACE ( 'NONE', #23339, 5.000000000000000000 ) ;
#61435=CARTESIAN_POINT ( 'NONE',  ( 5.000000000000000000, -61.50000000000000000, -6.123233995736766282E-16 ) ) ;
#61436=CARTESIAN_POINT ( 'NONE',  ( 5.000000000000000888, -89.58333333333334281, 2.886751345948126879 ) ) ;
#61437=CARTESIAN_POINT ( 'NONE',  ( 4.458734125000001214, -22.89583333196773651, 2.574251347313718519 ) ) ;
#61439=CARTESIAN_POINT ( 'NONE',  ( -2.229367062499996610, -70.39583333196773651, 3.861377020970582219 ) ) ;
#61443=CARTESIAN_POINT ( 'NONE',  ( 5.000000000000000000, -52.37499999726881583, -6.123233995736766282E-16 ) ) ;
#61444=CARTESIAN_POINT ( 'NONE',  ( -5.000000000000000000, -1.874999997268814944, 0.000000000000000000 ) ) ;
#61445=CARTESIAN_POINT ( 'NONE',  ( -3.152548672688508926E-16, 6.437500001365592972, -5.148502694627439702 ) ) ;
#61446=DIRECTION ( 'NONE',  ( -0.000000000000000000, 1.000000000000000000, -0.000000000000000000 ) ) ;
#61447=FACE_OUTER_BOUND ( 'NONE', #53091, .T. ) ;
#61449=CARTESIAN_POINT ( 'NONE',  ( -4.458734124999999437, -72.31249999863439371, 0.000000000000000000 ) ) ;
#61452=CARTESIAN_POINT ( 'NONE',  ( -5.000000000000000000, 0.000000000000000000, 0.000000000000000000 ) ) ;
#61455=CARTESIAN_POINT ( 'NONE',  ( -4.458734124999999437, -64.39583333196772230, -2.574251347313719407 ) ) ;
#61456=CARTESIAN_POINT ( 'NONE',  ( -5.000000000000000000, -97.87499999726881583, 0.000000000000000000 ) ) ;
#61457=CARTESIAN_POINT ( 'NONE',  ( 5.000000000000000000, 5.708333336064518981, -2.886751345948130876 ) ) ;
#61459=EDGE_CURVE ( 'NONE', #14760, #24668, #46899, .T. ) ;
#61462=CARTESIAN_POINT ( 'NONE',  ( -5.000000000000000000, -47.00000000000000000, 0.000000000000000000 ) ) ;
#61463=CARTESIAN_POINT ( 'NONE',  ( 2.500000000000002220, -72.54166666393548724, 4.330127018922192761 ) ) ;
#61466=CARTESIAN_POINT ( 'NONE',  ( 6.123233995736766282E-16, -120.0000000000000000, -5.000000000000000000 ) ) ;
#61467=DIRECTION ( 'NONE',  ( 0.000000000000000000, 0.000000000000000000, 1.000000000000000000 ) ) ;
#61470=CARTESIAN_POINT ( 'NONE',  ( -2.499999999999996447, -30.70833333060214443, 4.330127018922195425 ) ) ;
#61473=ORIENTED_EDGE ( 'NONE', *, *, #53079, .F. ) ;
#61479=EDGE_CURVE ( 'NONE', #19582, #42594, #24475, .T. ) ;
#61481=CARTESIAN_POINT ( 'NONE',  ( -2.229367062500000163, -33.72916666530107221, -3.861377020970580443 ) ) ;
#61482=CARTESIAN_POINT ( 'NONE',  ( 5.000000000000000000, -10.50000000000000178, -6.123233995736766282E-16 ) ) ;
#61484=( BOUNDED_CURVE ( )  B_SPLINE_CURVE ( 2, ( #19488, #14980, #20775, #15305, #25272, #35566, #15630, #54866, #9826 ),
 .UNSPECIFIED., .F., .F. ) 
 B_SPLINE_CURVE_WITH_KNOTS ( ( 3, 2, 2, 2, 3 ),
 ( 0.8803571428571428381, 0.8809523809523809312, 0.8821428571428571175, 0.8833333333333333037, 0.8839285714285713969 ),
 .UNSPECIFIED. ) 
 CURVE ( )  GEOMETRIC_REPRESENTATION_ITEM ( )  RATIONAL_B_SPLINE_CURVE ( ( 0.9330127018922194093, 0.9330127018922194093, 1.000000000000000000, 0.8660254037844387076, 1.000000000000000000, 0.8660254037844387076, 1.000000000000000000, 0.9330127018922194093, 0.9330127018922194093 ) ) 
 REPRESENTATION_ITEM ( '' )  );
#61493=CARTESIAN_POINT ( 'NONE',  ( -3.152548672688508926E-16, -81.81249999863440792, -5.148502694627439702 ) ) ;
#61500=CARTESIAN_POINT ( 'NONE',  ( -2.229367062500000163, -8.729166665301073991, -3.861377020970580443 ) ) ;
#61501=ORIENTED_EDGE ( 'NONE', *, *, #52922, .F. ) ;
#61503=CARTESIAN_POINT ( 'NONE',  ( 0.000000000000000000, -120.0000000000000000, 0.000000000000000000 ) ) ;
#61504=CARTESIAN_POINT ( 'NONE',  ( -2.229367062499996610, -9.395833331967736513, 3.861377020970582219 ) ) ;
#61507=CARTESIAN_POINT ( 'NONE',  ( -6.972266317189433020E-16, -88.25000000000000000, -5.000000000000000000 ) ) ;
#61509=( BOUNDED_CURVE ( )  B_SPLINE_CURVE ( 2, ( #7779, #21934, #32849, #42489, #56362, #27382, #18044, #61816, #41532 ),
 .UNSPECIFIED., .F., .F. ) 
 B_SPLINE_CURVE_WITH_KNOTS ( ( 3, 2, 2, 2, 3 ),
 ( 0.08750000000000000833, 0.08809523809523810145, 0.08928571428571428770, 0.09047619047619047394, 0.09107142857142856707 ),
 .UNSPECIFIED. ) 
 CURVE ( )  GEOMETRIC_REPRESENTATION_ITEM ( )  RATIONAL_B_SPLINE_CURVE ( ( 0.9330127018922192983, 0.9330127018922200755, 1.000000000000000000, 0.8660254037844387076, 1.000000000000000000, 0.8660254037844387076, 1.000000000000000000, 0.9330127018922194093, 0.9330127018922194093 ) ) 
 REPRESENTATION_ITEM ( '' )  );
#61510=CARTESIAN_POINT ( 'NONE',  ( -4.458734124999999437, 25.35416666803225993, -2.574251347313719407 ) ) ;
#61511=ORIENTED_EDGE ( 'NONE', *, *, #10608, .F. ) ;
#61512=CARTESIAN_POINT ( 'NONE',  ( -4.458734124999997661, -84.22916666530107932, 2.574251347313722516 ) ) ;
#61513=CARTESIAN_POINT ( 'NONE',  ( -5.000000000000000000, -78.08333333333332860, -2.886751345948128211 ) ) ;
#61514=CARTESIAN_POINT ( 'NONE',  ( -2.229367062500000163, -10.47916666530106866, -3.861377020970580443 ) ) ;
#61516=DIRECTION ( 'NONE',  ( 0.000000000000000000, 0.000000000000000000, 1.000000000000000000 ) ) ;
#61518=CARTESIAN_POINT ( 'NONE',  ( 1.060575238724906964E-15, -33.62499999726880873, 5.773502691896257311 ) ) ;
#61520=CARTESIAN_POINT ( 'NONE',  ( -4.458734124999999437, 26.60416666803225993, -2.574251347313719407 ) ) ;
#61521=CARTESIAN_POINT ( 'NONE',  ( -1.339745962155727277, -94.79465819873854571, 4.999999999999933387 ) ) ;
#61523=CARTESIAN_POINT ( 'NONE',  ( -3.152548672688508926E-16, -52.56249999863440792, -5.148502694627439702 ) ) ;
#61525=CARTESIAN_POINT ( 'NONE',  ( 5.000000000000000000, 16.50000000000000000, -6.123233995736766282E-16 ) ) ;
#61527=CARTESIAN_POINT ( 'NONE',  ( -6.972266317189433020E-16, -69.24999999999998579, -5.000000000000000000 ) ) ;
#61528=CARTESIAN_POINT ( 'NONE',  ( -4.458734124999999437, -49.39583333196773651, -2.574251347313719407 ) ) ;
#61529=CARTESIAN_POINT ( 'NONE',  ( 2.499999999999998668, -79.20833333060213022, -4.330127018922193649 ) ) ;
#61532=EDGE_CURVE ( 'NONE', #33389, #54885, #39116, .T. ) ;
#61534=CARTESIAN_POINT ( 'NONE',  ( -4.458734124999999437, -83.64583333196773651, -2.574251347313719407 ) ) ;
#61536=CARTESIAN_POINT ( 'NONE',  ( 5.000000000000000888, -32.58333333333333570, 2.886751345948126879 ) ) ;
#61540=CARTESIAN_POINT ( 'NONE',  ( 9.457646018065525792E-16, -98.06249999863440792, 5.148502694627439702 ) ) ;
#61541=CARTESIAN_POINT ( 'NONE',  ( -2.229367062500000163, 14.27083333469892601, -3.861377020970580443 ) ) ;
#61543=CARTESIAN_POINT ( 'NONE',  ( 5.000000000000000000, 18.70833333606451632, -2.886751345948129988 ) ) ;
#61548=CARTESIAN_POINT ( 'NONE',  ( -2.500000000000000444, -40.16666666666667140, -4.330127018922193649 ) ) ;
#61549=CARTESIAN_POINT ( 'NONE',  ( 2.499999999999998668, -78.33333333333332860, -4.330127018922193649 ) ) ;
#61554=CARTESIAN_POINT ( 'NONE',  ( 5.000000000000000000, -96.50000000000000000, -6.123233995736766282E-16 ) ) ;
#61556=CARTESIAN_POINT ( 'NONE',  ( 9.457646018065525792E-16, -20.31249999863440081, 5.148502694627439702 ) ) ;
#61563=ORIENTED_EDGE ( 'NONE', *, *, #58600, .F. ) ;
#61566=CARTESIAN_POINT ( 'NONE',  ( 2.229367062500001939, -62.22916666530106511, 3.861377020970579999 ) ) ;
#61573=FACE_OUTER_BOUND ( 'NONE', #49925, .T. ) ;
#61577=CARTESIAN_POINT ( 'NONE',  ( -4.458734124999998549, 7.770833334698925121, 2.574251347313722516 ) ) ;
#61580=CARTESIAN_POINT ( 'NONE',  ( 5.000000000000000000, -77.41666666666665719, -2.886751345948130876 ) ) ;
#61583=VERTEX_POINT ( 'NONE', #25285 ) ;
#61584=CARTESIAN_POINT ( 'NONE',  ( -3.152548672688508926E-16, -70.56249999863439371, -5.148502694627439702 ) ) ;
#61585=CARTESIAN_POINT ( 'NONE',  ( 1.339745962155612702, 14.83034180399266511, -5.000000000000000000 ) ) ;
#61586=CARTESIAN_POINT ( 'NONE',  ( 9.457646018065525792E-16, 5.937500001365592972, 5.148502694627439702 ) ) ;
#61588=AXIS2_PLACEMENT_3D ( 'NONE', #10404, #14583, #53518 ) ;
#61589=CARTESIAN_POINT ( 'NONE',  ( -2.229367062499996610, -60.39583333196774362, 3.861377020970582219 ) ) ;
#61590=CARTESIAN_POINT ( 'NONE',  ( -5.000000000000000000, -16.95833333060214443, -2.886751345948128211 ) ) ;
#61593=CARTESIAN_POINT ( 'NONE',  ( 5.000000000000000000, 19.70833333606451632, -2.886751345948130876 ) ) ;
#61595=CARTESIAN_POINT ( 'NONE',  ( 2.229367062500001939, -34.97916666530107221, 3.861377020970579999 ) ) ;
#61596=CARTESIAN_POINT ( 'NONE',  ( -3.152548672688508926E-16, -23.81249999863440792, -5.148502694627439702 ) ) ;
#61598=CARTESIAN_POINT ( 'NONE',  ( -2.229367062500000163, -109.4791666653010651, -3.861377020970580443 ) ) ;
#61600=VERTEX_POINT ( 'NONE', #63264 ) ;
#61601=CARTESIAN_POINT ( 'NONE',  ( -2.229367062500000163, -100.7291666653010651, -3.861377020970580443 ) ) ;
#61602=CARTESIAN_POINT ( 'NONE',  ( -2.229367062500000163, -33.47916666530107221, -3.861377020970580443 ) ) ;
#61603=CARTESIAN_POINT ( 'NONE',  ( 1.060575238724906964E-15, -60.62499999726880873, 5.773502691896257311 ) ) ;
#61607=CARTESIAN_POINT ( 'NONE',  ( -4.458734124999997661, -26.22916666530106866, 2.574251347313722516 ) ) ;
#61608=CARTESIAN_POINT ( 'NONE',  ( -2.229367062499996610, -68.39583333196773651, 3.861377020970582219 ) ) ;
#61613=CARTESIAN_POINT ( 'NONE',  ( -3.535250795749689387E-16, -17.25000000000000000, -5.773502691896257311 ) ) ;
#61619=CARTESIAN_POINT ( 'NONE',  ( 1.975475456537005874E-15, -51.62499999726880873, 5.000000000000000000 ) ) ;
#61621=CARTESIAN_POINT ( 'NONE',  ( -2.916731409357579869E-14, 18.25000000000000000, 5.000000000000000888 ) ) ;
#61623=CARTESIAN_POINT ( 'NONE',  ( 2.500000000000002220, 28.33333333333333215, 4.330127018922192761 ) ) ;
#61624=CARTESIAN_POINT ( 'NONE',  ( 1.339745962155612702, -14.29465819873851906, -5.000000000000000000 ) ) ;
#61625=CARTESIAN_POINT ( 'NONE',  ( 2.499999999999998668, -87.20833333060214443, -4.330127018922193649 ) ) ;
#61628=ORIENTED_EDGE ( 'NONE', *, *, #59774, .T. ) ;
#61629=CARTESIAN_POINT ( 'NONE',  ( -1.339745962155613812, -30.08034179853029144, -5.000000000000000000 ) ) ;
#61632=FACE_OUTER_BOUND ( 'NONE', #32989, .T. ) ;
#61639=VERTEX_POINT ( 'NONE', #10175 ) ;
#61642=CARTESIAN_POINT ( 'NONE',  ( -5.000000000000000000, -50.95833333060213732, -2.886751345948128211 ) ) ;
#61647=CARTESIAN_POINT ( 'NONE',  ( 9.457646018065525792E-16, -82.06249999863442213, 5.148502694627439702 ) ) ;
#61648=CARTESIAN_POINT ( 'NONE',  ( -3.152548672688508926E-16, 26.43750000136559208, -5.148502694627439702 ) ) ;
#61650=ORIENTED_EDGE ( 'NONE', *, *, #56183, .F. ) ;
#61655=FACE_OUTER_BOUND ( 'NONE', #4898, .T. ) ;
#61656=CARTESIAN_POINT ( 'NONE',  ( -4.999999999999998224, -82.91666666666667140, 2.886751345948131764 ) ) ;
#61657=( BOUNDED_CURVE ( )  B_SPLINE_CURVE ( 2, ( #59947, #54793, #24883, #55434, #39339, #34852, #444, #1417, #5905 ),
 .UNSPECIFIED., .F., .F. ) 
 B_SPLINE_CURVE_WITH_KNOTS ( ( 3, 2, 2, 2, 3 ),
 ( 0.4803571428571428714, 0.4809523809523809645, 0.4821428571428571508, 0.4833333333333333370, 0.4839285714285714302 ),
 .UNSPECIFIED. ) 
 CURVE ( )  GEOMETRIC_REPRESENTATION_ITEM ( )  RATIONAL_B_SPLINE_CURVE ( ( 0.9330127018922194093, 0.9330127018922194093, 1.000000000000000000, 0.8660254037844387076, 1.000000000000000000, 0.8660254037844387076, 1.000000000000000000, 0.9330127018922194093, 0.9330127018922194093 ) ) 
 REPRESENTATION_ITEM ( '' )  );
#61659=CARTESIAN_POINT ( 'NONE',  ( -2.229367062499996610, -55.14583333196773651, 3.861377020970582219 ) ) ;
#61661=CARTESIAN_POINT ( 'NONE',  ( -3.152548672688508926E-16, 26.43750000136559208, -5.148502694627439702 ) ) ;
#61662=ADVANCED_FACE ( 'NONE', ( #10486 ), #221, .T. ) ;
#61663=CARTESIAN_POINT ( 'NONE',  ( -3.535250795749689387E-16, -105.2500000000000000, -5.773502691896257311 ) ) ;
#61664=CARTESIAN_POINT ( 'NONE',  ( 6.123233995736766282E-16, -120.0000000000000000, -5.000000000000000000 ) ) ;
#61665=CARTESIAN_POINT ( 'NONE',  ( -2.229367062500000163, -39.72916666530107221, -3.861377020970580443 ) ) ;
#61666=CARTESIAN_POINT ( 'NONE',  ( 5.000000000000000888, 2.541666669397851130, 2.886751345948126879 ) ) ;
#61670=CARTESIAN_POINT ( 'NONE',  ( 4.458734125000000326, -102.8958333319677365, 2.574251347313718519 ) ) ;
#61671=CARTESIAN_POINT ( 'NONE',  ( 4.458734124999999437, -6.062499998634403475, -5.460374474430324690E-16 ) ) ;
#61674=CARTESIAN_POINT ( 'NONE',  ( 2.229367062500001939, -90.97916666530106511, 3.861377020970579999 ) ) ;
#61676=CARTESIAN_POINT ( 'NONE',  ( -4.458734124999999437, -84.64583333196773651, -2.574251347313719407 ) ) ;
#61678=LINE ( 'NONE', #22121, #24329 ) ;
#61681=CARTESIAN_POINT ( 'NONE',  ( -3.152548672688508926E-16, -10.56249999863440792, -5.148502694627439702 ) ) ;
#61682=CARTESIAN_POINT ( 'NONE',  ( 9.457646018065525792E-16, 16.68750000136559564, 5.148502694627439702 ) ) ;
#61684=CARTESIAN_POINT ( 'NONE',  ( -4.458734124999999437, -52.56249999863440792, 0.000000000000000000 ) ) ;
#61689=EDGE_LOOP ( 'NONE', ( #56360, #13826, #10344, #46728 ) ) ;
#61692=CARTESIAN_POINT ( 'NONE',  ( 1.339745962155611592, 26.41965820146970501, 5.000000000000000888 ) ) ;
#61693=CARTESIAN_POINT ( 'NONE',  ( -4.458734124999999437, -78.31249999863440792, 0.000000000000000000 ) ) ;
#61694=CARTESIAN_POINT ( 'NONE',  ( 4.458734125000001214, 25.85416666803225638, 2.574251347313718519 ) ) ;
#61695=ADVANCED_FACE ( 'NONE', ( #11124 ), #1502, .T. ) ;
#61701=CARTESIAN_POINT ( 'NONE',  ( -4.999999999999999112, -64.91666666666667140, 2.886751345948131764 ) ) ;
#61702=CARTESIAN_POINT ( 'NONE',  ( -5.000000000000000000, 30.00000000000000000, 0.000000000000000000 ) ) ;
#61709=CARTESIAN_POINT ( 'NONE',  ( 1.975475456537005874E-15, 5.250000000000000000, 5.000000000000000000 ) ) ;
#61716=ORIENTED_EDGE ( 'NONE', *, *, #58951, .T. ) ;
#61719=VECTOR ( 'NONE', #44245, 1000.000000000000000 ) ;
#61720=CARTESIAN_POINT ( 'NONE',  ( 4.458734124999998549, -53.97916666530107221, -2.574251347313721627 ) ) ;
#61722=CARTESIAN_POINT ( 'NONE',  ( -5.000000000000000000, 10.04166666939785024, -2.886751345948128211 ) ) ;
#61723=ORIENTED_EDGE ( 'NONE', *, *, #30719, .T. ) ;
#61730=CARTESIAN_POINT ( 'NONE',  ( -2.229367062499996610, -97.39583333196773651, 3.861377020970582219 ) ) ;
#61731=CARTESIAN_POINT ( 'NONE',  ( 2.500000000000002220, -2.666666666666664298, 4.330127018922192761 ) ) ;
#61737=CARTESIAN_POINT ( 'NONE',  ( -4.458734124999998549, -5.229166665301072214, 2.574251347313722516 ) ) ;
#61738=CARTESIAN_POINT ( 'NONE',  ( 9.457646018065525792E-16, -93.31249999863439371, 5.148502694627439702 ) ) ;
#61742=CARTESIAN_POINT ( 'NONE',  ( -4.458734124999999437, -21.56249999863440436, 0.000000000000000000 ) ) ;
#61743=CARTESIAN_POINT ( 'NONE',  ( -1.339745962155610925, -66.79465819873851729, 5.000000000000000000 ) ) ;
#61747=FACE_OUTER_BOUND ( 'NONE', #44454, .T. ) ;
#61749=CARTESIAN_POINT ( 'NONE',  ( -2.229367062500000163, 9.270833334698927786, -3.861377020970580443 ) ) ;
#61753=CARTESIAN_POINT ( 'NONE',  ( -5.000000000000000000, -88.08333333333332860, -2.886751345948128211 ) ) ;
#61754=CARTESIAN_POINT ( 'NONE',  ( -4.458734124999999437, -25.31249999863440792, 0.000000000000000000 ) ) ;
#61756=CARTESIAN_POINT ( 'NONE',  ( 4.458734124999999437, -73.06249999863439371, -5.460374474430324690E-16 ) ) ;
#61759=CARTESIAN_POINT ( 'NONE',  ( 2.229367062499998831, 4.354166668032260823, -3.861377020970580887 ) ) ;
#61764=CARTESIAN_POINT ( 'NONE',  ( -2.229367062499996610, -73.14583333196773651, 3.861377020970582219 ) ) ;
#61766=CARTESIAN_POINT ( 'NONE',  ( 1.060575238724906964E-15, 1.250000000000001110, 5.773502691896257311 ) ) ;
#61770=CARTESIAN_POINT ( 'NONE',  ( 2.229367062499998831, -66.64583333196773651, -3.861377020970580887 ) ) ;
#61771=CARTESIAN_POINT ( 'NONE',  ( 2.500000000000002220, -97.54166666393545881, 4.330127018922192761 ) ) ;
#61774=CARTESIAN_POINT ( 'NONE',  ( -2.229367062500000163, -105.7291666653010651, -3.861377020970580443 ) ) ;
#61776=CARTESIAN_POINT ( 'NONE',  ( 2.500000000000002220, -47.66666666666666430, 4.330127018922192761 ) ) ;
#61780=FACE_OUTER_BOUND ( 'NONE', #54974, .T. ) ;
#61783=( BOUNDED_CURVE ( )  B_SPLINE_CURVE ( 2, ( #19231, #33403, #57239, #33716, #53018, #8959, #28569, #48190, #53650 ),
 .UNSPECIFIED., .F., .F. ) 
 B_SPLINE_CURVE_WITH_KNOTS ( ( 3, 2, 2, 2, 3 ),
 ( 0.3267857142857142905, 0.3273809523809523836, 0.3285714285714285698, 0.3297619047619047561, 0.3303571428571428492 ),
 .UNSPECIFIED. ) 
 CURVE ( )  GEOMETRIC_REPRESENTATION_ITEM ( )  RATIONAL_B_SPLINE_CURVE ( ( 0.9330127018922194093, 0.9330127018922194093, 1.000000000000000000, 0.8660254037844387076, 1.000000000000000000, 0.8660254037844387076, 1.000000000000000000, 0.9330127018922194093, 0.9330127018922194093 ) ) 
 REPRESENTATION_ITEM ( '' )  );
#61784=FACE_OUTER_BOUND ( 'NONE', #5223, .T. ) ;
#61791=CYLINDRICAL_SURFACE ( 'NONE', #13503, 5.000000000000000000 ) ;
#61794=CARTESIAN_POINT ( 'NONE',  ( -4.458734124999999437, -34.56249999863440792, 0.000000000000000000 ) ) ;
#61795=CARTESIAN_POINT ( 'NONE',  ( -5.000000000000000000, -10.87499999726881583, 0.000000000000000000 ) ) ;
#61802=CARTESIAN_POINT ( 'NONE',  ( 1.339745962155615144, -70.58034179853028434, 4.999999999999999112 ) ) ;
#61803=CARTESIAN_POINT ( 'NONE',  ( -2.229367062499996610, -82.39583333196773651, 3.861377020970582219 ) ) ;
#61808=AXIS2_PLACEMENT_3D ( 'NONE', #31668, #28024, #3598 ) ;
#61810=CARTESIAN_POINT ( 'NONE',  ( 2.229367062500001939, -36.97916666530107221, 3.861377020970579999 ) ) ;
#61811=CARTESIAN_POINT ( 'NONE',  ( -4.458734124999999437, -8.645833331967736513, -2.574251347313719407 ) ) ;
#61813=LINE ( 'NONE', #32206, #20480 ) ;
#61814=EDGE_CURVE ( 'NONE', #45642, #26112, #56245, .T. ) ;
#61816=CARTESIAN_POINT ( 'NONE',  ( 1.339745962155615144, 17.29465819873852084, 4.999999999999999112 ) ) ;
#61817=CARTESIAN_POINT ( 'NONE',  ( 9.457646018065525792E-16, -4.312499998634408804, 5.148502694627439702 ) ) ;
#61824=CARTESIAN_POINT ( 'NONE',  ( 4.458734124999998549, 26.02083333469892779, -2.574251347313721627 ) ) ;
#61825=ORIENTED_EDGE ( 'NONE', *, *, #35378, .T. ) ;
#61826=CARTESIAN_POINT ( 'NONE',  ( -2.229367062500000163, -87.47916666530107932, -3.861377020970580443 ) ) ;
#61828=CARTESIAN_POINT ( 'NONE',  ( 4.458734124999999437, -10.81249999863440792, -5.460374474430324690E-16 ) ) ;
#61829=EDGE_CURVE ( 'NONE', #5205, #39251, #42619, .T. ) ;
#61831=ADVANCED_FACE ( 'NONE', ( #36855 ), #28455, .T. ) ;
#61834=CARTESIAN_POINT ( 'NONE',  ( -3.535250795749689387E-16, -36.12499999726880873, -5.773502691896257311 ) ) ;
#61836=CARTESIAN_POINT ( 'NONE',  ( -2.229367062500000163, 23.52083333469892779, -3.861377020970580443 ) ) ;
#61839=EDGE_CURVE ( 'NONE', #21770, #60996, #16406, .T. ) ;
#61840=CARTESIAN_POINT ( 'NONE',  ( -2.229367062500000163, -55.47916666530107221, -3.861377020970580443 ) ) ;
#61843=CARTESIAN_POINT ( 'NONE',  ( -5.000000000000000000, 15.00000000000000000, 0.000000000000000000 ) ) ;
#61847=CARTESIAN_POINT ( 'NONE',  ( 2.229367062500001939, -47.97916666530106511, 3.861377020970579999 ) ) ;
#61848=CARTESIAN_POINT ( 'NONE',  ( -2.500000000000000444, -85.04166666393547303, -4.330127018922193649 ) ) ;
#61853=CARTESIAN_POINT ( 'NONE',  ( 4.458734124999999437, -88.06249999863439371, -5.460374474430324690E-16 ) ) ;
#61855=CARTESIAN_POINT ( 'NONE',  ( -5.000000000000000000, -33.00000000000000000, 0.000000000000000000 ) ) ;
#61860=CARTESIAN_POINT ( 'NONE',  ( 4.458734124999998549, -95.72916666530109353, -2.574251347313721627 ) ) ;
#61861=CARTESIAN_POINT ( 'NONE',  ( 4.458734125000001214, 13.85416666803226171, 2.574251347313718519 ) ) ;
#61862=CARTESIAN_POINT ( 'NONE',  ( 2.499999999999998668, 18.79166666939785202, -4.330127018922193649 ) ) ;
#61864=CARTESIAN_POINT ( 'NONE',  ( 0.000000000000000000, -120.0000000000000000, 5.000000000000000000 ) ) ;
#61867=CARTESIAN_POINT ( 'NONE',  ( -6.972266317189433020E-16, -35.12499999726880873, -5.000000000000000000 ) ) ;
#61868=CARTESIAN_POINT ( 'NONE',  ( 5.000000000000000888, -82.58333333333332860, 2.886751345948126879 ) ) ;
#61869=CARTESIAN_POINT ( 'NONE',  ( 1.975475456537005874E-15, -75.62499999726880162, 5.000000000000000000 ) ) ;
#61871=CARTESIAN_POINT ( 'NONE',  ( 1.975475456537005874E-15, -25.62499999726881228, 5.000000000000000000 ) ) ;
#61874=CARTESIAN_POINT ( 'NONE',  ( 6.123233995736766282E-16, -120.0000000000000000, -5.000000000000000000 ) ) ;
#61875=CARTESIAN_POINT ( 'NONE',  ( 4.458734124999998549, -18.97916666530107221, -2.574251347313721627 ) ) ;
#61885=ORIENTED_EDGE ( 'NONE', *, *, #2070, .F. ) ;
#61886=CARTESIAN_POINT ( 'NONE',  ( 2.229367062500001939, -69.22916666530107932, 3.861377020970579999 ) ) ;
#61888=ORIENTED_EDGE ( 'NONE', *, *, #59045, .T. ) ;
#61889=( BOUNDED_CURVE ( )  B_SPLINE_CURVE ( 2, ( #38531, #13782, #33095, #27633, #52411, #52710, #42730, #17972, #62375 ),
 .UNSPECIFIED., .F., .F. ) 
 B_SPLINE_CURVE_WITH_KNOTS ( ( 3, 2, 2, 2, 3 ),
 ( 0.8375000000000000222, 0.8380952380952381153, 0.8392857142857143016, 0.8404761904761904878, 0.8410714285714285809 ),
 .UNSPECIFIED. ) 
 CURVE ( )  GEOMETRIC_REPRESENTATION_ITEM ( )  RATIONAL_B_SPLINE_CURVE ( ( 0.9330127018922194093, 0.9330127018922194093, 1.000000000000000000, 0.8660254037844387076, 1.000000000000000000, 0.8660254037844387076, 1.000000000000000000, 0.9330127018922194093, 0.9330127018922194093 ) ) 
 REPRESENTATION_ITEM ( '' )  );
#61892=CARTESIAN_POINT ( 'NONE',  ( -6.972266317189433020E-16, -39.12499999726880162, -5.000000000000000000 ) ) ;
#61894=ORIENTED_EDGE ( 'NONE', *, *, #55869, .T. ) ;
#61896=CARTESIAN_POINT ( 'NONE',  ( 9.457646018065525792E-16, 10.93750000136559208, 5.148502694627439702 ) ) ;
#61899=CARTESIAN_POINT ( 'NONE',  ( 5.000000000000000888, -78.45833333060214443, 2.886751345948126879 ) ) ;
#61902=CARTESIAN_POINT ( 'NONE',  ( -2.229367062499996610, -70.14583333196773651, 3.861377020970582219 ) ) ;
#61904=CARTESIAN_POINT ( 'NONE',  ( -4.458734124999999437, 7.687500001365594748, 0.000000000000000000 ) ) ;
#61905=CARTESIAN_POINT ( 'NONE',  ( 6.123233995736766282E-16, -120.0000000000000000, -5.000000000000000000 ) ) ;
#61906=CARTESIAN_POINT ( 'NONE',  ( -2.229367062500000163, -61.72916666530106511, -3.861377020970580443 ) ) ;
#61907=CARTESIAN_POINT ( 'NONE',  ( -2.500000000000000444, -21.04166666393548013, -4.330127018922193649 ) ) ;
#61908=CARTESIAN_POINT ( 'NONE',  ( 1.243387493232115550E-13, -19.25000000000000000, -5.000000000000000000 ) ) ;
#61910=CARTESIAN_POINT ( 'NONE',  ( 2.499999999999998668, 19.79166666939785202, -4.330127018922193649 ) ) ;
#61912=CARTESIAN_POINT ( 'NONE',  ( 2.229367062500001939, -42.97916666530107932, 3.861377020970579999 ) ) ;
#61913=CARTESIAN_POINT ( 'NONE',  ( 9.457646018065525792E-16, -24.31249999863440436, 5.148502694627439702 ) ) ;
#61916=CARTESIAN_POINT ( 'NONE',  ( -4.458734124999998549, -107.2291666653010509, 2.574251347313722516 ) ) ;
#61918=ORIENTED_EDGE ( 'NONE', *, *, #58198, .F. ) ;
#61919=CARTESIAN_POINT ( 'NONE',  ( 2.229367062500001939, -109.2291666653010651, 3.861377020970579999 ) ) ;
#61920=CARTESIAN_POINT ( 'NONE',  ( -2.229367062500000163, -32.47916666530106511, -3.861377020970580443 ) ) ;
#61921=CARTESIAN_POINT ( 'NONE',  ( 1.060575238724906964E-15, -67.62499999726881583, 5.773502691896257311 ) ) ;
#61924=EDGE_CURVE ( 'NONE', #8918, #2572, #55860, .T. ) ;
#61925=CARTESIAN_POINT ( 'NONE',  ( -4.458734124999999437, -29.39583333196773296, -2.574251347313719407 ) ) ;
#61926=CARTESIAN_POINT ( 'NONE',  ( -4.458734124999999437, -69.64583333196773651, -2.574251347313719407 ) ) ;
#61929=CARTESIAN_POINT ( 'NONE',  ( -5.000000000000000000, -33.08333333333332860, -2.886751345948128211 ) ) ;
#61930=CARTESIAN_POINT ( 'NONE',  ( -6.972266317189433020E-16, -5.124999997268812280, -5.000000000000000000 ) ) ;
#61931=CARTESIAN_POINT ( 'NONE',  ( -2.500000000000000444, -19.16666666666666430, -4.330127018922193649 ) ) ;
#61936=CARTESIAN_POINT ( 'NONE',  ( 1.339745962155615144, -84.58034179853028434, 4.999999999999999112 ) ) ;
#61941=CARTESIAN_POINT ( 'NONE',  ( 1.339745962155614700, 28.70534180126147561, -4.999999999999999112 ) ) ;
#61942=CARTESIAN_POINT ( 'NONE',  ( 1.975475456537005874E-15, -14.74999999999999822, 5.000000000000000000 ) ) ;
#61943=CARTESIAN_POINT ( 'NONE',  ( 2.500000000000002220, -87.54166666393547303, 4.330127018922192761 ) ) ;
#61945=ORIENTED_EDGE ( 'NONE', *, *, #57883, .F. ) ;
#61946=DIRECTION ( 'NONE',  ( -0.000000000000000000, 1.000000000000000000, -0.000000000000000000 ) ) ;
#61947=ORIENTED_EDGE ( 'NONE', *, *, #29034, .F. ) ;
#61952=EDGE_LOOP ( 'NONE', ( #30629, #13, #32353, #7530 ) ) ;
#61957=DIRECTION ( 'NONE',  ( 0.000000000000000000, 0.000000000000000000, 1.000000000000000000 ) ) ;
#61963=CARTESIAN_POINT ( 'NONE',  ( 4.458734124999998549, -82.72916666530106511, -2.574251347313721627 ) ) ;
#61964=CARTESIAN_POINT ( 'NONE',  ( 2.229367062500001939, 27.02083333469892423, 3.861377020970579999 ) ) ;
#61965=CARTESIAN_POINT ( 'NONE',  ( 1.975475456537005874E-15, -17.62499999726881938, 5.000000000000000000 ) ) ;
#61974=CARTESIAN_POINT ( 'NONE',  ( -3.152548672688508926E-16, -53.56249999863439371, -5.148502694627439702 ) ) ;
#61975=CARTESIAN_POINT ( 'NONE',  ( -4.458734124999998549, 20.77083333469892779, 2.574251347313722516 ) ) ;
#61976=CARTESIAN_POINT ( 'NONE',  ( -2.499999999999996447, -104.8333333333333286, 4.330127018922195425 ) ) ;
#61977=( BOUNDED_CURVE ( )  B_SPLINE_CURVE ( 2, ( #22512, #2574, #3211, #22190, #61435, #42421, #51774, #56611, #2899 ),
 .UNSPECIFIED., .F., .F. ) 
 B_SPLINE_CURVE_WITH_KNOTS ( ( 3, 2, 2, 2, 3 ),
 ( 0.6517857142857143016, 0.6523809523809523947, 0.6535714285714285809, 0.6547619047619047672, 0.6553571428571428603 ),
 .UNSPECIFIED. ) 
 CURVE ( )  GEOMETRIC_REPRESENTATION_ITEM ( )  RATIONAL_B_SPLINE_CURVE ( ( 0.9330127018922194093, 0.9330127018922194093, 1.000000000000000000, 0.8660254037844387076, 1.000000000000000000, 0.8660254037844387076, 1.000000000000000000, 0.9330127018922194093, 0.9330127018922194093 ) ) 
 REPRESENTATION_ITEM ( '' )  );
#61979=CARTESIAN_POINT ( 'NONE',  ( 4.458734124999998549, -41.97916666530107932, -2.574251347313721627 ) ) ;
#61980=CARTESIAN_POINT ( 'NONE',  ( -2.499999999999996447, -4.708333330602147981, 4.330127018922195425 ) ) ;
#61982=CYLINDRICAL_SURFACE ( 'NONE', #58369, 5.000000000000000000 ) ;
#61984=CARTESIAN_POINT ( 'NONE',  ( 9.457646018065525792E-16, -104.0624999986344079, 5.148502694627439702 ) ) ;
#61985=CARTESIAN_POINT ( 'NONE',  ( -3.152548672688508926E-16, -4.812499998634402587, -5.148502694627439702 ) ) ;
#61987=CARTESIAN_POINT ( 'NONE',  ( 1.975475456537005874E-15, -73.75000000000000000, 5.000000000000000000 ) ) ;
#61988=CARTESIAN_POINT ( 'NONE',  ( 4.458734125000001214, -94.89583333196773651, 2.574251347313718519 ) ) ;
#61990=CARTESIAN_POINT ( 'NONE',  ( -4.458734124999999437, -93.64583333196773651, -2.574251347313719407 ) ) ;
#61993=DIRECTION ( 'NONE',  ( -0.000000000000000000, 1.000000000000000000, -0.000000000000000000 ) ) ;
#61995=CARTESIAN_POINT ( 'NONE',  ( -4.458734124999999437, -11.39583333196774007, -2.574251347313719407 ) ) ;
#61996=CARTESIAN_POINT ( 'NONE',  ( -4.458734124999999437, 14.43750000136559386, 0.000000000000000000 ) ) ;
#61997=CARTESIAN_POINT ( 'NONE',  ( -4.458734124999999437, -52.64583333196773651, -2.574251347313719407 ) ) ;
#61998=CARTESIAN_POINT ( 'NONE',  ( 0.000000000000000000, -120.0000000000000000, 0.000000000000000000 ) ) ;
#62001=CARTESIAN_POINT ( 'NONE',  ( 1.975475456537005874E-15, -30.74999999999999645, 5.000000000000000000 ) ) ;
#62005=CARTESIAN_POINT ( 'NONE',  ( 1.975475456537005874E-15, -100.7499999999999858, 5.000000000000000000 ) ) ;
#62006=CARTESIAN_POINT ( 'NONE',  ( -2.229367062500000163, -77.47916666530106511, -3.861377020970580443 ) ) ;
#62007=CARTESIAN_POINT ( 'NONE',  ( 4.458734124999999437, 25.93750000136559564, -5.460374474430324690E-16 ) ) ;
#62012=CARTESIAN_POINT ( 'NONE',  ( -4.999999999999999112, -71.91666666666667140, 2.886751345948131764 ) ) ;
#62013=DIRECTION ( 'NONE',  ( 0.000000000000000000, 0.000000000000000000, 1.000000000000000000 ) ) ;
#62018=CARTESIAN_POINT ( 'NONE',  ( -5.000000000000000000, -72.08333333333332860, -2.886751345948128211 ) ) ;
#62022=CARTESIAN_POINT ( 'NONE',  ( -5.000000000000000000, 4.916666666666666075, -2.886751345948128211 ) ) ;
#62028=VERTEX_POINT ( 'NONE', #52906 ) ;
#62031=CARTESIAN_POINT ( 'NONE',  ( 4.458734125000001214, -50.14583333196773651, 2.574251347313718519 ) ) ;
#62032=( BOUNDED_CURVE ( )  B_SPLINE_CURVE ( 2, ( #45939, #35029, #25693, #45303, #11835, #21509, #5429, #25046, #618 ),
 .UNSPECIFIED., .F., .F. ) 
 B_SPLINE_CURVE_WITH_KNOTS ( ( 3, 2, 2, 2, 3 ),
 ( 0.4660714285714285809, 0.4666666666666666741, 0.4678571428571428603, 0.4690476190476190466, 0.4696428571428571397 ),
 .UNSPECIFIED. ) 
 CURVE ( )  GEOMETRIC_REPRESENTATION_ITEM ( )  RATIONAL_B_SPLINE_CURVE ( ( 0.9330127018922194093, 0.9330127018922194093, 1.000000000000000000, 0.8660254037844387076, 1.000000000000000000, 0.8660254037844387076, 1.000000000000000000, 0.9330127018922194093, 0.9330127018922194093 ) ) 
 REPRESENTATION_ITEM ( '' )  );
#62035=VERTEX_POINT ( 'NONE', #37177 ) ;
#62040=EDGE_CURVE ( 'NONE', #44900, #10824, #12719, .T. ) ;
#62043=CARTESIAN_POINT ( 'NONE',  ( -4.458734124999999437, -99.56249999863440792, 0.000000000000000000 ) ) ;
#62049=CARTESIAN_POINT ( 'NONE',  ( 9.457646018065525792E-16, -6.062499998634403475, 5.148502694627439702 ) ) ;
#62050=CARTESIAN_POINT ( 'NONE',  ( 2.229367062500001939, -95.22916666530106511, 3.861377020970579999 ) ) ;
#62053=CARTESIAN_POINT ( 'NONE',  ( 4.458734124999998549, -28.97916666530107577, -2.574251347313721627 ) ) ;
#62055=CARTESIAN_POINT ( 'NONE',  ( 2.500000000000002220, -46.66666666666666430, 4.330127018922192761 ) ) ;
#62059=DIRECTION ( 'NONE',  ( 0.000000000000000000, 0.000000000000000000, 1.000000000000000000 ) ) ;
#62061=CARTESIAN_POINT ( 'NONE',  ( 2.229367062499998831, 10.10416666803225993, -3.861377020970580887 ) ) ;
#62064=CARTESIAN_POINT ( 'NONE',  ( 0.000000000000000000, -114.9999999999999858, 0.000000000000000000 ) ) ;
#62065=CARTESIAN_POINT ( 'NONE',  ( -2.500000000000000444, -91.16666666666665719, -4.330127018922193649 ) ) ;
#62066=CARTESIAN_POINT ( 'NONE',  ( -4.458734124999998549, -23.22916666530107221, 2.574251347313722516 ) ) ;
#62068=CARTESIAN_POINT ( 'NONE',  ( 4.458734124999999437, -71.06249999863439371, -5.460374474430324690E-16 ) ) ;
#62069=CARTESIAN_POINT ( 'NONE',  ( 0.000000000000000000, -120.0000000000000000, 0.000000000000000000 ) ) ;
#62072=CARTESIAN_POINT ( 'NONE',  ( 4.458734125000000326, 3.104166668032260379, 2.574251347313718519 ) ) ;
#62074=CYLINDRICAL_SURFACE ( 'NONE', #53083, 5.000000000000000000 ) ;
#62076=CARTESIAN_POINT ( 'NONE',  ( -4.458734124999999437, -74.39583333196775072, -2.574251347313719407 ) ) ;
#62078=( BOUNDED_CURVE ( )  B_SPLINE_CURVE ( 2, ( #45110, #30951, #10699, #50897, #11327, #30307, #60244, #40914, #25488 ),
 .UNSPECIFIED., .F., .F. ) 
 B_SPLINE_CURVE_WITH_KNOTS ( ( 3, 2, 2, 2, 3 ),
 ( 0.7517857142857142794, 0.7523809523809523725, 0.7535714285714285587, 0.7547619047619047450, 0.7553571428571428381 ),
 .UNSPECIFIED. ) 
 CURVE ( )  GEOMETRIC_REPRESENTATION_ITEM ( )  RATIONAL_B_SPLINE_CURVE ( ( 0.9330127018922194093, 0.9330127018922194093, 1.000000000000000000, 0.8660254037844387076, 1.000000000000000000, 0.8660254037844387076, 1.000000000000000000, 0.9330127018922194093, 0.9330127018922194093 ) ) 
 REPRESENTATION_ITEM ( '' )  );
#62079=CARTESIAN_POINT ( 'NONE',  ( 5.000000000000000000, -7.500000000000000000, -6.123233995736766282E-16 ) ) ;
#62082=CARTESIAN_POINT ( 'NONE',  ( 4.458734125000001214, -61.89583333196773651, 2.574251347313718519 ) ) ;
#62083=CARTESIAN_POINT ( 'NONE',  ( 2.500000000000002220, -100.5416666639354588, 4.330127018922192761 ) ) ;
#62084=CARTESIAN_POINT ( 'NONE',  ( 5.000000000000000000, -41.49999999999999289, -6.123233995736766282E-16 ) ) ;
#62086=CARTESIAN_POINT ( 'NONE',  ( 4.458734124999999437, -108.0624999986343937, -5.460374474430324690E-16 ) ) ;
#62088=CARTESIAN_POINT ( 'NONE',  ( 2.499999999999998668, -48.33333333333332860, -4.330127018922193649 ) ) ;
#62093=DIRECTION ( 'NONE',  ( 0.000000000000000000, 0.000000000000000000, -1.000000000000000000 ) ) ;
#62098=CARTESIAN_POINT ( 'NONE',  ( 6.123233995736766282E-16, -120.0000000000000000, -5.000000000000000000 ) ) ;
#62104=ORIENTED_EDGE ( 'NONE', *, *, #26651, .T. ) ;
#62107=CARTESIAN_POINT ( 'NONE',  ( -2.229367062499996610, -38.39583333196773651, 3.861377020970582219 ) ) ;
#62111=EDGE_CURVE ( 'NONE', #62654, #7429, #29525, .T. ) ;
#62112=CARTESIAN_POINT ( 'NONE',  ( -6.972266317189433020E-16, -30.25000000000000000, -5.000000000000000000 ) ) ;
#62118=CARTESIAN_POINT ( 'NONE',  ( 4.458734124999998549, -84.97916666530106511, -2.574251347313721627 ) ) ;
#62121=CARTESIAN_POINT ( 'NONE',  ( -5.000000000000000000, -94.87499999726881583, 0.000000000000000000 ) ) ;
#62125=ORIENTED_EDGE ( 'NONE', *, *, #5916, .F. ) ;
#62127=DIRECTION ( 'NONE',  ( 0.000000000000000000, 0.000000000000000000, 1.000000000000000000 ) ) ;
#62128=CARTESIAN_POINT ( 'NONE',  ( 4.458734124999998549, -5.979166665301073103, -2.574251347313721627 ) ) ;
#62133=CARTESIAN_POINT ( 'NONE',  ( 4.458734124999999437, 24.93750000136559208, -5.460374474430324690E-16 ) ) ;
#62134=ORIENTED_EDGE ( 'NONE', *, *, #42834, .F. ) ;
#62135=CARTESIAN_POINT ( 'NONE',  ( -4.458734124999997661, -91.22916666530106511, 2.574251347313722516 ) ) ;
#62136=CARTESIAN_POINT ( 'NONE',  ( 5.000000000000000888, -60.45833333060213732, 2.886751345948126879 ) ) ;
#62137=CARTESIAN_POINT ( 'NONE',  ( -3.152548672688508926E-16, -7.562499998634404363, -5.148502694627439702 ) ) ;
#62138=EDGE_CURVE ( 'NONE', #3809, #55181, #38923, .T. ) ;
#62141=CARTESIAN_POINT ( 'NONE',  ( -5.000000000000000000, 15.00000000000000000, 0.000000000000000000 ) ) ;
#62142=CARTESIAN_POINT ( 'NONE',  ( -4.999999999999999112, -34.79166666393547303, 2.886751345948131764 ) ) ;
#62143=DIRECTION ( 'NONE',  ( 0.000000000000000000, 0.000000000000000000, 1.000000000000000000 ) ) ;
#62144=CARTESIAN_POINT ( 'NONE',  ( 4.458734124999999437, 17.18750000136559564, -5.460374474430324690E-16 ) ) ;
#62145=CARTESIAN_POINT ( 'NONE',  ( 5.000000000000000888, -7.583333333333330373, 2.886751345948126879 ) ) ;
#62148=CARTESIAN_POINT ( 'NONE',  ( -2.229367062499996610, -56.14583333196773651, 3.861377020970582219 ) ) ;
#62150=CARTESIAN_POINT ( 'NONE',  ( 0.000000000000000000, -120.0000000000000000, 0.000000000000000000 ) ) ;
#62151=CARTESIAN_POINT ( 'NONE',  ( 2.499999999999998668, 10.66666666666666430, -4.330127018922193649 ) ) ;
#62154=CARTESIAN_POINT ( 'NONE',  ( -4.458734124999998549, -48.22916666530106511, 2.574251347313722516 ) ) ;
#62155=CARTESIAN_POINT ( 'NONE',  ( 2.499999999999998668, -82.20833333060214443, -4.330127018922193649 ) ) ;
#62160=CARTESIAN_POINT ( 'NONE',  ( -3.152548672688508926E-16, -88.81249999863439371, -5.148502694627439702 ) ) ;
#62162=CARTESIAN_POINT ( 'NONE',  ( 2.499999999999998668, -35.33333333333332860, -4.330127018922193649 ) ) ;
#62164=ORIENTED_EDGE ( 'NONE', *, *, #5099, .F. ) ;
#62167=CARTESIAN_POINT ( 'NONE',  ( -3.152548672688508926E-16, -98.56249999863442213, -5.148502694627439702 ) ) ;
#62168=CARTESIAN_POINT ( 'NONE',  ( 4.458734124999999437, 6.937500001365594748, -5.460374474430324690E-16 ) ) ;
#62169=CARTESIAN_POINT ( 'NONE',  ( -4.999999999999999112, 10.20833333606451987, 2.886751345948131764 ) ) ;
#62172=CARTESIAN_POINT ( 'NONE',  ( -5.000000000000000000, -40.08333333333332860, -2.886751345948128211 ) ) ;
#62173=CARTESIAN_POINT ( 'NONE',  ( -5.000000000000000000, -81.08333333333332860, -2.886751345948128211 ) ) ;
#62177=CARTESIAN_POINT ( 'NONE',  ( -6.972266317189433020E-16, -61.25000000000000000, -5.000000000000000000 ) ) ;
#62178=CARTESIAN_POINT ( 'NONE',  ( -1.339745962155613812, -13.08034179853029144, -5.000000000000000000 ) ) ;
#62179=EDGE_CURVE ( 'NONE', #62654, #9564, #4634, .T. ) ;
#62182=CARTESIAN_POINT ( 'NONE',  ( -6.972266317189433020E-16, -107.2499999999999858, -5.000000000000000000 ) ) ;
#62183=CARTESIAN_POINT ( 'NONE',  ( -4.999999999999998224, -42.91666666666665719, 2.886751345948131764 ) ) ;
#62184=CARTESIAN_POINT ( 'NONE',  ( 4.458734124999999437, -21.06249999863440436, -5.460374474430324690E-16 ) ) ;
#62185=CARTESIAN_POINT ( 'NONE',  ( -4.999999999999998224, -57.91666666666665719, 2.886751345948131764 ) ) ;
#62191=VECTOR ( 'NONE', #11868, 1000.000000000000000 ) ;
#62194=VERTEX_POINT ( 'NONE', #5597 ) ;
#62195=DIRECTION ( 'NONE',  ( -0.000000000000000000, 1.000000000000000000, -0.000000000000000000 ) ) ;
#62197=EDGE_LOOP ( 'NONE', ( #10496, #32682, #16710, #19342 ) ) ;
#62198=CARTESIAN_POINT ( 'NONE',  ( 4.458734124999999437, -70.06249999863439371, -5.460374474430324690E-16 ) ) ;
#62199=CARTESIAN_POINT ( 'NONE',  ( 5.000000000000000888, -7.458333330602142652, 2.886751345948126879 ) ) ;
#62200=CARTESIAN_POINT ( 'NONE',  ( 0.000000000000000000, 0.000000000000000000, 0.000000000000000000 ) ) ;
#62202=VERTEX_POINT ( 'NONE', #35192 ) ;
#62203=EDGE_CURVE ( 'NONE', #1660, #52091, #42691, .T. ) ;
#62207=VERTEX_POINT ( 'NONE', #40326 ) ;
#62208=CARTESIAN_POINT ( 'NONE',  ( -2.229367062500000163, 9.520833334698927786, -3.861377020970580443 ) ) ;
#62209=( BOUNDED_CURVE ( )  B_SPLINE_CURVE ( 2, ( #57767, #48408, #8551, #9482, #3736, #52928, #17886, #62905, #42640 ),
 .UNSPECIFIED., .F., .F. ) 
 B_SPLINE_CURVE_WITH_KNOTS ( ( 3, 2, 2, 2, 3 ),
 ( 0.2946428571428571508, 0.2952380952380952439, 0.2964285714285714302, 0.2976190476190476164, 0.2982142857142857095 ),
 .UNSPECIFIED. ) 
 CURVE ( )  GEOMETRIC_REPRESENTATION_ITEM ( )  RATIONAL_B_SPLINE_CURVE ( ( 0.9330127018922194093, 0.9330127018922194093, 1.000000000000000000, 0.8660254037844387076, 1.000000000000000000, 0.8660254037844387076, 1.000000000000000000, 0.9330127018922194093, 0.9330127018922194093 ) ) 
 REPRESENTATION_ITEM ( '' )  );
#62215=CARTESIAN_POINT ( 'NONE',  ( 2.229367062500001939, -73.97916666530106511, 3.861377020970579999 ) ) ;
#62216=CARTESIAN_POINT ( 'NONE',  ( 5.000000000000000000, 14.70833333606451809, -2.886751345948130876 ) ) ;
#62217=CARTESIAN_POINT ( 'NONE',  ( 2.229367062500001939, 5.020833334698926897, 3.861377020970579999 ) ) ;
#62219=CARTESIAN_POINT ( 'NONE',  ( 9.457646018065525792E-16, -62.31249999863440792, 5.148502694627439702 ) ) ;
#62220=CARTESIAN_POINT ( 'NONE',  ( 5.000000000000000000, -22.37499999726881228, -6.123233995736766282E-16 ) ) ;
#62221=CARTESIAN_POINT ( 'NONE',  ( -4.999999999999998224, -18.91666666666666430, 2.886751345948131764 ) ) ;
#62222=DIRECTION ( 'NONE',  ( 0.000000000000000000, 0.000000000000000000, 1.000000000000000000 ) ) ;
#62226=CARTESIAN_POINT ( 'NONE',  ( -4.458734124999999437, -43.31249999863440081, 0.000000000000000000 ) ) ;
#62227=CARTESIAN_POINT ( 'NONE',  ( -4.458734124999999437, -25.56249999863440792, 0.000000000000000000 ) ) ;
#62228=CARTESIAN_POINT ( 'NONE',  ( -4.729367062499999719, 29.84375000068279604, 0.000000000000000000 ) ) ;
#62229=CARTESIAN_POINT ( 'NONE',  ( 4.458734124999998549, -106.7291666653010651, -2.574251347313721627 ) ) ;
#62231=ORIENTED_EDGE ( 'NONE', *, *, #37875, .T. ) ;
#62232=CARTESIAN_POINT ( 'NONE',  ( 4.458734124999999437, -110.0624999986343937, -5.460374474430324690E-16 ) ) ;
#62233=CARTESIAN_POINT ( 'NONE',  ( -2.229367062500000163, -34.47916666530107221, -3.861377020970580443 ) ) ;
#62234=CARTESIAN_POINT ( 'NONE',  ( -2.500000000000000444, -66.04166666393547303, -4.330127018922193649 ) ) ;
#62238=CARTESIAN_POINT ( 'NONE',  ( 2.229367062499998831, -30.64583333196773651, -3.861377020970580887 ) ) ;
#62239=CARTESIAN_POINT ( 'NONE',  ( -3.152548672688508926E-16, -70.81249999863439371, -5.148502694627439702 ) ) ;
#62244=CARTESIAN_POINT ( 'NONE',  ( 8.660254037844342889, 45.00000000000000000, 0.000000000000000000 ) ) ;
#62245=CARTESIAN_POINT ( 'NONE',  ( -5.000000000000000000, -16.08333333333333215, -2.886751345948128211 ) ) ;
#62248=LINE ( 'NONE', #17853, #32779 ) ;
#62250=CARTESIAN_POINT ( 'NONE',  ( -5.000000000000000000, 27.04166666939785202, -2.886751345948128211 ) ) ;
#62257=CARTESIAN_POINT ( 'NONE',  ( 2.499999999999998668, -14.33333333333333037, -4.330127018922193649 ) ) ;
#62259=ORIENTED_EDGE ( 'NONE', *, *, #12296, .F. ) ;
#62267=ORIENTED_EDGE ( 'NONE', *, *, #9879, .F. ) ;
#62269=ORIENTED_EDGE ( 'NONE', *, *, #6627, .F. ) ;
#62270=CARTESIAN_POINT ( 'NONE',  ( -5.000000000000000000, 0.04166666939785235169, -2.886751345948128211 ) ) ;
#62273=EDGE_CURVE ( 'NONE', #29833, #43959, #43072, .T. ) ;
#62274=EDGE_CURVE ( 'NONE', #43978, #454, #63187, .T. ) ;
#62276=FACE_OUTER_BOUND ( 'NONE', #23894, .T. ) ;
#62279=ORIENTED_EDGE ( 'NONE', *, *, #55435, .F. ) ;
#62281=CARTESIAN_POINT ( 'NONE',  ( -4.458734124999999437, -80.31249999863440792, 0.000000000000000000 ) ) ;
#62282=CARTESIAN_POINT ( 'NONE',  ( -4.458734124999999437, 24.68750000136559208, 0.000000000000000000 ) ) ;
#62283=VERTEX_POINT ( 'NONE', #62177 ) ;
#62284=CARTESIAN_POINT ( 'NONE',  ( -6.972266317189433020E-16, 14.74999999999999822, -5.000000000000000000 ) ) ;
#62288=CARTESIAN_POINT ( 'NONE',  ( 1.339745962155615144, -88.70534180126146850, 4.999999999999999112 ) ) ;
#62291=CARTESIAN_POINT ( 'NONE',  ( -2.229367062499996610, -56.14583333196773651, 3.861377020970582219 ) ) ;
#62293=CARTESIAN_POINT ( 'NONE',  ( 4.458734125000001214, 22.10416666803225993, 2.574251347313718519 ) ) ;
#62295=CARTESIAN_POINT ( 'NONE',  ( 4.458734124999998549, -43.97916666530105800, -2.574251347313721627 ) ) ;
#62296=CARTESIAN_POINT ( 'NONE',  ( -3.535250795749689387E-16, -5.124999997268809615, -5.773502691896257311 ) ) ;
#62297=CARTESIAN_POINT ( 'NONE',  ( 1.339745962155612702, -31.29465819873851373, -5.000000000000000000 ) ) ;
#62300=CARTESIAN_POINT ( 'NONE',  ( 4.458734124999998549, -101.7291666653010935, -2.574251347313721627 ) ) ;
#62301=CARTESIAN_POINT ( 'NONE',  ( -4.458734124999999437, -3.562499998634407916, 0.000000000000000000 ) ) ;
#62304=CARTESIAN_POINT ( 'NONE',  ( -4.458734124999999437, -91.31249999863440792, 0.000000000000000000 ) ) ;
#62306=CARTESIAN_POINT ( 'NONE',  ( 2.229367062500001939, -94.22916666530106511, 3.861377020970579999 ) ) ;
#62307=LINE ( 'NONE', #46240, #7914 ) ;
#62309=CARTESIAN_POINT ( 'NONE',  ( 4.458734124999998549, -11.72916666530107044, -2.574251347313721627 ) ) ;
#62310=CARTESIAN_POINT ( 'NONE',  ( -2.229367062499996610, 10.60416666803225993, 3.861377020970582219 ) ) ;
#62311=CARTESIAN_POINT ( 'NONE',  ( 4.458734124999999437, -55.06249999863440081, -5.460374474430324690E-16 ) ) ;
#62315=CARTESIAN_POINT ( 'NONE',  ( 5.000000000000000000, -84.41666666666667140, -2.886751345948130876 ) ) ;
#62316=ORIENTED_EDGE ( 'NONE', *, *, #468, .T. ) ;
#62320=CARTESIAN_POINT ( 'NONE',  ( 1.975475456537005874E-15, -68.74999999999998579, 5.000000000000000000 ) ) ;
#62322=CARTESIAN_POINT ( 'NONE',  ( 2.229367062500001939, -81.97916666530106511, 3.861377020970579999 ) ) ;
#62323=CARTESIAN_POINT ( 'NONE',  ( 4.458734124999999437, 24.93750000136559208, -5.460374474430324690E-16 ) ) ;
#62325=VECTOR ( 'NONE', #3137, 1000.000000000000000 ) ;
#62327=EDGE_CURVE ( 'NONE', #25261, #8589, #42539, .T. ) ;
#62328=CARTESIAN_POINT ( 'NONE',  ( -4.999999999999998224, 7.083333333333333925, 2.886751345948131764 ) ) ;
#62329=CYLINDRICAL_SURFACE ( 'NONE', #944, 5.000000000000000000 ) ;
#62331=CARTESIAN_POINT ( 'NONE',  ( 5.000000000000000000, -71.41666666666665719, -2.886751345948129988 ) ) ;
#62335=CARTESIAN_POINT ( 'NONE',  ( 1.975475456537005874E-15, -89.74999999999998579, 5.000000000000000000 ) ) ;
#62339=CARTESIAN_POINT ( 'NONE',  ( 5.000000000000000000, -62.50000000000000000, -6.123233995736766282E-16 ) ) ;
#62343=VERTEX_POINT ( 'NONE', #13596 ) ;
#62346=VERTEX_POINT ( 'NONE', #27124 ) ;
#62349=CARTESIAN_POINT ( 'NONE',  ( 4.458734124999999437, -54.06249999863440081, -5.460374474430324690E-16 ) ) ;
#62355=VERTEX_POINT ( 'NONE', #26808 ) ;
#62359=CARTESIAN_POINT ( 'NONE',  ( 4.458734124999999437, -100.0624999986344079, -5.460374474430324690E-16 ) ) ;
#62360=CARTESIAN_POINT ( 'NONE',  ( -5.000000000000000000, -68.87499999726880162, 0.000000000000000000 ) ) ;
#62361=ORIENTED_EDGE ( 'NONE', *, *, #10608, .T. ) ;
#62364=FACE_OUTER_BOUND ( 'NONE', #18443, .T. ) ;
#62365=AXIS2_PLACEMENT_3D ( 'NONE', #60728, #55266, #7644 ) ;
#62366=CARTESIAN_POINT ( 'NONE',  ( -2.229367062499996610, -8.145833331967736513, 3.861377020970582219 ) ) ;
#62367=CARTESIAN_POINT ( 'NONE',  ( -2.229367062500000163, -93.72916666530106511, -3.861377020970580443 ) ) ;
#62369=CARTESIAN_POINT ( 'NONE',  ( -4.458734124999999437, -30.64583333196774007, -2.574251347313719407 ) ) ;
#62375=CARTESIAN_POINT ( 'NONE',  ( 1.975475456537005874E-15, -88.62499999726880162, 5.000000000000000000 ) ) ;
#62377=CARTESIAN_POINT ( 'NONE',  ( -2.229367062499996610, 10.60416666803225993, 3.861377020970582219 ) ) ;
#62379=CARTESIAN_POINT ( 'NONE',  ( 4.330127018922154569, 45.00000000000000000, -7.499999999999971578 ) ) ;
#62380=CARTESIAN_POINT ( 'NONE',  ( 2.499999999999998668, -66.20833333060213022, -4.330127018922193649 ) ) ;
#62381=CARTESIAN_POINT ( 'NONE',  ( -5.000000000000000000, -92.00000000000000000, 0.000000000000000000 ) ) ;
#62382=CARTESIAN_POINT ( 'NONE',  ( -4.458734124999999437, -26.39583333196773651, -2.574251347313719407 ) ) ;
#62384=CARTESIAN_POINT ( 'NONE',  ( -2.229367062499996610, -75.39583333196773651, 3.861377020970582219 ) ) ;
#62385=ADVANCED_FACE ( 'NONE', ( #56723 ), #46740, .T. ) ;
#62389=CARTESIAN_POINT ( 'NONE',  ( 9.457646018065525792E-16, 0.9375000013655959696, 5.148502694627439702 ) ) ;
#62390=CARTESIAN_POINT ( 'NONE',  ( -4.458734124999999437, 28.35416666803226349, -2.574251347313719407 ) ) ;
#62391=CARTESIAN_POINT ( 'NONE',  ( 2.229367062499998831, -35.89583333196773651, -3.861377020970580887 ) ) ;
#62392=CARTESIAN_POINT ( 'NONE',  ( -6.972266317189433020E-16, -4.124999997268814056, -5.000000000000000000 ) ) ;
#62394=CARTESIAN_POINT ( 'NONE',  ( 4.458734125000001214, -70.89583333196773651, 2.574251347313718519 ) ) ;
#62396=CARTESIAN_POINT ( 'NONE',  ( 5.000000000000000000, -7.416666666666667851, -2.886751345948129988 ) ) ;
#62399=CARTESIAN_POINT ( 'NONE',  ( -4.458734124999999437, -62.31249999863440792, 0.000000000000000000 ) ) ;
#62400=CARTESIAN_POINT ( 'NONE',  ( 2.500000000000002220, -101.5416666639354588, 4.330127018922192761 ) ) ;
#62404=CARTESIAN_POINT ( 'NONE',  ( 2.229367062500001939, -105.2291666653010651, 3.861377020970579999 ) ) ;
#62406=CARTESIAN_POINT ( 'NONE',  ( -4.999999999999999112, -53.91666666666667140, 2.886751345948131764 ) ) ;
#62408=PLANE ( 'NONE',  #29394 ) ;
#62410=CARTESIAN_POINT ( 'NONE',  ( -6.972266317189433020E-16, -94.25000000000000000, -5.000000000000000000 ) ) ;
#62413=CARTESIAN_POINT ( 'NONE',  ( -5.000000000000000000, 13.00000000000000178, 0.000000000000000000 ) ) ;
#62418=AXIS2_PLACEMENT_3D ( 'NONE', #35124, #49272, #49582 ) ;
#62419=CARTESIAN_POINT ( 'NONE',  ( -2.499999999999996447, -5.833333333333336590, 4.330127018922195425 ) ) ;
#62422=VERTEX_POINT ( 'NONE', #12955 ) ;
#62430=CARTESIAN_POINT ( 'NONE',  ( -3.152548672688508926E-16, -35.81249999863440792, -5.148502694627439702 ) ) ;
#62431=DIRECTION ( 'NONE',  ( 0.000000000000000000, 0.000000000000000000, 1.000000000000000000 ) ) ;
#62438=CARTESIAN_POINT ( 'NONE',  ( 9.457646018065525792E-16, -85.31249999863439371, 5.148502694627439702 ) ) ;
#62440=ORIENTED_EDGE ( 'NONE', *, *, #22, .F. ) ;
#62442=( BOUNDED_CURVE ( )  B_SPLINE_CURVE ( 2, ( #6166, #45394, #54734, #706, #1359, #35750, #59565, #54413, #5843 ),
 .UNSPECIFIED., .F., .F. ) 
 B_SPLINE_CURVE_WITH_KNOTS ( ( 3, 2, 2, 2, 3 ),
 ( 0.4517857142857142905, 0.4523809523809523836, 0.4535714285714285698, 0.4547619047619047561, 0.4553571428571428492 ),
 .UNSPECIFIED. ) 
 CURVE ( )  GEOMETRIC_REPRESENTATION_ITEM ( )  RATIONAL_B_SPLINE_CURVE ( ( 0.9330127018922194093, 0.9330127018922194093, 1.000000000000000000, 0.8660254037844387076, 1.000000000000000000, 0.8660254037844387076, 1.000000000000000000, 0.9330127018922194093, 0.9330127018922194093 ) ) 
 REPRESENTATION_ITEM ( '' )  );
#62447=CARTESIAN_POINT ( 'NONE',  ( -4.458734124999998549, -11.47916666530107044, 2.574251347313722516 ) ) ;
#62450=CARTESIAN_POINT ( 'NONE',  ( -1.339745962155613812, -12.08034179853029322, -5.000000000000000000 ) ) ;
#62454=CARTESIAN_POINT ( 'NONE',  ( -2.229367062499996610, 24.60416666803225993, 3.861377020970582219 ) ) ;
#62456=CARTESIAN_POINT ( 'NONE',  ( -4.458734124999999437, -91.31249999863440792, 0.000000000000000000 ) ) ;
#62457=CARTESIAN_POINT ( 'NONE',  ( -2.500000000000000444, -31.16666666666666785, -4.330127018922193649 ) ) ;
#62458=CARTESIAN_POINT ( 'NONE',  ( 5.000000000000000000, -60.29166666393547303, -2.886751345948130876 ) ) ;
#62459=CARTESIAN_POINT ( 'NONE',  ( 2.229367062500001939, -6.979166665301073103, 3.861377020970579999 ) ) ;
#62461=AXIS2_PLACEMENT_3D ( 'NONE', #43929, #216, #9835 ) ;
#62465=CARTESIAN_POINT ( 'NONE',  ( -2.499999999999996447, -36.70833333060213732, 4.330127018922195425 ) ) ;
#62467=CARTESIAN_POINT ( 'NONE',  ( 9.457646018065525792E-16, 17.93750000136559208, 5.148502694627439702 ) ) ;
#62468=CARTESIAN_POINT ( 'NONE',  ( 1.339745962155612702, -7.294658198738518173, -5.000000000000000000 ) ) ;
#62470=CARTESIAN_POINT ( 'NONE',  ( -2.229367062500000163, -54.47916666530107221, -3.861377020970580443 ) ) ;
#62473=CARTESIAN_POINT ( 'NONE',  ( -5.000000000000000000, 11.00000000000000000, 0.000000000000000000 ) ) ;
#62475=CARTESIAN_POINT ( 'NONE',  ( 2.500000000000002220, -69.66666666666667140, 4.330127018922192761 ) ) ;
#62476=CARTESIAN_POINT ( 'NONE',  ( -4.458734124999998549, -49.22916666530106511, 2.574251347313722516 ) ) ;
#62477=CARTESIAN_POINT ( 'NONE',  ( 5.000000000000000000, -86.37499999726880162, -6.123233995736766282E-16 ) ) ;
#62479=CARTESIAN_POINT ( 'NONE',  ( -5.000000000000000000, -17.08333333333333215, -2.886751345948128211 ) ) ;
#62483=CARTESIAN_POINT ( 'NONE',  ( -2.229367062499996610, -92.39583333196773651, 3.861377020970582219 ) ) ;
#62485=CARTESIAN_POINT ( 'NONE',  ( 2.500000000000002220, -40.66666666666667140, 4.330127018922192761 ) ) ;
#62490=CARTESIAN_POINT ( 'NONE',  ( 2.229367062500001939, -94.97916666530106511, 3.861377020970579999 ) ) ;
#62491=CARTESIAN_POINT ( 'NONE',  ( -4.458734124999998549, 10.52083333469892779, 2.574251347313722516 ) ) ;
#62492=CARTESIAN_POINT ( 'NONE',  ( 5.000000000000000888, 9.541666669397852019, 2.886751345948126879 ) ) ;
#62499=CARTESIAN_POINT ( 'NONE',  ( -6.972266317189433020E-16, -40.12499999726880162, -5.000000000000000000 ) ) ;
#62500=CARTESIAN_POINT ( 'NONE',  ( 5.000000000000000000, -63.50000000000000000, -6.123233995736766282E-16 ) ) ;
#62503=CARTESIAN_POINT ( 'NONE',  ( -4.999999999999998224, -89.79166666393547303, 2.886751345948131764 ) ) ;
#62504=CARTESIAN_POINT ( 'NONE',  ( 4.458734125000001214, -20.14583333196774007, 2.574251347313718519 ) ) ;
#62514=ORIENTED_EDGE ( 'NONE', *, *, #13469, .F. ) ;
#62517=VERTEX_POINT ( 'NONE', #52201 ) ;
#62518=CARTESIAN_POINT ( 'NONE',  ( 4.458734125000001214, -66.14583333196772230, 2.574251347313718519 ) ) ;
#62523=CARTESIAN_POINT ( 'NONE',  ( 4.458734124999998549, 3.020833334698928674, -2.574251347313721627 ) ) ;
#62525=CARTESIAN_POINT ( 'NONE',  ( -6.972266317189433020E-16, -104.2500000000000000, -5.000000000000000000 ) ) ;
#62526=CARTESIAN_POINT ( 'NONE',  ( 9.457646018065525792E-16, 3.937500001365595192, 5.148502694627439702 ) ) ;
#62532=CARTESIAN_POINT ( 'NONE',  ( -4.458734124999997661, -75.22916666530106511, 2.574251347313722516 ) ) ;
#62533=CARTESIAN_POINT ( 'NONE',  ( -4.458734124999999437, 7.604166668032259935, -2.574251347313719407 ) ) ;
#62534=ADVANCED_FACE ( 'NONE', ( #17483 ), #23245, .T. ) ;
#62536=EDGE_CURVE ( 'NONE', #47780, #3809, #56627, .T. ) ;
#62537=CARTESIAN_POINT ( 'NONE',  ( -1.339745962155613812, -89.20534180126146850, -5.000000000000000000 ) ) ;
#62539=CARTESIAN_POINT ( 'NONE',  ( 4.458734124999998549, -57.97916666530107221, -2.574251347313721627 ) ) ;
#62540=CARTESIAN_POINT ( 'NONE',  ( 1.060575238724906964E-15, -18.62499999726881583, 5.773502691896257311 ) ) ;
#62546=CARTESIAN_POINT ( 'NONE',  ( 2.229367062500001939, -38.97916666530107221, 3.861377020970579999 ) ) ;
#62547=CARTESIAN_POINT ( 'NONE',  ( -2.229367062499996610, -26.39583333196774007, 3.861377020970582219 ) ) ;
#62550=CARTESIAN_POINT ( 'NONE',  ( 5.000000000000000000, 28.49999999999999645, -6.123233995736766282E-16 ) ) ;
#62552=ORIENTED_EDGE ( 'NONE', *, *, #6078, .F. ) ;
#62553=CARTESIAN_POINT ( 'NONE',  ( -4.458734124999998549, -31.22916666530107221, 2.574251347313722516 ) ) ;
#62554=CARTESIAN_POINT ( 'NONE',  ( -2.499999999999996447, -65.70833333060213022, 4.330127018922195425 ) ) ;
#62558=CARTESIAN_POINT ( 'NONE',  ( -4.458734124999999437, -26.31249999863440792, 0.000000000000000000 ) ) ;
#62559=ADVANCED_FACE ( 'NONE', ( #38966 ), #44107, .T. ) ;
#62560=CARTESIAN_POINT ( 'NONE',  ( 4.458734125000000326, -77.14583333196775072, 2.574251347313718519 ) ) ;
#62565=CARTESIAN_POINT ( 'NONE',  ( -2.500000000000000444, -15.16666666666666785, -4.330127018922193649 ) ) ;
#62570=CARTESIAN_POINT ( 'NONE',  ( -5.000000000000000000, 25.12500000273118417, 0.000000000000000000 ) ) ;
#62571=CARTESIAN_POINT ( 'NONE',  ( 1.339745962155615144, -81.58034179853029855, 4.999999999999999112 ) ) ;
#62574=CARTESIAN_POINT ( 'NONE',  ( 0.000000000000000000, -120.0000000000000000, 0.000000000000000000 ) ) ;
#62578=DIRECTION ( 'NONE',  ( -0.000000000000000000, 1.000000000000000000, -0.000000000000000000 ) ) ;
#62586=VERTEX_POINT ( 'NONE', #63437 ) ;
#62587=( BOUNDED_CURVE ( )  B_SPLINE_CURVE ( 2, ( #7185, #55112, #15559, #15874, #40626, #25517, #30976, #46413, #31614 ),
 .UNSPECIFIED., .F., .F. ) 
 B_SPLINE_CURVE_WITH_KNOTS ( ( 3, 2, 2, 2, 3 ),
 ( 0.1089285714285714302, 0.1095238095238095233, 0.1107142857142857095, 0.1119047619047619097, 0.1125000000000000028 ),
 .UNSPECIFIED. ) 
 CURVE ( )  GEOMETRIC_REPRESENTATION_ITEM ( )  RATIONAL_B_SPLINE_CURVE ( ( 0.9330127018922194093, 0.9330127018922194093, 1.000000000000000000, 0.8660254037844387076, 1.000000000000000000, 0.8660254037844387076, 1.000000000000000000, 0.9330127018922194093, 0.9330127018922194093 ) ) 
 REPRESENTATION_ITEM ( '' )  );
#62592=AXIS2_PLACEMENT_3D ( 'NONE', #62826, #17805, #57993 ) ;
#62597=CARTESIAN_POINT ( 'NONE',  ( 4.458734125000001214, -81.89583333196773651, 2.574251347313718519 ) ) ;
#62598=CARTESIAN_POINT ( 'NONE',  ( -4.458734124999999437, 18.60416666803225993, -2.574251347313719407 ) ) ;
#62599=CARTESIAN_POINT ( 'NONE',  ( -4.999999999999998224, -17.79166666393547658, 2.886751345948131764 ) ) ;
#62600=ORIENTED_EDGE ( 'NONE', *, *, #24677, .T. ) ;
#62604=CARTESIAN_POINT ( 'NONE',  ( 5.000000000000000000, -4.291666663935479242, -2.886751345948130876 ) ) ;
#62607=CARTESIAN_POINT ( 'NONE',  ( 4.458734124999998549, -57.72916666530107932, -2.574251347313721627 ) ) ;
#62609=CARTESIAN_POINT ( 'NONE',  ( -4.458734124999999437, 24.60416666803225993, -2.574251347313719407 ) ) ;
#62610=CARTESIAN_POINT ( 'NONE',  ( 2.500000000000002220, -42.66666666666667140, 4.330127018922192761 ) ) ;
#62611=CARTESIAN_POINT ( 'NONE',  ( -6.972266317189433020E-16, -16.12499999726881228, -5.000000000000000000 ) ) ;
#62613=CARTESIAN_POINT ( 'NONE',  ( 2.229367062499998831, -43.89583333196774362, -3.861377020970580887 ) ) ;
#62614=CARTESIAN_POINT ( 'NONE',  ( 5.000000000000000888, -5.458333330602148870, 2.886751345948126879 ) ) ;
#62618=CARTESIAN_POINT ( 'NONE',  ( 4.458734124999999437, -100.8124999986344079, -5.460374474430324690E-16 ) ) ;
#62619=CARTESIAN_POINT ( 'NONE',  ( -2.229367062499996610, -13.39583333196774007, 3.861377020970582219 ) ) ;
#62621=ORIENTED_EDGE ( 'NONE', *, *, #61924, .T. ) ;
#62623=CARTESIAN_POINT ( 'NONE',  ( -4.458734124999999437, -100.3124999986344079, 0.000000000000000000 ) ) ;
#62625=CARTESIAN_POINT ( 'NONE',  ( 9.457646018065525792E-16, -93.31249999863439371, 5.148502694627439702 ) ) ;
#62626=CARTESIAN_POINT ( 'NONE',  ( 1.060575238724906964E-15, -53.62499999726880873, 5.773502691896257311 ) ) ;
#62628=CARTESIAN_POINT ( 'NONE',  ( -1.339745962155610925, 19.33034180399266688, 5.000000000000000000 ) ) ;
#62630=CARTESIAN_POINT ( 'NONE',  ( -4.458734124999999437, -12.39583333196774184, -2.574251347313719407 ) ) ;
#62631=CARTESIAN_POINT ( 'NONE',  ( -3.152548672688508926E-16, 9.187500001365593860, -5.148502694627439702 ) ) ;
#62632=CARTESIAN_POINT ( 'NONE',  ( 4.458734124999998549, -56.97916666530107932, -2.574251347313721627 ) ) ;
#62633=CARTESIAN_POINT ( 'NONE',  ( -5.000000000000000000, -68.99999999999998579, 0.000000000000000000 ) ) ;
#62634=CARTESIAN_POINT ( 'NONE',  ( -1.339745962155669101, -36.79465819873851729, 4.999999999999966249 ) ) ;
#62637=EDGE_CURVE ( 'NONE', #4115, #44744, #29304, .T. ) ;
#62638=ORIENTED_EDGE ( 'NONE', *, *, #32539, .T. ) ;
#62642=EDGE_CURVE ( 'NONE', #41, #24503, #49271, .T. ) ;
#62645=CARTESIAN_POINT ( 'NONE',  ( 4.458734124999999437, -85.81249999863439371, -5.460374474430324690E-16 ) ) ;
#62646=CARTESIAN_POINT ( 'NONE',  ( 2.229367062499998831, 23.10416666803225993, -3.861377020970580887 ) ) ;
#62649=CARTESIAN_POINT ( 'NONE',  ( -5.000000000000000000, 6.916666666666664298, -2.886751345948128211 ) ) ;
#62652=CARTESIAN_POINT ( 'NONE',  ( -2.500000000000000444, -71.16666666666667140, -4.330127018922193649 ) ) ;
#62654=VERTEX_POINT ( 'NONE', #10655 ) ;
#62667=CARTESIAN_POINT ( 'NONE',  ( -2.229367062499996610, -55.39583333196773651, 3.861377020970582219 ) ) ;
#62669=CARTESIAN_POINT ( 'NONE',  ( -6.972266317189433020E-16, -106.1249999972688016, -5.000000000000000000 ) ) ;
#62674=ORIENTED_EDGE ( 'NONE', *, *, #9608, .F. ) ;
#62677=CARTESIAN_POINT ( 'NONE',  ( -4.458734124999998549, -99.47916666530105090, 2.574251347313722516 ) ) ;
#62679=ORIENTED_EDGE ( 'NONE', *, *, #7242, .F. ) ;
#62682=CARTESIAN_POINT ( 'NONE',  ( 2.500000000000002220, -83.66666666666667140, 4.330127018922192761 ) ) ;
#62684=CARTESIAN_POINT ( 'NONE',  ( -2.229367062499996610, -10.14583333196773829, 3.861377020970582219 ) ) ;
#62685=CARTESIAN_POINT ( 'NONE',  ( 2.229367062499998831, -98.89583333196773651, -3.861377020970580887 ) ) ;
#62687=CARTESIAN_POINT ( 'NONE',  ( 2.229367062500001939, -30.22916666530107221, 3.861377020970579999 ) ) ;
#62693=CARTESIAN_POINT ( 'NONE',  ( 2.229367062499998831, 7.104166668032259935, -3.861377020970580887 ) ) ;
#62695=CARTESIAN_POINT ( 'NONE',  ( -5.000000000000000000, 1.916666666666667407, -2.886751345948128211 ) ) ;
#62696=CARTESIAN_POINT ( 'NONE',  ( -6.972266317189433020E-16, 2.750000000000000000, -5.000000000000000000 ) ) ;
#62697=CARTESIAN_POINT ( 'NONE',  ( -4.999999999999999112, -89.91666666666665719, 2.886751345948131764 ) ) ;
#62698=CARTESIAN_POINT ( 'NONE',  ( 2.229367062499998831, -27.64583333196774007, -3.861377020970580887 ) ) ;
#62699=CARTESIAN_POINT ( 'NONE',  ( -1.339745962155610925, -76.66965819600731891, 5.000000000000000000 ) ) ;
#62700=CARTESIAN_POINT ( 'NONE',  ( 4.458734124999998549, -75.97916666530106511, -2.574251347313721627 ) ) ;
#62702=CARTESIAN_POINT ( 'NONE',  ( 0.000000000000000000, -120.0000000000000000, 5.000000000000000000 ) ) ;
#62704=CARTESIAN_POINT ( 'NONE',  ( -4.458734124999999437, 0.6041666680322611560, -2.574251347313719407 ) ) ;
#62705=CARTESIAN_POINT ( 'NONE',  ( -2.229367062500000163, 26.27083333469892779, -3.861377020970580443 ) ) ;
#62706=CARTESIAN_POINT ( 'NONE',  ( 4.458734125000000326, -40.14583333196773651, 2.574251347313718519 ) ) ;
#62711=CARTESIAN_POINT ( 'NONE',  ( -2.229367062499996610, -68.14583333196773651, 3.861377020970582219 ) ) ;
#62712=CARTESIAN_POINT ( 'NONE',  ( -3.535250795749689387E-16, -100.1249999972688158, -5.773502691896257311 ) ) ;
#62715=CARTESIAN_POINT ( 'NONE',  ( 1.975475456537005874E-15, 9.375000002731185944, 5.000000000000000000 ) ) ;
#62716=CARTESIAN_POINT ( 'NONE',  ( -4.458734124999999437, -106.6458333319677365, -2.574251347313719407 ) ) ;
#62718=CARTESIAN_POINT ( 'NONE',  ( -5.000000000000000000, -54.08333333333332860, -2.886751345948128211 ) ) ;
#62722=LINE ( 'NONE', #23159, #19127 ) ;
#62724=CARTESIAN_POINT ( 'NONE',  ( -6.972266317189433020E-16, -97.12499999726880162, -5.000000000000000000 ) ) ;
#62734=CARTESIAN_POINT ( 'NONE',  ( 2.500000000000002220, -45.54166666393547303, 4.330127018922192761 ) ) ;
#62740=CARTESIAN_POINT ( 'NONE',  ( -4.458734124999999437, -38.56249999863440081, 0.000000000000000000 ) ) ;
#62741=CARTESIAN_POINT ( 'NONE',  ( -6.972266317189433020E-16, -101.2499999999999858, -5.000000000000000000 ) ) ;
#62748=CARTESIAN_POINT ( 'NONE',  ( 1.339745962155612702, -54.29465819873851729, -5.000000000000000000 ) ) ;
#62750=CARTESIAN_POINT ( 'NONE',  ( 4.458734124999998549, -82.97916666530107932, -2.574251347313721627 ) ) ;
#62751=CARTESIAN_POINT ( 'NONE',  ( -6.972266317189433020E-16, -34.12499999726881583, -5.000000000000000000 ) ) ;
#62752=ORIENTED_EDGE ( 'NONE', *, *, #47992, .T. ) ;
#62753=CARTESIAN_POINT ( 'NONE',  ( -2.500000000000000444, -95.04166666393547303, -4.330127018922193649 ) ) ;
#62757=CARTESIAN_POINT ( 'NONE',  ( 2.499999999999998668, -78.33333333333332860, -4.330127018922193649 ) ) ;
#62758=CARTESIAN_POINT ( 'NONE',  ( 4.458734124999998549, -10.97916666530107044, -2.574251347313721627 ) ) ;
#62761=CARTESIAN_POINT ( 'NONE',  ( 2.500000000000002220, -77.54166666393547303, 4.330127018922192761 ) ) ;
#62763=CARTESIAN_POINT ( 'NONE',  ( 2.229367062500001939, 23.77083333469892779, 3.861377020970579999 ) ) ;
#62764=VERTEX_POINT ( 'NONE', #20647 ) ;
#62765=CARTESIAN_POINT ( 'NONE',  ( 9.457646018065525792E-16, -91.06249999863439371, 5.148502694627439702 ) ) ;
#62766=CARTESIAN_POINT ( 'NONE',  ( 5.000000000000000000, -47.41666666666666430, -2.886751345948130876 ) ) ;
#62768=CARTESIAN_POINT ( 'NONE',  ( 4.458734124999999437, -7.812499998634405252, -5.460374474430324690E-16 ) ) ;
#62770=DIRECTION ( 'NONE',  ( -0.000000000000000000, 1.000000000000000000, -0.000000000000000000 ) ) ;
#62772=CARTESIAN_POINT ( 'NONE',  ( 2.500000000000002220, -37.54166666393548013, 4.330127018922192761 ) ) ;
#62774=CARTESIAN_POINT ( 'NONE',  ( 2.229367062500001939, 18.02083333469892779, 3.861377020970579999 ) ) ;
#62777=CARTESIAN_POINT ( 'NONE',  ( 4.458734125000001214, -58.89583333196773651, 2.574251347313718519 ) ) ;
#62781=CARTESIAN_POINT ( 'NONE',  ( 5.000000000000000000, 11.50000000000000000, -6.123233995736766282E-16 ) ) ;
#62784=CARTESIAN_POINT ( 'NONE',  ( -4.458734124999999437, -47.31249999863440792, 0.000000000000000000 ) ) ;
#62785=CARTESIAN_POINT ( 'NONE',  ( 1.060575238724906964E-15, -85.62499999726880162, 5.773502691896257311 ) ) ;
#62787=DIRECTION ( 'NONE',  ( 0.000000000000000000, 0.000000000000000000, 1.000000000000000000 ) ) ;
#62789=CARTESIAN_POINT ( 'NONE',  ( 4.458734124999999437, -90.06249999863440792, -5.460374474430324690E-16 ) ) ;
#62791=CARTESIAN_POINT ( 'NONE',  ( 5.000000000000000000, -38.41666666666667140, -2.886751345948129988 ) ) ;
#62796=CARTESIAN_POINT ( 'NONE',  ( 4.458734125000001214, -96.89583333196772230, 2.574251347313718519 ) ) ;
#62797=CARTESIAN_POINT ( 'NONE',  ( 9.457646018065525792E-16, 5.687500001365592972, 5.148502694627439702 ) ) ;
#62798=CARTESIAN_POINT ( 'NONE',  ( 5.000000000000000000, 12.62500000273118417, -6.123233995736766282E-16 ) ) ;
#62807=CARTESIAN_POINT ( 'NONE',  ( 1.339745962155670655, -19.29465819873852084, -4.999999999999966249 ) ) ;
#62811=CARTESIAN_POINT ( 'NONE',  ( 4.458734125000001214, -18.14583333196773651, 2.574251347313718519 ) ) ;
#62823=EDGE_LOOP ( 'NONE', ( #1064, #40629, #34206, #20238 ) ) ;
#62824=CARTESIAN_POINT ( 'NONE',  ( 4.458734124999999437, -66.06249999863440792, -5.460374474430324690E-16 ) ) ;
#62825=CARTESIAN_POINT ( 'NONE',  ( -2.500000000000000444, 28.83333333333333215, -4.330127018922193649 ) ) ;
#62826=CARTESIAN_POINT ( 'NONE',  ( 0.000000000000000000, -120.0000000000000000, 0.000000000000000000 ) ) ;
#62830=CARTESIAN_POINT ( 'NONE',  ( -4.458734124999999437, 3.437500001365594748, 0.000000000000000000 ) ) ;
#62832=EDGE_CURVE ( 'NONE', #12555, #61001, #62442, .T. ) ;
#62840=CARTESIAN_POINT ( 'NONE',  ( 4.458734125000000326, -75.89583333196775072, 2.574251347313718519 ) ) ;
#62841=CARTESIAN_POINT ( 'NONE',  ( 2.500000000000002220, 14.45833333606451809, 4.330127018922192761 ) ) ;
#62842=CARTESIAN_POINT ( 'NONE',  ( 4.458734124999999437, 9.187500001365592084, -5.460374474430324690E-16 ) ) ;
#62845=CARTESIAN_POINT ( 'NONE',  ( -3.152548672688508926E-16, -58.81249999863440081, -5.148502694627439702 ) ) ;
#62846=CARTESIAN_POINT ( 'NONE',  ( 5.000000000000000000, -21.29166666393548013, -2.886751345948129988 ) ) ;
#62848=DIRECTION ( 'NONE',  ( 0.000000000000000000, 0.000000000000000000, 1.000000000000000000 ) ) ;
#62850=CARTESIAN_POINT ( 'NONE',  ( -6.972266317189433020E-16, -74.25000000000000000, -5.000000000000000000 ) ) ;
#62851=LINE ( 'NONE', #43210, #18189 ) ;
#62852=CARTESIAN_POINT ( 'NONE',  ( -4.458734124999999437, -40.39583333196773651, -2.574251347313719407 ) ) ;
#62853=CARTESIAN_POINT ( 'NONE',  ( -4.458734124999999437, -27.56249999863440081, 0.000000000000000000 ) ) ;
#62855=CARTESIAN_POINT ( 'NONE',  ( 2.499999999999998668, 27.66666666666666430, -4.330127018922193649 ) ) ;
#62858=CARTESIAN_POINT ( 'NONE',  ( -3.152548672688508926E-16, -105.8124999986344079, -5.148502694627439702 ) ) ;
#62859=CARTESIAN_POINT ( 'NONE',  ( 4.458734124999998549, -31.72916666530107577, -2.574251347313721627 ) ) ;
#62860=CARTESIAN_POINT ( 'NONE',  ( -3.535250795749689387E-16, -66.12499999726881583, -5.773502691896257311 ) ) ;
#62864=CARTESIAN_POINT ( 'NONE',  ( -4.458734124999999437, -74.56249999863440792, 0.000000000000000000 ) ) ;
#62868=CARTESIAN_POINT ( 'NONE',  ( 1.975475456537005874E-15, -5.624999997268812280, 5.000000000000000000 ) ) ;
#62869=CARTESIAN_POINT ( 'NONE',  ( 2.499999999999998668, -20.33333333333333570, -4.330127018922193649 ) ) ;
#62874=CARTESIAN_POINT ( 'NONE',  ( 2.500000000000002220, 26.45833333606451632, 4.330127018922192761 ) ) ;
#62877=DIRECTION ( 'NONE',  ( 0.000000000000000000, 0.000000000000000000, 1.000000000000000000 ) ) ;
#62879=CARTESIAN_POINT ( 'NONE',  ( 1.339745962155613146, 28.29465819873852084, 5.000000000000000888 ) ) ;
#62880=CARTESIAN_POINT ( 'NONE',  ( -6.972266317189433020E-16, -41.12499999726880162, -5.000000000000000000 ) ) ;
#62884=CARTESIAN_POINT ( 'NONE',  ( -4.999999999999998224, -71.79166666393547303, 2.886751345948131764 ) ) ;
#62887=EDGE_CURVE ( 'NONE', #11557, #34481, #20915, .T. ) ;
#62889=VERTEX_POINT ( 'NONE', #36846 ) ;
#62892=CARTESIAN_POINT ( 'NONE',  ( 1.975475456537005874E-15, 18.37500000273118062, 5.000000000000000000 ) ) ;
#62895=ORIENTED_EDGE ( 'NONE', *, *, #10820, .F. ) ;
#62896=CYLINDRICAL_SURFACE ( 'NONE', #42654, 5.000000000000000000 ) ;
#62900=VERTEX_POINT ( 'NONE', #47749 ) ;
#62901=( BOUNDED_CURVE ( )  B_SPLINE_CURVE ( 2, ( #53785, #29323, #9718, #49594, #29967, #30610, #5535, #60220, #1055 ),
 .UNSPECIFIED., .F., .F. ) 
 B_SPLINE_CURVE_WITH_KNOTS ( ( 3, 2, 2, 2, 3 ),
 ( 0.3517857142857143127, 0.3523809523809524058, 0.3535714285714285920, 0.3547619047619047783, 0.3553571428571428714 ),
 .UNSPECIFIED. ) 
 CURVE ( )  GEOMETRIC_REPRESENTATION_ITEM ( )  RATIONAL_B_SPLINE_CURVE ( ( 0.9330127018922194093, 0.9330127018922225179, 1.000000000000000000, 0.8660254037844387076, 1.000000000000000000, 0.8660254037844387076, 1.000000000000000000, 0.9330127018922194093, 0.9330127018922194093 ) ) 
 REPRESENTATION_ITEM ( '' )  );
#62902=CARTESIAN_POINT ( 'NONE',  ( 2.229367062500001939, -83.97916666530106511, 3.861377020970579999 ) ) ;
#62903=EDGE_CURVE ( 'NONE', #3585, #55695, #8212, .T. ) ;
#62904=CARTESIAN_POINT ( 'NONE',  ( -2.229367062499996610, 16.85416666803225993, 3.861377020970582219 ) ) ;
#62905=CARTESIAN_POINT ( 'NONE',  ( 1.339745962155615144, -12.58034179853029144, 4.999999999999999112 ) ) ;
#62911=CARTESIAN_POINT ( 'NONE',  ( 2.499999999999998668, -88.33333333333332860, -4.330127018922193649 ) ) ;
#62912=DIRECTION ( 'NONE',  ( -0.000000000000000000, 1.000000000000000000, -0.000000000000000000 ) ) ;
#62913=CARTESIAN_POINT ( 'NONE',  ( 5.000000000000000888, -13.45833333060214976, 2.886751345948126879 ) ) ;
#62914=CARTESIAN_POINT ( 'NONE',  ( -3.152548672688508926E-16, -57.56249999863440792, -5.148502694627439702 ) ) ;
#62915=CARTESIAN_POINT ( 'NONE',  ( 2.500000000000002220, 21.33333333333333215, 4.330127018922192761 ) ) ;
#62916=CARTESIAN_POINT ( 'NONE',  ( 2.229367062500001939, 23.02083333469892423, 3.861377020970579999 ) ) ;
#62917=CARTESIAN_POINT ( 'NONE',  ( 1.975475456537005874E-15, -42.75000000000000000, 5.000000000000000000 ) ) ;
#62918=DIRECTION ( 'NONE',  ( -0.000000000000000000, 1.000000000000000000, -0.000000000000000000 ) ) ;
#62919=CARTESIAN_POINT ( 'NONE',  ( -4.458734124999999437, -41.64583333196773651, -2.574251347313719407 ) ) ;
#62920=CARTESIAN_POINT ( 'NONE',  ( 2.500000000000002220, -1.541666663935480130, 4.330127018922192761 ) ) ;
#62923=CARTESIAN_POINT ( 'NONE',  ( 4.458734125000000326, -107.8958333319677365, 2.574251347313718519 ) ) ;
#62924=CARTESIAN_POINT ( 'NONE',  ( 2.229367062499998831, -12.89583333196774007, -3.861377020970580887 ) ) ;
#62925=VERTEX_POINT ( 'NONE', #56476 ) ;
#62927=CARTESIAN_POINT ( 'NONE',  ( -4.458734124999999437, -99.39583333196772230, -2.574251347313719407 ) ) ;
#62929=CARTESIAN_POINT ( 'NONE',  ( -2.229367062499996610, -92.39583333196773651, 3.861377020970582219 ) ) ;
#62931=CARTESIAN_POINT ( 'NONE',  ( 5.000000000000000000, -51.29166666393547303, -2.886751345948129988 ) ) ;
#62935=CARTESIAN_POINT ( 'NONE',  ( 2.229367062500001939, -13.97916666530107221, 3.861377020970579999 ) ) ;
#62936=CARTESIAN_POINT ( 'NONE',  ( -4.458734124999999437, 10.43750000136559386, 0.000000000000000000 ) ) ;
#62937=CARTESIAN_POINT ( 'NONE',  ( -4.458734124999999437, -59.64583333196775072, -2.574251347313719407 ) ) ;
#62941=CARTESIAN_POINT ( 'NONE',  ( 0.000000000000000000, -120.0000000000000000, 0.000000000000000000 ) ) ;
#62944=CARTESIAN_POINT ( 'NONE',  ( -2.499999999999996447, -37.83333333333332860, 4.330127018922195425 ) ) ;
#62945=CARTESIAN_POINT ( 'NONE',  ( 1.339745962155615144, -66.70534180126148271, 4.999999999999999112 ) ) ;
#62946=CARTESIAN_POINT ( 'NONE',  ( -1.339745962155610925, -24.79465819873852439, 5.000000000000000000 ) ) ;
#62947=CARTESIAN_POINT ( 'NONE',  ( -2.229367062499996610, -84.14583333196773651, 3.861377020970582219 ) ) ;
#62948=CARTESIAN_POINT ( 'NONE',  ( 4.458734124999999437, 19.93750000136559208, -5.460374474430324690E-16 ) ) ;
#62953=CARTESIAN_POINT ( 'NONE',  ( 5.000000000000000000, -68.49999999999998579, -6.123233995736766282E-16 ) ) ;
#62954=( BOUNDED_CURVE ( )  B_SPLINE_CURVE ( 2, ( #52542, #10038, #34161, #9716, #58622, #29652, #62825, #38984, #58928 ),
 .UNSPECIFIED., .F., .F. ) 
 B_SPLINE_CURVE_WITH_KNOTS ( ( 3, 2, 2, 2, 3 ),
 ( 0.005357142857142858060, 0.005952380952380952051, 0.007142857142857142634, 0.008333333333333333218, 0.008928571428571429811 ),
 .UNSPECIFIED. ) 
 CURVE ( )  GEOMETRIC_REPRESENTATION_ITEM ( )  RATIONAL_B_SPLINE_CURVE ( ( 0.9330127018922192983, 0.9330127018922194093, 1.000000000000000000, 0.8660254037844387076, 1.000000000000000000, 0.8660254037844387076, 1.000000000000000000, 0.9330127018922191873, 0.9330127018922192983 ) ) 
 REPRESENTATION_ITEM ( '' )  );
#62957=CARTESIAN_POINT ( 'NONE',  ( -6.972266317189433020E-16, -102.2499999999999858, -5.000000000000000000 ) ) ;
#62959=( BOUNDED_CURVE ( )  B_SPLINE_CURVE ( 2, ( #28460, #24906, #29381, #33605, #57747, #53225, #39049, #49015, #43865 ),
 .UNSPECIFIED., .F., .F. ) 
 B_SPLINE_CURVE_WITH_KNOTS ( ( 3, 2, 2, 2, 3 ),
 ( 0.1303571428571428659, 0.1309523809523809590, 0.1321428571428571452, 0.1333333333333333315, 0.1339285714285714246 ),
 .UNSPECIFIED. ) 
 CURVE ( )  GEOMETRIC_REPRESENTATION_ITEM ( )  RATIONAL_B_SPLINE_CURVE ( ( 0.9330127018922194093, 0.9330127018922194093, 1.000000000000000000, 0.8660254037844387076, 1.000000000000000000, 0.8660254037844387076, 1.000000000000000000, 0.9330127018922194093, 0.9330127018922194093 ) ) 
 REPRESENTATION_ITEM ( '' )  );
#62960=CARTESIAN_POINT ( 'NONE',  ( -2.500000000000000444, -90.16666666666665719, -4.330127018922193649 ) ) ;
#62964=ADVANCED_FACE ( 'NONE', ( #12711 ), #7580, .T. ) ;
#62966=ADVANCED_FACE ( 'NONE', ( #42610 ), #61297, .T. ) ;
#62968=VERTEX_POINT ( 'NONE', #22052 ) ;
#62971=VERTEX_POINT ( 'NONE', #18487 ) ;
#62975=CARTESIAN_POINT ( 'NONE',  ( 4.458734124999999437, -59.06249999863440081, -5.460374474430324690E-16 ) ) ;
#62976=EDGE_CURVE ( 'NONE', #40791, #56173, #62248, .T. ) ;
#62978=CARTESIAN_POINT ( 'NONE',  ( -1.339745962155613812, 9.919658201469706782, -5.000000000000000000 ) ) ;
#62981=EDGE_CURVE ( 'NONE', #24993, #49029, #28131, .T. ) ;
#62985=VERTEX_POINT ( 'NONE', #18167 ) ;
#62989=CARTESIAN_POINT ( 'NONE',  ( 2.229367062499998831, -103.8958333319677365, -3.861377020970580887 ) ) ;
#62992=ORIENTED_EDGE ( 'NONE', *, *, #39698, .F. ) ;
#62993=EDGE_CURVE ( 'NONE', #35341, #57091, #5313, .T. ) ;
#62996=CARTESIAN_POINT ( 'NONE',  ( 4.458734125000000326, -39.89583333196772941, 2.574251347313718519 ) ) ;
#62997=EDGE_CURVE ( 'NONE', #56652, #55713, #12648, .T. ) ;
#62998=EDGE_CURVE ( 'NONE', #57534, #7022, #3274, .T. ) ;
#63000=CARTESIAN_POINT ( 'NONE',  ( 9.457646018065525792E-16, -15.06249999863440259, 5.148502694627439702 ) ) ;
#63001=CARTESIAN_POINT ( 'NONE',  ( 2.229367062499998831, -99.89583333196773651, -3.861377020970580887 ) ) ;
#63003=CARTESIAN_POINT ( 'NONE',  ( -4.458734124999998549, -30.47916666530107221, 2.574251347313722516 ) ) ;
#63004=CARTESIAN_POINT ( 'NONE',  ( -2.499999999999996447, 12.16666666666666607, 4.330127018922195425 ) ) ;
#63007=CARTESIAN_POINT ( 'NONE',  ( 5.000000000000000000, -21.37499999726881228, -6.123233995736766282E-16 ) ) ;
#63011=CARTESIAN_POINT ( 'NONE',  ( -4.458734124999997661, 7.520833334698926009, 2.574251347313722516 ) ) ;
#63012=VERTEX_POINT ( 'NONE', #33900 ) ;
#63015=CARTESIAN_POINT ( 'NONE',  ( -3.535250795749689387E-16, -97.25000000000000000, -5.773502691896257311 ) ) ;
#63016=CARTESIAN_POINT ( 'NONE',  ( 9.457646018065525792E-16, -32.06249999863440792, 5.148502694627439702 ) ) ;
#63017=CARTESIAN_POINT ( 'NONE',  ( -2.499999999999996447, 7.291666669397852019, 4.330127018922195425 ) ) ;
#63018=CARTESIAN_POINT ( 'NONE',  ( -4.458734124999999437, -73.56249999863439371, 0.000000000000000000 ) ) ;
#63022=CARTESIAN_POINT ( 'NONE',  ( 4.458734124999998549, 3.270833334698929118, -2.574251347313721627 ) ) ;
#63023=CARTESIAN_POINT ( 'NONE',  ( 4.458734124999998549, 27.02083333469892423, -2.574251347313721627 ) ) ;
#63024=CARTESIAN_POINT ( 'NONE',  ( -4.458734124999999437, -40.64583333196773651, -2.574251347313719407 ) ) ;
#63029=CARTESIAN_POINT ( 'NONE',  ( 4.458734124999999437, -69.81249999863439371, -5.460374474430324690E-16 ) ) ;
#63030=CARTESIAN_POINT ( 'NONE',  ( 5.000000000000000000, -104.2916666639354588, -2.886751345948129988 ) ) ;
#63031=CARTESIAN_POINT ( 'NONE',  ( 2.499999999999998668, -41.33333333333333570, -4.330127018922193649 ) ) ;
#63032=CARTESIAN_POINT ( 'NONE',  ( -2.499999999999996447, -63.83333333333332860, 4.330127018922195425 ) ) ;
#63033=CARTESIAN_POINT ( 'NONE',  ( 2.229367062499998831, -107.8958333319677365, -3.861377020970580887 ) ) ;
#63035=CARTESIAN_POINT ( 'NONE',  ( 5.000000000000000888, -51.58333333333332149, 2.886751345948126879 ) ) ;
#63036=CARTESIAN_POINT ( 'NONE',  ( -2.499999999999996447, -65.83333333333332860, 4.330127018922195425 ) ) ;
#63040=CARTESIAN_POINT ( 'NONE',  ( 1.339745962155612702, -27.16965819600733312, -5.000000000000000000 ) ) ;
#63054=CARTESIAN_POINT ( 'NONE',  ( 4.458734124999998549, -38.97916666530107221, -2.574251347313721627 ) ) ;
#63061=LINE ( 'NONE', #38292, #19282 ) ;
#63063=CARTESIAN_POINT ( 'NONE',  ( -3.152548672688508926E-16, -88.81249999863439371, -5.148502694627439702 ) ) ;
#63064=CARTESIAN_POINT ( 'NONE',  ( 5.000000000000000000, -34.37499999726881583, -6.123233995736766282E-16 ) ) ;
#63066=EDGE_CURVE ( 'NONE', #25665, #10009, #11881, .T. ) ;
#63067=CARTESIAN_POINT ( 'NONE',  ( -2.499999999999996447, -46.83333333333333570, 4.330127018922195425 ) ) ;
#63069=CARTESIAN_POINT ( 'NONE',  ( 2.500000000000002220, -43.66666666666665719, 4.330127018922192761 ) ) ;
#63071=EDGE_LOOP ( 'NONE', ( #7214, #46158, #44843, #2673 ) ) ;
#63074=CARTESIAN_POINT ( 'NONE',  ( 2.229367062500001939, -13.22916666530107221, 3.861377020970579999 ) ) ;
#63076=CARTESIAN_POINT ( 'NONE',  ( 5.000000000000000000, -105.2916666639354730, -2.886751345948130876 ) ) ;
#63080=CARTESIAN_POINT ( 'NONE',  ( -4.458734124999999437, 19.43750000136559208, 0.000000000000000000 ) ) ;
#63081=VERTEX_POINT ( 'NONE', #4624 ) ;
#63082=CARTESIAN_POINT ( 'NONE',  ( 4.458734125000000326, -91.89583333196773651, 2.574251347313718519 ) ) ;
#63085=CARTESIAN_POINT ( 'NONE',  ( -4.458734124999999437, -16.31249999863440436, 0.000000000000000000 ) ) ;
#63086=CARTESIAN_POINT ( 'NONE',  ( -6.972266317189433020E-16, -39.12499999726880162, -5.000000000000000000 ) ) ;
#63087=CARTESIAN_POINT ( 'NONE',  ( -5.000000000000000000, -73.00000000000000000, 0.000000000000000000 ) ) ;
#63089=CARTESIAN_POINT ( 'NONE',  ( 0.000000000000000000, -120.0000000000000000, 5.000000000000000000 ) ) ;
#63090=CARTESIAN_POINT ( 'NONE',  ( -5.000000000000000000, -41.95833333060214443, -2.886751345948128211 ) ) ;
#63092=CARTESIAN_POINT ( 'NONE',  ( 4.458734124999998549, 21.27083333469892779, -2.574251347313721627 ) ) ;
#63095=CARTESIAN_POINT ( 'NONE',  ( 4.458734124999998549, -62.72916666530106511, -2.574251347313721627 ) ) ;
#63098=CARTESIAN_POINT ( 'NONE',  ( 1.060575238724906964E-15, 7.249999999999999112, 5.773502691896257311 ) ) ;
#63100=CARTESIAN_POINT ( 'NONE',  ( -5.000000000000000000, -59.87499999726880873, 0.000000000000000000 ) ) ;
#63101=CARTESIAN_POINT ( 'NONE',  ( 4.458734125000001214, -53.89583333196773651, 2.574251347313718519 ) ) ;
#63102=CARTESIAN_POINT ( 'NONE',  ( 5.000000000000000000, -84.29166666393547303, -2.886751345948129988 ) ) ;
#63105=( BOUNDED_CURVE ( )  B_SPLINE_CURVE ( 2, ( #43395, #63040, #18948, #38566, #14439, #58195, #14124, #33750, #53368 ),
 .UNSPECIFIED., .F., .F. ) 
 B_SPLINE_CURVE_WITH_KNOTS ( ( 3, 2, 2, 2, 3 ),
 ( 0.4017857142857143016, 0.4023809523809523947, 0.4035714285714285809, 0.4047619047619047672, 0.4053571428571428603 ),
 .UNSPECIFIED. ) 
 CURVE ( )  GEOMETRIC_REPRESENTATION_ITEM ( )  RATIONAL_B_SPLINE_CURVE ( ( 0.9330127018922194093, 0.9330127018922194093, 1.000000000000000000, 0.8660254037844387076, 1.000000000000000000, 0.8660254037844387076, 1.000000000000000000, 0.9330127018922194093, 0.9330127018922194093 ) ) 
 REPRESENTATION_ITEM ( '' )  );
#63106=CARTESIAN_POINT ( 'NONE',  ( -5.000000000000000000, -92.08333333333334281, -2.886751345948128211 ) ) ;
#63107=CARTESIAN_POINT ( 'NONE',  ( -3.152548672688508926E-16, -92.81249999863440792, -5.148502694627439702 ) ) ;
#63109=CARTESIAN_POINT ( 'NONE',  ( -5.000000000000000000, -37.08333333333332860, -2.886751345948128211 ) ) ;
#63110=DIRECTION ( 'NONE',  ( -0.000000000000000000, 1.000000000000000000, -0.000000000000000000 ) ) ;
#63113=CARTESIAN_POINT ( 'NONE',  ( 2.229367062500001939, -102.9791666653010651, 3.861377020970579999 ) ) ;
#63114=CARTESIAN_POINT ( 'NONE',  ( 4.458734124999999437, 8.937500001365592084, -5.460374474430324690E-16 ) ) ;
#63115=CARTESIAN_POINT ( 'NONE',  ( -5.000000000000000000, 13.12500000273118417, 0.000000000000000000 ) ) ;
#63116=CARTESIAN_POINT ( 'NONE',  ( -6.972266317189433020E-16, -44.12499999726880162, -5.000000000000000000 ) ) ;
#63120=FACE_OUTER_BOUND ( 'NONE', #7861, .T. ) ;
#63123=CARTESIAN_POINT ( 'NONE',  ( 0.000000000000000000, -120.0000000000000000, 5.000000000000000000 ) ) ;
#63124=CARTESIAN_POINT ( 'NONE',  ( 0.000000000000000000, -120.0000000000000000, 0.000000000000000000 ) ) ;
#63127=CARTESIAN_POINT ( 'NONE',  ( 2.500000000000002220, 6.458333336064519870, 4.330127018922192761 ) ) ;
#63128=CARTESIAN_POINT ( 'NONE',  ( 4.458734124999999437, -25.06249999863440792, -5.460374474430324690E-16 ) ) ;
#63136=ORIENTED_EDGE ( 'NONE', *, *, #63400, .F. ) ;
#63138=ORIENTED_EDGE ( 'NONE', *, *, #21654, .T. ) ;
#63139=CARTESIAN_POINT ( 'NONE',  ( -3.152548672688508926E-16, -69.81249999863439371, -5.148502694627439702 ) ) ;
#63144=CARTESIAN_POINT ( 'NONE',  ( -3.152548672688508926E-16, 0.1875000013655953035, -5.148502694627439702 ) ) ;
#63145=VERTEX_POINT ( 'NONE', #6151 ) ;
#63147=CYLINDRICAL_SURFACE ( 'NONE', #6023, 5.000000000000000000 ) ;
#63150=CARTESIAN_POINT ( 'NONE',  ( 5.000000000000000000, -92.37499999726880162, -6.123233995736766282E-16 ) ) ;
#63153=ORIENTED_EDGE ( 'NONE', *, *, #40615, .T. ) ;
#63154=CARTESIAN_POINT ( 'NONE',  ( -4.458734124999997661, -78.22916666530106511, 2.574251347313722516 ) ) ;
#63156=CARTESIAN_POINT ( 'NONE',  ( -4.458734124999999437, -0.3124999986344051406, 0.000000000000000000 ) ) ;
#63158=CARTESIAN_POINT ( 'NONE',  ( 2.229367062499998831, -67.89583333196773651, -3.861377020970580887 ) ) ;
#63159=CARTESIAN_POINT ( 'NONE',  ( 2.499999999999998668, -20.20833333060214798, -4.330127018922193649 ) ) ;
#63160=CARTESIAN_POINT ( 'NONE',  ( 5.000000000000000000, -96.29166666393547303, -2.886751345948130876 ) ) ;
#63161=CARTESIAN_POINT ( 'NONE',  ( 0.000000000000000000, -120.0000000000000000, 0.000000000000000000 ) ) ;
#63162=CARTESIAN_POINT ( 'NONE',  ( -4.999999999999998224, -64.79166666393547303, 2.886751345948131764 ) ) ;
#63163=CARTESIAN_POINT ( 'NONE',  ( 8.660254037844342889, 45.00000000000000000, 0.000000000000000000 ) ) ;
#63164=CARTESIAN_POINT ( 'NONE',  ( -2.229367062500000163, -41.47916666530107932, -3.861377020970580443 ) ) ;
#63165=CARTESIAN_POINT ( 'NONE',  ( -4.458734124999999437, -28.64583333196774007, -2.574251347313719407 ) ) ;
#63168=CARTESIAN_POINT ( 'NONE',  ( -5.000000000000000000, 26.91666666666666075, -2.886751345948128211 ) ) ;
#63170=CARTESIAN_POINT ( 'NONE',  ( 4.458734124999998549, -106.9791666653010509, -2.574251347313721627 ) ) ;
#63172=CARTESIAN_POINT ( 'NONE',  ( -4.458734124999999437, -36.31249999863440792, 0.000000000000000000 ) ) ;
#63173=CARTESIAN_POINT ( 'NONE',  ( 5.000000000000000000, -68.37499999726881583, -6.123233995736766282E-16 ) ) ;
#63176=CARTESIAN_POINT ( 'NONE',  ( 4.458734124999998549, -73.97916666530106511, -2.574251347313721627 ) ) ;
#63179=CARTESIAN_POINT ( 'NONE',  ( 1.975475456537005874E-15, -109.7499999999999858, 5.000000000000000000 ) ) ;
#63181=CARTESIAN_POINT ( 'NONE',  ( 5.000000000000000000, -20.41666666666666430, -2.886751345948129988 ) ) ;
#63183=ORIENTED_EDGE ( 'NONE', *, *, #38202, .F. ) ;
#63187=( BOUNDED_CURVE ( )  B_SPLINE_CURVE ( 2, ( #40641, #35507, #41265, #55127, #11052, #6242, #45790, #16201, #35829 ),
 .UNSPECIFIED., .F., .F. ) 
 B_SPLINE_CURVE_WITH_KNOTS ( ( 3, 2, 2, 2, 3 ),
 ( 0.9160714285714285365, 0.9166666666666666297, 0.9178571428571428159, 0.9190476190476190022, 0.9196428571428570953 ),
 .UNSPECIFIED. ) 
 CURVE ( )  GEOMETRIC_REPRESENTATION_ITEM ( )  RATIONAL_B_SPLINE_CURVE ( ( 0.9330127018922194093, 0.9330127018922194093, 1.000000000000000000, 0.8660254037844387076, 1.000000000000000000, 0.8660254037844387076, 1.000000000000000000, 0.9330127018922194093, 0.9330127018922194093 ) ) 
 REPRESENTATION_ITEM ( '' )  );
#63188=CARTESIAN_POINT ( 'NONE',  ( -3.535250795749689387E-16, 27.87500000273118417, -5.773502691896257311 ) ) ;
#63196=CARTESIAN_POINT ( 'NONE',  ( 5.000000000000000000, -91.29166666393547303, -2.886751345948130876 ) ) ;
#63198=CARTESIAN_POINT ( 'NONE',  ( -4.458734124999999437, -19.39583333196774007, -2.574251347313719407 ) ) ;
#63199=CARTESIAN_POINT ( 'NONE',  ( -5.000000000000000000, -71.87499999726880162, 0.000000000000000000 ) ) ;
#63203=ORIENTED_EDGE ( 'NONE', *, *, #38743, .F. ) ;
#63206=CARTESIAN_POINT ( 'NONE',  ( -6.972266317189433020E-16, -4.249999999999997335, -5.000000000000000000 ) ) ;
#63207=CARTESIAN_POINT ( 'NONE',  ( -6.972266317189433020E-16, -69.12499999726880162, -5.000000000000000000 ) ) ;
#63209=ORIENTED_EDGE ( 'NONE', *, *, #3884, .T. ) ;
#63216=CARTESIAN_POINT ( 'NONE',  ( -3.152548672688508926E-16, 19.43750000136559208, -5.148502694627439702 ) ) ;
#63218=VERTEX_POINT ( 'NONE', #56318 ) ;
#63221=CARTESIAN_POINT ( 'NONE',  ( 5.000000000000000888, -4.458333330602147981, 2.886751345948126879 ) ) ;
#63224=CARTESIAN_POINT ( 'NONE',  ( -2.229367062499996610, -59.14583333196773651, 3.861377020970582219 ) ) ;
#63226=CARTESIAN_POINT ( 'NONE',  ( -2.229367062500000163, 21.52083333469892779, -3.861377020970580443 ) ) ;
#63228=AXIS2_PLACEMENT_3D ( 'NONE', #986, #58851, #55324 ) ;
#63230=CARTESIAN_POINT ( 'NONE',  ( -2.229367062500000163, -43.72916666530106511, -3.861377020970580443 ) ) ;
#63231=CARTESIAN_POINT ( 'NONE',  ( -2.500000000000000444, -4.041666663935479242, -4.330127018922193649 ) ) ;
#63233=CARTESIAN_POINT ( 'NONE',  ( 6.123233995736766282E-16, -120.0000000000000000, -5.000000000000000000 ) ) ;
#63235=CARTESIAN_POINT ( 'NONE',  ( -2.229367062500000163, -105.4791666653010651, -3.861377020970580443 ) ) ;
#63236=CARTESIAN_POINT ( 'NONE',  ( 2.229367062500001939, -11.22916666530107044, 3.861377020970579999 ) ) ;
#63237=ORIENTED_EDGE ( 'NONE', *, *, #50786, .T. ) ;
#63239=CARTESIAN_POINT ( 'NONE',  ( -2.229367062500000163, -100.4791666653010651, -3.861377020970580443 ) ) ;
#63241=CARTESIAN_POINT ( 'NONE',  ( 4.458734125000001214, -93.14583333196773651, 2.574251347313718519 ) ) ;
#63243=CARTESIAN_POINT ( 'NONE',  ( 2.500000000000002220, -49.54166666393547303, 4.330127018922192761 ) ) ;
#63247=CARTESIAN_POINT ( 'NONE',  ( -4.458734124999997661, -20.22916666530107221, 2.574251347313722516 ) ) ;
#63248=CARTESIAN_POINT ( 'NONE',  ( 9.457646018065525792E-16, 8.687500001365595637, 5.148502694627439702 ) ) ;
#63249=CARTESIAN_POINT ( 'NONE',  ( -2.229367062500000163, -58.72916666530106511, -3.861377020970580443 ) ) ;
#63256=CARTESIAN_POINT ( 'NONE',  ( 0.000000000000000000, -120.0000000000000000, 0.000000000000000000 ) ) ;
#63257=EDGE_CURVE ( 'NONE', #31695, #248, #41177, .T. ) ;
#63258=LINE ( 'NONE', #53599, #37839 ) ;
#63259=CARTESIAN_POINT ( 'NONE',  ( 2.229367062500001939, -82.97916666530106511, 3.861377020970579999 ) ) ;
#63260=CARTESIAN_POINT ( 'NONE',  ( 2.229367062499998831, 20.10416666803225993, -3.861377020970580887 ) ) ;
#63262=CYLINDRICAL_SURFACE ( 'NONE', #10278, 5.000000000000000000 ) ;
#63264=CARTESIAN_POINT ( 'NONE',  ( -6.972266317189433020E-16, -78.24999999999998579, -5.000000000000000000 ) ) ;
#63266=CARTESIAN_POINT ( 'NONE',  ( 1.060575238724906964E-15, -70.74999999999998579, 5.773502691896257311 ) ) ;
#63268=ORIENTED_EDGE ( 'NONE', *, *, #55132, .F. ) ;
#63269=VERTEX_POINT ( 'NONE', #46336 ) ;
#63270=CARTESIAN_POINT ( 'NONE',  ( -2.499999999999996447, -89.83333333333332860, 4.330127018922195425 ) ) ;
#63274=AXIS2_PLACEMENT_3D ( 'NONE', #59603, #15535, #35155 ) ;
#63275=( BOUNDED_CURVE ( )  B_SPLINE_CURVE ( 2, ( #38917, #53718, #62757, #28328, #23517, #19622, #48572, #39233, #57930 ),
 .UNSPECIFIED., .F., .F. ) 
 B_SPLINE_CURVE_WITH_KNOTS ( ( 3, 2, 2, 2, 3 ),
 ( 0.7732142857142857428, 0.7738095238095238360, 0.7750000000000000222, 0.7761904761904762085, 0.7767857142857143016 ),
 .UNSPECIFIED. ) 
 CURVE ( )  GEOMETRIC_REPRESENTATION_ITEM ( )  RATIONAL_B_SPLINE_CURVE ( ( 0.9330127018922194093, 0.9330127018922194093, 1.000000000000000000, 0.8660254037844387076, 1.000000000000000000, 0.8660254037844387076, 1.000000000000000000, 0.9330127018922194093, 0.9330127018922194093 ) ) 
 REPRESENTATION_ITEM ( '' )  );
#63285=CARTESIAN_POINT ( 'NONE',  ( -3.152548672688508926E-16, -56.81249999863439371, -5.148502694627439702 ) ) ;
#63293=CARTESIAN_POINT ( 'NONE',  ( 4.458734124999998549, -103.9791666653010509, -2.574251347313721627 ) ) ;
#63294=CARTESIAN_POINT ( 'NONE',  ( -2.499999999999996447, -68.70833333060214443, 4.330127018922195425 ) ) ;
#63298=CARTESIAN_POINT ( 'NONE',  ( 9.457646018065525792E-16, -39.06249999863440081, 5.148502694627439702 ) ) ;
#63301=CARTESIAN_POINT ( 'NONE',  ( -4.458734124999999437, -14.39583333196773474, -2.574251347313719407 ) ) ;
#63302=CARTESIAN_POINT ( 'NONE',  ( 9.457646018065525792E-16, -103.3124999986344079, 5.148502694627439702 ) ) ;
#63305=CARTESIAN_POINT ( 'NONE',  ( -2.229367062500000163, -30.72916666530107221, -3.861377020970580443 ) ) ;
#63309=CARTESIAN_POINT ( 'NONE',  ( 5.000000000000000000, -17.50000000000000000, -6.123233995736766282E-16 ) ) ;
#63310=CYLINDRICAL_SURFACE ( 'NONE', #23379, 5.000000000000000000 ) ;
#63312=CARTESIAN_POINT ( 'NONE',  ( 9.457646018065525792E-16, 5.687500001365592972, 5.148502694627439702 ) ) ;
#63314=VECTOR ( 'NONE', #21421, 1000.000000000000000 ) ;
#63316=DIRECTION ( 'NONE',  ( -0.000000000000000000, 1.000000000000000000, -0.000000000000000000 ) ) ;
#63317=CARTESIAN_POINT ( 'NONE',  ( 5.000000000000000888, -97.58333333333332860, 2.886751345948126879 ) ) ;
#63318=CARTESIAN_POINT ( 'NONE',  ( -2.229367062500000163, -30.47916666530107221, -3.861377020970580443 ) ) ;
#63319=CARTESIAN_POINT ( 'NONE',  ( 1.339745962155615144, -73.70534180126146850, 4.999999999999999112 ) ) ;
#63320=CARTESIAN_POINT ( 'NONE',  ( -2.229367062500000163, -73.72916666530106511, -3.861377020970580443 ) ) ;
#63321=VECTOR ( 'NONE', #34353, 1000.000000000000000 ) ;
#63323=CARTESIAN_POINT ( 'NONE',  ( -4.999999999999998224, -101.7916666639354446, 2.886751345948131764 ) ) ;
#63328=CARTESIAN_POINT ( 'NONE',  ( -4.458734124999999437, -4.312499998634401699, 0.000000000000000000 ) ) ;
#63329=CARTESIAN_POINT ( 'NONE',  ( 4.458734125000001214, 28.85416666803225993, 2.574251347313718519 ) ) ;
#63330=CARTESIAN_POINT ( 'NONE',  ( -4.458734124999999437, -40.56249999863440081, 0.000000000000000000 ) ) ;
#63337=CARTESIAN_POINT ( 'NONE',  ( 4.458734124999999437, -71.81249999863439371, -5.460374474430324690E-16 ) ) ;
#63338=CARTESIAN_POINT ( 'NONE',  ( 2.499999999999998668, -104.2083333306021444, -4.330127018922193649 ) ) ;
#63341=CARTESIAN_POINT ( 'NONE',  ( 0.000000000000000000, -120.0000000000000000, 0.000000000000000000 ) ) ;
#63345=CARTESIAN_POINT ( 'NONE',  ( -3.535250795749689387E-16, -52.25000000000001421, -5.773502691896257311 ) ) ;
#63349=CARTESIAN_POINT ( 'NONE',  ( 1.975475456537005874E-15, -26.74999999999999645, 5.000000000000000000 ) ) ;
#63350=LINE ( 'NONE', #18648, #25760 ) ;
#63357=ORIENTED_EDGE ( 'NONE', *, *, #9875, .F. ) ;
#63358=CARTESIAN_POINT ( 'NONE',  ( 5.000000000000000000, 5.583333333333332149, -2.886751345948130876 ) ) ;
#63359=CARTESIAN_POINT ( 'NONE',  ( 1.975475456537005874E-15, -98.74999999999998579, 5.000000000000000000 ) ) ;
#63366=CARTESIAN_POINT ( 'NONE',  ( 4.458734125000001214, -40.14583333196772941, 2.574251347313718519 ) ) ;
#63369=CARTESIAN_POINT ( 'NONE',  ( -4.999999999999998224, -29.91666666666667140, 2.886751345948131764 ) ) ;
#63373=VECTOR ( 'NONE', #33336, 1000.000000000000000 ) ;
#63376=CARTESIAN_POINT ( 'NONE',  ( -3.152548672688508926E-16, -87.81249999863439371, -5.148502694627439702 ) ) ;
#63377=DIRECTION ( 'NONE',  ( -0.000000000000000000, 1.000000000000000000, -0.000000000000000000 ) ) ;
#63379=CARTESIAN_POINT ( 'NONE',  ( -1.339745962155613812, -47.20534180126147561, -5.000000000000000000 ) ) ;
#63382=( BOUNDED_CURVE ( )  B_SPLINE_CURVE ( 2, ( #34169, #37202, #3424, #9411, #4588, #23040, #24531, #38997, #47168 ),
 .UNSPECIFIED., .F., .F. ) 
 B_SPLINE_CURVE_WITH_KNOTS ( ( 3, 2, 2, 2, 3 ),
 ( 0.7017857142857142350, 0.7023809523809523281, 0.7035714285714286254, 0.7047619047619048116, 0.7053571428571429047 ),
 .UNSPECIFIED. ) 
 CURVE ( )  GEOMETRIC_REPRESENTATION_ITEM ( )  RATIONAL_B_SPLINE_CURVE ( ( 0.9330127018922194093, 0.9330127018922194093, 1.000000000000000000, 0.8660254037844387076, 1.000000000000000000, 0.8660254037844387076, 1.000000000000000000, 0.9330127018922194093, 0.9330127018922194093 ) ) 
 REPRESENTATION_ITEM ( '' )  );
#63385=CARTESIAN_POINT ( 'NONE',  ( -5.000000000000000000, -70.95833333060214443, -2.886751345948128211 ) ) ;
#63386=CARTESIAN_POINT ( 'NONE',  ( 2.229367062500001939, -11.22916666530107044, 3.861377020970579999 ) ) ;
#63387=CARTESIAN_POINT ( 'NONE',  ( 5.000000000000000000, -105.3749999972688158, -6.123233995736766282E-16 ) ) ;
#63391=CARTESIAN_POINT ( 'NONE',  ( -4.458734124999999437, 20.35416666803225993, -2.574251347313719407 ) ) ;
#63392=EDGE_LOOP ( 'NONE', ( #29008, #30614, #62231, #17518 ) ) ;
#63393=CARTESIAN_POINT ( 'NONE',  ( -4.458734124999999437, -91.39583333196773651, -2.574251347313719407 ) ) ;
#63396=CARTESIAN_POINT ( 'NONE',  ( 4.458734124999999437, -14.81249999863440436, -5.460374474430324690E-16 ) ) ;
#63397=DIRECTION ( 'NONE',  ( 0.000000000000000000, 0.000000000000000000, 1.000000000000000000 ) ) ;
#63400=EDGE_CURVE ( 'NONE', #19094, #45889, #51797, .T. ) ;
#63401=CARTESIAN_POINT ( 'NONE',  ( 5.000000000000000000, -41.29166666393548013, -2.886751345948129988 ) ) ;
#63403=CARTESIAN_POINT ( 'NONE',  ( 9.457646018065525792E-16, 19.93750000136559208, 5.148502694627439702 ) ) ;
#63405=ORIENTED_EDGE ( 'NONE', *, *, #5996, .T. ) ;
#63407=CARTESIAN_POINT ( 'NONE',  ( 4.458734124999998549, -59.72916666530106511, -2.574251347313721627 ) ) ;
#63409=AXIS2_PLACEMENT_3D ( 'NONE', #56918, #12836, #8342 ) ;
#63410=DIRECTION ( 'NONE',  ( -0.000000000000000000, 1.000000000000000000, -0.000000000000000000 ) ) ;
#63411=CARTESIAN_POINT ( 'NONE',  ( 5.000000000000000000, 8.583333333333330373, -2.886751345948129988 ) ) ;
#63413=CARTESIAN_POINT ( 'NONE',  ( -2.499999999999996447, -98.70833333060214443, 4.330127018922195425 ) ) ;
#63414=CARTESIAN_POINT ( 'NONE',  ( -4.458734124999999437, -51.31249999863440792, 0.000000000000000000 ) ) ;
#63415=CARTESIAN_POINT ( 'NONE',  ( 2.500000000000002220, -90.54166666393547303, 4.330127018922192761 ) ) ;
#63417=VECTOR ( 'NONE', #20605, 1000.000000000000000 ) ;
#63418=DIRECTION ( 'NONE',  ( -0.000000000000000000, 1.000000000000000000, -0.000000000000000000 ) ) ;
#63419=CARTESIAN_POINT ( 'NONE',  ( 4.458734125000000326, -91.14583333196773651, 2.574251347313718519 ) ) ;
#63421=CARTESIAN_POINT ( 'NONE',  ( -4.999999999999999112, -36.91666666666667140, 2.886751345948131764 ) ) ;
#63423=EDGE_CURVE ( 'NONE', #53577, #19571, #41002, .T. ) ;
#63426=CARTESIAN_POINT ( 'NONE',  ( 4.458734125000001214, -101.8958333319677365, 2.574251347313718519 ) ) ;
#63427=CARTESIAN_POINT ( 'NONE',  ( 9.457646018065525792E-16, 3.687500001365594748, 5.148502694627439702 ) ) ;
#63437=CARTESIAN_POINT ( 'NONE',  ( -6.972266317189433020E-16, -48.12499999726880873, -5.000000000000000000 ) ) ;
#63438=LINE ( 'NONE', #19035, #36419 ) ;
#63439=CARTESIAN_POINT ( 'NONE',  ( -2.499999999999996447, 25.16666666666666430, 4.330127018922195425 ) ) ;
#63442=CARTESIAN_POINT ( 'NONE',  ( 4.458734125000001214, -25.14583333196774007, 2.574251347313718519 ) ) ;
#63450=ORIENTED_EDGE ( 'NONE', *, *, #15706, .T. ) ;
#63451=DIRECTION ( 'NONE',  ( 0.000000000000000000, 0.000000000000000000, 1.000000000000000000 ) ) ;
#63452=ORIENTED_EDGE ( 'NONE', *, *, #13286, .T. ) ;
#63453=CARTESIAN_POINT ( 'NONE',  ( -4.458734124999998549, -74.47916666530106511, 2.574251347313722516 ) ) ;
#63455=VERTEX_POINT ( 'NONE', #22647 ) ;
#63459=VECTOR ( 'NONE', #28356, 1000.000000000000000 ) ;
#63460=CARTESIAN_POINT ( 'NONE',  ( 2.229367062499998831, 4.104166668032260823, -3.861377020970580887 ) ) ;
#63461=EDGE_LOOP ( 'NONE', ( #813, #18712, #30584, #33245 ) ) ;
#63462=( BOUNDED_CURVE ( )  B_SPLINE_CURVE ( 2, ( #1042, #26413, #11291, #20648, #50543, #26097, #60521, #40252, #15812 ),
 .UNSPECIFIED., .F., .F. ) 
 B_SPLINE_CURVE_WITH_KNOTS ( ( 3, 2, 2, 2, 3 ),
 ( 0.2589285714285714524, 0.2595238095238095455, 0.2607142857142857317, 0.2619047619047619180, 0.2625000000000000111 ),
 .UNSPECIFIED. ) 
 CURVE ( )  GEOMETRIC_REPRESENTATION_ITEM ( )  RATIONAL_B_SPLINE_CURVE ( ( 0.9330127018922194093, 0.9330127018922194093, 1.000000000000000000, 0.8660254037844387076, 1.000000000000000000, 0.8660254037844387076, 1.000000000000000000, 0.9330127018922194093, 0.9330127018922194093 ) ) 
 REPRESENTATION_ITEM ( '' )  );
#63463=CYLINDRICAL_SURFACE ( 'NONE', #63539, 5.000000000000000000 ) ;
#63466=CARTESIAN_POINT ( 'NONE',  ( 5.000000000000000888, -92.45833333060213022, 2.886751345948126879 ) ) ;
#63468=EDGE_LOOP ( 'NONE', ( #5796, #50078, #59473, #29114 ) ) ;
#63469=CARTESIAN_POINT ( 'NONE',  ( 9.457646018065525792E-16, -75.06249999863440792, 5.148502694627439702 ) ) ;
#63471=CARTESIAN_POINT ( 'NONE',  ( 4.458734124999999437, 1.187500001365596081, -5.460374474430324690E-16 ) ) ;
#63473=CARTESIAN_POINT ( 'NONE',  ( 1.975475456537005874E-15, -42.62499999726880873, 5.000000000000000000 ) ) ;
#63474=CARTESIAN_POINT ( 'NONE',  ( 9.457646018065525792E-16, -66.31249999863440792, 5.148502694627439702 ) ) ;
#63475=CARTESIAN_POINT ( 'NONE',  ( -4.999999999999999112, -23.79166666393548013, 2.886751345948131764 ) ) ;
#63476=CARTESIAN_POINT ( 'NONE',  ( 1.975475456537005874E-15, 24.24999999999999645, 5.000000000000000000 ) ) ;
#63479=CARTESIAN_POINT ( 'NONE',  ( -4.458734124999999437, -44.31249999863440081, 0.000000000000000000 ) ) ;
#63480=CARTESIAN_POINT ( 'NONE',  ( 2.229367062499998831, -24.89583333196773651, -3.861377020970580887 ) ) ;
#63482=LINE ( 'NONE', #62228, #42280 ) ;
#63483=CARTESIAN_POINT ( 'NONE',  ( 5.000000000000000888, 25.41666666666666430, 2.886751345948126879 ) ) ;
#63486=CARTESIAN_POINT ( 'NONE',  ( -4.458734124999998549, -39.22916666530107221, 2.574251347313722516 ) ) ;
#63487=CARTESIAN_POINT ( 'NONE',  ( 2.500000000000002220, -71.54166666393547303, 4.330127018922192761 ) ) ;
#63490=CARTESIAN_POINT ( 'NONE',  ( -4.458734124999999437, -74.64583333196773651, -2.574251347313719407 ) ) ;
#63494=CYLINDRICAL_SURFACE ( 'NONE', #33830, 5.000000000000000000 ) ;
#63495=CARTESIAN_POINT ( 'NONE',  ( 2.499999999999998668, -21.33333333333333570, -4.330127018922193649 ) ) ;
#63502=CARTESIAN_POINT ( 'NONE',  ( -2.499999999999996447, 27.29166666939785202, 4.330127018922195425 ) ) ;
#63505=CARTESIAN_POINT ( 'NONE',  ( 6.158835246850667461E-14, 7.875000002731183280, -4.999999999999999112 ) ) ;
#63509=CARTESIAN_POINT ( 'NONE',  ( 2.500000000000002220, -89.54166666393547303, 4.330127018922192761 ) ) ;
#63511=CARTESIAN_POINT ( 'NONE',  ( 0.000000000000000000, -120.0000000000000000, 0.000000000000000000 ) ) ;
#63512=CARTESIAN_POINT ( 'NONE',  ( 4.458734125000001214, -20.89583333196774007, 2.574251347313718519 ) ) ;
#63521=CARTESIAN_POINT ( 'NONE',  ( -4.999999999999998224, -2.916666666666664742, 2.886751345948131764 ) ) ;
#63523=ORIENTED_EDGE ( 'NONE', *, *, #5618, .F. ) ;
#63525=( BOUNDED_CURVE ( )  B_SPLINE_CURVE ( 2, ( #20098, #44538, #19137, #494, #39704, #59344, #38754, #28486, #19460 ),
 .UNSPECIFIED., .F., .F. ) 
 B_SPLINE_CURVE_WITH_KNOTS ( ( 3, 2, 2, 2, 3 ),
 ( 0.4946428571428571619, 0.4952380952380952550, 0.4964285714285714413, 0.4976190476190476275, 0.4982142857142857206 ),
 .UNSPECIFIED. ) 
 CURVE ( )  GEOMETRIC_REPRESENTATION_ITEM ( )  RATIONAL_B_SPLINE_CURVE ( ( 0.9330127018922194093, 0.9330127018922194093, 1.000000000000000000, 0.8660254037844387076, 1.000000000000000000, 0.8660254037844387076, 1.000000000000000000, 0.9330127018922194093, 0.9330127018922194093 ) ) 
 REPRESENTATION_ITEM ( '' )  );
#63526=CARTESIAN_POINT ( 'NONE',  ( 1.339745962155612702, -23.16965819600733312, -5.000000000000000000 ) ) ;
#63532=CARTESIAN_POINT ( 'NONE',  ( 2.229367062500001939, 21.02083333469892779, 3.861377020970579999 ) ) ;
#63534=ORIENTED_EDGE ( 'NONE', *, *, #3671, .F. ) ;
#63539=AXIS2_PLACEMENT_3D ( 'NONE', #11317, #6511, #26123 ) ;
#63541=CARTESIAN_POINT ( 'NONE',  ( -3.152548672688508926E-16, -58.56249999863439371, -5.148502694627439702 ) ) ;
#63543=CARTESIAN_POINT ( 'NONE',  ( -4.458734124999999437, 17.68750000136559208, 0.000000000000000000 ) ) ;
#63546=CARTESIAN_POINT ( 'NONE',  ( -2.229367062500000163, -47.72916666530106511, -3.861377020970580443 ) ) ;
#63547=CARTESIAN_POINT ( 'NONE',  ( 5.000000000000000888, -10.45833333060214621, 2.886751345948126879 ) ) ;
#63548=CARTESIAN_POINT ( 'NONE',  ( 5.000000000000000000, -31.41666666666667140, -2.886751345948130876 ) ) ;
#63550=CYLINDRICAL_SURFACE ( 'NONE', #36643, 5.000000000000000000 ) ;
#63551=CARTESIAN_POINT ( 'NONE',  ( -4.458734124999999437, -108.3124999986343937, 0.000000000000000000 ) ) ;
#63553=( BOUNDED_CURVE ( )  B_SPLINE_CURVE ( 2, ( #28107, #19395, #14563, #37768, #9739, #29343, #48977, #57399, #32941 ),
 .UNSPECIFIED., .F., .F. ) 
 B_SPLINE_CURVE_WITH_KNOTS ( ( 3, 2, 2, 2, 3 ),
 ( 0.4089285714285714191, 0.4095238095238095122, 0.4107142857142856984, 0.4119047619047618847, 0.4124999999999999778 ),
 .UNSPECIFIED. ) 
 CURVE ( )  GEOMETRIC_REPRESENTATION_ITEM ( )  RATIONAL_B_SPLINE_CURVE ( ( 0.9330127018922194093, 0.9330127018922194093, 1.000000000000000000, 0.8660254037844387076, 1.000000000000000000, 0.8660254037844387076, 1.000000000000000000, 0.9330127018922194093, 0.9330127018922194093 ) ) 
 REPRESENTATION_ITEM ( '' )  );
#63554=CARTESIAN_POINT ( 'NONE',  ( -4.458734124999999437, -8.562499998634406140, 0.000000000000000000 ) ) ;
#63555=ORIENTED_EDGE ( 'NONE', *, *, #21984, .F. ) ;
#63557=CARTESIAN_POINT ( 'NONE',  ( -4.458734124999999437, -96.31249999863440792, 0.000000000000000000 ) ) ;
#63559=CARTESIAN_POINT ( 'NONE',  ( -3.152548672688508926E-16, -96.81249999863440792, -5.148502694627439702 ) ) ;
#63560=LINE ( 'NONE', #50024, #48969 ) ;
#63561=CARTESIAN_POINT ( 'NONE',  ( 2.500000000000002220, -51.54166666393547303, 4.330127018922192761 ) ) ;
#63562=CARTESIAN_POINT ( 'NONE',  ( -1.339745962155613812, -37.08034179853029144, -5.000000000000000000 ) ) ;
#63565=CARTESIAN_POINT ( 'NONE',  ( 4.458734124999999437, -16.81249999863440436, -5.460374474430324690E-16 ) ) ;
#63566=CARTESIAN_POINT ( 'NONE',  ( -4.458734124999998549, 9.520833334698927786, 2.574251347313722516 ) ) ;
#63567=CARTESIAN_POINT ( 'NONE',  ( -2.229367062500000163, -59.72916666530106511, -3.861377020970580443 ) ) ;
#63570=CARTESIAN_POINT ( 'NONE',  ( 5.000000000000000888, -8.458333330602144429, 2.886751345948126879 ) ) ;
#63572=CARTESIAN_POINT ( 'NONE',  ( -2.499999999999996447, -6.833333333333330373, 4.330127018922195425 ) ) ;
#63576=CARTESIAN_POINT ( 'NONE',  ( 5.000000000000000000, -66.41666666666667140, -2.886751345948130876 ) ) ;
#63577=FACE_OUTER_BOUND ( 'NONE', #36612, .T. ) ;
#63578=CARTESIAN_POINT ( 'NONE',  ( -2.229367062500000163, -83.47916666530106511, -3.861377020970580443 ) ) ;
#63579=CARTESIAN_POINT ( 'NONE',  ( -2.229367062500000163, 19.27083333469892779, -3.861377020970580443 ) ) ;
#63581=CARTESIAN_POINT ( 'NONE',  ( -1.339745962155613812, -48.20534180126148271, -5.000000000000000000 ) ) ;
#63585=CARTESIAN_POINT ( 'NONE',  ( 5.000000000000000000, -77.50000000000000000, -6.123233995736766282E-16 ) ) ;
#63587=ORIENTED_EDGE ( 'NONE', *, *, #14160, .T. ) ;
#63596=VERTEX_POINT ( 'NONE', #18436 ) ;
#63603=CARTESIAN_POINT ( 'NONE',  ( -4.458734124999999437, -57.64583333196773651, -2.574251347313719407 ) ) ;
#63605=CARTESIAN_POINT ( 'NONE',  ( 5.000000000000000888, 3.541666669397852019, 2.886751345948126879 ) ) ;
#63606=ORIENTED_EDGE ( 'NONE', *, *, #5070, .T. ) ;
#63610=ORIENTED_EDGE ( 'NONE', *, *, #61924, .F. ) ;
#63612=CARTESIAN_POINT ( 'NONE',  ( -4.458734124999999437, -107.5624999986343937, 0.000000000000000000 ) ) ;
#63614=ORIENTED_EDGE ( 'NONE', *, *, #14250, .F. ) ;
#63617=CARTESIAN_POINT ( 'NONE',  ( -2.229367062500000163, -39.47916666530107221, -3.861377020970580443 ) ) ;
#63620=CARTESIAN_POINT ( 'NONE',  ( 1.339745962155613146, 29.70534180126147561, -4.999999999999999112 ) ) ;
#63621=CARTESIAN_POINT ( 'NONE',  ( 2.229367062499998831, -13.64583333196774184, -3.861377020970580887 ) ) ;
#63622=CARTESIAN_POINT ( 'NONE',  ( -2.229367062500000163, -98.72916666530105090, -3.861377020970580443 ) ) ;
#63623=ORIENTED_EDGE ( 'NONE', *, *, #15502, .T. ) ;
#63624=EDGE_CURVE ( 'NONE', #24216, #7754, #7770, .T. ) ;
#63626=CARTESIAN_POINT ( 'NONE',  ( 4.458734124999998549, -30.97916666530107577, -2.574251347313721627 ) ) ;
#63627=EDGE_CURVE ( 'NONE', #2700, #39916, #23269, .T. ) ;
#63633=CARTESIAN_POINT ( 'NONE',  ( 0.000000000000000000, -120.0000000000000000, 0.000000000000000000 ) ) ;
#63635=CARTESIAN_POINT ( 'NONE',  ( -3.152548672688508926E-16, 7.187500001365594748, -5.148502694627439702 ) ) ;
#63636=ORIENTED_EDGE ( 'NONE', *, *, #24773, .T. ) ;
#63637=CARTESIAN_POINT ( 'NONE',  ( 1.339745962155615144, 2.294658198738519950, 4.999999999999999112 ) ) ;
#63638=CARTESIAN_POINT ( 'NONE',  ( 5.000000000000000000, -95.50000000000000000, -6.123233995736766282E-16 ) ) ;
#63639=CARTESIAN_POINT ( 'NONE',  ( 9.457646018065525792E-16, -29.06249999863440081, 5.148502694627439702 ) ) ;
#63640=CYLINDRICAL_SURFACE ( 'NONE', #53123, 5.000000000000000000 ) ;
#63641=CARTESIAN_POINT ( 'NONE',  ( -2.229367062499996610, -78.39583333196773651, 3.861377020970582219 ) ) ;
#63642=AXIS2_PLACEMENT_3D ( 'NONE', #4170, #23785, #43387 ) ;
#63644=LINE ( 'NONE', #59130, #8910 ) ;
#63647=CARTESIAN_POINT ( 'NONE',  ( 9.457646018065525792E-16, -0.06249999863440491854, 5.148502694627439702 ) ) ;
#63648=CARTESIAN_POINT ( 'NONE',  ( 2.229367062500001939, 24.77083333469892779, 3.861377020970579999 ) ) ;
#63649=CARTESIAN_POINT ( 'NONE',  ( 9.457646018065525792E-16, -45.31249999863440081, 5.148502694627439702 ) ) ;
#63654=CARTESIAN_POINT ( 'NONE',  ( 4.458734124999999437, -68.81249999863439371, -5.460374474430324690E-16 ) ) ;
#63655=CARTESIAN_POINT ( 'NONE',  ( -4.999999999999999112, -103.7916666639354730, 2.886751345948131764 ) ) ;
#63658=CARTESIAN_POINT ( 'NONE',  ( -4.999999999999998224, 10.08333333333333393, 2.886751345948131764 ) ) ;
#63659=ADVANCED_FACE ( 'NONE', ( #32919 ), #52223, .T. ) ;
#63660=CARTESIAN_POINT ( 'NONE',  ( -4.458734124999997661, -110.4791666653010793, 2.574251347313722516 ) ) ;
#63662=CARTESIAN_POINT ( 'NONE',  ( 5.000000000000000000, -55.49999999999999289, -6.123233995736766282E-16 ) ) ;
#63663=CARTESIAN_POINT ( 'NONE',  ( 0.000000000000000000, -120.0000000000000000, 0.000000000000000000 ) ) ;
#63664=DIRECTION ( 'NONE',  ( 0.000000000000000000, 0.000000000000000000, 1.000000000000000000 ) ) ;
#63665=VERTEX_POINT ( 'NONE', #13295 ) ;
#63666=CARTESIAN_POINT ( 'NONE',  ( -2.499999999999996447, -26.83333333333333570, 4.330127018922195425 ) ) ;
#63699=COLOUR_RGB('Sky Blue',0.24,0.69,0.87);
#63700=FILL_AREA_STYLE_COLOUR('',#63699);
#63701=FILL_AREA_STYLE('',(#63700));
#63702=SURFACE_STYLE_FILL_AREA(#63701);
#63703=SURFACE_SIDE_STYLE('',(#63702));
#63704=SURFACE_STYLE_USAGE(.BOTH.,#63703);
#63705=PRESENTATION_STYLE_ASSIGNMENT((#63704));
ENDSEC;
END-ISO-10303-21;
